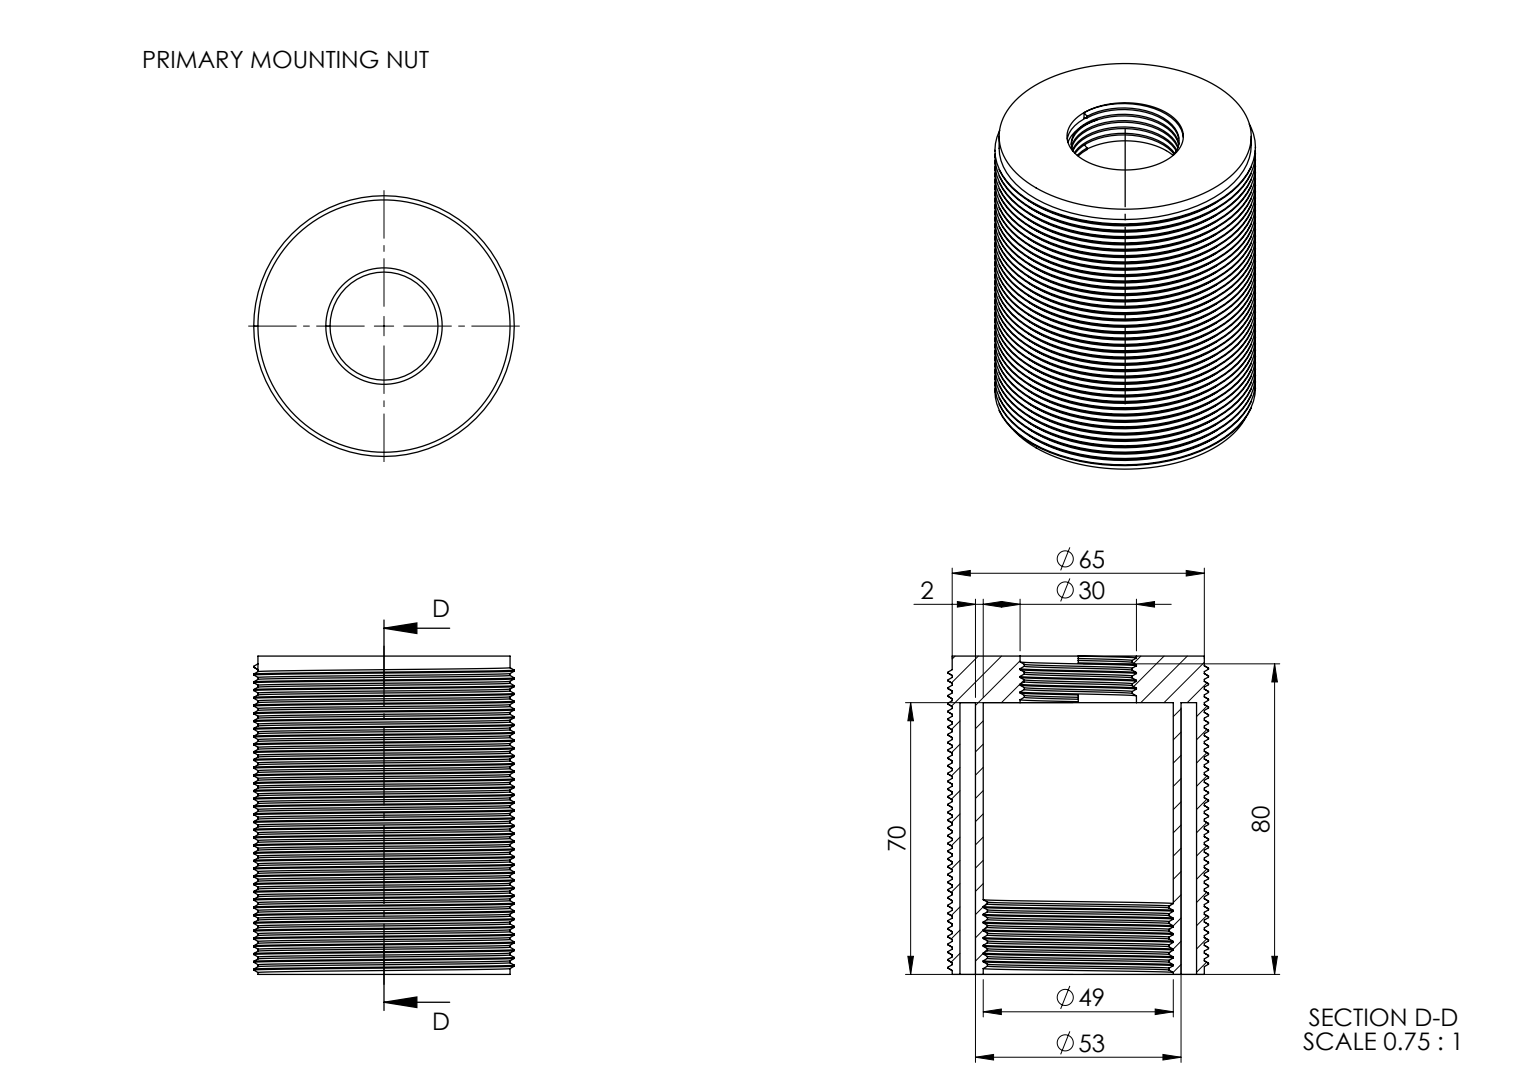
ISO-10303-21;
HEADER;
FILE_DESCRIPTION (('STEP AP214'),
    '1' );
FILE_NAME ('primary mounting nut.step',
    '2026-10-02T18:08:48',
    ( '' ),
    ( '' ),
    'SwSTEP 2.0',
    'SolidWorks 2026',
    '' );
FILE_SCHEMA (( 'AUTOMOTIVE_DESIGN' ));
ENDSEC;

DATA;
#4=ORIENTED_EDGE ( 'NONE', *, *, #32426, .T. ) ;
#10=CARTESIAN_POINT ( 'NONE',  ( -2.162160676586881955E-15, 52.87500000273119838, -35.31076352940723240 ) ) ;
#11=CARTESIAN_POINT ( 'NONE',  ( -2.092463501923844636E-15, 58.00000000546235412, -34.17252228774368916 ) ) ;
#14=CARTESIAN_POINT ( 'NONE',  ( -2.162160676586881955E-15, 42.62500000273119838, -35.31076352940723240 ) ) ;
#15=CARTESIAN_POINT ( 'NONE',  ( -4.635254915624208216, 72.40000000000001990, 14.26584774442730463 ) ) ;
#16=CARTESIAN_POINT ( 'NONE',  ( 33.58253175000000113, 68.47500000273119269, -10.91162601494193751 ) ) ;
#21=CARTESIAN_POINT ( 'NONE',  ( 6.277390505771533514E-15, 44.49999999999999289, 34.17252228774368916 ) ) ;
#23=CARTESIAN_POINT ( 'NONE',  ( -10.37757302488624411, 12.97500000273119092, -31.93888565452638417 ) ) ;
#27=CARTESIAN_POINT ( 'NONE',  ( 15.00000000000000355, 75.15000000546237402, 4.873795443493592394 ) ) ;
#28=CARTESIAN_POINT ( 'NONE',  ( 0.000000000000000000, 82.00000000000001421, 0.000000000000000000 ) ) ;
#30=EDGE_LOOP ( 'NONE', ( #10708, #16576, #32789, #18480 ) ) ;
#33=EDGE_CURVE ( 'NONE', #10375, #21334, #32773, .T. ) ;
#41=( BOUNDED_CURVE ( )  B_SPLINE_CURVE ( 2, ( #27655, #11863, #29882, #19433, #17198, #32453, #30382, #1391, #9453, #17026, #24905, #17535, #22341 ),
 .UNSPECIFIED., .F., .T. ) 
 B_SPLINE_CURVE_WITH_KNOTS ( ( 3, 2, 2, 2, 2, 2, 3 ),
 ( 0.2756410256410256610, 0.2769230769230769384, 0.2794871794871794934, 0.2820512820512820484, 0.2846153846153846034, 0.2871794871794871584, 0.2884615384615384914 ),
 .UNSPECIFIED. ) 
 CURVE ( )  GEOMETRIC_REPRESENTATION_ITEM ( )  RATIONAL_B_SPLINE_CURVE ( ( 0.9755282581475768211, 0.9755282581475768211, 1.000000000000000000, 0.9510565162951535312, 1.000000000000000000, 0.9510565162951535312, 1.000000000000000000, 0.9510565162951535312, 1.000000000000000000, 0.9510565162951535312, 1.000000000000000000, 0.9755282581475762660, 0.9755282581475768211 ) ) 
 REPRESENTATION_ITEM ( '' )  );
#43=CARTESIAN_POINT ( 'NONE',  ( 27.16883889988623935, 38.32500000273120122, -19.73931689729374384 ) ) ;
#46=CARTESIAN_POINT ( 'NONE',  ( -5.147494310547430452, 2.051254287009222299, -32.49999999999999289 ) ) ;
#49=CARTESIAN_POINT ( 'NONE',  ( -12.13525491562420910, 70.45000000546237118, 8.816778784387098611 ) ) ;
#51=CARTESIAN_POINT ( 'NONE',  ( 10.37757302488624056, 76.77500000273118985, -31.93888565452638417 ) ) ;
#57=CARTESIAN_POINT ( 'NONE',  ( -2.162160676586881955E-15, 60.62500000273117706, -35.31076352940723240 ) ) ;
#59=CARTESIAN_POINT ( 'NONE',  ( -5.147494310547423346, 66.94874572391552192, 32.50000000000000000 ) ) ;
#60=CARTESIAN_POINT ( 'NONE',  ( 14.47279130897151767, 8.824999997268804464, 19.92008829642072953 ) ) ;
#61=CARTESIAN_POINT ( 'NONE',  ( 27.16883889988624290, 1.925000002731186433, 19.73931689729373673 ) ) ;
#62=CARTESIAN_POINT ( 'NONE',  ( -1.778240108872766143E-15, 8.000000005462370112, -32.49999999999999289 ) ) ;
#65=CARTESIAN_POINT ( 'NONE',  ( -15.00000000000000000, 80.25000000546239676, 0.000000000000000000 ) ) ;
#67=CARTESIAN_POINT ( 'NONE',  ( -5.147494310547423346, 4.448745718453162468, 32.50000000000000000 ) ) ;
#71=CARTESIAN_POINT ( 'NONE',  ( 9.270509831248423538, 73.55000000546237970, -12.75976212528059861 ) ) ;
#73=CARTESIAN_POINT ( 'NONE',  ( 6.486482029760649416E-15, 29.62500000273120193, 35.31076352940723240 ) ) ;
#75=AXIS2_PLACEMENT_3D ( 'NONE', #28014, #5016, #30577 ) ;
#77=CARTESIAN_POINT ( 'NONE',  ( -2.162160676586882350E-15, 12.87500000273117884, -35.31076352940722529 ) ) ;
#78=PRODUCT_DEFINITION ( 'UNKNOWN', '', #3307, #996 ) ;
#79=CARTESIAN_POINT ( 'NONE',  ( -10.04305231718579172, 63.59999999999998721, -30.90933677959248982 ) ) ;
#81=CARTESIAN_POINT ( 'NONE',  ( -27.16883889988623935, 75.32500000273117280, 19.73931689729374739 ) ) ;
#82=CARTESIAN_POINT ( 'NONE',  ( 3.880418787951153803, 7.551254281546842861, 24.49999999999999645 ) ) ;
#84=CARTESIAN_POINT ( 'NONE',  ( 1.507698388325705758E-15, 17.12499999726880517, -24.62258325217400312 ) ) ;
#85=CARTESIAN_POINT ( 'NONE',  ( 33.58253175000000113, 58.12500000273118417, -4.112674001490185761E-15 ) ) ;
#87=ORIENTED_EDGE ( 'NONE', *, *, #10321, .T. ) ;
#89=CARTESIAN_POINT ( 'NONE',  ( 33.58253175000000113, 6.225000002731185589, -10.91162601494193574 ) ) ;
#90=CARTESIAN_POINT ( 'NONE',  ( -7.236395654485763274, 16.52499999726880731, 22.27133577429736633 ) ) ;
#92=EDGE_LOOP ( 'NONE', ( #2130, #17184, #1564 ) ) ;
#94=ORIENTED_EDGE ( 'NONE', *, *, #21026, .F. ) ;
#98=CARTESIAN_POINT ( 'NONE',  ( -20.75514604977248112, 77.42500000273119554, 28.56700777964554661 ) ) ;
#100=CARTESIAN_POINT ( 'NONE',  ( 1.577395562988744260E-15, 2.500000000000008882, -25.76082449383753925 ) ) ;
#101=CARTESIAN_POINT ( 'NONE',  ( 27.16883889988623935, 12.57500000273120655, -19.73931689729374384 ) ) ;
#102=CARTESIAN_POINT ( 'NONE',  ( 26.29305231718578995, 59.20000000000000284, -19.10302069950538240 ) ) ;
#103=CARTESIAN_POINT ( 'NONE',  ( 10.04305231718578817, 73.90000000546237402, -30.90933677959249337 ) ) ;
#105=CARTESIAN_POINT ( 'NONE',  ( -11.25946833292375793, 75.57500000273120122, 8.180482586598737171 ) ) ;
#107=CARTESIAN_POINT ( 'NONE',  ( 0.000000000000000000, 82.00000000000001421, 0.000000000000000000 ) ) ;
#108=CARTESIAN_POINT ( 'NONE',  ( -24.50000000000000000, 12.90000000000000036, -7.960532557706207157 ) ) ;
#109=CARTESIAN_POINT ( 'NONE',  ( 32.50000000000000711, 4.899999999999989697, 10.55989012756945122 ) ) ;
#112=CARTESIAN_POINT ( 'NONE',  ( 27.16883889988624290, 47.92500000273120264, 19.73931689729373673 ) ) ;
#114=CARTESIAN_POINT ( 'NONE',  ( -27.16883889988623935, 33.57500000273120122, 19.73931689729374739 ) ) ;
#117=CARTESIAN_POINT ( 'NONE',  ( 5.147494310547434893, 15.05125428700922541, 32.49999999999999289 ) ) ;
#118=CARTESIAN_POINT ( 'NONE',  ( -1.778240108872766143E-15, 22.00000000546237899, -32.49999999999999289 ) ) ;
#121=DIRECTION ( 'NONE',  ( -0.000000000000000000, 1.000000000000000000, -0.000000000000000000 ) ) ;
#124=CARTESIAN_POINT ( 'NONE',  ( -10.04305231718578462, 40.39999999999999147, 30.90933677959249337 ) ) ;
#127=CARTESIAN_POINT ( 'NONE',  ( 5.779280353836490358E-15, 12.49999999999999112, 32.49999999999999289 ) ) ;
#128=CARTESIAN_POINT ( 'NONE',  ( 10.37757302488624056, 26.52500000273119696, -31.93888565452638417 ) ) ;
#132=EDGE_CURVE ( 'NONE', #774, #12058, #32938, .T. ) ;
#138=CARTESIAN_POINT ( 'NONE',  ( -23.41746825000000243, 1.524999997268801755, -7.608796670333730638 ) ) ;
#139=CARTESIAN_POINT ( 'NONE',  ( 33.58253175000000113, 32.37500000273119127, -4.112674001490185761E-15 ) ) ;
#140=CARTESIAN_POINT ( 'NONE',  ( -32.50000000000000000, 36.40000000546236691, -10.55989012756945478 ) ) ;
#141=( BOUNDED_CURVE ( )  B_SPLINE_CURVE ( 2, ( #20409, #30859, #4610, #33262, #20067, #17493, #25204, #17837, #11988, #19888, #1681, #4780, #33084 ),
 .UNSPECIFIED., .F., .T. ) 
 B_SPLINE_CURVE_WITH_KNOTS ( ( 3, 2, 2, 2, 2, 2, 3 ),
 ( 0.2243589743589743668, 0.2256410256410256443, 0.2282051282051281993, 0.2307692307692307820, 0.2333333333333333370, 0.2358974358974358920, 0.2371794871794871973 ),
 .UNSPECIFIED. ) 
 CURVE ( )  GEOMETRIC_REPRESENTATION_ITEM ( )  RATIONAL_B_SPLINE_CURVE ( ( 0.9755282581475768211, 0.9755282581475768211, 1.000000000000000000, 0.9510565162951535312, 1.000000000000000000, 0.9510565162951535312, 1.000000000000000000, 0.9510565162951535312, 1.000000000000000000, 0.9510565162951535312, 1.000000000000000000, 0.9755282581475764880, 0.9755282581475768211 ) ) 
 REPRESENTATION_ITEM ( '' )  );
#144=CARTESIAN_POINT ( 'NONE',  ( 20.08610463437158344, 76.69999999999998863, 27.64615127144129403 ) ) ;
#145=CARTESIAN_POINT ( 'NONE',  ( 27.16883889988623935, 50.57500000273118701, -19.73931689729374384 ) ) ;
#148=CARTESIAN_POINT ( 'NONE',  ( -32.50000000000000000, 18.09999999999998010, 10.55989012756946366 ) ) ;
#150=CARTESIAN_POINT ( 'NONE',  ( 20.75514604977248467, 68.42500000273120975, -28.56700777964554305 ) ) ;
#151=CARTESIAN_POINT ( 'NONE',  ( -32.50000000000000000, 78.10000000000002274, 10.55989012756946366 ) ) ;
#153=CARTESIAN_POINT ( 'NONE',  ( 27.16883889988623935, 56.57500000273118701, -19.73931689729374384 ) ) ;
#154=CARTESIAN_POINT ( 'NONE',  ( 20.08610463437158344, 72.70000000000000284, 27.64615127144129403 ) ) ;
#155=CARTESIAN_POINT ( 'NONE',  ( -10.37757302488623701, 13.52500000273118630, 31.93888565452638417 ) ) ;
#158=AXIS2_PLACEMENT_3D ( 'NONE', #33870, #18769, #28713 ) ;
#159=CARTESIAN_POINT ( 'NONE',  ( 33.58253175000000113, 2.475000002731187809, -10.91162601494193574 ) ) ;
#167=LINE ( 'NONE', #25929, #20571 ) ;
#169=CARTESIAN_POINT ( 'NONE',  ( -23.41746825000000243, 8.024999997268801977, -7.608796670333730638 ) ) ;
#170=CARTESIAN_POINT ( 'NONE',  ( 10.04305231718578817, 69.90000000546237402, -30.90933677959249337 ) ) ;
#179=CARTESIAN_POINT ( 'NONE',  ( -33.58253175000000113, 53.37500000273118417, 0.000000000000000000 ) ) ;
#180=CARTESIAN_POINT ( 'NONE',  ( -20.08610463437156923, 54.80000000546237260, 27.64615127144130113 ) ) ;
#182=DIRECTION ( 'NONE',  ( -0.000000000000000000, -1.000000000000000000, -0.000000000000000000 ) ) ;
#183=CARTESIAN_POINT ( 'NONE',  ( 6.486482029760649416E-15, 41.62500000273116996, 35.31076352940723240 ) ) ;
#184=CARTESIAN_POINT ( 'NONE',  ( 12.13525491562420910, 73.45000000546237118, -8.816778784387098611 ) ) ;
#185=CARTESIAN_POINT ( 'NONE',  ( 10.37757302488624056, 68.77500000273117564, -31.93888565452638417 ) ) ;
#186=CARTESIAN_POINT ( 'NONE',  ( -32.50000000000000000, 0.6000000054623972900, 10.55989012756946366 ) ) ;
#190=CARTESIAN_POINT ( 'NONE',  ( 32.50000000000000000, 44.99999999999998579, -3.980102097228898626E-15 ) ) ;
#192=CARTESIAN_POINT ( 'NONE',  ( 20.75514604977249178, 14.07500000273119944, 28.56700777964553950 ) ) ;
#193=CYLINDRICAL_SURFACE ( 'NONE', #6349, 32.50000000000000000 ) ;
#195=CARTESIAN_POINT ( 'NONE',  ( -4.300734207923759378, 74.97500000273119269, -13.23629886949340495 ) ) ;
#197=CARTESIAN_POINT ( 'NONE',  ( -1.778240108872766143E-15, 21.50000000000000000, -32.49999999999999289 ) ) ;
#200=FACE_OUTER_BOUND ( 'NONE', #19419, .T. ) ;
#211=CARTESIAN_POINT ( 'NONE',  ( 33.58253175000000113, 40.12500000273119838, -4.112674001490185761E-15 ) ) ;
#216=ORIENTED_EDGE ( 'NONE', *, *, #8928, .T. ) ;
#219=CARTESIAN_POINT ( 'NONE',  ( 33.58253175000000823, 72.27500000273118985, 10.91162601494192863 ) ) ;
#223=EDGE_CURVE ( 'NONE', #23252, #23800, #3174, .T. ) ;
#224=EDGE_LOOP ( 'NONE', ( #22388, #1047, #13319, #25437 ) ) ;
#226=CARTESIAN_POINT ( 'NONE',  ( 27.16883889988624290, 61.92500000273118133, 19.73931689729373673 ) ) ;
#230=CARTESIAN_POINT ( 'NONE',  ( 23.41746824999999887, 7.224999997268826135, -7.608796670333727974 ) ) ;
#232=CARTESIAN_POINT ( 'NONE',  ( 33.58253175000000823, 4.025000002731196957, 10.91162601494192863 ) ) ;
#233=CARTESIAN_POINT ( 'NONE',  ( -27.16883889988624290, 31.17500000273118488, -19.73931689729374028 ) ) ;
#234=CARTESIAN_POINT ( 'NONE',  ( 32.50000000000000000, 5.600000005462384856, -10.55989012756945833 ) ) ;
#236=CARTESIAN_POINT ( 'NONE',  ( -33.58253175000000113, 79.37500000273118417, 0.000000000000000000 ) ) ;
#238=CARTESIAN_POINT ( 'NONE',  ( -26.29305231718579350, 31.79999999999999361, -19.10302069950537884 ) ) ;
#239=CARTESIAN_POINT ( 'NONE',  ( -1.778240108872766143E-15, 69.49999999999998579, -32.49999999999999289 ) ) ;
#243=CARTESIAN_POINT ( 'NONE',  ( -4.300734207923755825, 79.27500000273118985, 13.23629886949340673 ) ) ;
#246=CARTESIAN_POINT ( 'NONE',  ( 10.37757302488624767, 21.72500000273119980, 31.93888565452638417 ) ) ;
#249=CARTESIAN_POINT ( 'NONE',  ( -10.37757302488624411, 12.97500000273119092, -31.93888565452638417 ) ) ;
#250=CARTESIAN_POINT ( 'NONE',  ( -20.08610463437156923, 64.29999999999996874, 27.64615127144130113 ) ) ;
#252=CARTESIAN_POINT ( 'NONE',  ( 27.16883889988623935, 70.32500000273117280, -19.73931689729374384 ) ) ;
#255=CARTESIAN_POINT ( 'NONE',  ( 15.00000000000000355, 79.15000000546238823, 4.873795443493592394 ) ) ;
#256=CARTESIAN_POINT ( 'NONE',  ( 20.75514604977249178, 55.82500000273118701, 28.56700777964553950 ) ) ;
#260=CARTESIAN_POINT ( 'NONE',  ( 20.75514604977248467, 2.425000002731188875, -28.56700777964554305 ) ) ;
#261=CARTESIAN_POINT ( 'NONE',  ( 23.41746825000000243, 19.02499999726880375, 7.608796670333735079 ) ) ;
#263=ORIENTED_EDGE ( 'NONE', *, *, #29784, .F. ) ;
#268=CARTESIAN_POINT ( 'NONE',  ( 10.04305231718579705, 11.10000000546237864, 30.90933677959248982 ) ) ;
#270=CARTESIAN_POINT ( 'NONE',  ( -32.50000000000000000, 72.00000000000001421, 0.000000000000000000 ) ) ;
#272=CARTESIAN_POINT ( 'NONE',  ( 7.570916362186213000, 0.4000000000000114575, -23.30088464923126423 ) ) ;
#273=CARTESIAN_POINT ( 'NONE',  ( -20.75514604977248112, 11.67500000273118843, 28.56700777964554661 ) ) ;
#274=CARTESIAN_POINT ( 'NONE',  ( 32.50000000000000711, 60.89999999999999147, 10.55989012756945122 ) ) ;
#275=CARTESIAN_POINT ( 'NONE',  ( -11.25946833292375793, 77.07500000273121543, 8.180482586598737171 ) ) ;
#276=CARTESIAN_POINT ( 'NONE',  ( 32.50000000000000711, 73.40000000546235981, 10.55989012756945122 ) ) ;
#278=CARTESIAN_POINT ( 'NONE',  ( 13.91746825000000065, 76.27500000273118985, 4.522059556121114987 ) ) ;
#282=CARTESIAN_POINT ( 'NONE',  ( 4.445600272181915325E-13, 15.49999999999999822, -32.50000000000000000 ) ) ;
#283=CARTESIAN_POINT ( 'NONE',  ( -20.08610463437156923, 4.300000000000009592, 27.64615127144130113 ) ) ;
#286=CARTESIAN_POINT ( 'NONE',  ( -10.37757302488623701, 43.52500000273118275, 31.93888565452638417 ) ) ;
#289=CARTESIAN_POINT ( 'NONE',  ( -27.16883889988624290, 35.17500000273118843, -19.73931689729374028 ) ) ;
#290=CARTESIAN_POINT ( 'NONE',  ( 32.50000000000000000, 24.99999999999999289, -3.980102097228898626E-15 ) ) ;
#292=CARTESIAN_POINT ( 'NONE',  ( -19.82091636218621389, 9.199999999999985079, 14.40073868116558842 ) ) ;
#297=CARTESIAN_POINT ( 'NONE',  ( 14.47279130897151944, 0.9249999972688209837, -19.92008829642072598 ) ) ;
#298=CARTESIAN_POINT ( 'NONE',  ( -32.50000000000000000, 39.89999999999999147, -10.55989012756945300 ) ) ;
#301=DIRECTION ( 'NONE',  ( 0.000000000000000000, 0.000000000000000000, -1.000000000000000000 ) ) ;
#302=CARTESIAN_POINT ( 'NONE',  ( -20.75514604977248112, 21.42500000273119909, 28.56700777964554661 ) ) ;
#304=EDGE_LOOP ( 'NONE', ( #18948, #25383, #642, #30344 ) ) ;
#306=ORIENTED_EDGE ( 'NONE', *, *, #17553, .T. ) ;
#310=ORIENTED_EDGE ( 'NONE', *, *, #3089, .T. ) ;
#311=DIRECTION ( 'NONE',  ( -0.000000000000000000, -1.000000000000000000, -0.000000000000000000 ) ) ;
#312=CARTESIAN_POINT ( 'NONE',  ( 20.75514604977248467, 26.67500000273118133, -28.56700777964554305 ) ) ;
#313=CARTESIAN_POINT ( 'NONE',  ( -32.50000000000000000, 36.50000000546238255, 0.000000000000000000 ) ) ;
#315=DIRECTION ( 'NONE',  ( -0.000000000000000000, -1.000000000000000000, -0.000000000000000000 ) ) ;
#316=CARTESIAN_POINT ( 'NONE',  ( 5.779280353836490358E-15, 76.49999999999998579, 32.49999999999999289 ) ) ;
#317=CARTESIAN_POINT ( 'NONE',  ( 10.37757302488624767, 39.97500000273118559, 31.93888565452638417 ) ) ;
#319=ADVANCED_FACE ( 'NONE', ( #18042 ), #31233, .T. ) ;
#321=CARTESIAN_POINT ( 'NONE',  ( -32.50000000000000000, 23.90000000000000213, -10.55989012756945478 ) ) ;
#323=CARTESIAN_POINT ( 'NONE',  ( 27.16883889988623935, 68.32500000273117280, -19.73931689729374384 ) ) ;
#326=CARTESIAN_POINT ( 'NONE',  ( -2.162160676586882350E-15, 54.87500000273119838, -35.31076352940722529 ) ) ;
#329=CARTESIAN_POINT ( 'NONE',  ( 32.50000000000000000, 7.500000005462359454, -3.980102097228898626E-15 ) ) ;
#330=CARTESIAN_POINT ( 'NONE',  ( 20.75514604977249178, 11.82500000273118346, 28.56700777964553950 ) ) ;
#337=EDGE_CURVE ( 'NONE', #9595, #9120, #6660, .T. ) ;
#344=( BOUNDED_CURVE ( )  B_SPLINE_CURVE ( 2, ( #18329, #28774, #33583, #26207, #28942, #8342, #10762, #18832, #29443, #10593, #13679, #5610, #16585 ),
 .UNSPECIFIED., .F., .T. ) 
 B_SPLINE_CURVE_WITH_KNOTS ( ( 3, 2, 2, 2, 2, 2, 3 ),
 ( 0.2628205128205128305, 0.2641025641025641080, 0.2666666666666666630, 0.2692307692307692180, 0.2717948717948717730, 0.2743589743589743835, 0.2756410256410256610 ),
 .UNSPECIFIED. ) 
 CURVE ( )  GEOMETRIC_REPRESENTATION_ITEM ( )  RATIONAL_B_SPLINE_CURVE ( ( 0.9755282581475768211, 0.9755282581475768211, 1.000000000000000000, 0.9510565162951535312, 1.000000000000000000, 0.9510565162951535312, 1.000000000000000000, 0.9510565162951535312, 1.000000000000000000, 0.9510565162951535312, 1.000000000000000000, 0.9755282581475768211, 0.9755282581475768211 ) ) 
 REPRESENTATION_ITEM ( '' )  );
#345=CARTESIAN_POINT ( 'NONE',  ( -2.092463501923844636E-15, 68.00000000546236834, -34.17252228774368916 ) ) ;
#349=CYLINDRICAL_SURFACE ( 'NONE', #12439, 32.50000000000000000 ) ;
#354=CARTESIAN_POINT ( 'NONE',  ( -10.04305231718579172, 35.59999999999999432, -30.90933677959248982 ) ) ;
#355=CARTESIAN_POINT ( 'NONE',  ( 6.486482029760649416E-15, 51.87500000273119127, 35.31076352940723240 ) ) ;
#356=CARTESIAN_POINT ( 'NONE',  ( -20.08610463437157989, 58.20000000546238539, -27.64615127144129758 ) ) ;
#358=CARTESIAN_POINT ( 'NONE',  ( -20.75514604977248823, 32.82500000273118701, -28.56700777964554305 ) ) ;
#359=CARTESIAN_POINT ( 'NONE',  ( 5.779280353836490358E-15, 54.49999999999999289, 32.49999999999999289 ) ) ;
#360=CARTESIAN_POINT ( 'NONE',  ( 10.37757302488624056, 60.77500000273117564, -31.93888565452638417 ) ) ;
#361=( LENGTH_UNIT ( ) NAMED_UNIT ( * ) SI_UNIT ( .MILLI., .METRE. ) );
#364=CARTESIAN_POINT ( 'NONE',  ( -10.04305231718579172, 37.59999999999999432, -30.90933677959248982 ) ) ;
#366=CARTESIAN_POINT ( 'NONE',  ( 27.16883889988624290, 8.175000002731191984, 19.73931689729373673 ) ) ;
#367=CARTESIAN_POINT ( 'NONE',  ( 32.50000000000000711, 35.40000000546237402, 10.55989012756945122 ) ) ;
#369=CARTESIAN_POINT ( 'NONE',  ( -4.300734207923759378, 72.97500000273119269, -13.23629886949340495 ) ) ;
#370=CARTESIAN_POINT ( 'NONE',  ( -10.37757302488623701, 71.77500000273117564, 31.93888565452638417 ) ) ;
#382=AXIS2_PLACEMENT_3D ( 'NONE', #6259, #3850, #8998 ) ;
#385=CARTESIAN_POINT ( 'NONE',  ( -10.04305231718578462, 56.90000000546238823, 30.90933677959249337 ) ) ;
#386=CARTESIAN_POINT ( 'NONE',  ( 20.75514604977248467, 40.42500000273118133, -28.56700777964554305 ) ) ;
#390=VERTEX_POINT ( 'NONE', #7896 ) ;
#392=CARTESIAN_POINT ( 'NONE',  ( 5.147494310547426899, 51.44874571845315359, -32.50000000000000000 ) ) ;
#394=CARTESIAN_POINT ( 'NONE',  ( 33.58253175000000113, 68.37500000273119838, -4.112674001490185761E-15 ) ) ;
#398=ORIENTED_EDGE ( 'NONE', *, *, #26853, .F. ) ;
#399=CARTESIAN_POINT ( 'NONE',  ( 33.58253175000000113, 60.12500000273119127, -4.112674001490185761E-15 ) ) ;
#402=CARTESIAN_POINT ( 'NONE',  ( 26.29305231718578995, 19.70000000546237473, -19.10302069950538240 ) ) ;
#403=CARTESIAN_POINT ( 'NONE',  ( 24.50000000000000355, 16.09999999999998366, -7.960532557706203605 ) ) ;
#404=CARTESIAN_POINT ( 'NONE',  ( -18.94512977948575738, 7.924999997268811214, -13.76444248337723231 ) ) ;
#405=CARTESIAN_POINT ( 'NONE',  ( 10.37757302488624767, 29.97500000273117848, 31.93888565452638417 ) ) ;
#409=CARTESIAN_POINT ( 'NONE',  ( 11.25946833292375793, 78.07500000273121543, -8.180482586598735395 ) ) ;
#410=CARTESIAN_POINT ( 'NONE',  ( 5.779280353836490358E-15, 4.500000000000003553, 32.49999999999999289 ) ) ;
#414=CARTESIAN_POINT ( 'NONE',  ( -8.960552108402742093E-16, 78.37500000273116996, -14.63369212191046387 ) ) ;
#416=CARTESIAN_POINT ( 'NONE',  ( 20.75514604977248467, 24.42500000273119554, -28.56700777964554305 ) ) ;
#419=CARTESIAN_POINT ( 'NONE',  ( -10.37757302488623701, 17.77500000273118985, 31.93888565452638417 ) ) ;
#421=CARTESIAN_POINT ( 'NONE',  ( 10.37757302488624056, 72.52500000273120406, -31.93888565452638417 ) ) ;
#422=CARTESIAN_POINT ( 'NONE',  ( 32.50000000000000000, 3.600000005462360431, -10.55989012756945833 ) ) ;
#423=EDGE_CURVE ( 'NONE', #5175, #29096, #19145, .T. ) ;
#425=CYLINDRICAL_SURFACE ( 'NONE', #30310, 32.50000000000000000 ) ;
#426=CARTESIAN_POINT ( 'NONE',  ( 33.58253175000000823, 58.02500000273117564, 10.91162601494192685 ) ) ;
#427=EDGE_CURVE ( 'NONE', #23800, #20505, #26160, .T. ) ;
#433=CARTESIAN_POINT ( 'NONE',  ( 23.41746825000000243, 2.724999997268822138, -7.608796670333727974 ) ) ;
#435=ORIENTED_EDGE ( 'NONE', *, *, #9249, .F. ) ;
#437=CARTESIAN_POINT ( 'NONE',  ( -10.04305231718579172, 42.10000000546237686, -30.90933677959248982 ) ) ;
#438=VERTEX_POINT ( 'NONE', #27093 ) ;
#440=CARTESIAN_POINT ( 'NONE',  ( 32.50000000000000000, 11.60000000546236976, -10.55989012756945833 ) ) ;
#443=CARTESIAN_POINT ( 'NONE',  ( -15.14183272437241889, 0.7000000000000070610, -20.84094480462497856 ) ) ;
#444=CARTESIAN_POINT ( 'NONE',  ( 33.58253175000000113, 10.47500000273119802, -10.91162601494193751 ) ) ;
#445=( BOUNDED_CURVE ( )  B_SPLINE_CURVE ( 2, ( #6317, #10970, #27082, #6487, #8556, #26754, #24016, #26913, #19534, #11627, #31888, #19040, #21445 ),
 .UNSPECIFIED., .F., .T. ) 
 B_SPLINE_CURVE_WITH_KNOTS ( ( 3, 2, 2, 2, 2, 2, 3 ),
 ( 0.5192307692307692735, 0.5205128205128205510, 0.5230769230769231060, 0.5256410256410256610, 0.5282051282051282159, 0.5307692307692307709, 0.5320512820512820484 ),
 .UNSPECIFIED. ) 
 CURVE ( )  GEOMETRIC_REPRESENTATION_ITEM ( )  RATIONAL_B_SPLINE_CURVE ( ( 0.9755282581475768211, 0.9755282581475768211, 1.000000000000000000, 0.9510565162951535312, 1.000000000000000000, 0.9510565162951535312, 1.000000000000000000, 0.9510565162951535312, 1.000000000000000000, 0.9510565162951535312, 1.000000000000000000, 0.9755282581475768211, 0.9755282581475768211 ) ) 
 REPRESENTATION_ITEM ( '' )  );
#446=CARTESIAN_POINT ( 'NONE',  ( 26.29305231718579350, 60.79999999999999005, 19.10302069950537529 ) ) ;
#447=CARTESIAN_POINT ( 'NONE',  ( 11.25946833292375793, 78.07500000273121543, -8.180482586598735395 ) ) ;
#448=CARTESIAN_POINT ( 'NONE',  ( 3.000384657911015469E-15, 0.000000000000000000, -24.50000000000000000 ) ) ;
#450=CARTESIAN_POINT ( 'NONE',  ( -11.25946833292375793, 77.57500000273121543, 8.180482586598737171 ) ) ;
#453=LINE ( 'NONE', #5276, #30284 ) ;
#454=CARTESIAN_POINT ( 'NONE',  ( 32.50000000000000000, 65.10000000000000853, -10.55989012756945833 ) ) ;
#455=CARTESIAN_POINT ( 'NONE',  ( -33.58253175000000113, 79.37500000273118417, 0.000000000000000000 ) ) ;
#458=CARTESIAN_POINT ( 'NONE',  ( -10.37757302488624411, 44.72500000273119269, -31.93888565452638417 ) ) ;
#461=CARTESIAN_POINT ( 'NONE',  ( 20.75514604977249178, 36.07500000273117990, 28.56700777964553950 ) ) ;
#462=CARTESIAN_POINT ( 'NONE',  ( 20.08610463437157279, 23.80000000546236194, -27.64615127144129758 ) ) ;
#465=CARTESIAN_POINT ( 'NONE',  ( -32.50000000000000000, 44.40000000546238113, -10.55989012756945300 ) ) ;
#468=CARTESIAN_POINT ( 'NONE',  ( -14.47279130897152299, 5.924999997268808549, 19.92008829642072243 ) ) ;
#471=CARTESIAN_POINT ( 'NONE',  ( -15.00000000000000000, 76.25000000546239676, 0.000000000000000000 ) ) ;
#472=CARTESIAN_POINT ( 'NONE',  ( 20.75514604977248467, 20.42500000273120264, -28.56700777964554305 ) ) ;
#480=EDGE_CURVE ( 'NONE', #3734, #23926, #32237, .T. ) ;
#481=ORIENTED_EDGE ( 'NONE', *, *, #22056, .T. ) ;
#482=CARTESIAN_POINT ( 'NONE',  ( -18.94512977948576093, 1.824999997268816898, 13.76444248337722698 ) ) ;
#483=CARTESIAN_POINT ( 'NONE',  ( -20.75514604977248112, 25.67500000273118488, 28.56700777964554661 ) ) ;
#484=( BOUNDED_CURVE ( )  B_SPLINE_CURVE ( 2, ( #8782, #6212, #1213, #29708, #6384, #19601, #24574, #27149, #3642, #11694, #1046, #11526, #32454 ),
 .UNSPECIFIED., .F., .F. ) 
 B_SPLINE_CURVE_WITH_KNOTS ( ( 3, 2, 2, 2, 2, 2, 3 ),
 ( 0.9166666666666666297, 0.9222222222222222765, 0.9333333333333333481, 0.9444444444444444198, 0.9555555555555556024, 0.9666666666666666741, 0.9722222222222222099 ),
 .UNSPECIFIED. ) 
 CURVE ( )  GEOMETRIC_REPRESENTATION_ITEM ( )  RATIONAL_B_SPLINE_CURVE ( ( 0.9755282581475768211, 0.9755282581475765991, 1.000000000000000000, 0.9510565162951535312, 1.000000000000000000, 0.9510565162951535312, 1.000000000000000000, 0.9510565162951535312, 1.000000000000000000, 0.9510565162951535312, 1.000000000000000000, 0.9755282581475768211, 0.9755282581475768211 ) ) 
 REPRESENTATION_ITEM ( '' )  );
#485=CARTESIAN_POINT ( 'NONE',  ( -26.29305231718579350, 32.30000000546237260, -19.10302069950537884 ) ) ;
#487=CARTESIAN_POINT ( 'NONE',  ( 26.29305231718579350, 52.80000000000001137, 19.10302069950537529 ) ) ;
#488=CARTESIAN_POINT ( 'NONE',  ( -24.50000000000000711, 11.09999999999999787, 7.960532557706201828 ) ) ;
#489=CARTESIAN_POINT ( 'NONE',  ( 10.37757302488624056, 44.77500000273118275, -31.93888565452638417 ) ) ;
#491=CARTESIAN_POINT ( 'NONE',  ( -2.092463501923844636E-15, 21.49999999999998934, -34.17252228774368916 ) ) ;
#493=CARTESIAN_POINT ( 'NONE',  ( 20.75514604977248467, 64.42500000273116711, -28.56700777964554305 ) ) ;
#496=CARTESIAN_POINT ( 'NONE',  ( 10.37757302488624056, 50.77500000273118985, -31.93888565452638417 ) ) ;
#499=CARTESIAN_POINT ( 'NONE',  ( -27.16883889988623935, 5.325000002731172799, 19.73931689729374739 ) ) ;
#511=CARTESIAN_POINT ( 'NONE',  ( 1.093617666956751375E-13, 61.50000000000000000, -32.50000000000000711 ) ) ;
#513=CARTESIAN_POINT ( 'NONE',  ( -10.04305231718578462, 70.90000000546237402, 30.90933677959249337 ) ) ;
#521=CARTESIAN_POINT ( 'NONE',  ( -10.37757302488623701, 47.77500000273118985, 31.93888565452638417 ) ) ;
#522=CARTESIAN_POINT ( 'NONE',  ( -32.50000000000000000, 56.40000000546238113, -10.55989012756945478 ) ) ;
#524=CARTESIAN_POINT ( 'NONE',  ( 33.58253175000000113, 36.22500000273119980, -10.91162601494193751 ) ) ;
#525=CARTESIAN_POINT ( 'NONE',  ( 10.04305231718579705, 54.59999999999998010, 30.90933677959248982 ) ) ;
#526=CARTESIAN_POINT ( 'NONE',  ( -27.16883889988623935, 61.57500000273119412, 19.73931689729374739 ) ) ;
#530=CARTESIAN_POINT ( 'NONE',  ( -32.50000000000000000, 41.89999999999999147, -10.55989012756945478 ) ) ;
#532=CARTESIAN_POINT ( 'NONE',  ( -10.37757302488624411, 4.975000002731183812, -31.93888565452638417 ) ) ;
#533=CARTESIAN_POINT ( 'NONE',  ( 10.04305231718579705, 35.10000000546236976, 30.90933677959248982 ) ) ;
#534=LINE ( 'NONE', #11021, #18280 ) ;
#535=CARTESIAN_POINT ( 'NONE',  ( -27.16883889988624290, 71.17500000273119554, -19.73931689729374028 ) ) ;
#536=CARTESIAN_POINT ( 'NONE',  ( 0.000000000000000000, 80.00000000000001421, -32.50000000000000000 ) ) ;
#538=ORIENTED_EDGE ( 'NONE', *, *, #24194, .T. ) ;
#545=( BOUNDED_CURVE ( )  B_SPLINE_CURVE ( 2, ( #31536, #23134, #8029, #31023, #13353, #23827, #28284, #20753, #2715, #28961, #5457, #117, #10438 ),
 .UNSPECIFIED., .F., .T. ) 
 B_SPLINE_CURVE_WITH_KNOTS ( ( 3, 2, 2, 2, 2, 2, 3 ),
 ( 0.8012820512820513219, 0.8025641025641025994, 0.8051282051282051544, 0.8076923076923077094, 0.8102564102564102644, 0.8128205128205128194, 0.8141025641025640969 ),
 .UNSPECIFIED. ) 
 CURVE ( )  GEOMETRIC_REPRESENTATION_ITEM ( )  RATIONAL_B_SPLINE_CURVE ( ( 0.9755282581475768211, 0.9755282581475768211, 1.000000000000000000, 0.9510565162951535312, 1.000000000000000000, 0.9510565162951535312, 1.000000000000000000, 0.9510565162951535312, 1.000000000000000000, 0.9510565162951535312, 1.000000000000000000, 0.9755282581475768211, 0.9755282581475768211 ) ) 
 REPRESENTATION_ITEM ( '' )  );
#552=CARTESIAN_POINT ( 'NONE',  ( -2.162160676586882350E-15, 36.62500000273119127, -35.31076352940722529 ) ) ;
#558=CARTESIAN_POINT ( 'NONE',  ( -5.147494310547531704, 50.94874572391553613, 32.49999999999996447 ) ) ;
#560=CARTESIAN_POINT ( 'NONE',  ( -27.16883889988623935, 69.57500000273120122, 19.73931689729374739 ) ) ;
#561=ORIENTED_EDGE ( 'NONE', *, *, #13358, .F. ) ;
#564=VERTEX_POINT ( 'NONE', #663 ) ;
#565=DIRECTION ( 'NONE',  ( -0.000000000000000000, -1.000000000000000000, -0.000000000000000000 ) ) ;
#566=CARTESIAN_POINT ( 'NONE',  ( 33.58253175000000113, 56.22500000273117138, -10.91162601494193751 ) ) ;
#568=CARTESIAN_POINT ( 'NONE',  ( 32.50000000000000711, 17.40000000546238823, 10.55989012756945122 ) ) ;
#569=CARTESIAN_POINT ( 'NONE',  ( 0.000000000000000000, 80.00000000000001421, -32.50000000000000000 ) ) ;
#570=CARTESIAN_POINT ( 'NONE',  ( -23.41746825000000243, 6.224999997268827912, 7.608796670333725309 ) ) ;
#571=CARTESIAN_POINT ( 'NONE',  ( 20.75514604977249178, 30.07500000273118701, 28.56700777964553950 ) ) ;
#572=CARTESIAN_POINT ( 'NONE',  ( 3.980102097228898626E-15, 80.00000000000001421, 32.50000000000000000 ) ) ;
#574=CARTESIAN_POINT ( 'NONE',  ( 13.91746824999999887, 77.87500000273116996, -1.704398294459741270E-15 ) ) ;
#575=CARTESIAN_POINT ( 'NONE',  ( 5.779280353836490358E-15, 8.500000000000000000, 32.49999999999999289 ) ) ;
#579=CARTESIAN_POINT ( 'NONE',  ( -8.960552108402742093E-16, 76.37500000273116996, -14.63369212191046387 ) ) ;
#581=CARTESIAN_POINT ( 'NONE',  ( 27.16883889988624290, 23.92500000273117777, 19.73931689729373673 ) ) ;
#584=CARTESIAN_POINT ( 'NONE',  ( -27.16883889988624290, 17.17500000273119909, -19.73931689729374028 ) ) ;
#586=CARTESIAN_POINT ( 'NONE',  ( 10.37757302488624767, 67.72500000273117848, 31.93888565452638417 ) ) ;
#587=LINE ( 'NONE', #26690, #24962 ) ;
#590=CARTESIAN_POINT ( 'NONE',  ( -33.58253175000000113, 55.22500000273117848, 10.91162601494193929 ) ) ;
#592=ORIENTED_EDGE ( 'NONE', *, *, #5855, .F. ) ;
#595=CARTESIAN_POINT ( 'NONE',  ( 1.507698388325705758E-15, 9.124999997268822938, -24.62258325217400312 ) ) ;
#597=ORIENTED_EDGE ( 'NONE', *, *, #28712, .F. ) ;
#599=CARTESIAN_POINT ( 'NONE',  ( -10.04305231718578462, 68.90000000546237402, 30.90933677959249337 ) ) ;
#601=VERTEX_POINT ( 'NONE', #830 ) ;
#603=CARTESIAN_POINT ( 'NONE',  ( 20.08610463437158344, 11.20000000546238184, 27.64615127144129403 ) ) ;
#604=CARTESIAN_POINT ( 'NONE',  ( -19.82091636218621034, 2.799999999999997158, -14.40073868116559552 ) ) ;
#605=CARTESIAN_POINT ( 'NONE',  ( -10.37757302488624411, 76.72500000273119269, -31.93888565452638417 ) ) ;
#607=CARTESIAN_POINT ( 'NONE',  ( -7.570916362186215665, 7.399999999999989697, 23.30088464923126423 ) ) ;
#608=CARTESIAN_POINT ( 'NONE',  ( -20.75514604977248823, 11.07500000273117813, -28.56700777964554305 ) ) ;
#610=CARTESIAN_POINT ( 'NONE',  ( 10.37757302488624056, 24.52500000273119696, -31.93888565452638417 ) ) ;
#611=CARTESIAN_POINT ( 'NONE',  ( -8.601468415847515203, 77.17500000273120975, 11.83890561707634959 ) ) ;
#613=AXIS2_PLACEMENT_3D ( 'NONE', #20476, #12571, #28521 ) ;
#615=AXIS2_PLACEMENT_3D ( 'NONE', #16459, #8052, #21610 ) ;
#616=CARTESIAN_POINT ( 'NONE',  ( -8.601468415847518756, 77.07500000273117280, -11.83890561707634781 ) ) ;
#622=CARTESIAN_POINT ( 'NONE',  ( -2.162160676586881955E-15, 42.62500000273119838, -35.31076352940723240 ) ) ;
#625=CARTESIAN_POINT ( 'NONE',  ( 33.58253175000000823, 34.27500000273116854, 10.91162601494192685 ) ) ;
#626=CARTESIAN_POINT ( 'NONE',  ( -1.778240108872766143E-15, 16.00000000546237899, -32.49999999999999289 ) ) ;
#632=CARTESIAN_POINT ( 'NONE',  ( 23.41746824999999887, 2.624999997268812280, 0.000000000000000000 ) ) ;
#636=CARTESIAN_POINT ( 'NONE',  ( -27.16883889988623935, 21.32500000273118701, 19.73931689729374739 ) ) ;
#639=ORIENTED_EDGE ( 'NONE', *, *, #18179, .T. ) ;
#641=( BOUNDED_CURVE ( )  B_SPLINE_CURVE ( 2, ( #9073, #30506, #22800, #33255, #4263, #16979, #33077, #4432, #7006, #20237, #14568, #27436, #17488 ),
 .UNSPECIFIED., .F., .F. ) 
 B_SPLINE_CURVE_WITH_KNOTS ( ( 3, 2, 2, 2, 2, 2, 3 ),
 ( 0.1602564102564102699, 0.1615384615384615474, 0.1641025641025641024, 0.1666666666666666574, 0.1692307692307692402, 0.1717948717948717952, 0.1730769230769230727 ),
 .UNSPECIFIED. ) 
 CURVE ( )  GEOMETRIC_REPRESENTATION_ITEM ( )  RATIONAL_B_SPLINE_CURVE ( ( 0.9755282581475768211, 0.9755282581475770431, 1.000000000000000000, 0.9510565162951535312, 1.000000000000000000, 0.9510565162951535312, 1.000000000000000000, 0.9510565162951535312, 1.000000000000000000, 0.9510565162951535312, 1.000000000000000000, 0.9755282581475768211, 0.9755282581475768211 ) ) 
 REPRESENTATION_ITEM ( '' )  );
#642=ORIENTED_EDGE ( 'NONE', *, *, #21531, .T. ) ;
#645=CARTESIAN_POINT ( 'NONE',  ( 20.08610463437158344, 38.69999999999999574, 27.64615127144129403 ) ) ;
#646=ORIENTED_EDGE ( 'NONE', *, *, #15565, .T. ) ;
#648=CARTESIAN_POINT ( 'NONE',  ( -20.75514604977248823, 27.07500000273119412, -28.56700777964554305 ) ) ;
#649=CARTESIAN_POINT ( 'NONE',  ( 32.50000000000000711, 31.40000000546238823, 10.55989012756945122 ) ) ;
#652=CARTESIAN_POINT ( 'NONE',  ( -5.147494310547423346, 54.94874572391552903, 32.50000000000000000 ) ) ;
#653=CARTESIAN_POINT ( 'NONE',  ( 4.635254915624212657, 72.59999999999999432, 14.26584774442730286 ) ) ;
#654=CARTESIAN_POINT ( 'NONE',  ( 33.58253175000000823, 44.27500000273120406, 10.91162601494192863 ) ) ;
#655=EDGE_CURVE ( 'NONE', #33572, #1522, #5309, .T. ) ;
#657=CARTESIAN_POINT ( 'NONE',  ( 32.50000000000000711, 18.90000000000001634, 10.55989012756945122 ) ) ;
#659=CARTESIAN_POINT ( 'NONE',  ( 20.75514604977248467, 62.42500000273118133, -28.56700777964554305 ) ) ;
#661=CARTESIAN_POINT ( 'NONE',  ( 20.75514604977248467, 54.67500000273119554, -28.56700777964554305 ) ) ;
#663=CARTESIAN_POINT ( 'NONE',  ( -8.891200544363830713E-16, 75.75000000546236834, -15.00000000000000000 ) ) ;
#664=CARTESIAN_POINT ( 'NONE',  ( -27.16883889988624290, 6.925000002731191096, -19.73931689729374028 ) ) ;
#667=CARTESIAN_POINT ( 'NONE',  ( -32.50000000000000000, 20.10000000000000497, 10.55989012756946366 ) ) ;
#671=CARTESIAN_POINT ( 'NONE',  ( 20.08610463437157279, 1.800000005462388364, -27.64615127144129758 ) ) ;
#674=CARTESIAN_POINT ( 'NONE',  ( 5.147494310547434893, 48.55125428154685352, 32.49999999999999289 ) ) ;
#675=CARTESIAN_POINT ( 'NONE',  ( 0.000000000000000000, 80.00000000000001421, -32.50000000000000000 ) ) ;
#677=CIRCLE ( 'NONE', #3964, 30.50000000000000000 ) ;
#680=VECTOR ( 'NONE', #25652, 1000.000000000000000 ) ;
#684=VERTEX_POINT ( 'NONE', #9066 ) ;
#689=CARTESIAN_POINT ( 'NONE',  ( -10.37757302488624411, 48.97500000273119269, -31.93888565452638417 ) ) ;
#690=CARTESIAN_POINT ( 'NONE',  ( 32.50000000000000711, 53.40000000546238823, 10.55989012756945122 ) ) ;
#692=CARTESIAN_POINT ( 'NONE',  ( -10.37757302488623701, 37.52500000273117564, 31.93888565452638417 ) ) ;
#694=CARTESIAN_POINT ( 'NONE',  ( -20.75514604977248112, 63.67500000273116711, 28.56700777964554661 ) ) ;
#695=CARTESIAN_POINT ( 'NONE',  ( -1.053607264507113999E-13, 63.00000000546238255, 32.50000000000000711 ) ) ;
#696=CARTESIAN_POINT ( 'NONE',  ( -32.50000000000000000, 39.89999999999999858, -10.55989012756945478 ) ) ;
#698=CARTESIAN_POINT ( 'NONE',  ( -33.58253175000000113, 5.275000002731187188, -10.91162601494193218 ) ) ;
#699=VECTOR ( 'NONE', #19060, 1000.000000000000000 ) ;
#700=CARTESIAN_POINT ( 'NONE',  ( 26.29305231718579350, 12.79999999999997762, 19.10302069950537529 ) ) ;
#701=CARTESIAN_POINT ( 'NONE',  ( -4.300734207923755825, 73.77500000273118985, 13.23629886949340673 ) ) ;
#702=CARTESIAN_POINT ( 'NONE',  ( -2.162160676586882350E-15, 72.87500000273115575, -35.31076352940722529 ) ) ;
#703=CARTESIAN_POINT ( 'NONE',  ( 7.570916362186213000, 4.149999994537633796, -23.30088464923126423 ) ) ;
#705=EDGE_LOOP ( 'NONE', ( #26640, #8768, #26705, #27002 ) ) ;
#717=CARTESIAN_POINT ( 'NONE',  ( 27.16883889988624290, 39.92500000273119554, 19.73931689729373673 ) ) ;
#720=CARTESIAN_POINT ( 'NONE',  ( 4.445600272181915325E-13, 14.00000000546237544, -32.50000000000000000 ) ) ;
#721=ORIENTED_EDGE ( 'NONE', *, *, #5519, .F. ) ;
#723=DIRECTION ( 'NONE',  ( -0.000000000000000000, 1.000000000000000000, -0.000000000000000000 ) ) ;
#725=CARTESIAN_POINT ( 'NONE',  ( 27.16883889988624290, 68.17500000273119554, 19.73931689729373673 ) ) ;
#726=VERTEX_POINT ( 'NONE', #9227 ) ;
#730=ORIENTED_EDGE ( 'NONE', *, *, #3699, .F. ) ;
#732=CARTESIAN_POINT ( 'NONE',  ( 33.58253175000000113, 54.12500000273118417, -4.112674001490185761E-15 ) ) ;
#734=CARTESIAN_POINT ( 'NONE',  ( -32.50000000000000000, 20.50000000546237189, 0.000000000000000000 ) ) ;
#735=CYLINDRICAL_SURFACE ( 'NONE', #19090, 24.50000000000000000 ) ;
#736=CARTESIAN_POINT ( 'NONE',  ( -18.94512977948576093, 6.324999997268820451, 13.76444248337722698 ) ) ;
#737=CARTESIAN_POINT ( 'NONE',  ( 33.58253175000000823, 24.27500000273120051, 10.91162601494192863 ) ) ;
#739=CARTESIAN_POINT ( 'NONE',  ( 23.41746824999999887, 19.12499999726882649, 0.000000000000000000 ) ) ;
#740=( BOUNDED_CURVE ( )  B_SPLINE_CURVE ( 2, ( #17852, #9600, #28472, #17505, #1696, #12172, #20082, #14927, #28305, #4967, #15102, #7193, #18196 ),
 .UNSPECIFIED., .F., .T. ) 
 B_SPLINE_CURVE_WITH_KNOTS ( ( 3, 2, 2, 2, 2, 2, 3 ),
 ( 0.4294871794871795156, 0.4307692307692307931, 0.4333333333333333481, 0.4358974358974359031, 0.4384615384615384581, 0.4410256410256410131, 0.4423076923076922906 ),
 .UNSPECIFIED. ) 
 CURVE ( )  GEOMETRIC_REPRESENTATION_ITEM ( )  RATIONAL_B_SPLINE_CURVE ( ( 0.9755282581475768211, 0.9755282581475772652, 1.000000000000000000, 0.9510565162951535312, 1.000000000000000000, 0.9510565162951535312, 1.000000000000000000, 0.9510565162951535312, 1.000000000000000000, 0.9510565162951535312, 1.000000000000000000, 0.9755282581475768211, 0.9755282581475768211 ) ) 
 REPRESENTATION_ITEM ( '' )  );
#741=EDGE_CURVE ( 'NONE', #30741, #33572, #33071, .T. ) ;
#745=CARTESIAN_POINT ( 'NONE',  ( -8.601468415847515203, 77.17500000273120975, 11.83890561707634959 ) ) ;
#747=CARTESIAN_POINT ( 'NONE',  ( 20.75514604977249178, 25.82500000273117280, 28.56700777964553950 ) ) ;
#752=CARTESIAN_POINT ( 'NONE',  ( -27.16883889988624290, 11.17500000273119554, -19.73931689729374028 ) ) ;
#755=EDGE_CURVE ( 'NONE', #26901, #13370, #4599, .T. ) ;
#756=CARTESIAN_POINT ( 'NONE',  ( -33.58253175000000113, 71.22500000273117848, 10.91162601494193929 ) ) ;
#757=EDGE_CURVE ( 'NONE', #12435, #15614, #30959, .T. ) ;
#760=CARTESIAN_POINT ( 'NONE',  ( -8.960552108402744065E-16, 76.87500000273115575, -14.63369212191046209 ) ) ;
#762=CARTESIAN_POINT ( 'NONE',  ( 2.445080149700053643E-15, 72.75000000546238255, 15.00000000000000000 ) ) ;
#763=CARTESIAN_POINT ( 'NONE',  ( -27.16883889988623935, 55.32500000273118701, 19.73931689729374739 ) ) ;
#766=ORIENTED_EDGE ( 'NONE', *, *, #17973, .F. ) ;
#768=CARTESIAN_POINT ( 'NONE',  ( -33.58253175000000113, 3.225000002731193138, 10.91162601494193929 ) ) ;
#769=CARTESIAN_POINT ( 'NONE',  ( -23.41746824999999887, 7.624999997268816720, -2.867812753649727150E-15 ) ) ;
#771=VERTEX_POINT ( 'NONE', #7000 ) ;
#773=CARTESIAN_POINT ( 'NONE',  ( -5.147494310547450880, 68.94874572391553613, 32.49999999999999289 ) ) ;
#774=VERTEX_POINT ( 'NONE', #17482 ) ;
#778=CARTESIAN_POINT ( 'NONE',  ( 6.486482029760649416E-15, 71.62500000273119838, 35.31076352940723240 ) ) ;
#780=CARTESIAN_POINT ( 'NONE',  ( 15.14183272437241889, 5.699999999999993960, 20.84094480462498211 ) ) ;
#781=CARTESIAN_POINT ( 'NONE',  ( 10.37757302488624767, 7.975000002731186477, 31.93888565452638417 ) ) ;
#782=CARTESIAN_POINT ( 'NONE',  ( -2.162160676586881955E-15, 18.62500000273117351, -35.31076352940723240 ) ) ;
#783=CARTESIAN_POINT ( 'NONE',  ( -11.25946833292375793, 76.67500000273119554, -8.180482586598733619 ) ) ;
#786=CARTESIAN_POINT ( 'NONE',  ( -9.270509831248425314, 81.70000000000001705, -12.75976212528059861 ) ) ;
#791=CARTESIAN_POINT ( 'NONE',  ( -33.58253175000000113, 43.12500000273116996, 0.000000000000000000 ) ) ;
#794=CARTESIAN_POINT ( 'NONE',  ( 10.37757302488624767, 35.97500000273118559, 31.93888565452638417 ) ) ;
#799=CARTESIAN_POINT ( 'NONE',  ( 32.50000000000000000, 31.00000000000000000, -3.980102097228898626E-15 ) ) ;
#802=CARTESIAN_POINT ( 'NONE',  ( 14.47279130897151767, 2.324999997268806240, 19.92008829642072953 ) ) ;
#803=CARTESIAN_POINT ( 'NONE',  ( -26.29305231718578995, 52.70000000546237828, 19.10302069950538595 ) ) ;
#805=EDGE_CURVE ( 'NONE', #16083, #1686, #6827, .T. ) ;
#806=DIRECTION ( 'NONE',  ( 1.000000000000000000, 0.000000000000000000, 0.000000000000000000 ) ) ;
#807=CARTESIAN_POINT ( 'NONE',  ( 33.58253175000000113, 18.12500000273117706, -4.112674001490185761E-15 ) ) ;
#808=CARTESIAN_POINT ( 'NONE',  ( 14.47279130897151767, 3.424999997268800112, -19.92008829642072598 ) ) ;
#815=CARTESIAN_POINT ( 'NONE',  ( -1.778240108872766143E-15, 9.499999999999992895, -32.49999999999999289 ) ) ;
#816=CARTESIAN_POINT ( 'NONE',  ( -14.47279130897151589, 7.324999997268822227, -19.92008829642072598 ) ) ;
#817=CARTESIAN_POINT ( 'NONE',  ( -20.75514604977248823, 29.07500000273119056, -28.56700777964554305 ) ) ;
#819=CARTESIAN_POINT ( 'NONE',  ( -20.08610463437156923, 32.80000000546237260, 27.64615127144130113 ) ) ;
#820=CARTESIAN_POINT ( 'NONE',  ( -20.08610463437156923, 76.30000000000001137, 27.64615127144130113 ) ) ;
#821=CARTESIAN_POINT ( 'NONE',  ( 26.29305231718579350, 33.30000000546237970, 19.10302069950537529 ) ) ;
#822=CARTESIAN_POINT ( 'NONE',  ( 15.00000000000000355, 72.89999999999999147, 4.873795443493592394 ) ) ;
#823=CARTESIAN_POINT ( 'NONE',  ( 10.37757302488624767, 41.97500000273118559, 31.93888565452638417 ) ) ;
#825=CARTESIAN_POINT ( 'NONE',  ( 32.50000000000000000, 22.99999999999999289, -3.980102097228898626E-15 ) ) ;
#827=CARTESIAN_POINT ( 'NONE',  ( -10.37757302488624411, 62.72500000273117848, -31.93888565452638417 ) ) ;
#828=CARTESIAN_POINT ( 'NONE',  ( 6.486482029760648627E-15, 53.87500000273119127, 35.31076352940722529 ) ) ;
#830=CARTESIAN_POINT ( 'NONE',  ( 2.067204126564591252E-14, 2.500000000000004885, -24.50000000000000000 ) ) ;
#831=CARTESIAN_POINT ( 'NONE',  ( -2.162160676586881955E-15, 6.625000002731173510, -35.31076352940723240 ) ) ;
#837=CARTESIAN_POINT ( 'NONE',  ( -20.08610463437156923, 58.80000000546239391, 27.64615127144130113 ) ) ;
#838=CARTESIAN_POINT ( 'NONE',  ( 3.880418787951134707, 13.55125428154684997, 24.50000000000000000 ) ) ;
#841=EDGE_CURVE ( 'NONE', #4493, #3462, #27944, .T. ) ;
#842=CYLINDRICAL_SURFACE ( 'NONE', #18274, 32.50000000000000000 ) ;
#846=EDGE_CURVE ( 'NONE', #5395, #23148, #33249, .T. ) ;
#849=CYLINDRICAL_SURFACE ( 'NONE', #14082, 24.50000000000000000 ) ;
#850=ORIENTED_EDGE ( 'NONE', *, *, #11450, .F. ) ;
#856=CARTESIAN_POINT ( 'NONE',  ( 6.486482029760649416E-15, 45.87500000273117706, 35.31076352940723240 ) ) ;
#857=CARTESIAN_POINT ( 'NONE',  ( -20.08610463437157989, 52.20000000546236407, -27.64615127144129758 ) ) ;
#859=CARTESIAN_POINT ( 'NONE',  ( -27.16883889988624290, 36.92500000273118843, -19.73931689729374028 ) ) ;
#860=CARTESIAN_POINT ( 'NONE',  ( 5.779280353836490358E-15, 24.50000000000000711, 32.49999999999999289 ) ) ;
#861=CARTESIAN_POINT ( 'NONE',  ( 33.58253175000000823, 62.27500000273118275, 10.91162601494192863 ) ) ;
#862=CARTESIAN_POINT ( 'NONE',  ( -10.04305231718578462, 40.39999999999999147, 30.90933677959249337 ) ) ;
#864=CARTESIAN_POINT ( 'NONE',  ( 27.16883889988624290, 6.175000002731190207, 19.73931689729373673 ) ) ;
#867=CARTESIAN_POINT ( 'NONE',  ( -20.75514604977248823, 73.07500000273115859, -28.56700777964554305 ) ) ;
#872=CARTESIAN_POINT ( 'NONE',  ( 24.50000000000000355, 1.849999994537612436, -7.960532557706203605 ) ) ;
#875=AXIS2_PLACEMENT_3D ( 'NONE', #13004, #5617, #5447 ) ;
#886=ADVANCED_FACE ( 'NONE', ( #6499 ), #15076, .T. ) ;
#888=ORIENTED_EDGE ( 'NONE', *, *, #28451, .T. ) ;
#892=CARTESIAN_POINT ( 'NONE',  ( -27.16883889988623935, 67.57500000273120122, 19.73931689729374739 ) ) ;
#896=ORIENTED_EDGE ( 'NONE', *, *, #24751, .F. ) ;
#897=CARTESIAN_POINT ( 'NONE',  ( 5.147494310547481966, 65.94874572391552192, -32.49999999999998579 ) ) ;
#898=CARTESIAN_POINT ( 'NONE',  ( 10.37757302488624767, 57.72500000273117848, 31.93888565452638417 ) ) ;
#900=CARTESIAN_POINT ( 'NONE',  ( 32.50000000000000711, 13.40000000546237047, 10.55989012756945122 ) ) ;
#901=CARTESIAN_POINT ( 'NONE',  ( -20.08610463437157989, 66.20000000546238539, -27.64615127144129758 ) ) ;
#902=CARTESIAN_POINT ( 'NONE',  ( 23.41746824999999887, 17.02499999726880731, 7.608796670333735079 ) ) ;
#903=CARTESIAN_POINT ( 'NONE',  ( 33.58253175000000113, 24.37500000273118417, -4.112674001490185761E-15 ) ) ;
#904=CARTESIAN_POINT ( 'NONE',  ( -10.04305231718578462, 24.90000000546238468, 30.90933677959249337 ) ) ;
#908=VECTOR ( 'NONE', #32914, 1000.000000000000000 ) ;
#912=CARTESIAN_POINT ( 'NONE',  ( 13.91746824999999887, 75.87500000273116996, -1.704398294459741270E-15 ) ) ;
#914=CARTESIAN_POINT ( 'NONE',  ( 20.75514604977248467, 22.42500000273119909, -28.56700777964554305 ) ) ;
#918=CARTESIAN_POINT ( 'NONE',  ( 6.486482029760648627E-15, 9.875000002731187720, 35.31076352940722529 ) ) ;
#922=CARTESIAN_POINT ( 'NONE',  ( 8.601468415847520532, 78.07500000273118701, 11.83890561707634603 ) ) ;
#924=DIRECTION ( 'NONE',  ( 0.000000000000000000, 0.000000000000000000, -1.000000000000000000 ) ) ;
#925=CARTESIAN_POINT ( 'NONE',  ( -27.16883889988624290, 48.92500000273120264, -19.73931689729374028 ) ) ;
#929=CARTESIAN_POINT ( 'NONE',  ( -5.147494310547423346, 16.44874571845315359, 32.50000000000000000 ) ) ;
#930=CARTESIAN_POINT ( 'NONE',  ( -14.47279130897152122, 5.924999997268808549, 19.92008829642072243 ) ) ;
#932=ORIENTED_EDGE ( 'NONE', *, *, #13358, .T. ) ;
#933=AXIS2_PLACEMENT_3D ( 'NONE', #24052, #13238, #23712 ) ;
#936=ORIENTED_EDGE ( 'NONE', *, *, #9999, .F. ) ;
#938=CARTESIAN_POINT ( 'NONE',  ( -27.16883889988623935, 59.57500000273119412, 19.73931689729374739 ) ) ;
#939=CARTESIAN_POINT ( 'NONE',  ( 5.147494310547426899, 69.94874572391553613, -32.50000000000000000 ) ) ;
#940=CARTESIAN_POINT ( 'NONE',  ( -33.58253175000000113, 75.22500000273119269, 10.91162601494193929 ) ) ;
#942=CARTESIAN_POINT ( 'NONE',  ( -24.50000000000001066, 5.100000000000012967, 7.960532557706201828 ) ) ;
#943=CARTESIAN_POINT ( 'NONE',  ( -2.162160676586881955E-15, 10.87500000273118417, -35.31076352940723240 ) ) ;
#944=CARTESIAN_POINT ( 'NONE',  ( -33.58253175000000113, 17.12500000273120548, 0.000000000000000000 ) ) ;
#945=CARTESIAN_POINT ( 'NONE',  ( -13.91746824999999532, 72.77500000273118985, -4.522059556121115875 ) ) ;
#947=CARTESIAN_POINT ( 'NONE',  ( -8.601468415847515203, 71.67500000273116711, 11.83890561707634959 ) ) ;
#952=CARTESIAN_POINT ( 'NONE',  ( -33.58253175000000113, 45.12500000273117706, 0.000000000000000000 ) ) ;
#955=CARTESIAN_POINT ( 'NONE',  ( -20.75514604977248112, 27.67500000273117777, 28.56700777964554661 ) ) ;
#959=CARTESIAN_POINT ( 'NONE',  ( -12.13525491562421088, 75.80000000000001137, -8.816778784387096835 ) ) ;
#962=CARTESIAN_POINT ( 'NONE',  ( -7.236395654485757944, 7.224999997268804819, -22.27133577429736988 ) ) ;
#965=CARTESIAN_POINT ( 'NONE',  ( -9.270509831248419985, 76.55000000546239391, 12.75976212528060039 ) ) ;
#966=CARTESIAN_POINT ( 'NONE',  ( -27.16883889988624290, 16.92500000273117067, -19.73931689729374028 ) ) ;
#967=CARTESIAN_POINT ( 'NONE',  ( -4.523095164977116484E-15, 4.624999997268820273, 24.62258325217400312 ) ) ;
#969=VERTEX_POINT ( 'NONE', #14731 ) ;
#972=ORIENTED_EDGE ( 'NONE', *, *, #6119, .F. ) ;
#976=CARTESIAN_POINT ( 'NONE',  ( -24.50000000000000000, 16.74999999453763522, -3.000384657911015469E-15 ) ) ;
#977=CARTESIAN_POINT ( 'NONE',  ( -18.94512977948575738, 5.424999997268809437, -13.76444248337723231 ) ) ;
#978=CARTESIAN_POINT ( 'NONE',  ( -10.37757302488624411, 30.97500000273117848, -31.93888565452638417 ) ) ;
#979=CARTESIAN_POINT ( 'NONE',  ( -32.50000000000000000, 28.40000000546235981, -10.55989012756945478 ) ) ;
#980=CARTESIAN_POINT ( 'NONE',  ( -26.29305231718579350, 73.80000000000001137, -19.10302069950537884 ) ) ;
#981=CARTESIAN_POINT ( 'NONE',  ( -7.570916362186210335, 10.59999999999999787, -23.30088464923126779 ) ) ;
#983=CARTESIAN_POINT ( 'NONE',  ( -33.58253175000000113, 43.37500000273119838, 0.000000000000000000 ) ) ;
#984=CARTESIAN_POINT ( 'NONE',  ( -14.47279130897152122, 12.42499999726880766, 19.92008829642072243 ) ) ;
#985=CARTESIAN_POINT ( 'NONE',  ( 32.50000000000000000, 13.00000000000001066, -3.980102097228898626E-15 ) ) ;
#988=CARTESIAN_POINT ( 'NONE',  ( 27.16883889988624290, 63.92500000273118843, 19.73931689729373673 ) ) ;
#989=CARTESIAN_POINT ( 'NONE',  ( -10.37757302488623701, 45.77500000273118985, 31.93888565452638417 ) ) ;
#992=CARTESIAN_POINT ( 'NONE',  ( -33.58253175000000113, 3.225000002731193138, 10.91162601494193929 ) ) ;
#996=PRODUCT_DEFINITION_CONTEXT ( 'detailed design', #19086, 'design' ) ;
#1008=DIRECTION ( 'NONE',  ( 0.000000000000000000, -1.000000000000000000, 0.000000000000000000 ) ) ;
#1013=CARTESIAN_POINT ( 'NONE',  ( 20.08610463437158344, 20.69999999999998508, 27.64615127144129403 ) ) ;
#1014=CARTESIAN_POINT ( 'NONE',  ( -33.58253175000000113, 49.27500000273118985, -10.91162601494193218 ) ) ;
#1015=CARTESIAN_POINT ( 'NONE',  ( 10.04305231718579705, 47.10000000546238397, 30.90933677959248982 ) ) ;
#1017=CARTESIAN_POINT ( 'NONE',  ( -20.75514604977248823, 36.82500000273117990, -28.56700777964554305 ) ) ;
#1019=CARTESIAN_POINT ( 'NONE',  ( 27.16883889988624290, 60.17500000273118133, 19.73931689729373673 ) ) ;
#1022=CARTESIAN_POINT ( 'NONE',  ( 10.04305231718579705, 40.59999999999999432, 30.90933677959248982 ) ) ;
#1025=CARTESIAN_POINT ( 'NONE',  ( -33.58253175000000113, 1.375000002731191495, 0.000000000000000000 ) ) ;
#1028=CARTESIAN_POINT ( 'NONE',  ( -27.16883889988623935, 71.57500000273120122, 19.73931689729374739 ) ) ;
#1029=FACE_OUTER_BOUND ( 'NONE', #7707, .T. ) ;
#1033=CARTESIAN_POINT ( 'NONE',  ( 24.50000000000000000, 5.749999994537624559, 0.000000000000000000 ) ) ;
#1035=CARTESIAN_POINT ( 'NONE',  ( 2.445080149700053643E-15, 74.50000000000001421, 15.00000000000000000 ) ) ;
#1045=FACE_OUTER_BOUND ( 'NONE', #30735, .T. ) ;
#1046=CARTESIAN_POINT ( 'NONE',  ( -7.570916362186215665, 17.39999999999999858, 23.30088464923126423 ) ) ;
#1047=ORIENTED_EDGE ( 'NONE', *, *, #18602, .T. ) ;
#1056=CARTESIAN_POINT ( 'NONE',  ( -20.08610463437156923, 48.80000000546236549, 27.64615127144130113 ) ) ;
#1057=CARTESIAN_POINT ( 'NONE',  ( 27.16883889988624290, 53.92500000273120264, 19.73931689729373673 ) ) ;
#1059=CARTESIAN_POINT ( 'NONE',  ( 32.50000000000000000, 13.50000000546236478, -3.980102097228898626E-15 ) ) ;
#1060=CARTESIAN_POINT ( 'NONE',  ( 15.14183272437242067, 15.44999999453762207, 20.84094480462498211 ) ) ;
#1061=CARTESIAN_POINT ( 'NONE',  ( -18.94512977948576093, 16.32499999726880091, 13.76444248337722698 ) ) ;
#1062=CARTESIAN_POINT ( 'NONE',  ( 32.50000000000000000, 57.09999999999999432, -10.55989012756945833 ) ) ;
#1064=CARTESIAN_POINT ( 'NONE',  ( -2.162160676586881955E-15, 24.87500000273117351, -35.31076352940723240 ) ) ;
#1065=CARTESIAN_POINT ( 'NONE',  ( 2.375766604868043252, 77.44874571845313938, -14.99999999999999822 ) ) ;
#1067=CARTESIAN_POINT ( 'NONE',  ( 13.91746825000000065, 75.77500000273120406, 4.522059556121114987 ) ) ;
#1068=CARTESIAN_POINT ( 'NONE',  ( -7.570916362186215665, 1.400000000000012346, 23.30088464923126423 ) ) ;
#1071=ORIENTED_EDGE ( 'NONE', *, *, #11450, .T. ) ;
#1073=CARTESIAN_POINT ( 'NONE',  ( 8.601468415847520532, 75.57500000273120122, 11.83890561707634781 ) ) ;
#1075=CARTESIAN_POINT ( 'NONE',  ( 33.58253175000000823, 18.02500000273118630, 10.91162601494192863 ) ) ;
#1079=CARTESIAN_POINT ( 'NONE',  ( -33.58253175000000113, 9.275000002731177418, -10.91162601494193041 ) ) ;
#1083=CARTESIAN_POINT ( 'NONE',  ( -8.601468415847518756, 77.07500000273118701, -11.83890561707634603 ) ) ;
#1085=CARTESIAN_POINT ( 'NONE',  ( -7.570916362186210335, 2.349999994537638415, -23.30088464923126779 ) ) ;
#1086=CARTESIAN_POINT ( 'NONE',  ( 20.75514604977249178, 51.82500000273120122, 28.56700777964553950 ) ) ;
#1090=CYLINDRICAL_SURFACE ( 'NONE', #17945, 32.50000000000000000 ) ;
#1091=CARTESIAN_POINT ( 'NONE',  ( -23.41746825000000243, 7.524999997268816188, -7.608796670333730638 ) ) ;
#1093=EDGE_LOOP ( 'NONE', ( #6927, #11913, #5390 ) ) ;
#1098=CARTESIAN_POINT ( 'NONE',  ( 33.58253175000000113, 58.37500000273118417, -4.112674001490185761E-15 ) ) ;
#1100=CARTESIAN_POINT ( 'NONE',  ( -10.37757302488624411, 72.72500000273119269, -31.93888565452638417 ) ) ;
#1102=CARTESIAN_POINT ( 'NONE',  ( -24.50000000000001066, 3.099999999999989875, 7.960532557706201828 ) ) ;
#1103=CARTESIAN_POINT ( 'NONE',  ( -33.58253175000000113, 5.275000002731187188, -10.91162601494193218 ) ) ;
#1104=CARTESIAN_POINT ( 'NONE',  ( 10.37757302488624767, 19.72500000273119625, 31.93888565452638417 ) ) ;
#1107=CARTESIAN_POINT ( 'NONE',  ( 13.91746824999999532, 72.47500000273119269, -4.522059556121118540 ) ) ;
#1112=CARTESIAN_POINT ( 'NONE',  ( -2.162160676586881955E-15, 34.62500000273119127, -35.31076352940723240 ) ) ;
#1115=CARTESIAN_POINT ( 'NONE',  ( -33.58253175000000113, 31.47500000273117138, 10.91162601494193929 ) ) ;
#1119=CARTESIAN_POINT ( 'NONE',  ( -5.147494310547430452, 44.05125428700922896, -32.49999999999999289 ) ) ;
#1122=CARTESIAN_POINT ( 'NONE',  ( 18.94512977948576093, 2.824999997268817786, -13.76444248337722875 ) ) ;
#1124=CARTESIAN_POINT ( 'NONE',  ( 3.000384657911015469E-15, 0.000000000000000000, -24.50000000000000000 ) ) ;
#1126=CARTESIAN_POINT ( 'NONE',  ( -9.270509831248423538, 75.95000000546238539, -12.75976212528059861 ) ) ;
#1127=CARTESIAN_POINT ( 'NONE',  ( -10.37757302488624411, 12.72500000273119092, -31.93888565452638417 ) ) ;
#1128=CARTESIAN_POINT ( 'NONE',  ( 18.94512977948575738, 6.924999997268810326, 13.76444248337723408 ) ) ;
#1130=ORIENTED_EDGE ( 'NONE', *, *, #31881, .F. ) ;
#1133=VERTEX_POINT ( 'NONE', #31022 ) ;
#1138=CARTESIAN_POINT ( 'NONE',  ( 10.04305231718579705, 38.59999999999999432, 30.90933677959248982 ) ) ;
#1139=CARTESIAN_POINT ( 'NONE',  ( -24.50000000000000355, 18.64999999453763380, -7.960532557706207157 ) ) ;
#1140=CARTESIAN_POINT ( 'NONE',  ( -23.41746825000000598, 5.724999997268815477, 7.608796670333726198 ) ) ;
#1141=CARTESIAN_POINT ( 'NONE',  ( -10.37757302488624411, 20.97500000273119625, -31.93888565452638417 ) ) ;
#1142=CARTESIAN_POINT ( 'NONE',  ( -26.29305231718579350, 30.30000000546237260, -19.10302069950537884 ) ) ;
#1143=CARTESIAN_POINT ( 'NONE',  ( 26.29305231718578995, 71.19999999999998863, -19.10302069950538240 ) ) ;
#1144=LINE ( 'NONE', #19370, #25835 ) ;
#1145=CARTESIAN_POINT ( 'NONE',  ( -15.14183272437242778, 11.29999999999999361, 20.84094480462497856 ) ) ;
#1147=CARTESIAN_POINT ( 'NONE',  ( 33.58253175000000113, 38.37500000273119838, -4.112674001490185761E-15 ) ) ;
#1151=CARTESIAN_POINT ( 'NONE',  ( 18.94512977948576093, 7.324999997268822227, -13.76444248337722875 ) ) ;
#1152=CARTESIAN_POINT ( 'NONE',  ( 26.29305231718578995, 13.19999999999998863, -19.10302069950538240 ) ) ;
#1155=CARTESIAN_POINT ( 'NONE',  ( 27.16883889988623935, 60.32500000273119412, -19.73931689729374384 ) ) ;
#1156=CARTESIAN_POINT ( 'NONE',  ( -20.75514604977248823, 45.07500000273117990, -28.56700777964554305 ) ) ;
#1158=ADVANCED_FACE ( 'NONE', ( #10099 ), #7341, .F. ) ;
#1160=CARTESIAN_POINT ( 'NONE',  ( 27.16883889988623935, 4.325000002731171911, -19.73931689729374384 ) ) ;
#1167=CARTESIAN_POINT ( 'NONE',  ( -14.45873412499999944, 71.68750000136559208, 0.000000000000000000 ) ) ;
#1168=EDGE_CURVE ( 'NONE', #33174, #33755, #10608, .T. ) ;
#1169=CYLINDRICAL_SURFACE ( 'NONE', #10005, 15.00000000000000000 ) ;
#1170=EDGE_CURVE ( 'NONE', #17032, #21850, #8028, .T. ) ;
#1178=CARTESIAN_POINT ( 'NONE',  ( 3.000384657911015469E-15, 0.000000000000000000, -24.50000000000000000 ) ) ;
#1179=VERTEX_POINT ( 'NONE', #5114 ) ;
#1183=CARTESIAN_POINT ( 'NONE',  ( -5.147494310547423346, 64.94874572391549350, 32.50000000000000000 ) ) ;
#1184=CARTESIAN_POINT ( 'NONE',  ( 27.16883889988623935, 44.57500000273117990, -19.73931689729374384 ) ) ;
#1185=CARTESIAN_POINT ( 'NONE',  ( 6.277390505771533514E-15, 51.00000000546238255, 34.17252228774368916 ) ) ;
#1187=CARTESIAN_POINT ( 'NONE',  ( 10.37757302488624056, 30.52500000273117209, -31.93888565452638417 ) ) ;
#1188=CARTESIAN_POINT ( 'NONE',  ( 32.50000000000000711, 77.40000000546238823, 10.55989012756945122 ) ) ;
#1189=CARTESIAN_POINT ( 'NONE',  ( -10.37757302488623701, 57.77500000273119696, 31.93888565452638417 ) ) ;
#1190=( NAMED_UNIT ( * ) PLANE_ANGLE_UNIT ( ) SI_UNIT ( $, .RADIAN. ) );
#1192=CARTESIAN_POINT ( 'NONE',  ( 20.08610463437158344, 32.69999999999998863, 27.64615127144129403 ) ) ;
#1194=CARTESIAN_POINT ( 'NONE',  ( 20.75514604977248467, 4.675000002731176885, -28.56700777964554305 ) ) ;
#1197=CARTESIAN_POINT ( 'NONE',  ( 33.58253175000000113, 64.47500000273120691, -10.91162601494193574 ) ) ;
#1198=CARTESIAN_POINT ( 'NONE',  ( -3.880418787951099180, 18.30125427608446387, -24.50000000000001421 ) ) ;
#1200=CARTESIAN_POINT ( 'NONE',  ( 24.50000000000000355, 7.649999994537632908, 7.960532557706212486 ) ) ;
#1202=CARTESIAN_POINT ( 'NONE',  ( 5.779280353836490358E-15, 5.000000005462372776, 32.49999999999999289 ) ) ;
#1212=CYLINDRICAL_SURFACE ( 'NONE', #29644, 24.50000000000000000 ) ;
#1213=CARTESIAN_POINT ( 'NONE',  ( -7.570916362186210335, 16.60000000000000497, -23.30088464923126779 ) ) ;
#1217=CARTESIAN_POINT ( 'NONE',  ( -32.50000000000000000, 75.89999999999996305, -10.55989012756945300 ) ) ;
#1219=VERTEX_POINT ( 'NONE', #31123 ) ;
#1223=VECTOR ( 'NONE', #14066, 1000.000000000000000 ) ;
#1224=CARTESIAN_POINT ( 'NONE',  ( 5.147494310547434893, 26.55125428154685352, 32.49999999999999289 ) ) ;
#1225=CARTESIAN_POINT ( 'NONE',  ( 10.37757302488624767, 49.72500000273119269, 31.93888565452638417 ) ) ;
#1227=CARTESIAN_POINT ( 'NONE',  ( -26.29305231718578995, 8.700000005462394270, 19.10302069950538595 ) ) ;
#1230=CARTESIAN_POINT ( 'NONE',  ( -18.94512977948576093, 18.32499999726880446, 13.76444248337722698 ) ) ;
#1231=CARTESIAN_POINT ( 'NONE',  ( 32.50000000000000000, 51.09999999999998721, -10.55989012756945833 ) ) ;
#1233=CARTESIAN_POINT ( 'NONE',  ( 33.58253175000000113, 24.47500000273118914, -10.91162601494193751 ) ) ;
#1236=CARTESIAN_POINT ( 'NONE',  ( 13.91746824999999532, 75.97500000273119269, -4.522059556121118540 ) ) ;
#1238=CARTESIAN_POINT ( 'NONE',  ( -32.50000000000000000, 34.00000000000000000, 0.000000000000000000 ) ) ;
#1240=ORIENTED_EDGE ( 'NONE', *, *, #655, .T. ) ;
#1242=CARTESIAN_POINT ( 'NONE',  ( 10.04305231718578817, 71.90000000546237402, -30.90933677959249337 ) ) ;
#1247=CARTESIAN_POINT ( 'NONE',  ( -10.37757302488624411, 8.975000002731187365, -31.93888565452638417 ) ) ;
#1251=CARTESIAN_POINT ( 'NONE',  ( -11.25946833292375793, 79.57500000273121543, 8.180482586598737171 ) ) ;
#1254=CARTESIAN_POINT ( 'NONE',  ( 33.58253175000000823, 52.02500000273118985, 10.91162601494192685 ) ) ;
#1259=DIRECTION ( 'NONE',  ( -0.000000000000000000, -1.000000000000000000, -0.000000000000000000 ) ) ;
#1260=CARTESIAN_POINT ( 'NONE',  ( 18.94512977948575738, 8.424999997268811214, 13.76444248337723408 ) ) ;
#1265=CARTESIAN_POINT ( 'NONE',  ( -32.50000000000000000, 34.60000000546236976, 10.55989012756946366 ) ) ;
#1266=EDGE_LOOP ( 'NONE', ( #10520, #19154, #1302, #23049 ) ) ;
#1268=CARTESIAN_POINT ( 'NONE',  ( -10.37757302488623701, 61.77500000273117564, 31.93888565452638417 ) ) ;
#1270=CARTESIAN_POINT ( 'NONE',  ( -10.37757302488623701, 73.52500000273121827, 31.93888565452638417 ) ) ;
#1272=CARTESIAN_POINT ( 'NONE',  ( 24.50000000000000355, 6.100000000000010303, -7.960532557706203605 ) ) ;
#1273=CARTESIAN_POINT ( 'NONE',  ( 27.16883889988624290, 2.175000002731186655, 19.73931689729373673 ) ) ;
#1274=CARTESIAN_POINT ( 'NONE',  ( 20.75514604977248467, 14.42500000273119021, -28.56700777964554305 ) ) ;
#1275=CARTESIAN_POINT ( 'NONE',  ( -13.91746824999999887, 70.87500000273119838, 0.000000000000000000 ) ) ;
#1277=CARTESIAN_POINT ( 'NONE',  ( -13.91746824999999532, 71.47500000273119269, 4.522059556121122093 ) ) ;
#1279=CIRCLE ( 'NONE', #33640, 32.50000000000000000 ) ;
#1280=CARTESIAN_POINT ( 'NONE',  ( -19.82091636218621034, 8.549999994537621717, -14.40073868116559552 ) ) ;
#1282=CARTESIAN_POINT ( 'NONE',  ( 9.270509831248423538, 79.55000000546237970, -12.75976212528059861 ) ) ;
#1284=CARTESIAN_POINT ( 'NONE',  ( 10.37757302488624767, 37.72500000273118559, 31.93888565452638417 ) ) ;
#1287=CARTESIAN_POINT ( 'NONE',  ( -27.16883889988623935, 27.57500000273119412, 19.73931689729374739 ) ) ;
#1288=DIRECTION ( 'NONE',  ( -0.000000000000000000, -1.000000000000000000, -0.000000000000000000 ) ) ;
#1290=CARTESIAN_POINT ( 'NONE',  ( -24.50000000000000000, 14.64999999453761603, -7.960532557706207157 ) ) ;
#1293=CARTESIAN_POINT ( 'NONE',  ( -18.94512977948576093, 13.82499999726882756, 13.76444248337722698 ) ) ;
#1298=CARTESIAN_POINT ( 'NONE',  ( 27.16883889988623935, 10.32500000273117635, -19.73931689729374384 ) ) ;
#1299=CARTESIAN_POINT ( 'NONE',  ( -23.41746825000000598, 4.224999997268803931, 7.608796670333726198 ) ) ;
#1302=ORIENTED_EDGE ( 'NONE', *, *, #9021, .T. ) ;
#1305=ORIENTED_EDGE ( 'NONE', *, *, #10511, .F. ) ;
#1308=CARTESIAN_POINT ( 'NONE',  ( 20.08610463437157279, 39.30000000000001137, -27.64615127144129758 ) ) ;
#1309=CARTESIAN_POINT ( 'NONE',  ( 15.14183272437241889, 19.44999999453763806, 20.84094480462498211 ) ) ;
#1310=CARTESIAN_POINT ( 'NONE',  ( 7.236395654485755280, 4.224999997268802154, 22.27133577429736988 ) ) ;
#1311=CARTESIAN_POINT ( 'NONE',  ( 27.16883889988624290, 22.17500000273120264, 19.73931689729373673 ) ) ;
#1312=CARTESIAN_POINT ( 'NONE',  ( 10.04305231718578817, 25.90000000546238823, -30.90933677959249337 ) ) ;
#1313=CARTESIAN_POINT ( 'NONE',  ( 6.277390505771533514E-15, 72.50000000000001421, 34.17252228774368916 ) ) ;
#1314=DIRECTION ( 'NONE',  ( 0.000000000000000000, 0.000000000000000000, -1.000000000000000000 ) ) ;
#1317=CARTESIAN_POINT ( 'NONE',  ( -33.58253175000000113, 33.47500000273119269, 10.91162601494193929 ) ) ;
#1321=CARTESIAN_POINT ( 'NONE',  ( 7.236395654485760609, 9.524999997268801977, -22.27133577429736633 ) ) ;
#1322=CARTESIAN_POINT ( 'NONE',  ( -10.04305231718579172, 15.60000000000000320, -30.90933677959248982 ) ) ;
#1325=EDGE_CURVE ( 'NONE', #33879, #30610, #2908, .T. ) ;
#1327=CARTESIAN_POINT ( 'NONE',  ( 6.486482029760649416E-15, 59.62500000273118417, 35.31076352940723240 ) ) ;
#1328=CARTESIAN_POINT ( 'NONE',  ( 33.58253175000000113, 44.47500000273119980, -10.91162601494193574 ) ) ;
#1330=CARTESIAN_POINT ( 'NONE',  ( 7.570916362186213000, 10.39999999999999325, -23.30088464923126423 ) ) ;
#1333=( BOUNDED_CURVE ( )  B_SPLINE_CURVE ( 2, ( #15070, #17820, #9916, #23127, #1664, #17476, #22612, #9222, #28276, #28106, #9570, #4763, #19706 ),
 .UNSPECIFIED., .F., .T. ) 
 B_SPLINE_CURVE_WITH_KNOTS ( ( 3, 2, 2, 2, 2, 2, 3 ),
 ( 0.3525641025641025883, 0.3538461538461538658, 0.3564102564102564208, 0.3589743589743589758, 0.3615384615384615308, 0.3641025641025640858, 0.3653846153846153633 ),
 .UNSPECIFIED. ) 
 CURVE ( )  GEOMETRIC_REPRESENTATION_ITEM ( )  RATIONAL_B_SPLINE_CURVE ( ( 0.9755282581475768211, 0.9755282581475772652, 1.000000000000000000, 0.9510565162951535312, 1.000000000000000000, 0.9510565162951535312, 1.000000000000000000, 0.9510565162951535312, 1.000000000000000000, 0.9510565162951535312, 1.000000000000000000, 0.9755282581475768211, 0.9755282581475768211 ) ) 
 REPRESENTATION_ITEM ( '' )  );
#1337=CYLINDRICAL_SURFACE ( 'NONE', #3434, 32.50000000000000000 ) ;
#1339=CARTESIAN_POINT ( 'NONE',  ( 24.50000000000000000, 13.89999999999999680, 7.960532557706212486 ) ) ;
#1342=CYLINDRICAL_SURFACE ( 'NONE', #21108, 15.00000000000000000 ) ;
#1343=CARTESIAN_POINT ( 'NONE',  ( 33.58253175000000113, 34.22500000273117138, -10.91162601494193574 ) ) ;
#1350=ORIENTED_EDGE ( 'NONE', *, *, #9950, .T. ) ;
#1356=CARTESIAN_POINT ( 'NONE',  ( 20.75514604977249178, 44.07500000273117990, 28.56700777964553950 ) ) ;
#1357=CARTESIAN_POINT ( 'NONE',  ( 26.29305231718579350, 53.30000000546236549, 19.10302069950537529 ) ) ;
#1359=CARTESIAN_POINT ( 'NONE',  ( 6.486482029760649416E-15, 29.62500000273120193, 35.31076352940723240 ) ) ;
#1360=CARTESIAN_POINT ( 'NONE',  ( 10.04305231718579705, 77.10000000546237686, 30.90933677959248982 ) ) ;
#1361=CARTESIAN_POINT ( 'NONE',  ( -2.162160676586881955E-15, 58.87500000273117706, -35.31076352940723240 ) ) ;
#1362=( NAMED_UNIT ( * ) SI_UNIT ( $, .STERADIAN. ) SOLID_ANGLE_UNIT ( ) );
#1363=EDGE_CURVE ( 'NONE', #32007, #6723, #33631, .T. ) ;
#1365=CARTESIAN_POINT ( 'NONE',  ( 20.08610463437157279, 31.30000000000000071, -27.64615127144129758 ) ) ;
#1367=CARTESIAN_POINT ( 'NONE',  ( -27.16883889988623935, 73.32500000273117280, 19.73931689729374739 ) ) ;
#1369=FACE_OUTER_BOUND ( 'NONE', #17714, .T. ) ;
#1371=CARTESIAN_POINT ( 'NONE',  ( 10.37757302488624767, 63.97500000273120691, 31.93888565452638417 ) ) ;
#1375=CARTESIAN_POINT ( 'NONE',  ( -19.82091636218621389, 2.949999994537627401, 14.40073868116558842 ) ) ;
#1376=AXIS2_PLACEMENT_3D ( 'NONE', #6186, #27460, #21818 ) ;
#1390=AXIS2_PLACEMENT_3D ( 'NONE', #28452, #10100, #31024 ) ;
#1391=CARTESIAN_POINT ( 'NONE',  ( -32.50000000000000000, 57.89999999999999858, -10.55989012756945300 ) ) ;
#1392=CARTESIAN_POINT ( 'NONE',  ( -3.880418787951127602, 4.301254276084477191, -24.50000000000000000 ) ) ;
#1395=CARTESIAN_POINT ( 'NONE',  ( -5.147494310547423346, 76.44874571845313938, 32.50000000000000000 ) ) ;
#1397=EDGE_LOOP ( 'NONE', ( #10454, #24913, #25682, #18863, #18814, #27071, #26820, #24496 ) ) ;
#1400=CARTESIAN_POINT ( 'NONE',  ( -24.50000000000000711, 12.84999999453761532, 7.960532557706201828 ) ) ;
#1401=CARTESIAN_POINT ( 'NONE',  ( 33.58253175000000113, 46.12500000273117706, -4.112674001490185761E-15 ) ) ;
#1403=CARTESIAN_POINT ( 'NONE',  ( 20.08610463437157279, 13.80000000546235839, -27.64615127144129758 ) ) ;
#1405=CARTESIAN_POINT ( 'NONE',  ( -18.94512977948575738, 15.92499999726881832, -13.76444248337723231 ) ) ;
#1406=CARTESIAN_POINT ( 'NONE',  ( 10.04305231718579705, 54.59999999999998010, 30.90933677959248982 ) ) ;
#1407=CARTESIAN_POINT ( 'NONE',  ( -8.891200544363830713E-16, 71.75000000546238255, -15.00000000000000000 ) ) ;
#1408=CARTESIAN_POINT ( 'NONE',  ( 6.486482029760649416E-15, 15.87500000273120015, 35.31076352940723240 ) ) ;
#1411=CARTESIAN_POINT ( 'NONE',  ( 8.601468415847520532, 77.57500000273118701, 11.83890561707634781 ) ) ;
#1413=CARTESIAN_POINT ( 'NONE',  ( 5.779280353836490358E-15, 34.49999999999998579, 32.49999999999999289 ) ) ;
#1417=CARTESIAN_POINT ( 'NONE',  ( 32.50000000000000711, 71.40000000546240244, 10.55989012756945122 ) ) ;
#1422=CARTESIAN_POINT ( 'NONE',  ( -10.37757302488624411, 10.97500000273118914, -31.93888565452638417 ) ) ;
#1425=CARTESIAN_POINT ( 'NONE',  ( 8.601468415847520532, 80.07500000273118701, 11.83890561707634603 ) ) ;
#1428=CARTESIAN_POINT ( 'NONE',  ( -27.16883889988624290, 50.92500000273120264, -19.73931689729374028 ) ) ;
#1430=ORIENTED_EDGE ( 'NONE', *, *, #8739, .T. ) ;
#1432=CARTESIAN_POINT ( 'NONE',  ( 23.41746824999999887, 14.62499999726882294, 0.000000000000000000 ) ) ;
#1434=( BOUNDED_CURVE ( )  B_SPLINE_CURVE ( 2, ( #18708, #3410, #13883, #11465, #16132, #13552, #24015, #31887, #821, #22110, #30143, #14548, #25007 ),
 .UNSPECIFIED., .F., .T. ) 
 B_SPLINE_CURVE_WITH_KNOTS ( ( 3, 2, 2, 2, 2, 2, 3 ),
 ( 0.5705128205128204844, 0.5717948717948717618, 0.5743589743589743168, 0.5769230769230768718, 0.5794871794871795379, 0.5820512820512820928, 0.5833333333333333703 ),
 .UNSPECIFIED. ) 
 CURVE ( )  GEOMETRIC_REPRESENTATION_ITEM ( )  RATIONAL_B_SPLINE_CURVE ( ( 0.9755282581475768211, 0.9755282581475768211, 1.000000000000000000, 0.9510565162951535312, 1.000000000000000000, 0.9510565162951535312, 1.000000000000000000, 0.9510565162951535312, 1.000000000000000000, 0.9510565162951535312, 1.000000000000000000, 0.9755282581475768211, 0.9755282581475768211 ) ) 
 REPRESENTATION_ITEM ( '' )  );
#1435=ORIENTED_EDGE ( 'NONE', *, *, #13848, .T. ) ;
#1438=CARTESIAN_POINT ( 'NONE',  ( 7.570916362186207671, 5.599999999999994316, 23.30088464923126779 ) ) ;
#1439=ORIENTED_EDGE ( 'NONE', *, *, #19442, .T. ) ;
#1440=( BOUNDED_SURFACE ( )  B_SPLINE_SURFACE ( 1, 2, ( 
 ( #26586, #29145, #13713, #31724, #10968, #2737, #24179, #10632, #31886, #18707, #18867, #16458, #29315, #29477, #26416, #26249, #21443, #21110, #8215, #5818, #31554, #3082, #3409, #5481, #26911, #13200, #16294, #21609, #23677, #5981, #32054, #2910, #8554, #19038, #13882, #24348, #13378, #820, #21282, #11301, #5649, #21779, #16131, #7879, #18369, #21938, #9213, #32717, #11796, #17127, #22274, #3907, #29812, #14213, #19198, #16791, #19532, #19697, #27249, #11625, #6315, #16958, #980, #22433, #27080, #32388, #6486, #6812, #27583, #27417, #24669, #16625, #3574, #11464, #30315, #1313, #30142, #14716, #6646, #14547, #8883, #4072, #6140, #3742, #14376, #1488, #25006, #19369, #1143, #29637, #24835, #22109, #32553, #11962, #32880, #24507, #9379, #25176, #19861, #17293, #8715, #14046, #27754, #9052, #29981, #4242, #1654, #12129, #32226, #17467, #33582, #18156, #4584, #7325, #27927, #7670, #33408, #23297, #17635, #20215, #25861, #20382, #30483, #25528, #2528, #22601, #28267, #28096, #22950, #4411, #33055, #10256, #20038, #7503, #2351, #9905, #14888, #9560, #20737, #6984, #17987, #12825, #25349, #12647, #30833, #23118, #31179, #10082, #28598, #7152, #1828, #15230, #12306, #12481, #20561, #22778, #17809, #5098, #33230, #15583, #9729, #4753, #28435, #30655, #26034, #4925, #15061, #15405, #2174, #25693, #33764, #2005, #31006, #15920, #6401, #7839, #16875, #13160, #5439, #26206, #2700, #23975, #13512, #26544, #31848, #3040, #18666, #10592, #28941, #33929, #31518, #274, #446, #8012, #26376, #21069, #31682, #15752, #3658, #18328, #23636, #21239, #22025, #8341, #8176, #2867, #31346, #28773, #102, #11543, #16093, #10928, #29898, #21403, #29276, #18497, #18831, #20897, #13336, #29104, #16711, #6231, #23809, #10761, #10420, #5609, #27165, #14134, #24590, #1062, #5270, #32469, #27338, #8970, #19453, #23467, #12996, #1742, #11884, #14297, #14804, #30062, #24755, #22519, #32640, #25269, #33326, #19780, #32970, #9135, #22868, #14635, #4500, #32802, #1406, #7072, #1572, #11710, #6731, #17728, #3824, #9474, #9295, #28013, #19617, #3993, #12049, #12397, #33146, #19955, #30229, #22194, #6568, #17042, #1921, #6902, #17383, #20300, #27848, #20131, #14465, #22695, #27502, #22355, #30403, #17556, #4331, #24921, #17214, #1231, #12222, #27673, #4162, #9651, #30576, #25095, #14976, #30750, #25445, #9823, #7239, #33499, #26123, #2270, #4673, #5191, #20475, #15152, #12912, #23041, #15675, #23723, #10175, #23388, #10002, #13250, #5015, #28861, #23216, #25782, #31437, #25953, #2097, #31097, #8098, #28185, #33850, #33676, #28520, #30926, #25616, #15838, #12570, #13083, #7929, #7419, #18246, #15497, #28693, #2784, #2620, #26295, #12743, #17905, #20821, #28358, #18071, #23557, #4844, #10345, #190, #15326, #10677, #20657, #31265, #21, #7594, #21158, #10509, #2446, #20987, #7760, #18416, #5358, #31600, #11182, #21487, #11504, #13425, #21984, #18751, #11017, #31766, #8259, #29519, #19079, #32098, #3452, #8595, #24226, #16176, #530, #5528, #3126, #5862, #6022, #13598, #31934, #26632, #3290, #21325, #16669, #21653, #16500, #1022, #26953, #862, #29193, #13924, #26463, #24064, #696, #21819, #24388, #5699, #8427, #16008, #11343, #18916, #29361, #32267, #8760, #10850, #19243, #32432, #26796, #29682, #29025, #23893, #6187, #16340, #2955, #27126, #13755, #364, #3620, #14094, #24550, #18585, #24882, #27634, #14257, #27975, #19744, #9609, #3952, #6532, #12182, #6692, #16839, #11842, #22825, #8930, #14597, #14427, #9260, #3787, #19411, #30535, #6360, #27805, #22652, #11673, #32929, #30190, #9428, #17514, #30362, #7031, #27462, #27295, #1535, #22156, #32766, #6863, #32598, #4122, #4460, #9098, #14936, #24715, #25054, #14764, #1192, #25401, #25229, #19579, #4289, #22480, #12011, #33104, #30027, #19913, #22321, #1879, #17005, #12356, #1365, #17176, #17342, #1703, #20090, #29860, #12872, #18206, #23349, #4977, #30882, #15281, #20262, #17862, #20614, #20782, #28313, #12700, #7378, #18035, #2055, #23515, #28146, #33457, #7551, #7886, #28649, #28481, #25741, #17686, #4632, #12531, #15455, #15111, #5145, #2223, #15632, #25575, #9956, #4801, #25910, #2404, #30707, #7202, #33285, #18375, #33811, #20947, #10468, #31396, #2580, #7719, #28820, #20432, #13044, #33975, #23000, #5318, #10304, #23171, #26084, #31226, #15798, #33633, #26254, #2742, #13206, #10132, #9782, #31058, #21116, #26917, #10637, #24021, #321, #3414, #29149, #28988, #5487, #18713, #2916, #16301, #26758, #825, #13888, #13383, #32060, #5655, #31728, #29643, #3250, #8560, #13720, #21448, #31891, #16137, #24354, #8057, #491, #3581, #31559, #10808, #21288, #18872, #27087, #8387, #26591, #21615, #10974, #23682, #8219, #18542, #3087, #15966, #19044, #13559, #26422, #23855, #11306, #29321, #5823, #21784, #29482, #24184, #657, #11145, #5986, #16463, #32232, #8722, #19206, #6146, #148, #16631, #19705, #30151, #12138, #24844, #4081, #17302, #6655, #16800, #20047, #16966, #22611, #14222, #27764, #11972, #29819, #33064, #14725, #9569, #30492, #29989, #17138, #17475, #32728, #1322, #32888, #3915, #22283, #6993, #9387, #9221, #6493, #32394, #8889, #27257, #27936, #27591, #14555, #14053, #25016, #30324, #24678, #19871, #21944, #22117, #1496, #4250, #22442, #1152, #27424, #985, #6820, #11634, #14387, #25186, #1663, #6324, #24515, #11470, #19374, #3748, #32561, #9060, #19541, #11805, #14895, #15415, #30664, #25359, #23126, #33240, #25870, #33938, #20391, #33591, #9738, #23476, #15239, #5107, #33417, #2015, #7679, #2183, #12316, #7334, #18336, #4420, #10092, #9915, #4762, #20224, #1837, #26043, #22787, #23307, #18165, #7161, #28442, #25702, #4933, #13005, #2360, #2538, #22959, #17644, #31014, #28105, #28275, #12833, #4592, #20570, #10430, #15068, #20905, #25536, #7512, #10264, #12490, #31356, #20746, #30843, #33773, #17996, #31189, #28607, #17818, #15591, #12657, #7848, #26215, #21412, #109, #18505, #23647, #10600, #21248, #31691, #283, #18675, #10771, #13345, #21078, #8020, #5278, #31526, #26385, #8185, #28951, #5448, #15929, #2877, #13169, #16102, #2708, #23817, #29114, #5618, #13520, #26553, #3048, #23984 ),
 ( #455, #28781, #10936, #15762, #10371, #15357, #7621, #20331, #20849, #7452, #31295, #30781, #25647, #23070, #31129, #18101, #12430, #22899, #25477, #10539, #28549, #13112, #2649, #23586, #28723, #33878, #51, #2125, #5218, #15701, #7274, #21016, #5046, #4876, #7787, #20688, #33709, #12600, #18276, #26155, #31467, #25811, #7959, #18446, #33357, #28889, #9854, #2302, #33531, #5389, #30955, #17757, #28215, #20509, #4702, #15530, #25983, #1956, #15183, #10034, #17937, #28387, #12774, #23248, #2476, #10207, #12943, #23416, #13628, #8288, #16531, #219, #26660, #29713, #13279, #2987, #26492, #11050, #19272, #24092, #18778, #13787, #3156, #15867, #13456, #10706, #29222, #21187, #11211, #5728, #31629, #2812, #26982, #16206, #8127, #13952, #24255, #18615, #560, #31964, #23924, #29053, #21515, #5558, #21684, #8458, #16037, #23754, #3481, #18947, #394, #24415, #725, #10879, #29392, #5892, #16370, #26824, #892, #3320, #32131, #8626, #26324, #21849, #19109, #29547, #11373, #6048, #32294, #8788, #21354, #31796, #23146, #20069, #10111, #6842, #33437, #2036, #11990, #17157, #4101, #1515, #9408, #12159, #1860, #19891, #33264, #9758, #22978, #30513, #20243, #17321, #27784, #22633, #4270, #14744, #30684, #7182, #4199, #27204, #32506, #1442, #9330, #8837, #32673, #9511, #24789, #19816, #27033, #21893, #14501, #24625, #3528, #27539, #19320, #14000, #1268, #11418, #4026, #12085, #9007, #11748, #32343, #1607, #27373, #17249, #11581, #14168, #30268, #14333, #24462, #19487, #30915, #16578, #22227, #22062, #16911, #29762, #938, #14670, #6269, #11919, #6768, #16746, #6602, #3861, #17079, #25130, #24958, #22553, #1098, #3695, #9169, #29936, #6440, #22390, #19653, #30095, #33006, #32839, #20464, #27709, #13073, #13239, #23204, #5518, #23713, #18405, #7920, #20977, #26285, #31427, #23548, #5005, #23378, #28348, #25942, #28683, #28850, #2436, #20812, #15488, #26113, #10163, #31590, #2259, #7585, #15664, #15998, #2775, #2611, #33840, #25773, #12733, #20646, #26454, #10499, #5349, #23884, #15830, #179, #18063, #10669, #15314, #12903, #10, #21148, #8089, #4834, #18576, #29017, #2945, #28508, #10336, #13416, #355, #33666, #10839, #21316, #7409, #17895, #31088, #31256, #7748, #18237, #5181, #8753, #24053, #8249, #16491, #26622, #19237, #27287, #13747, #26946, #3118, #16832, #8588, #32424, #26788, #29353, #1014, #29512, #5689, #689, #11665, #31758, #3446, #3280, #32092, #13589, #18741, #19404, #29184, #16662, #11497, #521, #21812, #19072, #32260, #6353, #29675, #29852, #16332, #16167, #24383, #11008, #21646, #6180, #21478, #13916, #3779, #31925, #14250, #8417, #856, #3612, #18906, #24707, #14085, #5853, #27119, #11336, #24543, #21976, #24218, #8921, #11175, #1184, #6016, #25568, #22313, #14587, #1356, #11835, #14928, #14420, #4282, #15103, #30354, #25394, #32591, #27454, #20083, #30181, #9090, #33098, #24873, #19572, #6856, #16996, #9601, #17676, #4113, #17334, #3945, #7194, #32921, #22818, #17169, #19737, #1871, #19905, #30020, #25047, #2048, #22147, #27798, #27626, #22473, #32758, #6524, #9772, #9252, #7024, #12349, #6685, #12173, #9420, #22645, #30698, #30526, #20255, #1528, #12002, #14756, #25219, #1697, #17506, #27968, #4450, #28138, #33277, #4624, #20424, #18197, #18366, #28306, #10630, #28811, #4794, #7877, #26074, #31217, #26247, #23161, #5136, #15446, #5479, #7368, #15958, #12692, #4968, #25734, #2213, #23508, #13037, #2569, #31387, #33966, #28640, #10123, #28473, #33450, #31050, #33803, #10460, #7542, #25901, #20604, #7710, #15273, #2735, #17853, #33624, #20773, #21107, #5308, #15622, #2394, #30873, #18027, #12863, #31551, #20938, #15790, #28980, #13198, #23675, #23340, #139, #10296, #8049, #18534, #26414, #12523, #9948, #22991, #16456, #24504, #13549, #18865, #21777, #11138, #978, #29474, #11298, #5815, #16789, #8881, #8551, #19036, #11462, #13711, #26908, #6138, #5979, #5647, #19367, #16292, #21936, #3079, #16623, #817, #18705, #32386, #3572, #29810, #6311, #29312, #3407, #2907, #21607, #24177, #32224, #26749, #13879, #31721, #8713, #3243, #19196, #8212, #24011, #648, #29143, #32050, #23847, #312, #13376, #10800, #24346, #21279, #14043, #16129, #27077, #29635, #26583, #483, #10966, #21440, #31884, #8380, #19858, #6644, #22599, #22431, #1486, #3905, #12127, #30481, #33053, #17124, #6982, #9558, #24667, #17465, #14211, #27581, #14374, #27925, #32714, #32551, #9050, #22272, #6484, #30313, #6810, #4408, #14885, #16956, #1652, #9211, #1311, #33228, #17289, #20035, #27752, #25004, #11960, #19694, #25346, #11623, #4070, #7150, #1141, #24833, #11793, #32878, #30653, #9377, #30140, #25173, #14545, #27247, #4240, #22106, #14714, #19529, #1826, #12304, #29979, #27415, #22776, #9727, #20213, #3740, #15582, #22948, #17985, #33762, #31177, #2526, #10419, #9903, #10254, #10590, #25859, #20896, #28093, #33406, #26033, #25691, #4582, #28596, #20380, #15059, #2348, #12478, #5095, #13159, #33579, #12823, #30829, #2699, #28433, #18327, #12645, #15228, #31345, #15403, #25526, #20559, #31517, #17632, #23294, #23116, #4923, #7323, #2003, #5268, #17807, #12995, #7837, #28265, #7667, #20735, #18154, #26205, #23466, #15750, #2172, #4751, #33928, #10078, #7501, #28772, #31004, #23635, #101, #21068, #16583, #15919, #13677, #13840, #23808, #6102, #24307, #273, #3370, #21569, #26713, #21739, #18665, #608, #10927, #943, #2865, #11423, #8174, #444, #21238, #31681, #18997, #8510, #32014, #26875, #29441, #24141, #5608, #23974, #28939, #26543, #29275, #5943, #3038, #21401, #16092, #3209, #10760, #32184, #13334, #29103, #16256, #27038, #781, #11100, #31847, #26375, #13511, #8340, #3533, #16423, #11263, #24468, #8679, #19162, #18830, #29600, #5776, #14005, #21898, #8011, #18496, #5438, #4203, #11925, #19997, #9012, #14338, #17254, #12090, #1103, #22395, #9174, #32844, #6943, #19821, #30445, #16917, #16751, #24965, #11587, #22234, #30273, #22067, #27544, #27887, #32511, #17426, #6274, #4031, #14675, #14173, #4370, #25135, #24630, #27715, #9336, #17084, #22559, #19492, #1447, #1273, #25311, #27209, #1784, #29941, #24794, #6445, #27377, #6773 ) ),
 .UNSPECIFIED., .F., .F., .T. ) 
 B_SPLINE_SURFACE_WITH_KNOTS ( ( 2, 2 ),
 ( 3, 2, 2, 2, 2, 2, 2, 2, 2, 2, 2, 2, 2, 2, 2, 2, 2, 2, 2, 2, 2, 2, 2, 2, 2, 2, 2, 2, 2, 2, 2, 2, 2, 2, 2, 2, 2, 2, 2, 2, 2, 2, 2, 2, 2, 2, 2, 2, 2, 2, 2, 2, 2, 2, 2, 2, 2, 2, 2, 2, 2, 2, 2, 2, 2, 2, 2, 2, 2, 2, 2, 2, 2, 2, 2, 2, 2, 2, 2, 2, 2, 2, 2, 2, 2, 2, 2, 2, 2, 2, 2, 2, 2, 2, 2, 2, 2, 2, 2, 2, 2, 2, 2, 2, 2, 2, 2, 2, 2, 2, 2, 2, 2, 2, 2, 2, 2, 2, 2, 2, 2, 2, 2, 2, 2, 2, 2, 2, 2, 2, 2, 2, 2, 2, 2, 2, 2, 2, 2, 2, 2, 2, 2, 2, 2, 2, 2, 2, 2, 2, 2, 2, 2, 2, 2, 2, 2, 2, 2, 2, 2, 2, 2, 2, 2, 2, 2, 2, 2, 2, 2, 2, 2, 2, 2, 2, 2, 2, 2, 2, 2, 2, 2, 2, 2, 2, 2, 2, 2, 2, 2, 2, 2, 2, 2, 2, 2, 2, 2, 2, 2, 2, 2, 2, 2, 2, 2, 2, 2, 2, 2, 2, 2, 2, 2, 2, 2, 2, 2, 2, 2, 2, 2, 2, 2, 2, 2, 2, 2, 2, 2, 2, 2, 2, 2, 2, 2, 2, 2, 2, 2, 2, 2, 2, 2, 2, 2, 2, 2, 2, 2, 2, 2, 2, 2, 2, 2, 2, 2, 2, 2, 2, 2, 2, 2, 2, 2, 2, 2, 2, 2, 2, 2, 2, 2, 2, 2, 2, 2, 2, 2, 2, 2, 2, 2, 2, 2, 2, 2, 2, 2, 2, 2, 2, 2, 2, 2, 2, 2, 2, 2, 2, 2, 2, 2, 2, 2, 2, 2, 2, 2, 2, 2, 2, 2, 2, 2, 2, 2, 2, 2, 2, 2, 2, 2, 2, 2, 2, 2, 2, 2, 2, 2, 2, 2, 2, 2, 2, 2, 2, 2, 2, 2, 2, 2, 2, 2, 2, 2, 2, 2, 2, 2, 2, 2, 2, 2, 2, 2, 2, 2, 2, 2, 2, 2, 2, 2, 2, 2, 2, 2, 2, 2, 2, 2, 2, 2, 2, 2, 2, 2, 2, 2, 2, 2, 2, 2, 2, 2, 2, 3 ),
 ( 0.000000000000000000, 1.000000000000000000 ),
 ( 0.000000000000000000, 0.002564102564102564100, 0.005128205128205128201, 0.007692307692307692735, 0.01025641025641025640, 0.01282051282051282007, 0.01538461538461538547, 0.01794871794871794740, 0.02051282051282051280, 0.02307692307692307820, 0.02564102564102564014, 0.02820512820512820554, 0.03076923076923077094, 0.03333333333333333287, 0.03589743589743589480, 0.03846153846153846367, 0.04102564102564102561, 0.04358974358974358754, 0.04615384615384615641, 0.04871794871794871834, 0.05128205128205128027, 0.05384615384615384914, 0.05641025641025641107, 0.05897435897435897301, 0.06153846153846154188, 0.06410256410256409687, 0.06666666666666666574, 0.06923076923076923461, 0.07179487179487178961, 0.07435897435897435848, 0.07692307692307692735, 0.07948717948717948234, 0.08205128205128205121, 0.08461538461538462008, 0.08717948717948717507, 0.08974358974358974395, 0.09230769230769231282, 0.09487179487179486781, 0.09743589743589743668, 0.1000000000000000056, 0.1025641025641025605, 0.1051282051282051294, 0.1076923076923076983, 0.1102564102564102533, 0.1128205128205128221, 0.1153846153846153910, 0.1179487179487179460, 0.1205128205128205149, 0.1230769230769230838, 0.1256410256410256387, 0.1282051282051281937, 0.1307692307692307765, 0.1333333333333333315, 0.1358974358974358865, 0.1384615384615384692, 0.1410256410256410242, 0.1435897435897435792, 0.1461538461538461620, 0.1487179487179487170, 0.1512820512820512719, 0.1538461538461538547, 0.1564102564102564097, 0.1589743589743589647, 0.1615384615384615474, 0.1641025641025641024, 0.1666666666666666574, 0.1692307692307692402, 0.1717948717948717952, 0.1743589743589743501, 0.1769230769230769329, 0.1794871794871794879, 0.1820512820512820429, 0.1846153846153846256, 0.1871794871794871806, 0.1897435897435897356, 0.1923076923076923184, 0.1948717948717948734, 0.1974358974358974284, 0.2000000000000000111, 0.2025641025641025661, 0.2051282051282051211, 0.2076923076923077038, 0.2102564102564102588, 0.2128205128205128138, 0.2153846153846153966, 0.2179487179487179516, 0.2205128205128205066, 0.2230769230769230893, 0.2256410256410256443, 0.2282051282051281993, 0.2307692307692307820, 0.2333333333333333370, 0.2358974358974358920, 0.2384615384615384748, 0.2410256410256410298, 0.2435897435897435848, 0.2461538461538461675, 0.2487179487179487225, 0.2512820512820512775, 0.2538461538461538325, 0.2564102564102563875, 0.2589743589743589980, 0.2615384615384615530, 0.2641025641025641080, 0.2666666666666666630, 0.2692307692307692180, 0.2717948717948717730, 0.2743589743589743835, 0.2769230769230769384, 0.2794871794871794934, 0.2820512820512820484, 0.2846153846153846034, 0.2871794871794871584, 0.2897435897435897689, 0.2923076923076923239, 0.2948717948717948789, 0.2974358974358974339, 0.2999999999999999889, 0.3025641025641025439, 0.3051282051282051544, 0.3076923076923077094, 0.3102564102564102644, 0.3128205128205128194, 0.3153846153846153744, 0.3179487179487179294, 0.3205128205128205399, 0.3230769230769230949, 0.3256410256410256499, 0.3282051282051282048, 0.3307692307692307598, 0.3333333333333333148, 0.3358974358974358698, 0.3384615384615384803, 0.3410256410256410353, 0.3435897435897435903, 0.3461538461538461453, 0.3487179487179487003, 0.3512820512820512553, 0.3538461538461538658, 0.3564102564102564208, 0.3589743589743589758, 0.3615384615384615308, 0.3641025641025640858, 0.3666666666666666408, 0.3692307692307692513, 0.3717948717948718063, 0.3743589743589743613, 0.3769230769230769162, 0.3794871794871794712, 0.3820512820512820262, 0.3846153846153846367, 0.3871794871794871917, 0.3897435897435897467, 0.3923076923076923017, 0.3948717948717948567, 0.3974358974358974117, 0.4000000000000000222, 0.4025641025641025772, 0.4051282051282051322, 0.4076923076923076872, 0.4102564102564102422, 0.4128205128205127972, 0.4153846153846154077, 0.4179487179487179627, 0.4205128205128205177, 0.4230769230769230727, 0.4256410256410256276, 0.4282051282051281826, 0.4307692307692307931, 0.4333333333333333481, 0.4358974358974359031, 0.4384615384615384581, 0.4410256410256410131, 0.4435897435897435681, 0.4461538461538461786, 0.4487179487179487336, 0.4512820512820512886, 0.4538461538461538436, 0.4564102564102563986, 0.4589743589743589536, 0.4615384615384615641, 0.4641025641025641191, 0.4666666666666666741, 0.4692307692307692291, 0.4717948717948717841, 0.4743589743589743390, 0.4769230769230769496, 0.4794871794871795045, 0.4820512820512820595, 0.4846153846153846145, 0.4871794871794871695, 0.4897435897435897245, 0.4923076923076923350, 0.4948717948717948900, 0.4974358974358974450, 0.5000000000000000000, 0.5025641025641025550, 0.5051282051282051100, 0.5076923076923076650, 0.5102564102564102200, 0.5128205128205127750, 0.5153846153846153300, 0.5179487179487179960, 0.5205128205128205510, 0.5230769230769231060, 0.5256410256410256610, 0.5282051282051282159, 0.5307692307692307709, 0.5333333333333333259, 0.5358974358974358809, 0.5384615384615384359, 0.5410256410256409909, 0.5435897435897435459, 0.5461538461538461009, 0.5487179487179487669, 0.5512820512820513219, 0.5538461538461538769, 0.5564102564102564319, 0.5589743589743589869, 0.5615384615384615419, 0.5641025641025640969, 0.5666666666666666519, 0.5692307692307692069, 0.5717948717948717618, 0.5743589743589743168, 0.5769230769230768718, 0.5794871794871795379, 0.5820512820512820928, 0.5846153846153846478, 0.5871794871794872028, 0.5897435897435897578, 0.5923076923076923128, 0.5948717948717948678, 0.5974358974358974228, 0.5999999999999999778, 0.6025641025641025328, 0.6051282051282050878, 0.6076923076923076428, 0.6102564102564103088, 0.6128205128205128638, 0.6153846153846154188, 0.6179487179487179738, 0.6205128205128205288, 0.6230769230769230838, 0.6256410256410256387, 0.6282051282051281937, 0.6307692307692307487, 0.6333333333333333037, 0.6358974358974358587, 0.6384615384615384137, 0.6410256410256410797, 0.6435897435897436347, 0.6461538461538461897, 0.6487179487179487447, 0.6512820512820512997, 0.6538461538461538547, 0.6564102564102564097, 0.6589743589743589647, 0.6615384615384615197, 0.6641025641025640747, 0.6666666666666666297, 0.6692307692307691847, 0.6717948717948717396, 0.6743589743589744057, 0.6769230769230769607, 0.6794871794871795156, 0.6820512820512820706, 0.6846153846153846256, 0.6871794871794871806, 0.6897435897435897356, 0.6923076923076922906, 0.6948717948717948456, 0.6974358974358974006, 0.6999999999999999556, 0.7025641025641025106, 0.7051282051282051766, 0.7076923076923077316, 0.7102564102564102866, 0.7128205128205128416, 0.7153846153846153966, 0.7179487179487179516, 0.7205128205128205066, 0.7230769230769230616, 0.7256410256410256165, 0.7282051282051281715, 0.7307692307692307265, 0.7333333333333332815, 0.7358974358974359475, 0.7384615384615385025, 0.7410256410256410575, 0.7435897435897436125, 0.7461538461538461675, 0.7487179487179487225, 0.7512820512820512775, 0.7538461538461538325, 0.7564102564102563875, 0.7589743589743589425, 0.7615384615384614975, 0.7641025641025640525, 0.7666666666666667185, 0.7692307692307692735, 0.7717948717948718285, 0.7743589743589743835, 0.7769230769230769384, 0.7794871794871794934, 0.7820512820512820484, 0.7846153846153846034, 0.7871794871794871584, 0.7897435897435897134, 0.7923076923076922684, 0.7948717948717948234, 0.7974358974358974894, 0.8000000000000000444, 0.8025641025641025994, 0.8051282051282051544, 0.8076923076923077094, 0.8102564102564102644, 0.8128205128205128194, 0.8153846153846153744, 0.8179487179487179294, 0.8205128205128204844, 0.8230769230769230393, 0.8256410256410255943, 0.8282051282051282604, 0.8307692307692308153, 0.8333333333333333703, 0.8358974358974359253, 0.8384615384615384803, 0.8410256410256410353, 0.8435897435897435903, 0.8461538461538461453, 0.8487179487179487003, 0.8512820512820512553, 0.8538461538461538103, 0.8564102564102563653, 0.8589743589743589203, 0.8615384615384615863, 0.8641025641025641413, 0.8666666666666666963, 0.8692307692307692513, 0.8717948717948718063, 0.8743589743589743613, 0.8769230769230769162, 0.8794871794871794712, 0.8820512820512820262, 0.8846153846153845812, 0.8871794871794871362, 0.8897435897435896912, 0.8923076923076923572, 0.8948717948717949122, 0.8974358974358974672, 0.9000000000000000222, 0.9025641025641025772, 0.9051282051282051322, 0.9076923076923076872, 0.9102564102564102422, 0.9128205128205127972, 0.9153846153846153522, 0.9179487179487179072, 0.9205128205128204621, 0.9230769230769231282, 0.9256410256410256832, 0.9282051282051282382, 0.9307692307692307931, 0.9333333333333333481, 0.9358974358974359031, 0.9384615384615384581, 0.9410256410256410131, 0.9435897435897435681, 0.9461538461538461231, 0.9487179487179486781, 0.9512820512820512331, 0.9538461538461538991, 0.9564102564102564541, 0.9589743589743590091, 0.9615384615384615641, 0.9641025641025641191, 0.9666666666666666741, 0.9692307692307692291, 0.9717948717948717841, 0.9743589743589743390, 0.9769230769230768940, 0.9794871794871794490, 0.9820512820512820040, 0.9846153846153846700, 0.9871794871794872250, 0.9897435897435897800, 0.9923076923076923350, 0.9948717948717948900, 0.9974358974358974450, 1.000000000000000000 ),
 .UNSPECIFIED. ) 
 GEOMETRIC_REPRESENTATION_ITEM ( )  RATIONAL_B_SPLINE_SURFACE ( (
 ( 1.000000000000000000, 0.9510565162951535312, 1.000000000000000000, 0.9510565162951535312, 1.000000000000000000, 0.9510565162951535312, 1.000000000000000000, 0.9510565162951535312, 1.000000000000000000, 0.9510565162951535312, 1.000000000000000000, 0.9510565162951535312, 1.000000000000000000, 0.9510565162951535312, 1.000000000000000000, 0.9510565162951535312, 1.000000000000000000, 0.9510565162951535312, 1.000000000000000000, 0.9510565162951535312, 1.000000000000000000, 0.9510565162951535312, 1.000000000000000000, 0.9510565162951535312, 1.000000000000000000, 0.9510565162951535312, 1.000000000000000000, 0.9510565162951535312, 1.000000000000000000, 0.9510565162951535312, 1.000000000000000000, 0.9510565162951535312, 1.000000000000000000, 0.9510565162951535312, 1.000000000000000000, 0.9510565162951535312, 1.000000000000000000, 0.9510565162951535312, 1.000000000000000000, 0.9510565162951535312, 1.000000000000000000, 0.9510565162951535312, 1.000000000000000000, 0.9510565162951535312, 1.000000000000000000, 0.9510565162951535312, 1.000000000000000000, 0.9510565162951535312, 1.000000000000000000, 0.9510565162951535312, 1.000000000000000000, 0.9510565162951535312, 1.000000000000000000, 0.9510565162951535312, 1.000000000000000000, 0.9510565162951535312, 1.000000000000000000, 0.9510565162951535312, 1.000000000000000000, 0.9510565162951535312, 1.000000000000000000, 0.9510565162951535312, 1.000000000000000000, 0.9510565162951535312, 1.000000000000000000, 0.9510565162951535312, 1.000000000000000000, 0.9510565162951535312, 1.000000000000000000, 0.9510565162951535312, 1.000000000000000000, 0.9510565162951535312, 1.000000000000000000, 0.9510565162951535312, 1.000000000000000000, 0.9510565162951535312, 1.000000000000000000, 0.9510565162951535312, 1.000000000000000000, 0.9510565162951535312, 1.000000000000000000, 0.9510565162951535312, 1.000000000000000000, 0.9510565162951535312, 1.000000000000000000, 0.9510565162951535312, 1.000000000000000000, 0.9510565162951535312, 1.000000000000000000, 0.9510565162951535312, 1.000000000000000000, 0.9510565162951535312, 1.000000000000000000, 0.9510565162951535312, 1.000000000000000000, 0.9510565162951535312, 1.000000000000000000, 0.9510565162951535312, 1.000000000000000000, 0.9510565162951535312, 1.000000000000000000, 0.9510565162951535312, 1.000000000000000000, 0.9510565162951535312, 1.000000000000000000, 0.9510565162951535312, 1.000000000000000000, 0.9510565162951535312, 1.000000000000000000, 0.9510565162951535312, 1.000000000000000000, 0.9510565162951535312, 1.000000000000000000, 0.9510565162951535312, 1.000000000000000000, 0.9510565162951535312, 1.000000000000000000, 0.9510565162951535312, 1.000000000000000000, 0.9510565162951535312, 1.000000000000000000, 0.9510565162951535312, 1.000000000000000000, 0.9510565162951535312, 1.000000000000000000, 0.9510565162951535312, 1.000000000000000000, 0.9510565162951535312, 1.000000000000000000, 0.9510565162951535312, 1.000000000000000000, 0.9510565162951535312, 1.000000000000000000, 0.9510565162951535312, 1.000000000000000000, 0.9510565162951535312, 1.000000000000000000, 0.9510565162951535312, 1.000000000000000000, 0.9510565162951535312, 1.000000000000000000, 0.9510565162951535312, 1.000000000000000000, 0.9510565162951535312, 1.000000000000000000, 0.9510565162951535312, 1.000000000000000000, 0.9510565162951535312, 1.000000000000000000, 0.9510565162951535312, 1.000000000000000000, 0.9510565162951535312, 1.000000000000000000, 0.9510565162951535312, 1.000000000000000000, 0.9510565162951535312, 1.000000000000000000, 0.9510565162951535312, 1.000000000000000000, 0.9510565162951535312, 1.000000000000000000, 0.9510565162951535312, 1.000000000000000000, 0.9510565162951535312, 1.000000000000000000, 0.9510565162951535312, 1.000000000000000000, 0.9510565162951535312, 1.000000000000000000, 0.9510565162951535312, 1.000000000000000000, 0.9510565162951535312, 1.000000000000000000, 0.9510565162951535312, 1.000000000000000000, 0.9510565162951535312, 1.000000000000000000, 0.9510565162951535312, 1.000000000000000000, 0.9510565162951535312, 1.000000000000000000, 0.9510565162951535312, 1.000000000000000000, 0.9510565162951535312, 1.000000000000000000, 0.9510565162951535312, 1.000000000000000000, 0.9510565162951535312, 1.000000000000000000, 0.9510565162951535312, 1.000000000000000000, 0.9510565162951535312, 1.000000000000000000, 0.9510565162951535312, 1.000000000000000000, 0.9510565162951535312, 1.000000000000000000, 0.9510565162951535312, 1.000000000000000000, 0.9510565162951535312, 1.000000000000000000, 0.9510565162951535312, 1.000000000000000000, 0.9510565162951535312, 1.000000000000000000, 0.9510565162951535312, 1.000000000000000000, 0.9510565162951535312, 1.000000000000000000, 0.9510565162951535312, 1.000000000000000000, 0.9510565162951535312, 1.000000000000000000, 0.9510565162951535312, 1.000000000000000000, 0.9510565162951535312, 1.000000000000000000, 0.9510565162951535312, 1.000000000000000000, 0.9510565162951535312, 1.000000000000000000, 0.9510565162951535312, 1.000000000000000000, 0.9510565162951535312, 1.000000000000000000, 0.9510565162951535312, 1.000000000000000000, 0.9510565162951535312, 1.000000000000000000, 0.9510565162951535312, 1.000000000000000000, 0.9510565162951535312, 1.000000000000000000, 0.9510565162951535312, 1.000000000000000000, 0.9510565162951535312, 1.000000000000000000, 0.9510565162951535312, 1.000000000000000000, 0.9510565162951535312, 1.000000000000000000, 0.9510565162951535312, 1.000000000000000000, 0.9510565162951535312, 1.000000000000000000, 0.9510565162951535312, 1.000000000000000000, 0.9510565162951535312, 1.000000000000000000, 0.9510565162951535312, 1.000000000000000000, 0.9510565162951535312, 1.000000000000000000, 0.9510565162951535312, 1.000000000000000000, 0.9510565162951535312, 1.000000000000000000, 0.9510565162951535312, 1.000000000000000000, 0.9510565162951535312, 1.000000000000000000, 0.9510565162951535312, 1.000000000000000000, 0.9510565162951535312, 1.000000000000000000, 0.9510565162951535312, 1.000000000000000000, 0.9510565162951535312, 1.000000000000000000, 0.9510565162951535312, 1.000000000000000000, 0.9510565162951535312, 1.000000000000000000, 0.9510565162951535312, 1.000000000000000000, 0.9510565162951535312, 1.000000000000000000, 0.9510565162951535312, 1.000000000000000000, 0.9510565162951535312, 1.000000000000000000, 0.9510565162951535312, 1.000000000000000000, 0.9510565162951535312, 1.000000000000000000, 0.9510565162951535312, 1.000000000000000000, 0.9510565162951535312, 1.000000000000000000, 0.9510565162951535312, 1.000000000000000000, 0.9510565162951535312, 1.000000000000000000, 0.9510565162951535312, 1.000000000000000000, 0.9510565162951535312, 1.000000000000000000, 0.9510565162951535312, 1.000000000000000000, 0.9510565162951535312, 1.000000000000000000, 0.9510565162951535312, 1.000000000000000000, 0.9510565162951535312, 1.000000000000000000, 0.9510565162951535312, 1.000000000000000000, 0.9510565162951535312, 1.000000000000000000, 0.9510565162951535312, 1.000000000000000000, 0.9510565162951535312, 1.000000000000000000, 0.9510565162951535312, 1.000000000000000000, 0.9510565162951535312, 1.000000000000000000, 0.9510565162951535312, 1.000000000000000000, 0.9510565162951535312, 1.000000000000000000, 0.9510565162951535312, 1.000000000000000000, 0.9510565162951535312, 1.000000000000000000, 0.9510565162951535312, 1.000000000000000000, 0.9510565162951535312, 1.000000000000000000, 0.9510565162951535312, 1.000000000000000000, 0.9510565162951535312, 1.000000000000000000, 0.9510565162951535312, 1.000000000000000000, 0.9510565162951535312, 1.000000000000000000, 0.9510565162951535312, 1.000000000000000000, 0.9510565162951535312, 1.000000000000000000, 0.9510565162951535312, 1.000000000000000000, 0.9510565162951535312, 1.000000000000000000, 0.9510565162951535312, 1.000000000000000000, 0.9510565162951535312, 1.000000000000000000, 0.9510565162951535312, 1.000000000000000000, 0.9510565162951535312, 1.000000000000000000, 0.9510565162951535312, 1.000000000000000000, 0.9510565162951535312, 1.000000000000000000, 0.9510565162951535312, 1.000000000000000000, 0.9510565162951535312, 1.000000000000000000, 0.9510565162951535312, 1.000000000000000000, 0.9510565162951535312, 1.000000000000000000, 0.9510565162951535312, 1.000000000000000000, 0.9510565162951535312, 1.000000000000000000, 0.9510565162951535312, 1.000000000000000000, 0.9510565162951535312, 1.000000000000000000, 0.9510565162951535312, 1.000000000000000000, 0.9510565162951535312, 1.000000000000000000, 0.9510565162951535312, 1.000000000000000000, 0.9510565162951535312, 1.000000000000000000, 0.9510565162951535312, 1.000000000000000000, 0.9510565162951535312, 1.000000000000000000, 0.9510565162951535312, 1.000000000000000000, 0.9510565162951535312, 1.000000000000000000, 0.9510565162951535312, 1.000000000000000000, 0.9510565162951535312, 1.000000000000000000, 0.9510565162951535312, 1.000000000000000000, 0.9510565162951535312, 1.000000000000000000, 0.9510565162951535312, 1.000000000000000000, 0.9510565162951535312, 1.000000000000000000, 0.9510565162951535312, 1.000000000000000000, 0.9510565162951535312, 1.000000000000000000, 0.9510565162951535312, 1.000000000000000000, 0.9510565162951535312, 1.000000000000000000, 0.9510565162951535312, 1.000000000000000000, 0.9510565162951535312, 1.000000000000000000, 0.9510565162951535312, 1.000000000000000000, 0.9510565162951535312, 1.000000000000000000, 0.9510565162951535312, 1.000000000000000000, 0.9510565162951535312, 1.000000000000000000, 0.9510565162951535312, 1.000000000000000000, 0.9510565162951535312, 1.000000000000000000, 0.9510565162951535312, 1.000000000000000000, 0.9510565162951535312, 1.000000000000000000, 0.9510565162951535312, 1.000000000000000000, 0.9510565162951535312, 1.000000000000000000, 0.9510565162951535312, 1.000000000000000000, 0.9510565162951535312, 1.000000000000000000, 0.9510565162951535312, 1.000000000000000000, 0.9510565162951535312, 1.000000000000000000, 0.9510565162951535312, 1.000000000000000000, 0.9510565162951535312, 1.000000000000000000, 0.9510565162951535312, 1.000000000000000000, 0.9510565162951535312, 1.000000000000000000, 0.9510565162951535312, 1.000000000000000000, 0.9510565162951535312, 1.000000000000000000, 0.9510565162951535312, 1.000000000000000000, 0.9510565162951535312, 1.000000000000000000, 0.9510565162951535312, 1.000000000000000000, 0.9510565162951535312, 1.000000000000000000, 0.9510565162951535312, 1.000000000000000000, 0.9510565162951535312, 1.000000000000000000, 0.9510565162951535312, 1.000000000000000000, 0.9510565162951535312, 1.000000000000000000, 0.9510565162951535312, 1.000000000000000000, 0.9510565162951535312, 1.000000000000000000, 0.9510565162951535312, 1.000000000000000000, 0.9510565162951535312, 1.000000000000000000, 0.9510565162951535312, 1.000000000000000000, 0.9510565162951535312, 1.000000000000000000, 0.9510565162951535312, 1.000000000000000000, 0.9510565162951535312, 1.000000000000000000, 0.9510565162951535312, 1.000000000000000000, 0.9510565162951535312, 1.000000000000000000, 0.9510565162951535312, 1.000000000000000000, 0.9510565162951535312, 1.000000000000000000, 0.9510565162951535312, 1.000000000000000000, 0.9510565162951535312, 1.000000000000000000, 0.9510565162951535312, 1.000000000000000000, 0.9510565162951535312, 1.000000000000000000, 0.9510565162951535312, 1.000000000000000000, 0.9510565162951535312, 1.000000000000000000, 0.9510565162951535312, 1.000000000000000000, 0.9510565162951535312, 1.000000000000000000, 0.9510565162951535312, 1.000000000000000000, 0.9510565162951535312, 1.000000000000000000, 0.9510565162951535312, 1.000000000000000000, 0.9510565162951535312, 1.000000000000000000, 0.9510565162951535312, 1.000000000000000000, 0.9510565162951535312, 1.000000000000000000, 0.9510565162951535312, 1.000000000000000000, 0.9510565162951535312, 1.000000000000000000, 0.9510565162951535312, 1.000000000000000000, 0.9510565162951535312, 1.000000000000000000, 0.9510565162951535312, 1.000000000000000000, 0.9510565162951535312, 1.000000000000000000, 0.9510565162951535312, 1.000000000000000000, 0.9510565162951535312, 1.000000000000000000, 0.9510565162951535312, 1.000000000000000000, 0.9510565162951535312, 1.000000000000000000, 0.9510565162951535312, 1.000000000000000000, 0.9510565162951535312, 1.000000000000000000, 0.9510565162951535312, 1.000000000000000000, 0.9510565162951535312, 1.000000000000000000, 0.9510565162951535312, 1.000000000000000000, 0.9510565162951535312, 1.000000000000000000, 0.9510565162951535312, 1.000000000000000000, 0.9510565162951535312, 1.000000000000000000, 0.9510565162951535312, 1.000000000000000000, 0.9510565162951535312, 1.000000000000000000, 0.9510565162951535312, 1.000000000000000000, 0.9510565162951535312, 1.000000000000000000, 0.9510565162951535312, 1.000000000000000000, 0.9510565162951535312, 1.000000000000000000, 0.9510565162951535312, 1.000000000000000000, 0.9510565162951535312, 1.000000000000000000, 0.9510565162951535312, 1.000000000000000000, 0.9510565162951535312, 1.000000000000000000, 0.9510565162951535312, 1.000000000000000000, 0.9510565162951535312, 1.000000000000000000, 0.9510565162951535312, 1.000000000000000000, 0.9510565162951535312, 1.000000000000000000, 0.9510565162951535312, 1.000000000000000000, 0.9510565162951535312, 1.000000000000000000, 0.9510565162951535312, 1.000000000000000000, 0.9510565162951535312, 1.000000000000000000, 0.9510565162951535312, 1.000000000000000000, 0.9510565162951535312, 1.000000000000000000, 0.9510565162951535312, 1.000000000000000000, 0.9510565162951535312, 1.000000000000000000, 0.9510565162951535312, 1.000000000000000000, 0.9510565162951535312, 1.000000000000000000, 0.9510565162951535312, 1.000000000000000000, 0.9510565162951535312, 1.000000000000000000, 0.9510565162951535312, 1.000000000000000000, 0.9510565162951535312, 1.000000000000000000, 0.9510565162951535312, 1.000000000000000000, 0.9510565162951535312, 1.000000000000000000, 0.9510565162951535312, 1.000000000000000000, 0.9510565162951535312, 1.000000000000000000, 0.9510565162951535312, 1.000000000000000000, 0.9510565162951535312, 1.000000000000000000, 0.9510565162951535312, 1.000000000000000000, 0.9510565162951535312, 1.000000000000000000, 0.9510565162951535312, 1.000000000000000000, 0.9510565162951535312, 1.000000000000000000, 0.9510565162951535312, 1.000000000000000000, 0.9510565162951535312, 1.000000000000000000, 0.9510565162951535312, 1.000000000000000000, 0.9510565162951535312, 1.000000000000000000, 0.9510565162951535312, 1.000000000000000000, 0.9510565162951535312, 1.000000000000000000, 0.9510565162951535312, 1.000000000000000000, 0.9510565162951535312, 1.000000000000000000, 0.9510565162951535312, 1.000000000000000000, 0.9510565162951535312, 1.000000000000000000, 0.9510565162951535312, 1.000000000000000000, 0.9510565162951535312, 1.000000000000000000, 0.9510565162951535312, 1.000000000000000000, 0.9510565162951535312, 1.000000000000000000, 0.9510565162951535312, 1.000000000000000000, 0.9510565162951535312, 1.000000000000000000, 0.9510565162951535312, 1.000000000000000000, 0.9510565162951535312, 1.000000000000000000, 0.9510565162951535312, 1.000000000000000000, 0.9510565162951535312, 1.000000000000000000, 0.9510565162951535312, 1.000000000000000000, 0.9510565162951535312, 1.000000000000000000, 0.9510565162951535312, 1.000000000000000000, 0.9510565162951535312, 1.000000000000000000, 0.9510565162951535312, 1.000000000000000000, 0.9510565162951535312, 1.000000000000000000, 0.9510565162951535312, 1.000000000000000000, 0.9510565162951535312, 1.000000000000000000, 0.9510565162951535312, 1.000000000000000000, 0.9510565162951535312, 1.000000000000000000, 0.9510565162951535312, 1.000000000000000000, 0.9510565162951535312, 1.000000000000000000, 0.9510565162951535312, 1.000000000000000000, 0.9510565162951535312, 1.000000000000000000, 0.9510565162951535312, 1.000000000000000000, 0.9510565162951535312, 1.000000000000000000, 0.9510565162951535312, 1.000000000000000000, 0.9510565162951535312, 1.000000000000000000, 0.9510565162951535312, 1.000000000000000000, 0.9510565162951535312, 1.000000000000000000, 0.9510565162951535312, 1.000000000000000000, 0.9510565162951535312, 1.000000000000000000, 0.9510565162951535312, 1.000000000000000000, 0.9510565162951535312, 1.000000000000000000, 0.9510565162951535312, 1.000000000000000000, 0.9510565162951535312, 1.000000000000000000, 0.9510565162951535312, 1.000000000000000000, 0.9510565162951535312, 1.000000000000000000, 0.9510565162951535312, 1.000000000000000000, 0.9510565162951535312, 1.000000000000000000, 0.9510565162951535312, 1.000000000000000000, 0.9510565162951535312, 1.000000000000000000, 0.9510565162951535312, 1.000000000000000000, 0.9510565162951535312, 1.000000000000000000, 0.9510565162951535312, 1.000000000000000000, 0.9510565162951535312, 1.000000000000000000, 0.9510565162951535312, 1.000000000000000000, 0.9510565162951535312, 1.000000000000000000, 0.9510565162951535312, 1.000000000000000000, 0.9510565162951535312, 1.000000000000000000, 0.9510565162951535312, 1.000000000000000000, 0.9510565162951535312, 1.000000000000000000, 0.9510565162951535312, 1.000000000000000000, 0.9510565162951535312, 1.000000000000000000, 0.9510565162951535312, 1.000000000000000000, 0.9510565162951535312, 1.000000000000000000, 0.9510565162951535312, 1.000000000000000000, 0.9510565162951535312, 1.000000000000000000, 0.9510565162951535312, 1.000000000000000000, 0.9510565162951535312, 1.000000000000000000, 0.9510565162951535312, 1.000000000000000000, 0.9510565162951535312, 1.000000000000000000, 0.9510565162951535312, 1.000000000000000000, 0.9510565162951535312, 1.000000000000000000),
 ( 1.000000000000000000, 0.9510565162951535312, 1.000000000000000000, 0.9510565162951535312, 1.000000000000000000, 0.9510565162951535312, 1.000000000000000000, 0.9510565162951535312, 1.000000000000000000, 0.9510565162951535312, 1.000000000000000000, 0.9510565162951535312, 1.000000000000000000, 0.9510565162951535312, 1.000000000000000000, 0.9510565162951535312, 1.000000000000000000, 0.9510565162951535312, 1.000000000000000000, 0.9510565162951535312, 1.000000000000000000, 0.9510565162951535312, 1.000000000000000000, 0.9510565162951535312, 1.000000000000000000, 0.9510565162951535312, 1.000000000000000000, 0.9510565162951535312, 1.000000000000000000, 0.9510565162951535312, 1.000000000000000000, 0.9510565162951535312, 1.000000000000000000, 0.9510565162951535312, 1.000000000000000000, 0.9510565162951535312, 1.000000000000000000, 0.9510565162951535312, 1.000000000000000000, 0.9510565162951535312, 1.000000000000000000, 0.9510565162951535312, 1.000000000000000000, 0.9510565162951535312, 1.000000000000000000, 0.9510565162951535312, 1.000000000000000000, 0.9510565162951535312, 1.000000000000000000, 0.9510565162951535312, 1.000000000000000000, 0.9510565162951535312, 1.000000000000000000, 0.9510565162951535312, 1.000000000000000000, 0.9510565162951535312, 1.000000000000000000, 0.9510565162951535312, 1.000000000000000000, 0.9510565162951535312, 1.000000000000000000, 0.9510565162951535312, 1.000000000000000000, 0.9510565162951535312, 1.000000000000000000, 0.9510565162951535312, 1.000000000000000000, 0.9510565162951535312, 1.000000000000000000, 0.9510565162951535312, 1.000000000000000000, 0.9510565162951535312, 1.000000000000000000, 0.9510565162951535312, 1.000000000000000000, 0.9510565162951535312, 1.000000000000000000, 0.9510565162951535312, 1.000000000000000000, 0.9510565162951535312, 1.000000000000000000, 0.9510565162951535312, 1.000000000000000000, 0.9510565162951535312, 1.000000000000000000, 0.9510565162951535312, 1.000000000000000000, 0.9510565162951535312, 1.000000000000000000, 0.9510565162951535312, 1.000000000000000000, 0.9510565162951535312, 1.000000000000000000, 0.9510565162951535312, 1.000000000000000000, 0.9510565162951535312, 1.000000000000000000, 0.9510565162951535312, 1.000000000000000000, 0.9510565162951535312, 1.000000000000000000, 0.9510565162951535312, 1.000000000000000000, 0.9510565162951535312, 1.000000000000000000, 0.9510565162951535312, 1.000000000000000000, 0.9510565162951535312, 1.000000000000000000, 0.9510565162951535312, 1.000000000000000000, 0.9510565162951535312, 1.000000000000000000, 0.9510565162951535312, 1.000000000000000000, 0.9510565162951535312, 1.000000000000000000, 0.9510565162951535312, 1.000000000000000000, 0.9510565162951535312, 1.000000000000000000, 0.9510565162951535312, 1.000000000000000000, 0.9510565162951535312, 1.000000000000000000, 0.9510565162951535312, 1.000000000000000000, 0.9510565162951535312, 1.000000000000000000, 0.9510565162951535312, 1.000000000000000000, 0.9510565162951535312, 1.000000000000000000, 0.9510565162951535312, 1.000000000000000000, 0.9510565162951535312, 1.000000000000000000, 0.9510565162951535312, 1.000000000000000000, 0.9510565162951535312, 1.000000000000000000, 0.9510565162951535312, 1.000000000000000000, 0.9510565162951535312, 1.000000000000000000, 0.9510565162951535312, 1.000000000000000000, 0.9510565162951535312, 1.000000000000000000, 0.9510565162951535312, 1.000000000000000000, 0.9510565162951535312, 1.000000000000000000, 0.9510565162951535312, 1.000000000000000000, 0.9510565162951535312, 1.000000000000000000, 0.9510565162951535312, 1.000000000000000000, 0.9510565162951535312, 1.000000000000000000, 0.9510565162951535312, 1.000000000000000000, 0.9510565162951535312, 1.000000000000000000, 0.9510565162951535312, 1.000000000000000000, 0.9510565162951535312, 1.000000000000000000, 0.9510565162951535312, 1.000000000000000000, 0.9510565162951535312, 1.000000000000000000, 0.9510565162951535312, 1.000000000000000000, 0.9510565162951535312, 1.000000000000000000, 0.9510565162951535312, 1.000000000000000000, 0.9510565162951535312, 1.000000000000000000, 0.9510565162951535312, 1.000000000000000000, 0.9510565162951535312, 1.000000000000000000, 0.9510565162951535312, 1.000000000000000000, 0.9510565162951535312, 1.000000000000000000, 0.9510565162951535312, 1.000000000000000000, 0.9510565162951535312, 1.000000000000000000, 0.9510565162951535312, 1.000000000000000000, 0.9510565162951535312, 1.000000000000000000, 0.9510565162951535312, 1.000000000000000000, 0.9510565162951535312, 1.000000000000000000, 0.9510565162951535312, 1.000000000000000000, 0.9510565162951535312, 1.000000000000000000, 0.9510565162951535312, 1.000000000000000000, 0.9510565162951535312, 1.000000000000000000, 0.9510565162951535312, 1.000000000000000000, 0.9510565162951535312, 1.000000000000000000, 0.9510565162951535312, 1.000000000000000000, 0.9510565162951535312, 1.000000000000000000, 0.9510565162951535312, 1.000000000000000000, 0.9510565162951535312, 1.000000000000000000, 0.9510565162951535312, 1.000000000000000000, 0.9510565162951535312, 1.000000000000000000, 0.9510565162951535312, 1.000000000000000000, 0.9510565162951535312, 1.000000000000000000, 0.9510565162951535312, 1.000000000000000000, 0.9510565162951535312, 1.000000000000000000, 0.9510565162951535312, 1.000000000000000000, 0.9510565162951535312, 1.000000000000000000, 0.9510565162951535312, 1.000000000000000000, 0.9510565162951535312, 1.000000000000000000, 0.9510565162951535312, 1.000000000000000000, 0.9510565162951535312, 1.000000000000000000, 0.9510565162951535312, 1.000000000000000000, 0.9510565162951535312, 1.000000000000000000, 0.9510565162951535312, 1.000000000000000000, 0.9510565162951535312, 1.000000000000000000, 0.9510565162951535312, 1.000000000000000000, 0.9510565162951535312, 1.000000000000000000, 0.9510565162951535312, 1.000000000000000000, 0.9510565162951535312, 1.000000000000000000, 0.9510565162951535312, 1.000000000000000000, 0.9510565162951535312, 1.000000000000000000, 0.9510565162951535312, 1.000000000000000000, 0.9510565162951535312, 1.000000000000000000, 0.9510565162951535312, 1.000000000000000000, 0.9510565162951535312, 1.000000000000000000, 0.9510565162951535312, 1.000000000000000000, 0.9510565162951535312, 1.000000000000000000, 0.9510565162951535312, 1.000000000000000000, 0.9510565162951535312, 1.000000000000000000, 0.9510565162951535312, 1.000000000000000000, 0.9510565162951535312, 1.000000000000000000, 0.9510565162951535312, 1.000000000000000000, 0.9510565162951535312, 1.000000000000000000, 0.9510565162951535312, 1.000000000000000000, 0.9510565162951535312, 1.000000000000000000, 0.9510565162951535312, 1.000000000000000000, 0.9510565162951535312, 1.000000000000000000, 0.9510565162951535312, 1.000000000000000000, 0.9510565162951535312, 1.000000000000000000, 0.9510565162951535312, 1.000000000000000000, 0.9510565162951535312, 1.000000000000000000, 0.9510565162951535312, 1.000000000000000000, 0.9510565162951535312, 1.000000000000000000, 0.9510565162951535312, 1.000000000000000000, 0.9510565162951535312, 1.000000000000000000, 0.9510565162951535312, 1.000000000000000000, 0.9510565162951535312, 1.000000000000000000, 0.9510565162951535312, 1.000000000000000000, 0.9510565162951535312, 1.000000000000000000, 0.9510565162951535312, 1.000000000000000000, 0.9510565162951535312, 1.000000000000000000, 0.9510565162951535312, 1.000000000000000000, 0.9510565162951535312, 1.000000000000000000, 0.9510565162951535312, 1.000000000000000000, 0.9510565162951535312, 1.000000000000000000, 0.9510565162951535312, 1.000000000000000000, 0.9510565162951535312, 1.000000000000000000, 0.9510565162951535312, 1.000000000000000000, 0.9510565162951535312, 1.000000000000000000, 0.9510565162951535312, 1.000000000000000000, 0.9510565162951535312, 1.000000000000000000, 0.9510565162951535312, 1.000000000000000000, 0.9510565162951535312, 1.000000000000000000, 0.9510565162951535312, 1.000000000000000000, 0.9510565162951535312, 1.000000000000000000, 0.9510565162951535312, 1.000000000000000000, 0.9510565162951535312, 1.000000000000000000, 0.9510565162951535312, 1.000000000000000000, 0.9510565162951535312, 1.000000000000000000, 0.9510565162951535312, 1.000000000000000000, 0.9510565162951535312, 1.000000000000000000, 0.9510565162951535312, 1.000000000000000000, 0.9510565162951535312, 1.000000000000000000, 0.9510565162951535312, 1.000000000000000000, 0.9510565162951535312, 1.000000000000000000, 0.9510565162951535312, 1.000000000000000000, 0.9510565162951535312, 1.000000000000000000, 0.9510565162951535312, 1.000000000000000000, 0.9510565162951535312, 1.000000000000000000, 0.9510565162951535312, 1.000000000000000000, 0.9510565162951535312, 1.000000000000000000, 0.9510565162951535312, 1.000000000000000000, 0.9510565162951535312, 1.000000000000000000, 0.9510565162951535312, 1.000000000000000000, 0.9510565162951535312, 1.000000000000000000, 0.9510565162951535312, 1.000000000000000000, 0.9510565162951535312, 1.000000000000000000, 0.9510565162951535312, 1.000000000000000000, 0.9510565162951535312, 1.000000000000000000, 0.9510565162951535312, 1.000000000000000000, 0.9510565162951535312, 1.000000000000000000, 0.9510565162951535312, 1.000000000000000000, 0.9510565162951535312, 1.000000000000000000, 0.9510565162951535312, 1.000000000000000000, 0.9510565162951535312, 1.000000000000000000, 0.9510565162951535312, 1.000000000000000000, 0.9510565162951535312, 1.000000000000000000, 0.9510565162951535312, 1.000000000000000000, 0.9510565162951535312, 1.000000000000000000, 0.9510565162951535312, 1.000000000000000000, 0.9510565162951535312, 1.000000000000000000, 0.9510565162951535312, 1.000000000000000000, 0.9510565162951535312, 1.000000000000000000, 0.9510565162951535312, 1.000000000000000000, 0.9510565162951535312, 1.000000000000000000, 0.9510565162951535312, 1.000000000000000000, 0.9510565162951535312, 1.000000000000000000, 0.9510565162951535312, 1.000000000000000000, 0.9510565162951535312, 1.000000000000000000, 0.9510565162951535312, 1.000000000000000000, 0.9510565162951535312, 1.000000000000000000, 0.9510565162951535312, 1.000000000000000000, 0.9510565162951535312, 1.000000000000000000, 0.9510565162951535312, 1.000000000000000000, 0.9510565162951535312, 1.000000000000000000, 0.9510565162951535312, 1.000000000000000000, 0.9510565162951535312, 1.000000000000000000, 0.9510565162951535312, 1.000000000000000000, 0.9510565162951535312, 1.000000000000000000, 0.9510565162951535312, 1.000000000000000000, 0.9510565162951535312, 1.000000000000000000, 0.9510565162951535312, 1.000000000000000000, 0.9510565162951535312, 1.000000000000000000, 0.9510565162951535312, 1.000000000000000000, 0.9510565162951535312, 1.000000000000000000, 0.9510565162951535312, 1.000000000000000000, 0.9510565162951535312, 1.000000000000000000, 0.9510565162951535312, 1.000000000000000000, 0.9510565162951535312, 1.000000000000000000, 0.9510565162951535312, 1.000000000000000000, 0.9510565162951535312, 1.000000000000000000, 0.9510565162951535312, 1.000000000000000000, 0.9510565162951535312, 1.000000000000000000, 0.9510565162951535312, 1.000000000000000000, 0.9510565162951535312, 1.000000000000000000, 0.9510565162951535312, 1.000000000000000000, 0.9510565162951535312, 1.000000000000000000, 0.9510565162951535312, 1.000000000000000000, 0.9510565162951535312, 1.000000000000000000, 0.9510565162951535312, 1.000000000000000000, 0.9510565162951535312, 1.000000000000000000, 0.9510565162951535312, 1.000000000000000000, 0.9510565162951535312, 1.000000000000000000, 0.9510565162951535312, 1.000000000000000000, 0.9510565162951535312, 1.000000000000000000, 0.9510565162951535312, 1.000000000000000000, 0.9510565162951535312, 1.000000000000000000, 0.9510565162951535312, 1.000000000000000000, 0.9510565162951535312, 1.000000000000000000, 0.9510565162951535312, 1.000000000000000000, 0.9510565162951535312, 1.000000000000000000, 0.9510565162951535312, 1.000000000000000000, 0.9510565162951535312, 1.000000000000000000, 0.9510565162951535312, 1.000000000000000000, 0.9510565162951535312, 1.000000000000000000, 0.9510565162951535312, 1.000000000000000000, 0.9510565162951535312, 1.000000000000000000, 0.9510565162951535312, 1.000000000000000000, 0.9510565162951535312, 1.000000000000000000, 0.9510565162951535312, 1.000000000000000000, 0.9510565162951535312, 1.000000000000000000, 0.9510565162951535312, 1.000000000000000000, 0.9510565162951535312, 1.000000000000000000, 0.9510565162951535312, 1.000000000000000000, 0.9510565162951535312, 1.000000000000000000, 0.9510565162951535312, 1.000000000000000000, 0.9510565162951535312, 1.000000000000000000, 0.9510565162951535312, 1.000000000000000000, 0.9510565162951535312, 1.000000000000000000, 0.9510565162951535312, 1.000000000000000000, 0.9510565162951535312, 1.000000000000000000, 0.9510565162951535312, 1.000000000000000000, 0.9510565162951535312, 1.000000000000000000, 0.9510565162951535312, 1.000000000000000000, 0.9510565162951535312, 1.000000000000000000, 0.9510565162951535312, 1.000000000000000000, 0.9510565162951535312, 1.000000000000000000, 0.9510565162951535312, 1.000000000000000000, 0.9510565162951535312, 1.000000000000000000, 0.9510565162951535312, 1.000000000000000000, 0.9510565162951535312, 1.000000000000000000, 0.9510565162951535312, 1.000000000000000000, 0.9510565162951535312, 1.000000000000000000, 0.9510565162951535312, 1.000000000000000000, 0.9510565162951535312, 1.000000000000000000, 0.9510565162951535312, 1.000000000000000000, 0.9510565162951535312, 1.000000000000000000, 0.9510565162951535312, 1.000000000000000000, 0.9510565162951535312, 1.000000000000000000, 0.9510565162951535312, 1.000000000000000000, 0.9510565162951535312, 1.000000000000000000, 0.9510565162951535312, 1.000000000000000000, 0.9510565162951535312, 1.000000000000000000, 0.9510565162951535312, 1.000000000000000000, 0.9510565162951535312, 1.000000000000000000, 0.9510565162951535312, 1.000000000000000000, 0.9510565162951535312, 1.000000000000000000, 0.9510565162951535312, 1.000000000000000000, 0.9510565162951535312, 1.000000000000000000, 0.9510565162951535312, 1.000000000000000000, 0.9510565162951535312, 1.000000000000000000, 0.9510565162951535312, 1.000000000000000000, 0.9510565162951535312, 1.000000000000000000, 0.9510565162951535312, 1.000000000000000000, 0.9510565162951535312, 1.000000000000000000, 0.9510565162951535312, 1.000000000000000000, 0.9510565162951535312, 1.000000000000000000, 0.9510565162951535312, 1.000000000000000000, 0.9510565162951535312, 1.000000000000000000, 0.9510565162951535312, 1.000000000000000000, 0.9510565162951535312, 1.000000000000000000, 0.9510565162951535312, 1.000000000000000000, 0.9510565162951535312, 1.000000000000000000, 0.9510565162951535312, 1.000000000000000000, 0.9510565162951535312, 1.000000000000000000, 0.9510565162951535312, 1.000000000000000000, 0.9510565162951535312, 1.000000000000000000, 0.9510565162951535312, 1.000000000000000000, 0.9510565162951535312, 1.000000000000000000, 0.9510565162951535312, 1.000000000000000000, 0.9510565162951535312, 1.000000000000000000, 0.9510565162951535312, 1.000000000000000000, 0.9510565162951535312, 1.000000000000000000, 0.9510565162951535312, 1.000000000000000000, 0.9510565162951535312, 1.000000000000000000, 0.9510565162951535312, 1.000000000000000000, 0.9510565162951535312, 1.000000000000000000, 0.9510565162951535312, 1.000000000000000000, 0.9510565162951535312, 1.000000000000000000, 0.9510565162951535312, 1.000000000000000000, 0.9510565162951535312, 1.000000000000000000, 0.9510565162951535312, 1.000000000000000000, 0.9510565162951535312, 1.000000000000000000, 0.9510565162951535312, 1.000000000000000000, 0.9510565162951535312, 1.000000000000000000, 0.9510565162951535312, 1.000000000000000000, 0.9510565162951535312, 1.000000000000000000, 0.9510565162951535312, 1.000000000000000000, 0.9510565162951535312, 1.000000000000000000, 0.9510565162951535312, 1.000000000000000000, 0.9510565162951535312, 1.000000000000000000, 0.9510565162951535312, 1.000000000000000000, 0.9510565162951535312, 1.000000000000000000, 0.9510565162951535312, 1.000000000000000000, 0.9510565162951535312, 1.000000000000000000, 0.9510565162951535312, 1.000000000000000000, 0.9510565162951535312, 1.000000000000000000, 0.9510565162951535312, 1.000000000000000000, 0.9510565162951535312, 1.000000000000000000, 0.9510565162951535312, 1.000000000000000000, 0.9510565162951535312, 1.000000000000000000, 0.9510565162951535312, 1.000000000000000000, 0.9510565162951535312, 1.000000000000000000, 0.9510565162951535312, 1.000000000000000000, 0.9510565162951535312, 1.000000000000000000, 0.9510565162951535312, 1.000000000000000000, 0.9510565162951535312, 1.000000000000000000, 0.9510565162951535312, 1.000000000000000000, 0.9510565162951535312, 1.000000000000000000, 0.9510565162951535312, 1.000000000000000000, 0.9510565162951535312, 1.000000000000000000, 0.9510565162951535312, 1.000000000000000000, 0.9510565162951535312, 1.000000000000000000, 0.9510565162951535312, 1.000000000000000000, 0.9510565162951535312, 1.000000000000000000, 0.9510565162951535312, 1.000000000000000000, 0.9510565162951535312, 1.000000000000000000, 0.9510565162951535312, 1.000000000000000000, 0.9510565162951535312, 1.000000000000000000, 0.9510565162951535312, 1.000000000000000000, 0.9510565162951535312, 1.000000000000000000, 0.9510565162951535312, 1.000000000000000000, 0.9510565162951535312, 1.000000000000000000, 0.9510565162951535312, 1.000000000000000000, 0.9510565162951535312, 1.000000000000000000, 0.9510565162951535312, 1.000000000000000000, 0.9510565162951535312, 1.000000000000000000, 0.9510565162951535312, 1.000000000000000000, 0.9510565162951535312, 1.000000000000000000) ) ) 
 REPRESENTATION_ITEM ( '' )  SURFACE ( )  );
#1442=CARTESIAN_POINT ( 'NONE',  ( -33.58253175000000113, 63.27500000273118985, -10.91162601494193218 ) ) ;
#1444=CARTESIAN_POINT ( 'NONE',  ( -27.16883889988624290, 70.92500000273119554, -19.73931689729374028 ) ) ;
#1446=CARTESIAN_POINT ( 'NONE',  ( -15.14183272437241889, 12.70000000000000639, -20.84094480462497856 ) ) ;
#1447=CARTESIAN_POINT ( 'NONE',  ( 33.58253175000000823, 2.275000002731194293, 10.91162601494192863 ) ) ;
#1448=CARTESIAN_POINT ( 'NONE',  ( -33.58253175000000113, 19.22500000273118204, 10.91162601494193929 ) ) ;
#1449=CARTESIAN_POINT ( 'NONE',  ( -5.147494310547423346, 0.9487457239155284716, 32.50000000000000000 ) ) ;
#1451=CARTESIAN_POINT ( 'NONE',  ( 2.688165632520823219E-15, 71.87500000273121259, 14.63369212191046387 ) ) ;
#1453=CARTESIAN_POINT ( 'NONE',  ( 32.50000000000000711, 22.90000000000000213, 10.55989012756945122 ) ) ;
#1455=CARTESIAN_POINT ( 'NONE',  ( -15.00000000000000000, 78.15000000546235981, -4.873795443493594171 ) ) ;
#1457=EDGE_CURVE ( 'NONE', #7536, #10957, #5384, .T. ) ;
#1458=CARTESIAN_POINT ( 'NONE',  ( 33.58253175000000823, 38.02500000273117564, 10.91162601494192863 ) ) ;
#1461=CARTESIAN_POINT ( 'NONE',  ( -2.162160676586882350E-15, 26.87500000273117706, -35.31076352940722529 ) ) ;
#1462=CARTESIAN_POINT ( 'NONE',  ( 26.29305231718579350, 40.80000000000000426, 19.10302069950537529 ) ) ;
#1464=CARTESIAN_POINT ( 'NONE',  ( -20.08610463437157989, 8.200000005462390718, -27.64615127144129758 ) ) ;
#1466=CARTESIAN_POINT ( 'NONE',  ( -13.91746824999999887, 71.37500000273119838, 0.000000000000000000 ) ) ;
#1468=CARTESIAN_POINT ( 'NONE',  ( 23.41746824999999887, 8.524999997268812635, 7.608796670333735079 ) ) ;
#1474=CARTESIAN_POINT ( 'NONE',  ( -33.58253175000000113, 11.22500000273120335, 10.91162601494193929 ) ) ;
#1475=CARTESIAN_POINT ( 'NONE',  ( 18.94512977948576093, 9.324999997268824004, -13.76444248337722875 ) ) ;
#1477=ORIENTED_EDGE ( 'NONE', *, *, #11880, .F. ) ;
#1484=CARTESIAN_POINT ( 'NONE',  ( -24.50000000000000000, 14.74999999453763166, -3.000384657911015469E-15 ) ) ;
#1485=CARTESIAN_POINT ( 'NONE',  ( 23.41746824999999887, 6.624999997268815832, 0.000000000000000000 ) ) ;
#1486=CARTESIAN_POINT ( 'NONE',  ( 10.37757302488624056, 24.77500000273119696, -31.93888565452638417 ) ) ;
#1487=CARTESIAN_POINT ( 'NONE',  ( 32.50000000000000000, 23.60000000546236976, -10.55989012756945833 ) ) ;
#1488=CARTESIAN_POINT ( 'NONE',  ( -2.092463501923844636E-15, 71.50000000000001421, -34.17252228774368916 ) ) ;
#1490=CARTESIAN_POINT ( 'NONE',  ( -1.778240108872766143E-15, 44.00000000546238255, -32.49999999999999289 ) ) ;
#1492=CARTESIAN_POINT ( 'NONE',  ( 27.16883889988624290, 36.17500000273118843, 19.73931689729373673 ) ) ;
#1495=CARTESIAN_POINT ( 'NONE',  ( -18.94512977948575738, 7.924999997268811214, -13.76444248337723231 ) ) ;
#1496=CARTESIAN_POINT ( 'NONE',  ( -2.092463501923844636E-15, 13.50000000000001066, -34.17252228774368916 ) ) ;
#1499=CARTESIAN_POINT ( 'NONE',  ( -33.58253175000000113, 57.22500000273117848, 10.91162601494193929 ) ) ;
#1500=CARTESIAN_POINT ( 'NONE',  ( 33.58253175000000113, 48.47500000273118559, -10.91162601494193574 ) ) ;
#1502=CARTESIAN_POINT ( 'NONE',  ( 5.147494310547426899, 67.94874572391553613, -32.50000000000000000 ) ) ;
#1505=CARTESIAN_POINT ( 'NONE',  ( -1.778240108872766143E-15, 38.00000000546237544, -32.49999999999999289 ) ) ;
#1506=CARTESIAN_POINT ( 'NONE',  ( -10.04305231718579172, 41.60000000000000142, -30.90933677959248982 ) ) ;
#1510=DIRECTION ( 'NONE',  ( -0.000000000000000000, -1.000000000000000000, -0.000000000000000000 ) ) ;
#1513=CARTESIAN_POINT ( 'NONE',  ( 9.270509831248425314, 70.95000000546235697, 12.75976212528059683 ) ) ;
#1514=CARTESIAN_POINT ( 'NONE',  ( -20.75514604977248112, 29.42500000273118133, 28.56700777964554661 ) ) ;
#1515=CARTESIAN_POINT ( 'NONE',  ( -33.58253175000000113, 65.27500000273117564, -10.91162601494193218 ) ) ;
#1520=VECTOR ( 'NONE', #23993, 1000.000000000000000 ) ;
#1521=FACE_BOUND ( 'NONE', #23198, .T. ) ;
#1522=VERTEX_POINT ( 'NONE', #29217 ) ;
#1527=CARTESIAN_POINT ( 'NONE',  ( 20.08610463437158344, 56.69999999999998153, 27.64615127144129403 ) ) ;
#1528=CARTESIAN_POINT ( 'NONE',  ( -20.75514604977248823, 39.07500000273119412, -28.56700777964554305 ) ) ;
#1529=CARTESIAN_POINT ( 'NONE',  ( -26.29305231718578995, 40.70000000546236407, 19.10302069950538595 ) ) ;
#1531=CARTESIAN_POINT ( 'NONE',  ( -20.75514604977248823, 26.82500000273117280, -28.56700777964554305 ) ) ;
#1532=CARTESIAN_POINT ( 'NONE',  ( 7.313012447739250820E-14, 13.24999999453762456, 24.50000000000000000 ) ) ;
#1533=CARTESIAN_POINT ( 'NONE',  ( -27.16883889988624290, 55.17500000273118133, -19.73931689729374028 ) ) ;
#1535=CARTESIAN_POINT ( 'NONE',  ( -32.50000000000000000, 33.90000000000001279, -10.55989012756945478 ) ) ;
#1537=( BOUNDED_CURVE ( )  B_SPLINE_CURVE ( 2, ( #4163, #14636, #25096, #1573, #8178, #7420, #7240, #1922, #4332, #30927, #25270, #1743, #4674 ),
 .UNSPECIFIED., .F., .T. ) 
 B_SPLINE_CURVE_WITH_KNOTS ( ( 3, 2, 2, 2, 2, 2, 3 ),
 ( 0.08333333333333334259, 0.08888888888888889228, 0.1000000000000000056, 0.1111111111111111049, 0.1222222222222222182, 0.1333333333333333315, 0.1388888888888888673 ),
 .UNSPECIFIED. ) 
 CURVE ( )  GEOMETRIC_REPRESENTATION_ITEM ( )  RATIONAL_B_SPLINE_CURVE ( ( 0.9755282581475768211, 0.9755282581475768211, 1.000000000000000000, 0.9510565162951535312, 1.000000000000000000, 0.9510565162951535312, 1.000000000000000000, 0.9510565162951535312, 1.000000000000000000, 0.9510565162951535312, 1.000000000000000000, 0.9755282581475768211, 0.9755282581475768211 ) ) 
 REPRESENTATION_ITEM ( '' )  );
#1538=CARTESIAN_POINT ( 'NONE',  ( -33.58253175000000113, 79.02500000273118985, -10.91162601494193218 ) ) ;
#1540=CARTESIAN_POINT ( 'NONE',  ( 6.486482029760648627E-15, 67.87500000273118417, 35.31076352940722529 ) ) ;
#1542=ORIENTED_EDGE ( 'NONE', *, *, #10080, .F. ) ;
#1543=CARTESIAN_POINT ( 'NONE',  ( -24.50000000000000355, 2.649999994537616477, -7.960532557706207157 ) ) ;
#1545=CARTESIAN_POINT ( 'NONE',  ( 10.04305231718578817, 47.39999999999999858, -30.90933677959249337 ) ) ;
#1555=CARTESIAN_POINT ( 'NONE',  ( 0.000000000000000000, 80.00000000000001421, -32.50000000000000000 ) ) ;
#1559=VERTEX_POINT ( 'NONE', #5551 ) ;
#1563=CARTESIAN_POINT ( 'NONE',  ( -26.29305231718579350, 60.30000000546237260, -19.10302069950537884 ) ) ;
#1564=ORIENTED_EDGE ( 'NONE', *, *, #32911, .F. ) ;
#1565=CARTESIAN_POINT ( 'NONE',  ( -10.04305231718579172, 74.10000000546237686, -30.90933677959248982 ) ) ;
#1566=CARTESIAN_POINT ( 'NONE',  ( 33.58253175000000113, 50.22500000273118559, -10.91162601494193751 ) ) ;
#1567=CARTESIAN_POINT ( 'NONE',  ( -14.47279130897151589, 15.32499999726880269, -19.92008829642072598 ) ) ;
#1569=CARTESIAN_POINT ( 'NONE',  ( -32.50000000000000000, 10.40000000546237935, -10.55989012756945478 ) ) ;
#1571=CARTESIAN_POINT ( 'NONE',  ( 18.94512977948576093, 13.32499999726882756, -13.76444248337722875 ) ) ;
#1572=CARTESIAN_POINT ( 'NONE',  ( -10.04305231718578462, 54.40000000000000568, 30.90933677959249337 ) ) ;
#1573=CARTESIAN_POINT ( 'NONE',  ( 15.14183272437242067, 1.700000000000004396, 20.84094480462498211 ) ) ;
#1574=CARTESIAN_POINT ( 'NONE',  ( -20.75514604977248112, 19.67500000273119909, 28.56700777964554661 ) ) ;
#1577=CARTESIAN_POINT ( 'NONE',  ( 11.25946833292375793, 71.67500000273119554, 8.180482586598731842 ) ) ;
#1578=CARTESIAN_POINT ( 'NONE',  ( -7.570916362186215665, 13.39999999999999503, 23.30088464923126423 ) ) ;
#1579=CARTESIAN_POINT ( 'NONE',  ( -20.08610463437156923, 22.29999999999999361, 27.64615127144130113 ) ) ;
#1581=VERTEX_POINT ( 'NONE', #10534 ) ;
#1583=CARTESIAN_POINT ( 'NONE',  ( -13.91746824999999532, 70.97500000273116427, 4.522059556121122093 ) ) ;
#1585=ADVANCED_FACE ( 'NONE', ( #13622 ), #23917, .F. ) ;
#1591=CARTESIAN_POINT ( 'NONE',  ( 8.601468415847520532, 74.07500000273120122, 11.83890561707634603 ) ) ;
#1593=CARTESIAN_POINT ( 'NONE',  ( -2.162160676586882350E-15, 52.62500000273117706, -35.31076352940722529 ) ) ;
#1597=CARTESIAN_POINT ( 'NONE',  ( 4.635254915624212657, 78.60000000000000853, 14.26584774442730286 ) ) ;
#1600=DIRECTION ( 'NONE',  ( 1.000000000000000000, 0.000000000000000000, -0.000000000000000000 ) ) ;
#1601=CARTESIAN_POINT ( 'NONE',  ( 18.94512977948576093, 10.82499999726882578, -13.76444248337722875 ) ) ;
#1603=VERTEX_POINT ( 'NONE', #10701 ) ;
#1605=VERTEX_POINT ( 'NONE', #13450 ) ;
#1607=CARTESIAN_POINT ( 'NONE',  ( -20.75514604977248823, 61.07500000273119412, -28.56700777964554305 ) ) ;
#1609=CARTESIAN_POINT ( 'NONE',  ( 33.58253175000000823, 70.02500000273121827, 10.91162601494192863 ) ) ;
#1611=CARTESIAN_POINT ( 'NONE',  ( 24.50000000000000355, 14.09999999999999254, -7.960532557706203605 ) ) ;
#1613=CARTESIAN_POINT ( 'NONE',  ( -33.58253175000000113, 9.225000002731178483, 10.91162601494193929 ) ) ;
#1614=CARTESIAN_POINT ( 'NONE',  ( -4.300734207923755825, 71.27500000273117564, 13.23629886949340673 ) ) ;
#1616=CARTESIAN_POINT ( 'NONE',  ( 26.29305231718578995, 37.20000000000000995, -19.10302069950538240 ) ) ;
#1619=CARTESIAN_POINT ( 'NONE',  ( 32.50000000000000000, 61.50000000546238255, -3.980102097228898626E-15 ) ) ;
#1621=CARTESIAN_POINT ( 'NONE',  ( 4.635254915624212657, 76.85000000546237686, 14.26584774442730286 ) ) ;
#1623=CARTESIAN_POINT ( 'NONE',  ( -27.16883889988624290, 38.92500000273118843, -19.73931689729374028 ) ) ;
#1626=CARTESIAN_POINT ( 'NONE',  ( 27.16883889988623935, 30.57500000273119412, -19.73931689729374384 ) ) ;
#1627=CARTESIAN_POINT ( 'NONE',  ( 7.313012447739250820E-14, 17.24999999453762456, 24.50000000000000000 ) ) ;
#1628=CARTESIAN_POINT ( 'NONE',  ( -10.04305231718578462, 8.900000005462372243, 30.90933677959249337 ) ) ;
#1629=CARTESIAN_POINT ( 'NONE',  ( 20.08610463437157279, 33.29999999999999716, -27.64615127144129758 ) ) ;
#1631=CARTESIAN_POINT ( 'NONE',  ( -18.94512977948576093, 9.824999997268824004, 13.76444248337722698 ) ) ;
#1633=( BOUNDED_CURVE ( )  B_SPLINE_CURVE ( 2, ( #18273, #5216, #2647, #23584, #49, #18945, #24413 ),
 .UNSPECIFIED., .F., .T. ) 
 B_SPLINE_CURVE_WITH_KNOTS ( ( 3, 2, 2, 3 ),
 ( 0.9499999999999999556, 0.9599999999999999645, 0.9799999999999999822, 1.000000000000000000 ),
 .UNSPECIFIED. ) 
 CURVE ( )  GEOMETRIC_REPRESENTATION_ITEM ( )  RATIONAL_B_SPLINE_CURVE ( ( 0.9755282581475768211, 0.9755282581475768211, 1.000000000000000000, 0.9510565162951535312, 1.000000000000000000, 0.9510565162951535312, 1.000000000000000000 ) ) 
 REPRESENTATION_ITEM ( '' )  );
#1637=( BOUNDED_CURVE ( )  B_SPLINE_CURVE ( 2, ( #30999, #31340, #15055, #10413, #9723, #7497, #7662 ),
 .UNSPECIFIED., .F., .T. ) 
 B_SPLINE_CURVE_WITH_KNOTS ( ( 3, 2, 2, 3 ),
 ( 0.000000000000000000, 0.002564102564102564100, 0.005128205128205128201, 0.006410256410256410901 ),
 .UNSPECIFIED. ) 
 CURVE ( )  GEOMETRIC_REPRESENTATION_ITEM ( )  RATIONAL_B_SPLINE_CURVE ( ( 1.000000000000000000, 0.9510565162951535312, 1.000000000000000000, 0.9510565162951535312, 1.000000000000000000, 0.9755282581475768211, 0.9755282581475768211 ) ) 
 REPRESENTATION_ITEM ( '' )  );
#1638=CARTESIAN_POINT ( 'NONE',  ( -20.75514604977248112, 13.42500000273119198, 28.56700777964554661 ) ) ;
#1639=CARTESIAN_POINT ( 'NONE',  ( 14.47279130897151589, 12.82499999726882400, 19.92008829642072953 ) ) ;
#1641=EDGE_LOOP ( 'NONE', ( #19114, #3299, #32177, #24096 ) ) ;
#1645=ORIENTED_EDGE ( 'NONE', *, *, #18742, .F. ) ;
#1649=CARTESIAN_POINT ( 'NONE',  ( 24.50000000000000355, 13.84999999453764197, -7.960532557706203605 ) ) ;
#1650=ADVANCED_FACE ( 'NONE', ( #31958 ), #29048, .T. ) ;
#1651=CARTESIAN_POINT ( 'NONE',  ( -7.236395654485763274, 10.02499999726880198, 22.27133577429736633 ) ) ;
#1652=CARTESIAN_POINT ( 'NONE',  ( 33.58253175000000113, 22.37500000273118417, -4.112674001490185761E-15 ) ) ;
#1653=CARTESIAN_POINT ( 'NONE',  ( -32.50000000000000000, 26.60000000546239107, 10.55989012756946366 ) ) ;
#1654=CARTESIAN_POINT ( 'NONE',  ( 10.04305231718578817, 69.40000000000001990, -30.90933677959249337 ) ) ;
#1655=CARTESIAN_POINT ( 'NONE',  ( 26.29305231718579350, 47.30000000546235839, 19.10302069950537529 ) ) ;
#1658=CARTESIAN_POINT ( 'NONE',  ( 20.75514604977248467, 34.67500000273118843, -28.56700777964554305 ) ) ;
#1659=CARTESIAN_POINT ( 'NONE',  ( 26.29305231718579350, 43.30000000546238681, 19.10302069950537529 ) ) ;
#1662=CARTESIAN_POINT ( 'NONE',  ( 18.94512977948575738, 12.92499999726881654, 13.76444248337723408 ) ) ;
#1663=CARTESIAN_POINT ( 'NONE',  ( 6.277390505771533514E-15, 12.49999999999998401, 34.17252228774368916 ) ) ;
#1664=CARTESIAN_POINT ( 'NONE',  ( -26.29305231718578995, 52.19999999999999574, 19.10302069950538595 ) ) ;
#1666=CARTESIAN_POINT ( 'NONE',  ( -10.37757302488623701, 55.52500000273119696, 31.93888565452638417 ) ) ;
#1668=CARTESIAN_POINT ( 'NONE',  ( 20.75514604977249178, 48.07500000273120122, 28.56700777964553950 ) ) ;
#1670=CARTESIAN_POINT ( 'NONE',  ( 32.50000000000000711, 67.40000000546240244, 10.55989012756945122 ) ) ;
#1671=CARTESIAN_POINT ( 'NONE',  ( 5.779280353836490358E-15, 50.50000000000000000, 32.49999999999999289 ) ) ;
#1676=CARTESIAN_POINT ( 'NONE',  ( -1.053607264507113999E-13, 63.00000000546238255, 32.50000000000000711 ) ) ;
#1678=CARTESIAN_POINT ( 'NONE',  ( 10.04305231718579705, 41.10000000546237686, 30.90933677959248982 ) ) ;
#1681=CARTESIAN_POINT ( 'NONE',  ( -10.04305231718579172, 60.10000000546239818, -30.90933677959248982 ) ) ;
#1682=CARTESIAN_POINT ( 'NONE',  ( 27.16883889988624290, 29.92500000273118488, 19.73931689729373673 ) ) ;
#1684=AXIS2_PLACEMENT_3D ( 'NONE', #15585, #25863, #20563 ) ;
#1686=VERTEX_POINT ( 'NONE', #26487 ) ;
#1694=EDGE_CURVE ( 'NONE', #7536, #19359, #32051, .T. ) ;
#1696=CARTESIAN_POINT ( 'NONE',  ( -26.29305231718578995, 46.19999999999998863, 19.10302069950538595 ) ) ;
#1697=CARTESIAN_POINT ( 'NONE',  ( 20.75514604977248467, 38.67500000273117422, -28.56700777964554305 ) ) ;
#1698=CARTESIAN_POINT ( 'NONE',  ( -20.08610463437157989, 42.20000000546239249, -27.64615127144129758 ) ) ;
#1700=CARTESIAN_POINT ( 'NONE',  ( 33.58253175000000823, 30.02500000273118985, 10.91162601494192863 ) ) ;
#1701=CARTESIAN_POINT ( 'NONE',  ( -33.58253175000000113, 53.37500000273118417, 0.000000000000000000 ) ) ;
#1703=CARTESIAN_POINT ( 'NONE',  ( 32.50000000000000000, 31.00000000000000000, -3.980102097228898626E-15 ) ) ;
#1705=CARTESIAN_POINT ( 'NONE',  ( -10.37757302488623701, 77.52500000273118985, 31.93888565452638417 ) ) ;
#1708=CARTESIAN_POINT ( 'NONE',  ( -32.50000000000000000, 37.89999999999999858, -10.55989012756945300 ) ) ;
#1709=CARTESIAN_POINT ( 'NONE',  ( -20.75514604977248823, 67.07500000273118701, -28.56700777964554305 ) ) ;
#1711=ORIENTED_EDGE ( 'NONE', *, *, #805, .F. ) ;
#1712=CARTESIAN_POINT ( 'NONE',  ( -33.58253175000000113, 19.12500000273118062, 0.000000000000000000 ) ) ;
#1713=CARTESIAN_POINT ( 'NONE',  ( 19.82091636218621034, 11.54999999453762349, 14.40073868116559730 ) ) ;
#1715=CARTESIAN_POINT ( 'NONE',  ( 0.000000000000000000, 80.00000000000001421, -32.50000000000000000 ) ) ;
#1725=CARTESIAN_POINT ( 'NONE',  ( 6.277390505771533514E-15, 77.00000000546235412, 34.17252228774368916 ) ) ;
#1730=CARTESIAN_POINT ( 'NONE',  ( 20.75514604977249178, 72.07500000273120122, 28.56700777964553950 ) ) ;
#1732=VERTEX_POINT ( 'NONE', #14281 ) ;
#1734=CARTESIAN_POINT ( 'NONE',  ( 20.08610463437157279, 65.80000000546237970, -27.64615127144129758 ) ) ;
#1735=ORIENTED_EDGE ( 'NONE', *, *, #7267, .T. ) ;
#1737=CARTESIAN_POINT ( 'NONE',  ( -27.16883889988623935, 47.32500000273117990, 19.73931689729374739 ) ) ;
#1738=CARTESIAN_POINT ( 'NONE',  ( 5.779280353836490358E-15, 55.00000000546238965, 32.49999999999999289 ) ) ;
#1739=CARTESIAN_POINT ( 'NONE',  ( -10.04305231718579172, 6.100000005462375086, -30.90933677959248982 ) ) ;
#1742=CARTESIAN_POINT ( 'NONE',  ( -20.08610463437156923, 56.29999999999999716, 27.64615127144130113 ) ) ;
#1743=CARTESIAN_POINT ( 'NONE',  ( 3.880418787951150694, 2.448745718453165132, -24.49999999999999645 ) ) ;
#1744=CARTESIAN_POINT ( 'NONE',  ( -27.16883889988624290, 19.17500000273120264, -19.73931689729374028 ) ) ;
#1745=CARTESIAN_POINT ( 'NONE',  ( 3.880418787951141812, 0.4487457184531665200, -24.50000000000000000 ) ) ;
#1747=CARTESIAN_POINT ( 'NONE',  ( 13.91746824999999887, 71.87500000273119838, -1.704398294459741270E-15 ) ) ;
#1758=CARTESIAN_POINT ( 'NONE',  ( 33.58253175000000113, 4.375000002731193938, -4.112674001490185761E-15 ) ) ;
#1762=CARTESIAN_POINT ( 'NONE',  ( 10.04305231718579705, 68.59999999999999432, 30.90933677959248982 ) ) ;
#1764=CARTESIAN_POINT ( 'NONE',  ( 20.75514604977249178, 45.82500000273118701, 28.56700777964553950 ) ) ;
#1769=PLANE ( 'NONE',  #26702 ) ;
#1771=CARTESIAN_POINT ( 'NONE',  ( -4.523095164977116484E-15, 10.12499999726881938, 24.62258325217400312 ) ) ;
#1773=ORIENTED_EDGE ( 'NONE', *, *, #8175, .T. ) ;
#1775=CIRCLE ( 'NONE', #13857, 26.50000000000000355 ) ;
#1777=( BOUNDED_CURVE ( )  B_SPLINE_CURVE ( 2, ( #17992, #22606, #25698, #33235, #17472, #20741, #4929, #9734, #12829, #31011, #15410, #23301, #7157 ),
 .UNSPECIFIED., .F., .T. ) 
 B_SPLINE_CURVE_WITH_KNOTS ( ( 3, 2, 2, 2, 2, 2, 3 ),
 ( 0.5833333333333333703, 0.5846153846153846478, 0.5871794871794872028, 0.5897435897435897578, 0.5923076923076923128, 0.5948717948717948678, 0.5961538461538461453 ),
 .UNSPECIFIED. ) 
 CURVE ( )  GEOMETRIC_REPRESENTATION_ITEM ( )  RATIONAL_B_SPLINE_CURVE ( ( 0.9755282581475768211, 0.9755282581475768211, 1.000000000000000000, 0.9510565162951535312, 1.000000000000000000, 0.9510565162951535312, 1.000000000000000000, 0.9510565162951535312, 1.000000000000000000, 0.9510565162951535312, 1.000000000000000000, 0.9755282581475768211, 0.9755282581475768211 ) ) 
 REPRESENTATION_ITEM ( '' )  );
#1778=ORIENTED_EDGE ( 'NONE', *, *, #3857, .T. ) ;
#1779=CARTESIAN_POINT ( 'NONE',  ( 5.147494310547408247, 69.05125428700922896, 32.50000000000000711 ) ) ;
#1780=CARTESIAN_POINT ( 'NONE',  ( 33.58253175000000823, 66.02500000273118985, 10.91162601494192863 ) ) ;
#1783=CARTESIAN_POINT ( 'NONE',  ( 19.82091636218621389, 10.19999999999998685, -14.40073868116559197 ) ) ;
#1784=CARTESIAN_POINT ( 'NONE',  ( 6.486482029760649416E-15, 1.875000002731177728, 35.31076352940723240 ) ) ;
#1785=CARTESIAN_POINT ( 'NONE',  ( 6.486482029760649416E-15, 7.625000002731170845, 35.31076352940723240 ) ) ;
#1788=CARTESIAN_POINT ( 'NONE',  ( 32.50000000000000000, 37.09999999999999432, -10.55989012756945833 ) ) ;
#1790=CARTESIAN_POINT ( 'NONE',  ( 5.779280353836490358E-15, 19.00000000546237544, 32.49999999999999289 ) ) ;
#1791=EDGE_CURVE ( 'NONE', #438, #17032, #10195, .T. ) ;
#1794=CARTESIAN_POINT ( 'NONE',  ( -9.270509831248425314, 75.95000000546237118, -12.75976212528059861 ) ) ;
#1796=CARTESIAN_POINT ( 'NONE',  ( -20.75514604977248112, 37.42500000273118843, 28.56700777964554661 ) ) ;
#1800=CARTESIAN_POINT ( 'NONE',  ( 33.58253175000000113, 22.37500000273118417, -4.112674001490185761E-15 ) ) ;
#1801=CARTESIAN_POINT ( 'NONE',  ( -5.147494310547430452, 12.05125428700922718, -32.49999999999999289 ) ) ;
#1802=AXIS2_PLACEMENT_3D ( 'NONE', #18407, #5351, #3448 ) ;
#1803=EDGE_CURVE ( 'NONE', #29733, #5805, #14784, .T. ) ;
#1804=CARTESIAN_POINT ( 'NONE',  ( -26.29305231718579350, 17.79999999999998295, -19.10302069950537884 ) ) ;
#1805=CARTESIAN_POINT ( 'NONE',  ( 20.08610463437157279, 79.29999999999999716, -27.64615127144129758 ) ) ;
#1807=CARTESIAN_POINT ( 'NONE',  ( -7.236395654485763274, 12.02499999726880375, 22.27133577429736633 ) ) ;
#1812=CARTESIAN_POINT ( 'NONE',  ( 6.486482029760648627E-15, 13.62500000273118417, 35.31076352940722529 ) ) ;
#1813=CARTESIAN_POINT ( 'NONE',  ( -14.47279130897151589, 11.82499999726882578, -19.92008829642072598 ) ) ;
#1818=ORIENTED_EDGE ( 'NONE', *, *, #11970, .T. ) ;
#1821=CARTESIAN_POINT ( 'NONE',  ( -1.778240108872766143E-15, 7.500000000000001776, -32.49999999999999289 ) ) ;
#1823=CARTESIAN_POINT ( 'NONE',  ( 18.94512977948576093, 1.324999997268816454, -13.76444248337722875 ) ) ;
#1825=CARTESIAN_POINT ( 'NONE',  ( 14.47279130897151589, 12.32499999726880802, 19.92008829642072953 ) ) ;
#1826=CARTESIAN_POINT ( 'NONE',  ( -27.16883889988623935, 19.57500000273118701, 19.73931689729374739 ) ) ;
#1827=CARTESIAN_POINT ( 'NONE',  ( 32.50000000000000711, 25.40000000546236691, 10.55989012756945122 ) ) ;
#1828=CARTESIAN_POINT ( 'NONE',  ( 32.50000000000000000, 65.00000000000000000, -3.980102097228898626E-15 ) ) ;
#1829=DIRECTION ( 'NONE',  ( -0.000000000000000000, -1.000000000000000000, -0.000000000000000000 ) ) ;
#1832=CARTESIAN_POINT ( 'NONE',  ( -33.58253175000000113, 37.47500000273118559, 10.91162601494193929 ) ) ;
#1833=CARTESIAN_POINT ( 'NONE',  ( 10.04305231718579705, 43.10000000546237686, 30.90933677959248982 ) ) ;
#1836=CARTESIAN_POINT ( 'NONE',  ( 23.41746825000000243, 15.22499999726880482, -7.608796670333727974 ) ) ;
#1837=CARTESIAN_POINT ( 'NONE',  ( 32.50000000000000711, 8.900000000000011013, 10.55989012756945122 ) ) ;
#1838=CARTESIAN_POINT ( 'NONE',  ( 26.29305231718579350, 9.300000005462383257, 19.10302069950537529 ) ) ;
#1840=CARTESIAN_POINT ( 'NONE',  ( 10.37757302488624056, 54.52500000273119696, -31.93888565452638417 ) ) ;
#1842=CARTESIAN_POINT ( 'NONE',  ( -2.162160676586882350E-15, 40.87500000273119838, -35.31076352940722529 ) ) ;
#1843=( BOUNDED_CURVE ( )  B_SPLINE_CURVE ( 2, ( #32968, #22353, #6566, #30573, #9293, #22693, #7070, #2095, #17554, #19778, #25443, #1918, #12395 ),
 .UNSPECIFIED., .F., .F. ) 
 B_SPLINE_CURVE_WITH_KNOTS ( ( 3, 2, 2, 2, 2, 2, 3 ),
 ( 0.3500000000000000333, 0.3599999999999999867, 0.3800000000000000044, 0.4000000000000000222, 0.4199999999999999845, 0.4400000000000000022, 0.4500000000000000111 ),
 .UNSPECIFIED. ) 
 CURVE ( )  GEOMETRIC_REPRESENTATION_ITEM ( )  RATIONAL_B_SPLINE_CURVE ( ( 0.9755282581475768211, 0.9755282581475768211, 1.000000000000000000, 0.9510565162951535312, 1.000000000000000000, 0.9510565162951535312, 1.000000000000000000, 0.9510565162951535312, 1.000000000000000000, 0.9510565162951535312, 1.000000000000000000, 0.9755282581475768211, 0.9755282581475768211 ) ) 
 REPRESENTATION_ITEM ( '' )  );
#1845=CARTESIAN_POINT ( 'NONE',  ( -5.147494310547430452, 49.55125428154685352, -32.49999999999999289 ) ) ;
#1847=EDGE_CURVE ( 'NONE', #3734, #17459, #13698, .T. ) ;
#1849=CARTESIAN_POINT ( 'NONE',  ( -5.147494310547430452, 41.55125428154684641, -32.49999999999999289 ) ) ;
#1851=FACE_OUTER_BOUND ( 'NONE', #29137, .T. ) ;
#1855=CARTESIAN_POINT ( 'NONE',  ( -5.147494310547427787, 78.05125428700921475, -32.49999999999999289 ) ) ;
#1858=CARTESIAN_POINT ( 'NONE',  ( 5.779280353836490358E-15, 34.49999999999998579, 32.49999999999999289 ) ) ;
#1859=CARTESIAN_POINT ( 'NONE',  ( -33.58253175000000113, 31.22500000273118204, 10.91162601494193929 ) ) ;
#1860=CARTESIAN_POINT ( 'NONE',  ( -10.37757302488624411, 64.97500000273120691, -31.93888565452638417 ) ) ;
#1865=VERTEX_POINT ( 'NONE', #24906 ) ;
#1871=CARTESIAN_POINT ( 'NONE',  ( -33.58253175000000113, 41.27500000273117564, -10.91162601494193218 ) ) ;
#1872=CARTESIAN_POINT ( 'NONE',  ( 26.29305231718579350, 43.30000000546238681, 19.10302069950537529 ) ) ;
#1874=CARTESIAN_POINT ( 'NONE',  ( -20.75514604977248112, 29.42500000273118133, 28.56700777964554661 ) ) ;
#1876=CARTESIAN_POINT ( 'NONE',  ( -20.75514604977248112, 55.67500000273118843, 28.56700777964554661 ) ) ;
#1879=CARTESIAN_POINT ( 'NONE',  ( -10.04305231718579172, 31.59999999999999076, -30.90933677959248982 ) ) ;
#1881=CARTESIAN_POINT ( 'NONE',  ( 10.37757302488624056, 76.52500000273118985, -31.93888565452638417 ) ) ;
#1883=CARTESIAN_POINT ( 'NONE',  ( 5.779280353836490358E-15, 38.50000000000000000, 32.49999999999999289 ) ) ;
#1884=CARTESIAN_POINT ( 'NONE',  ( 33.58253175000000113, 68.37500000273119838, -4.112674001490185761E-15 ) ) ;
#1887=CARTESIAN_POINT ( 'NONE',  ( 27.16883889988624290, 19.92500000273117422, 19.73931689729373673 ) ) ;
#1889=CARTESIAN_POINT ( 'NONE',  ( 15.14183272437241889, 11.44999999453763095, 20.84094480462498211 ) ) ;
#1891=EDGE_CURVE ( 'NONE', #6637, #30070, #484, .T. ) ;
#1903=CARTESIAN_POINT ( 'NONE',  ( 7.236395654485760609, 1.524999997268822183, -22.27133577429736633 ) ) ;
#1904=CARTESIAN_POINT ( 'NONE',  ( -20.08610463437156923, 76.80000000546239391, 27.64615127144130113 ) ) ;
#1905=CARTESIAN_POINT ( 'NONE',  ( 0.000000000000000000, 70.00000000000000000, 0.000000000000000000 ) ) ;
#1909=CARTESIAN_POINT ( 'NONE',  ( -33.58253175000000113, 75.37500000273116996, 0.000000000000000000 ) ) ;
#1912=CARTESIAN_POINT ( 'NONE',  ( -20.08610463437157989, 66.20000000546238539, -27.64615127144129758 ) ) ;
#1913=EDGE_LOOP ( 'NONE', ( #4571, #8333, #33317, #766, #26937, #32376, #8454, #22179 ) ) ;
#1915=CARTESIAN_POINT ( 'NONE',  ( -10.37757302488624411, 48.72500000273119269, -31.93888565452638417 ) ) ;
#1916=CARTESIAN_POINT ( 'NONE',  ( -23.41746825000000598, 17.72499999726881725, 7.608796670333726198 ) ) ;
#1917=CARTESIAN_POINT ( 'NONE',  ( -10.04305231718578462, 6.900000005462370467, 30.90933677959249337 ) ) ;
#1918=CARTESIAN_POINT ( 'NONE',  ( -2.375766604868045029, 77.55125428154684641, -14.99999999999999822 ) ) ;
#1921=CARTESIAN_POINT ( 'NONE',  ( 10.04305231718579705, 52.60000000000000853, 30.90933677959248982 ) ) ;
#1922=CARTESIAN_POINT ( 'NONE',  ( 24.50000000000000000, 2.099999999999991651, -7.960532557706203605 ) ) ;
#1923=CARTESIAN_POINT ( 'NONE',  ( -2.162160676586881955E-15, 16.87500000273120193, -35.31076352940723240 ) ) ;
#1924=DIRECTION ( 'NONE',  ( -0.000000000000000000, -1.000000000000000000, -0.000000000000000000 ) ) ;
#1926=CARTESIAN_POINT ( 'NONE',  ( -8.601468415847515203, 71.17500000273115290, 11.83890561707634959 ) ) ;
#1938=CARTESIAN_POINT ( 'NONE',  ( 27.16883889988623935, 4.575000002731199444, -19.73931689729374384 ) ) ;
#1940=EDGE_CURVE ( 'NONE', #28718, #20887, #4791, .T. ) ;
#1944=CARTESIAN_POINT ( 'NONE',  ( 32.50000000000000000, 69.00000000000000000, -3.980102097228898626E-15 ) ) ;
#1946=CARTESIAN_POINT ( 'NONE',  ( -2.162160676586882350E-15, 44.62500000273119838, -35.31076352940722529 ) ) ;
#1948=CARTESIAN_POINT ( 'NONE',  ( 10.04305231718579705, 21.10000000546238752, 30.90933677959248982 ) ) ;
#1953=CARTESIAN_POINT ( 'NONE',  ( 5.147494310547434893, 42.55125428154684641, 32.49999999999999289 ) ) ;
#1954=CARTESIAN_POINT ( 'NONE',  ( 1.507698388325705758E-15, 13.12499999726881228, -24.62258325217400312 ) ) ;
#1956=CARTESIAN_POINT ( 'NONE',  ( -20.75514604977248112, 73.67500000273120975, 28.56700777964554661 ) ) ;
#1960=EDGE_LOOP ( 'NONE', ( #18655, #11215, #15221, #19732 ) ) ;
#1963=CARTESIAN_POINT ( 'NONE',  ( 20.75514604977249178, 65.82500000273115859, 28.56700777964553950 ) ) ;
#1965=CARTESIAN_POINT ( 'NONE',  ( -7.570916362186215665, 9.399999999999991473, 23.30088464923126423 ) ) ;
#1966=CARTESIAN_POINT ( 'NONE',  ( 14.47279130897151767, 4.824999997268814234, 19.92008829642072953 ) ) ;
#1967=CARTESIAN_POINT ( 'NONE',  ( 33.58253175000000113, 10.22500000273117671, -10.91162601494193751 ) ) ;
#1968=CARTESIAN_POINT ( 'NONE',  ( -7.570916362186215665, 7.149999994537637349, 23.30088464923126423 ) ) ;
#1970=CARTESIAN_POINT ( 'NONE',  ( -9.270509831248425314, 75.69999999999998863, -12.75976212528059861 ) ) ;
#1972=CARTESIAN_POINT ( 'NONE',  ( -10.04305231718578462, 70.40000000000001990, 30.90933677959249337 ) ) ;
#1975=CARTESIAN_POINT ( 'NONE',  ( 9.270509831248425314, 74.95000000546237118, 12.75976212528059683 ) ) ;
#1977=CARTESIAN_POINT ( 'NONE',  ( -27.16883889988623935, 29.32500000273119412, 19.73931689729374739 ) ) ;
#1980=CARTESIAN_POINT ( 'NONE',  ( -10.37757302488624411, 18.97500000273119625, -31.93888565452638417 ) ) ;
#1982=CARTESIAN_POINT ( 'NONE',  ( -24.50000000000000000, 14.74999999453763166, -3.000384657911015469E-15 ) ) ;
#1983=CARTESIAN_POINT ( 'NONE',  ( 32.50000000000000000, 33.00000000000000000, -3.980102097228898626E-15 ) ) ;
#1985=CARTESIAN_POINT ( 'NONE',  ( 23.41746824999999887, 16.62499999726882294, 0.000000000000000000 ) ) ;
#1986=CARTESIAN_POINT ( 'NONE',  ( 27.16883889988624290, 63.92500000273118843, 19.73931689729373673 ) ) ;
#1990=CARTESIAN_POINT ( 'NONE',  ( -2.162160676586882350E-15, 8.625000002731168181, -35.31076352940722529 ) ) ;
#1991=CARTESIAN_POINT ( 'NONE',  ( -4.523095164977116484E-15, 12.62499999726879985, 24.62258325217400312 ) ) ;
#1999=DIRECTION ( 'NONE',  ( -0.000000000000000000, -1.000000000000000000, -0.000000000000000000 ) ) ;
#2001=CARTESIAN_POINT ( 'NONE',  ( 23.41746825000000243, 7.024999997268802865, 7.608796670333735079 ) ) ;
#2002=CARTESIAN_POINT ( 'NONE',  ( 7.236395654485755280, 14.22499999726881192, 22.27133577429736988 ) ) ;
#2003=CARTESIAN_POINT ( 'NONE',  ( 27.16883889988623935, 14.57500000273120833, -19.73931689729374384 ) ) ;
#2004=CARTESIAN_POINT ( 'NONE',  ( -32.50000000000000000, 24.60000000546236620, 10.55989012756946366 ) ) ;
#2005=CARTESIAN_POINT ( 'NONE',  ( 32.50000000000000711, 62.89999999999999147, 10.55989012756945122 ) ) ;
#2006=CARTESIAN_POINT ( 'NONE',  ( -8.891200544363830713E-16, 77.75000000546236834, -15.00000000000000000 ) ) ;
#2009=CARTESIAN_POINT ( 'NONE',  ( 33.58253175000000823, 32.27500000273117564, 10.91162601494192863 ) ) ;
#2010=CARTESIAN_POINT ( 'NONE',  ( -4.300734207923759378, 80.97500000273119269, -13.23629886949340495 ) ) ;
#2014=CARTESIAN_POINT ( 'NONE',  ( -14.47279130897152122, 18.42499999726882365, 19.92008829642072243 ) ) ;
#2015=CARTESIAN_POINT ( 'NONE',  ( -32.50000000000000000, 10.00000000000000888, 0.000000000000000000 ) ) ;
#2016=CYLINDRICAL_SURFACE ( 'NONE', #30194, 32.50000000000000000 ) ;
#2018=CARTESIAN_POINT ( 'NONE',  ( -33.58253175000000113, 51.22500000273119269, 10.91162601494193929 ) ) ;
#2020=CARTESIAN_POINT ( 'NONE',  ( 27.16883889988624290, 40.17500000273119554, 19.73931689729373673 ) ) ;
#2023=CARTESIAN_POINT ( 'NONE',  ( 19.82091636218621389, 10.19999999999998685, -14.40073868116559197 ) ) ;
#2024=CARTESIAN_POINT ( 'NONE',  ( -32.50000000000000000, 49.99999999999998579, 0.000000000000000000 ) ) ;
#2029=CARTESIAN_POINT ( 'NONE',  ( -32.50000000000000000, 62.50000000546238255, 0.000000000000000000 ) ) ;
#2035=CARTESIAN_POINT ( 'NONE',  ( 10.37757302488624056, 32.52500000273117564, -31.93888565452638417 ) ) ;
#2036=CARTESIAN_POINT ( 'NONE',  ( -20.75514604977248112, 65.67500000273118133, 28.56700777964554661 ) ) ;
#2042=ORIENTED_EDGE ( 'NONE', *, *, #20115, .T. ) ;
#2048=CARTESIAN_POINT ( 'NONE',  ( -2.162160676586881955E-15, 40.87500000273119838, -35.31076352940723240 ) ) ;
#2049=CARTESIAN_POINT ( 'NONE',  ( 10.04305231718579705, 41.10000000546237686, 30.90933677959248982 ) ) ;
#2051=CARTESIAN_POINT ( 'NONE',  ( -27.16883889988624290, 22.92500000273117777, -19.73931689729374028 ) ) ;
#2053=CARTESIAN_POINT ( 'NONE',  ( 33.58253175000000113, 52.47500000273117138, -10.91162601494193751 ) ) ;
#2055=CARTESIAN_POINT ( 'NONE',  ( 20.08610463437157279, 29.30000000000000782, -27.64615127144129758 ) ) ;
#2057=CARTESIAN_POINT ( 'NONE',  ( -27.16883889988624290, 76.92500000273119554, -19.73931689729374028 ) ) ;
#2058=CARTESIAN_POINT ( 'NONE',  ( -10.04305231718579172, 70.10000000546237686, -30.90933677959248982 ) ) ;
#2059=CARTESIAN_POINT ( 'NONE',  ( -10.04305231718578462, 20.90000000546238113, 30.90933677959249337 ) ) ;
#2060=CARTESIAN_POINT ( 'NONE',  ( -33.58253175000000113, 59.47500000273119269, 10.91162601494193929 ) ) ;
#2063=CARTESIAN_POINT ( 'NONE',  ( -10.37757302488624411, 18.72500000273119625, -31.93888565452638417 ) ) ;
#2064=CARTESIAN_POINT ( 'NONE',  ( 7.570916362186213000, 10.14999999453763913, -23.30088464923126423 ) ) ;
#2066=CARTESIAN_POINT ( 'NONE',  ( 32.50000000000000000, 46.99999999999998579, -3.980102097228898626E-15 ) ) ;
#2078=CARTESIAN_POINT ( 'NONE',  ( -26.29305231718578995, 54.19999999999999574, 19.10302069950538595 ) ) ;
#2079=CARTESIAN_POINT ( 'NONE',  ( 20.08610463437157279, 75.80000000546237970, -27.64615127144129758 ) ) ;
#2084=CARTESIAN_POINT ( 'NONE',  ( -20.75514604977248112, 75.67500000273118133, 28.56700777964554661 ) ) ;
#2087=CARTESIAN_POINT ( 'NONE',  ( 32.50000000000000711, 61.40000000546237402, 10.55989012756945122 ) ) ;
#2089=ORIENTED_EDGE ( 'NONE', *, *, #29548, .T. ) ;
#2091=CARTESIAN_POINT ( 'NONE',  ( -27.16883889988624290, 42.92500000273119554, -19.73931689729374028 ) ) ;
#2092=CARTESIAN_POINT ( 'NONE',  ( 3.980102097228898626E-15, 80.00000000000001421, 32.50000000000000000 ) ) ;
#2094=CARTESIAN_POINT ( 'NONE',  ( 32.50000000000000000, 7.600000005462379526, -10.55989012756945833 ) ) ;
#2095=CARTESIAN_POINT ( 'NONE',  ( -15.00000000000000000, 77.90000000000000568, -4.873795443493594171 ) ) ;
#2097=CARTESIAN_POINT ( 'NONE',  ( -26.29305231718579350, 47.80000000000001137, -19.10302069950537884 ) ) ;
#2099=CARTESIAN_POINT ( 'NONE',  ( -33.58253175000000113, 15.27500000273118985, -10.91162601494193218 ) ) ;
#2100=CARTESIAN_POINT ( 'NONE',  ( -20.08610463437157989, 24.20000000546238184, -27.64615127144129758 ) ) ;
#2102=CARTESIAN_POINT ( 'NONE',  ( 11.25946833292375793, 76.17500000273119554, 8.180482586598731842 ) ) ;
#2103=CARTESIAN_POINT ( 'NONE',  ( -20.75514604977248823, 79.07500000273121543, -28.56700777964554305 ) ) ;
#2117=CARTESIAN_POINT ( 'NONE',  ( 11.25946833292375793, 72.17500000273119554, 8.180482586598731842 ) ) ;
#2119=CARTESIAN_POINT ( 'NONE',  ( 10.37757302488624056, 46.52500000273118985, -31.93888565452638417 ) ) ;
#2121=VERTEX_POINT ( 'NONE', #13415 ) ;
#2123=CARTESIAN_POINT ( 'NONE',  ( -26.29305231718579350, 4.300000005462378816, -19.10302069950537884 ) ) ;
#2125=CARTESIAN_POINT ( 'NONE',  ( 20.75514604977248467, 76.67500000273116711, -28.56700777964554305 ) ) ;
#2126=VERTEX_POINT ( 'NONE', #21645 ) ;
#2129=EDGE_CURVE ( 'NONE', #12058, #1865, #8800, .T. ) ;
#2130=ORIENTED_EDGE ( 'NONE', *, *, #28233, .F. ) ;
#2131=CARTESIAN_POINT ( 'NONE',  ( -10.04305231718579172, 14.10000000546238219, -30.90933677959248982 ) ) ;
#2132=CARTESIAN_POINT ( 'NONE',  ( 20.75514604977249178, 69.82500000273118701, 28.56700777964553950 ) ) ;
#2134=CARTESIAN_POINT ( 'NONE',  ( -19.82091636218621034, 14.80000000000000782, -14.40073868116559552 ) ) ;
#2136=CARTESIAN_POINT ( 'NONE',  ( 27.16883889988623935, 10.32500000273117635, -19.73931689729374384 ) ) ;
#2137=CARTESIAN_POINT ( 'NONE',  ( 20.08610463437158344, 28.69999999999999574, 27.64615127144129403 ) ) ;
#2139=CARTESIAN_POINT ( 'NONE',  ( 15.00000000000000000, 73.00000000000001421, -1.836970198721029589E-15 ) ) ;
#2144=CARTESIAN_POINT ( 'NONE',  ( 12.13525491562420910, 73.45000000546237118, -8.816778784387098611 ) ) ;
#2146=CARTESIAN_POINT ( 'NONE',  ( 27.16883889988623935, 28.32500000273119412, -19.73931689729374384 ) ) ;
#2149=CARTESIAN_POINT ( 'NONE',  ( -2.162160676586882350E-15, 20.87500000273119127, -35.31076352940722529 ) ) ;
#2150=CARTESIAN_POINT ( 'NONE',  ( -10.04305231718578462, 12.90000000546237580, 30.90933677959249337 ) ) ;
#2151=CARTESIAN_POINT ( 'NONE',  ( -20.75514604977248823, 74.82500000273115859, -28.56700777964554305 ) ) ;
#2152=CARTESIAN_POINT ( 'NONE',  ( 19.82091636218621389, 8.200000000000013500, -14.40073868116559197 ) ) ;
#2155=CARTESIAN_POINT ( 'NONE',  ( 14.47279130897151767, 14.32499999726880624, 19.92008829642072953 ) ) ;
#2156=CARTESIAN_POINT ( 'NONE',  ( 27.16883889988623935, 66.32500000273117280, -19.73931689729374384 ) ) ;
#2159=CARTESIAN_POINT ( 'NONE',  ( -33.58253175000000113, 9.125000002731198379, 0.000000000000000000 ) ) ;
#2160=CARTESIAN_POINT ( 'NONE',  ( -23.41746825000000243, 14.02499999726881263, -7.608796670333730638 ) ) ;
#2162=ORIENTED_EDGE ( 'NONE', *, *, #22859, .F. ) ;
#2164=ORIENTED_EDGE ( 'NONE', *, *, #33212, .F. ) ;
#2170=CARTESIAN_POINT ( 'NONE',  ( -23.41746825000000243, 6.024999997268805529, -7.608796670333730638 ) ) ;
#2171=CARTESIAN_POINT ( 'NONE',  ( -18.94512977948575738, 9.424999997268812990, -13.76444248337723231 ) ) ;
#2172=CARTESIAN_POINT ( 'NONE',  ( -33.58253175000000113, 13.37500000273117351, 0.000000000000000000 ) ) ;
#2173=CARTESIAN_POINT ( 'NONE',  ( 26.29305231718578995, 15.70000000546237295, -19.10302069950538240 ) ) ;
#2174=CARTESIAN_POINT ( 'NONE',  ( 26.29305231718578995, 63.20000000000000284, -19.10302069950538240 ) ) ;
#2175=CARTESIAN_POINT ( 'NONE',  ( 5.779280353836490358E-15, 6.500000000000002665, 32.49999999999999289 ) ) ;
#2176=CARTESIAN_POINT ( 'NONE',  ( 32.50000000000000000, 73.50000000546236834, -3.980102097228898626E-15 ) ) ;
#2178=CARTESIAN_POINT ( 'NONE',  ( 10.37757302488624056, 30.77500000273120051, -31.93888565452638417 ) ) ;
#2179=CARTESIAN_POINT ( 'NONE',  ( -11.25946833292375793, 79.57500000273121543, 8.180482586598737171 ) ) ;
#2182=CARTESIAN_POINT ( 'NONE',  ( -7.236395654485757944, 13.72499999726881015, -22.27133577429736988 ) ) ;
#2183=CARTESIAN_POINT ( 'NONE',  ( -26.29305231718579350, 9.800000000000002487, -19.10302069950537884 ) ) ;
#2186=CARTESIAN_POINT ( 'NONE',  ( -27.16883889988624290, 52.92500000273120264, -19.73931689729374028 ) ) ;
#2188=CARTESIAN_POINT ( 'NONE',  ( -20.75514604977248112, 41.67500000273117422, 28.56700777964554661 ) ) ;
#2191=CARTESIAN_POINT ( 'NONE',  ( -19.82091636218621034, 8.800000000000002487, -14.40073868116559552 ) ) ;
#2192=FACE_OUTER_BOUND ( 'NONE', #4061, .T. ) ;
#2195=CARTESIAN_POINT ( 'NONE',  ( 8.601468415847516980, 80.67500000273115290, -11.83890561707634603 ) ) ;
#2196=LINE ( 'NONE', #10278, #24858 ) ;
#2197=CARTESIAN_POINT ( 'NONE',  ( -4.934616302121927505E-14, 70.50000000000000000, 32.50000000000000000 ) ) ;
#2200=CARTESIAN_POINT ( 'NONE',  ( 26.29305231718578995, 11.19999999999998863, -19.10302069950538240 ) ) ;
#2201=CARTESIAN_POINT ( 'NONE',  ( 10.37757302488624056, 24.52500000273119696, -31.93888565452638417 ) ) ;
#2207=ORIENTED_EDGE ( 'NONE', *, *, #12302, .F. ) ;
#2212=CARTESIAN_POINT ( 'NONE',  ( 3.980102097228898626E-15, 80.00000000000001421, 32.50000000000000000 ) ) ;
#2213=CARTESIAN_POINT ( 'NONE',  ( 10.37757302488624767, 35.97500000273118559, 31.93888565452638417 ) ) ;
#2214=CARTESIAN_POINT ( 'NONE',  ( 10.04305231718578817, 41.90000000546237402, -30.90933677959249337 ) ) ;
#2217=CARTESIAN_POINT ( 'NONE',  ( -33.58253175000000113, 23.12500000273118417, 0.000000000000000000 ) ) ;
#2219=CARTESIAN_POINT ( 'NONE',  ( -20.75514604977248112, 49.67500000273118133, 28.56700777964554661 ) ) ;
#2223=CARTESIAN_POINT ( 'NONE',  ( -26.29305231718579350, 27.79999999999999005, -19.10302069950537884 ) ) ;
#2225=CARTESIAN_POINT ( 'NONE',  ( -2.162160676586881955E-15, 66.62500000273118417, -35.31076352940723240 ) ) ;
#2228=CARTESIAN_POINT ( 'NONE',  ( 6.486482029760648627E-15, 61.87500000273117706, 35.31076352940722529 ) ) ;
#2231=EDGE_CURVE ( 'NONE', #21272, #32007, #8416, .T. ) ;
#2233=CARTESIAN_POINT ( 'NONE',  ( -20.75514604977248823, 16.82500000273120122, -28.56700777964554305 ) ) ;
#2234=CARTESIAN_POINT ( 'NONE',  ( -19.82091636218621034, 10.54999999453762349, -14.40073868116559552 ) ) ;
#2238=LINE ( 'NONE', #20959, #2903 ) ;
#2239=DIRECTION ( 'NONE',  ( 0.000000000000000000, 1.000000000000000000, 0.000000000000000000 ) ) ;
#2241=ADVANCED_FACE ( 'NONE', ( #11007 ), #7919, .T. ) ;
#2246=CARTESIAN_POINT ( 'NONE',  ( 32.50000000000000000, 63.00000000000000000, -3.980102097228898626E-15 ) ) ;
#2249=CARTESIAN_POINT ( 'NONE',  ( 20.08610463437158344, 77.20000000546238539, 27.64615127144129403 ) ) ;
#2251=VECTOR ( 'NONE', #32207, 1000.000000000000000 ) ;
#2255=CARTESIAN_POINT ( 'NONE',  ( -27.16883889988623935, 73.57500000273120122, 19.73931689729374739 ) ) ;
#2259=CARTESIAN_POINT ( 'NONE',  ( -2.162160676586881955E-15, 54.87500000273119127, -35.31076352940723240 ) ) ;
#2260=CARTESIAN_POINT ( 'NONE',  ( 32.50000000000000711, 65.40000000546237402, 10.55989012756945122 ) ) ;
#2263=CARTESIAN_POINT ( 'NONE',  ( -10.37757302488623701, 43.52500000273118275, 31.93888565452638417 ) ) ;
#2264=CARTESIAN_POINT ( 'NONE',  ( -14.47279130897152122, 15.92499999726881121, 19.92008829642072243 ) ) ;
#2266=CARTESIAN_POINT ( 'NONE',  ( -33.58253175000000113, 69.37500000273119838, 0.000000000000000000 ) ) ;
#2267=CARTESIAN_POINT ( 'NONE',  ( -26.29305231718578995, 6.700000005462392494, 19.10302069950538595 ) ) ;
#2269=CARTESIAN_POINT ( 'NONE',  ( -1.778240108872766143E-15, 50.00000000546237544, -32.49999999999999289 ) ) ;
#2270=CARTESIAN_POINT ( 'NONE',  ( -20.08610463437157989, 49.70000000000000284, -27.64615127144129758 ) ) ;
#2272=CARTESIAN_POINT ( 'NONE',  ( -2.162160676586881955E-15, 12.87500000273117884, -35.31076352940723240 ) ) ;
#2273=CARTESIAN_POINT ( 'NONE',  ( -3.880418787951136483, 6.551254281546842861, -24.50000000000000000 ) ) ;
#2275=CARTESIAN_POINT ( 'NONE',  ( 11.25946833292375793, 80.17500000273119554, 8.180482586598731842 ) ) ;
#2276=CARTESIAN_POINT ( 'NONE',  ( -20.75514604977248112, 77.67500000273119554, 28.56700777964554661 ) ) ;
#2277=CARTESIAN_POINT ( 'NONE',  ( 5.779280353836490358E-15, 44.49999999999999289, 32.49999999999999289 ) ) ;
#2279=EDGE_LOOP ( 'NONE', ( #16616, #14323, #15089, #592 ) ) ;
#2292=CARTESIAN_POINT ( 'NONE',  ( -8.601468415847518756, 73.07500000273115859, -11.83890561707634603 ) ) ;
#2294=AXIS2_PLACEMENT_3D ( 'NONE', #9518, #16753, #24632 ) ;
#2295=CARTESIAN_POINT ( 'NONE',  ( 6.486482029760648627E-15, 47.62500000273118417, 35.31076352940722529 ) ) ;
#2302=CARTESIAN_POINT ( 'NONE',  ( 20.75514604977248467, 74.67500000273118133, -28.56700777964554305 ) ) ;
#2303=ORIENTED_EDGE ( 'NONE', *, *, #8928, .F. ) ;
#2306=ORIENTED_EDGE ( 'NONE', *, *, #4748, .F. ) ;
#2307=CARTESIAN_POINT ( 'NONE',  ( 32.50000000000000000, 29.60000000546238041, -10.55989012756945833 ) ) ;
#2308=CARTESIAN_POINT ( 'NONE',  ( 27.16883889988624290, 63.92500000273118843, 19.73931689729373673 ) ) ;
#2310=CARTESIAN_POINT ( 'NONE',  ( -15.14183272437242600, 17.30000000000000782, 20.84094480462497856 ) ) ;
#2311=CARTESIAN_POINT ( 'NONE',  ( 3.980102097228898626E-15, 80.00000000000001421, 32.50000000000000000 ) ) ;
#2312=CARTESIAN_POINT ( 'NONE',  ( 33.58253175000000113, 6.125000002731195714, -4.112674001490185761E-15 ) ) ;
#2315=CARTESIAN_POINT ( 'NONE',  ( -4.635254915624211769, 75.59999999999999432, -14.26584774442730286 ) ) ;
#2320=CARTESIAN_POINT ( 'NONE',  ( 12.13525491562420910, 71.45000000546237118, -8.816778784387098611 ) ) ;
#2322=CARTESIAN_POINT ( 'NONE',  ( 10.37757302488624767, 31.72500000273117848, 31.93888565452638417 ) ) ;
#2325=CARTESIAN_POINT ( 'NONE',  ( 33.58253175000000113, 24.37500000273118417, -4.112674001490185761E-15 ) ) ;
#2326=CARTESIAN_POINT ( 'NONE',  ( -32.50000000000000000, 64.00000000000000000, 0.000000000000000000 ) ) ;
#2327=CARTESIAN_POINT ( 'NONE',  ( -10.04305231718579172, 26.10000000546236620, -30.90933677959248982 ) ) ;
#2329=AXIS2_PLACEMENT_3D ( 'NONE', #5294, #29129, #33951 ) ;
#2330=CARTESIAN_POINT ( 'NONE',  ( 18.94512977948575738, 18.42499999726882010, 13.76444248337723408 ) ) ;
#2331=CARTESIAN_POINT ( 'NONE',  ( 10.37757302488624056, 66.52500000273120406, -31.93888565452638417 ) ) ;
#2332=EDGE_CURVE ( 'NONE', #6218, #23029, #17197, .T. ) ;
#2336=CARTESIAN_POINT ( 'NONE',  ( -10.37757302488623701, 5.525000002731205839, 31.93888565452638417 ) ) ;
#2337=CARTESIAN_POINT ( 'NONE',  ( 18.94512977948576093, 2.824999997268817786, -13.76444248337722875 ) ) ;
#2344=CARTESIAN_POINT ( 'NONE',  ( 24.50000000000000000, 19.74999999453763877, 0.000000000000000000 ) ) ;
#2346=CARTESIAN_POINT ( 'NONE',  ( -18.94512977948576093, 4.324999997268818674, 13.76444248337722698 ) ) ;
#2347=CARTESIAN_POINT ( 'NONE',  ( 7.236395654485760609, 15.02499999726880731, -22.27133577429736633 ) ) ;
#2348=CARTESIAN_POINT ( 'NONE',  ( 10.37757302488624056, 16.77500000273118985, -31.93888565452638417 ) ) ;
#2349=CARTESIAN_POINT ( 'NONE',  ( -10.04305231718579172, 20.10000000546238752, -30.90933677959248982 ) ) ;
#2350=AXIS2_PLACEMENT_3D ( 'NONE', #3763, #24691, #6833 ) ;
#2351=CARTESIAN_POINT ( 'NONE',  ( 10.04305231718579705, 66.59999999999999432, 30.90933677959248982 ) ) ;
#2353=CYLINDRICAL_SURFACE ( 'NONE', #25262, 32.50000000000000000 ) ;
#2359=CARTESIAN_POINT ( 'NONE',  ( 1.507698388325705758E-15, 17.62499999726881938, -24.62258325217400312 ) ) ;
#2360=CARTESIAN_POINT ( 'NONE',  ( -32.50000000000000000, 7.900000000000012790, -10.55989012756945478 ) ) ;
#2361=CARTESIAN_POINT ( 'NONE',  ( -2.375766604868045029, 73.55125428154683220, -14.99999999999999822 ) ) ;
#2363=( BOUNDED_CURVE ( )  B_SPLINE_CURVE ( 2, ( #13188, #18355, #10283, #28626, #33609, #31373, #18183, #21097, #18523, #26063, #20762, #7864, #15432 ),
 .UNSPECIFIED., .F., .T. ) 
 B_SPLINE_CURVE_WITH_KNOTS ( ( 3, 2, 2, 2, 2, 2, 3 ),
 ( 0.8611111111111111605, 0.8666666666666666963, 0.8777777777777777679, 0.8888888888888888395, 0.9000000000000000222, 0.9111111111111110938, 0.9166666666666666297 ),
 .UNSPECIFIED. ) 
 CURVE ( )  GEOMETRIC_REPRESENTATION_ITEM ( )  RATIONAL_B_SPLINE_CURVE ( ( 0.9755282581475768211, 0.9755282581475770431, 1.000000000000000000, 0.9510565162951535312, 1.000000000000000000, 0.9510565162951535312, 1.000000000000000000, 0.9510565162951535312, 1.000000000000000000, 0.9510565162951535312, 1.000000000000000000, 0.9755282581475770431, 0.9755282581475768211 ) ) 
 REPRESENTATION_ITEM ( '' )  );
#2364=CARTESIAN_POINT ( 'NONE',  ( -33.58253175000000113, 51.12500000273117706, 0.000000000000000000 ) ) ;
#2366=CARTESIAN_POINT ( 'NONE',  ( 33.58253175000000823, 38.27500000273119696, 10.91162601494192685 ) ) ;
#2370=CARTESIAN_POINT ( 'NONE',  ( 23.95873412499999944, 1.437499995903229744, 0.000000000000000000 ) ) ;
#2373=CARTESIAN_POINT ( 'NONE',  ( -32.50000000000000000, 78.50000000546236834, 0.000000000000000000 ) ) ;
#2374=DIRECTION ( 'NONE',  ( -0.000000000000000000, 1.000000000000000000, -0.000000000000000000 ) ) ;
#2375=CARTESIAN_POINT ( 'NONE',  ( 3.880418787951172011, 11.55125428154683576, 24.49999999999998579 ) ) ;
#2377=EDGE_CURVE ( 'NONE', #17974, #13948, #20725, .T. ) ;
#2381=CARTESIAN_POINT ( 'NONE',  ( 6.486482029760648627E-15, 27.62500000273118062, 35.31076352940722529 ) ) ;
#2384=VERTEX_POINT ( 'NONE', #3778 ) ;
#2393=DIRECTION ( 'NONE',  ( -0.000000000000000000, 1.000000000000000000, -0.000000000000000000 ) ) ;
#2394=CARTESIAN_POINT ( 'NONE',  ( -33.58253175000000113, 33.47500000273119269, 10.91162601494193929 ) ) ;
#2395=CARTESIAN_POINT ( 'NONE',  ( 32.50000000000000000, 37.50000000546238255, -3.980102097228898626E-15 ) ) ;
#2399=CARTESIAN_POINT ( 'NONE',  ( 10.37757302488624767, 23.72500000273119980, 31.93888565452638417 ) ) ;
#2400=CARTESIAN_POINT ( 'NONE',  ( 32.50000000000000000, 77.09999999999998010, -10.55989012756945833 ) ) ;
#2401=CARTESIAN_POINT ( 'NONE',  ( -2.162160676586881955E-15, 48.87500000273117706, -35.31076352940723240 ) ) ;
#2404=CARTESIAN_POINT ( 'NONE',  ( 26.29305231718578995, 27.20000000000000284, -19.10302069950538240 ) ) ;
#2406=CARTESIAN_POINT ( 'NONE',  ( -27.16883889988623935, 67.32500000273117280, 19.73931689729374739 ) ) ;
#2410=CARTESIAN_POINT ( 'NONE',  ( -10.37757302488623701, 61.77500000273117564, 31.93888565452638417 ) ) ;
#2412=CARTESIAN_POINT ( 'NONE',  ( 32.50000000000000711, 7.400000005462386454, 10.55989012756945122 ) ) ;
#2413=CARTESIAN_POINT ( 'NONE',  ( 10.37757302488624767, 13.72500000273119092, 31.93888565452638417 ) ) ;
#2415=CARTESIAN_POINT ( 'NONE',  ( 19.82091636218621389, 1.949999994537626735, -14.40073868116559197 ) ) ;
#2423=CARTESIAN_POINT ( 'NONE',  ( 5.147494310547481966, 61.44874571845315359, -32.49999999999998579 ) ) ;
#2425=CARTESIAN_POINT ( 'NONE',  ( 26.29305231718579350, 63.30000000546237260, 19.10302069950537529 ) ) ;
#2426=CARTESIAN_POINT ( 'NONE',  ( -20.08610463437157989, 78.20000000546235697, -27.64615127144129758 ) ) ;
#2431=CARTESIAN_POINT ( 'NONE',  ( 20.75514604977249178, 78.07500000273117280, 28.56700777964553950 ) ) ;
#2433=EDGE_CURVE ( 'NONE', #28550, #7938, #3992, .T. ) ;
#2436=CARTESIAN_POINT ( 'NONE',  ( -33.58253175000000113, 55.47500000273119980, 10.91162601494193929 ) ) ;
#2437=CARTESIAN_POINT ( 'NONE',  ( -32.50000000000000000, 56.60000000546236976, 10.55989012756946366 ) ) ;
#2439=CARTESIAN_POINT ( 'NONE',  ( 27.16883889988623935, 40.32500000273120122, -19.73931689729374384 ) ) ;
#2441=CARTESIAN_POINT ( 'NONE',  ( -33.58253175000000113, 67.27500000273117564, -10.91162601494193218 ) ) ;
#2442=CARTESIAN_POINT ( 'NONE',  ( 10.04305231718579705, 3.100000005462372421, 30.90933677959248982 ) ) ;
#2443=ADVANCED_FACE ( 'NONE', ( #22312 ), #9419, .T. ) ;
#2445=CARTESIAN_POINT ( 'NONE',  ( 0.000000000000000000, 80.00000000000001421, 0.000000000000000000 ) ) ;
#2446=CARTESIAN_POINT ( 'NONE',  ( -32.50000000000000000, 44.10000000000000142, 10.55989012756946366 ) ) ;
#2447=LINE ( 'NONE', #10176, #26928 ) ;
#2448=CARTESIAN_POINT ( 'NONE',  ( 10.37757302488624767, 13.97500000273119092, 31.93888565452638417 ) ) ;
#2449=CARTESIAN_POINT ( 'NONE',  ( -26.29305231718578995, 74.19999999999998863, 19.10302069950538595 ) ) ;
#2451=CARTESIAN_POINT ( 'NONE',  ( -13.91746824999999532, 77.27500000273117564, -4.522059556121115875 ) ) ;
#2452=CARTESIAN_POINT ( 'NONE',  ( 20.75514604977249178, 78.07500000273118701, 28.56700777964553950 ) ) ;
#2467=CYLINDRICAL_SURFACE ( 'NONE', #158, 32.50000000000000000 ) ;
#2468=CARTESIAN_POINT ( 'NONE',  ( 20.75514604977249178, 43.82500000273119412, 28.56700777964553950 ) ) ;
#2472=ORIENTED_EDGE ( 'NONE', *, *, #1363, .F. ) ;
#2476=CARTESIAN_POINT ( 'NONE',  ( -10.37757302488624411, 72.97500000273119269, -31.93888565452638417 ) ) ;
#2477=ORIENTED_EDGE ( 'NONE', *, *, #6511, .T. ) ;
#2483=CARTESIAN_POINT ( 'NONE',  ( 20.75514604977248467, 62.42500000273118133, -28.56700777964554305 ) ) ;
#2486=CARTESIAN_POINT ( 'NONE',  ( 7.236395654485755280, 2.724999997268801266, 22.27133577429736988 ) ) ;
#2487=CARTESIAN_POINT ( 'NONE',  ( -10.37757302488623701, 3.525000002731204507, 31.93888565452638417 ) ) ;
#2489=CARTESIAN_POINT ( 'NONE',  ( 33.58253175000000113, 78.37500000273116996, -4.112674001490185761E-15 ) ) ;
#2491=CARTESIAN_POINT ( 'NONE',  ( -10.04305231718579172, 69.59999999999999432, -30.90933677959248982 ) ) ;
#2495=CARTESIAN_POINT ( 'NONE',  ( -12.13525491562420910, 72.45000000546237118, 8.816778784387098611 ) ) ;
#2497=CARTESIAN_POINT ( 'NONE',  ( -2.162160676586881955E-15, 32.62500000273119838, -35.31076352940723240 ) ) ;
#2501=CARTESIAN_POINT ( 'NONE',  ( 20.75514604977248467, 22.67500000273119198, -28.56700777964554305 ) ) ;
#2502=CARTESIAN_POINT ( 'NONE',  ( -9.270509831248423538, 79.70000000000000284, -12.75976212528059861 ) ) ;
#2504=CARTESIAN_POINT ( 'NONE',  ( 27.16883889988624290, 75.92500000273119554, 19.73931689729373673 ) ) ;
#2506=CARTESIAN_POINT ( 'NONE',  ( -5.147494310547213736, 26.05125428700921475, -32.50000000000007105 ) ) ;
#2508=DIRECTION ( 'NONE',  ( 0.000000000000000000, 0.000000000000000000, -1.000000000000000000 ) ) ;
#2509=CARTESIAN_POINT ( 'NONE',  ( 20.75514604977248467, 62.42500000273118133, -28.56700777964554305 ) ) ;
#2512=CARTESIAN_POINT ( 'NONE',  ( 33.58253175000000113, 8.225000002731182036, -10.91162601494193574 ) ) ;
#2513=VECTOR ( 'NONE', #32270, 1000.000000000000000 ) ;
#2514=CARTESIAN_POINT ( 'NONE',  ( 1.507698388325705758E-15, 3.124999997268809615, -24.62258325217400312 ) ) ;
#2523=CARTESIAN_POINT ( 'NONE',  ( -1.778240108872766143E-15, 71.50000000000001421, -32.49999999999999289 ) ) ;
#2524=CARTESIAN_POINT ( 'NONE',  ( -23.41746824999999887, 2.124999997268811391, -2.867812753649727150E-15 ) ) ;
#2525=CARTESIAN_POINT ( 'NONE',  ( -7.570916362186210335, 0.5999999999999894307, -23.30088464923126779 ) ) ;
#2526=CARTESIAN_POINT ( 'NONE',  ( 33.58253175000000823, 18.27500000273118275, 10.91162601494192863 ) ) ;
#2527=EDGE_CURVE ( 'NONE', #22201, #20335, #24215, .T. ) ;
#2528=CARTESIAN_POINT ( 'NONE',  ( -10.04305231718579172, 67.59999999999999432, -30.90933677959248982 ) ) ;
#2530=CARTESIAN_POINT ( 'NONE',  ( -32.50000000000000000, 30.00000000000000000, 0.000000000000000000 ) ) ;
#2532=CARTESIAN_POINT ( 'NONE',  ( -8.601468415847515203, 73.67500000273120975, 11.83890561707634959 ) ) ;
#2535=EDGE_CURVE ( 'NONE', #2384, #4493, #31224, .T. ) ;
#2537=CARTESIAN_POINT ( 'NONE',  ( -14.47279130897151589, 17.82499999726881157, -19.92008829642072598 ) ) ;
#2538=CARTESIAN_POINT ( 'NONE',  ( -26.29305231718579350, 7.800000000000001599, -19.10302069950537884 ) ) ;
#2539=CARTESIAN_POINT ( 'NONE',  ( -1.778240108872766143E-15, 18.00000000546237544, -32.49999999999999289 ) ) ;
#2541=CARTESIAN_POINT ( 'NONE',  ( -27.16883889988624290, 48.92500000273120264, -19.73931689729374028 ) ) ;
#2544=CARTESIAN_POINT ( 'NONE',  ( -10.37757302488623701, 41.77500000273118275, 31.93888565452638417 ) ) ;
#2545=DIRECTION ( 'NONE',  ( -0.000000000000000000, -1.000000000000000000, -0.000000000000000000 ) ) ;
#2547=CARTESIAN_POINT ( 'NONE',  ( -20.08610463437157989, 61.69999999999999574, -27.64615127144129758 ) ) ;
#2548=DIRECTION ( 'NONE',  ( 1.000000000000000000, 0.000000000000000000, 0.000000000000000000 ) ) ;
#2553=CARTESIAN_POINT ( 'NONE',  ( 24.50000000000000000, 12.09999999999999609, -7.960532557706203605 ) ) ;
#2556=CARTESIAN_POINT ( 'NONE',  ( -24.50000000000000000, 10.74999999453762811, -3.000384657911015469E-15 ) ) ;
#2557=CARTESIAN_POINT ( 'NONE',  ( -10.37757302488623701, 25.52500000273119696, 31.93888565452638417 ) ) ;
#2559=ORIENTED_EDGE ( 'NONE', *, *, #9203, .F. ) ;
#2565=VERTEX_POINT ( 'NONE', #33097 ) ;
#2568=CIRCLE ( 'NONE', #27225, 30.50000000000000000 ) ;
#2569=CARTESIAN_POINT ( 'NONE',  ( -20.75514604977248112, 35.67500000273118843, 28.56700777964554661 ) ) ;
#2570=CARTESIAN_POINT ( 'NONE',  ( -2.092463501923844636E-15, 40.00000000546237544, -34.17252228774368916 ) ) ;
#2571=EDGE_CURVE ( 'NONE', #18361, #11875, #25218, .T. ) ;
#2572=( BOUNDED_CURVE ( )  B_SPLINE_CURVE ( 2, ( #31231, #4981, #15460, #7723, #18211, #14768, #25233, #1708, #12186, #15970, #28992, #28824, #18717 ),
 .UNSPECIFIED., .F., .T. ) 
 B_SPLINE_CURVE_WITH_KNOTS ( ( 3, 2, 2, 2, 2, 2, 3 ),
 ( 0.5320512820512820484, 0.5333333333333333259, 0.5358974358974358809, 0.5384615384615384359, 0.5410256410256409909, 0.5435897435897435459, 0.5448717948717948234 ),
 .UNSPECIFIED. ) 
 CURVE ( )  GEOMETRIC_REPRESENTATION_ITEM ( )  RATIONAL_B_SPLINE_CURVE ( ( 0.9755282581475768211, 0.9755282581475768211, 1.000000000000000000, 0.9510565162951535312, 1.000000000000000000, 0.9510565162951535312, 1.000000000000000000, 0.9510565162951535312, 1.000000000000000000, 0.9510565162951535312, 1.000000000000000000, 0.9755282581475768211, 0.9755282581475768211 ) ) 
 REPRESENTATION_ITEM ( '' )  );
#2575=CARTESIAN_POINT ( 'NONE',  ( 33.58253175000000113, 20.12500000273118062, -4.112674001490185761E-15 ) ) ;
#2576=CARTESIAN_POINT ( 'NONE',  ( 26.29305231718579350, 76.80000000000001137, 19.10302069950537529 ) ) ;
#2577=CARTESIAN_POINT ( 'NONE',  ( 20.75514604977249178, 52.07500000273119412, 28.56700777964553950 ) ) ;
#2580=CARTESIAN_POINT ( 'NONE',  ( -20.08610463437156923, 26.29999999999998295, 27.64615127144130113 ) ) ;
#2582=CARTESIAN_POINT ( 'NONE',  ( 10.37757302488624056, 68.52500000273120406, -31.93888565452638417 ) ) ;
#2583=CARTESIAN_POINT ( 'NONE',  ( -32.50000000000000000, 77.90000000000000568, -10.55989012756945300 ) ) ;
#2585=CARTESIAN_POINT ( 'NONE',  ( -20.75514604977248823, 61.07500000273119412, -28.56700777964554305 ) ) ;
#2587=CARTESIAN_POINT ( 'NONE',  ( 10.37757302488624767, 11.72500000273118914, 31.93888565452638417 ) ) ;
#2589=DIRECTION ( 'NONE',  ( -0.000000000000000000, 1.000000000000000000, -0.000000000000000000 ) ) ;
#2592=DIRECTION ( 'NONE',  ( -0.000000000000000000, -1.000000000000000000, -0.000000000000000000 ) ) ;
#2600=CARTESIAN_POINT ( 'NONE',  ( -5.147494310547423346, 54.44874571845315359, 32.50000000000000000 ) ) ;
#2602=CARTESIAN_POINT ( 'NONE',  ( -26.29305231718579350, 70.30000000546237970, -19.10302069950537884 ) ) ;
#2606=ORIENTED_EDGE ( 'NONE', *, *, #25136, .F. ) ;
#2611=CARTESIAN_POINT ( 'NONE',  ( 33.58253175000000113, 54.37500000273118417, -4.112674001490185761E-15 ) ) ;
#2612=CARTESIAN_POINT ( 'NONE',  ( -26.29305231718578995, 54.70000000546237828, 19.10302069950538595 ) ) ;
#2614=CARTESIAN_POINT ( 'NONE',  ( 10.37757302488624767, 43.72500000273119269, 31.93888565452638417 ) ) ;
#2615=CARTESIAN_POINT ( 'NONE',  ( -12.13525491562420910, 72.19999999999998863, 8.816778784387098611 ) ) ;
#2616=CARTESIAN_POINT ( 'NONE',  ( -33.58253175000000113, 71.37500000273119838, 0.000000000000000000 ) ) ;
#2617=CARTESIAN_POINT ( 'NONE',  ( 32.50000000000000711, 1.400000005462371799, 10.55989012756945122 ) ) ;
#2620=CARTESIAN_POINT ( 'NONE',  ( -32.50000000000000000, 45.99999999999998579, 0.000000000000000000 ) ) ;
#2622=CARTESIAN_POINT ( 'NONE',  ( -2.162160676586881955E-15, 8.875000002731189497, -35.31076352940723240 ) ) ;
#2625=CARTESIAN_POINT ( 'NONE',  ( 8.601468415847516980, 78.67500000273119554, -11.83890561707634781 ) ) ;
#2627=DIRECTION ( 'NONE',  ( 0.000000000000000000, 1.000000000000000000, 0.000000000000000000 ) ) ;
#2630=ORIENTED_EDGE ( 'NONE', *, *, #12936, .T. ) ;
#2631=DIRECTION ( 'NONE',  ( 0.000000000000000000, -1.000000000000000000, 0.000000000000000000 ) ) ;
#2641=CARTESIAN_POINT ( 'NONE',  ( 33.58253175000000113, 38.12500000273119838, -4.112674001490185761E-15 ) ) ;
#2644=CARTESIAN_POINT ( 'NONE',  ( -26.29305231718578995, 2.700000005462388497, 19.10302069950538595 ) ) ;
#2647=CARTESIAN_POINT ( 'NONE',  ( -4.635254915624208216, 70.65000000546240244, 14.26584774442730463 ) ) ;
#2649=CARTESIAN_POINT ( 'NONE',  ( -27.16883889988624290, 77.17500000273119554, -19.73931689729374028 ) ) ;
#2654=VECTOR ( 'NONE', #16217, 1000.000000000000000 ) ;
#2656=CARTESIAN_POINT ( 'NONE',  ( -10.37757302488624411, 62.72500000273117848, -31.93888565452638417 ) ) ;
#2659=CARTESIAN_POINT ( 'NONE',  ( -18.94512977948576093, 4.324999997268818674, 13.76444248337722698 ) ) ;
#2661=CARTESIAN_POINT ( 'NONE',  ( -10.37757302488624411, 2.725000002731181592, -31.93888565452638417 ) ) ;
#2662=CARTESIAN_POINT ( 'NONE',  ( -15.00000000000000000, 78.25000000546239676, 0.000000000000000000 ) ) ;
#2664=CARTESIAN_POINT ( 'NONE',  ( 5.779280353836490358E-15, 57.00000000546238965, 32.49999999999999289 ) ) ;
#2666=CARTESIAN_POINT ( 'NONE',  ( -1.778240108872766143E-15, 9.499999999999992895, -32.49999999999999289 ) ) ;
#2671=CARTESIAN_POINT ( 'NONE',  ( -9.270509831248425314, 71.95000000546238539, -12.75976212528059861 ) ) ;
#2674=CARTESIAN_POINT ( 'NONE',  ( 33.58253175000000113, 30.12500000273118772, -4.112674001490185761E-15 ) ) ;
#2677=CARTESIAN_POINT ( 'NONE',  ( 33.58253175000000113, 18.37500000273117706, -4.112674001490185761E-15 ) ) ;
#2678=CARTESIAN_POINT ( 'NONE',  ( -32.50000000000000000, 63.89999999999998437, -10.55989012756945300 ) ) ;
#2680=CARTESIAN_POINT ( 'NONE',  ( -20.75514604977248112, 77.42500000273119554, 28.56700777964554661 ) ) ;
#2683=CARTESIAN_POINT ( 'NONE',  ( -23.41746825000000243, 15.72499999726882081, 7.608796670333725309 ) ) ;
#2684=CARTESIAN_POINT ( 'NONE',  ( 27.16883889988624290, 65.92500000273118133, 19.73931689729373673 ) ) ;
#2687=CARTESIAN_POINT ( 'NONE',  ( -27.16883889988624290, 4.925000002731189319, -19.73931689729374028 ) ) ;
#2688=CARTESIAN_POINT ( 'NONE',  ( -14.47279130897152122, 18.42499999726882365, 19.92008829642072243 ) ) ;
#2694=CARTESIAN_POINT ( 'NONE',  ( 32.50000000000000711, 11.40000000546237757, 10.55989012756945122 ) ) ;
#2696=CARTESIAN_POINT ( 'NONE',  ( -27.16883889988624290, 78.92500000273116711, -19.73931689729374028 ) ) ;
#2698=CARTESIAN_POINT ( 'NONE',  ( 18.94512977948575738, 18.42499999726882010, 13.76444248337723408 ) ) ;
#2699=CARTESIAN_POINT ( 'NONE',  ( 20.75514604977249178, 16.07500000273119412, 28.56700777964553950 ) ) ;
#2700=CARTESIAN_POINT ( 'NONE',  ( -32.50000000000000000, 62.00000000000000000, 0.000000000000000000 ) ) ;
#2704=CARTESIAN_POINT ( 'NONE',  ( 4.300734207923757602, 78.77500000273118985, -13.23629886949340673 ) ) ;
#2707=CARTESIAN_POINT ( 'NONE',  ( 19.82091636218621034, 15.80000000000000782, 14.40073868116559730 ) ) ;
#2708=CARTESIAN_POINT ( 'NONE',  ( 20.08610463437158344, 2.700000000000001954, 27.64615127144129403 ) ) ;
#2709=CARTESIAN_POINT ( 'NONE',  ( -2.375766604868041476, 74.44874571845315359, 14.99999999999999822 ) ) ;
#2711=CARTESIAN_POINT ( 'NONE',  ( 33.58253175000000113, 48.22500000273119269, -10.91162601494193751 ) ) ;
#2713=CARTESIAN_POINT ( 'NONE',  ( 27.16883889988624290, 34.17500000273118843, 19.73931689729373673 ) ) ;
#2715=CARTESIAN_POINT ( 'NONE',  ( 26.29305231718579350, 15.30000000546238859, 19.10302069950537529 ) ) ;
#2719=CARTESIAN_POINT ( 'NONE',  ( 5.147494310547434893, 6.551254281546842861, 32.49999999999999289 ) ) ;
#2721=CARTESIAN_POINT ( 'NONE',  ( 15.14183272437242067, 9.449999994537636283, 20.84094480462498211 ) ) ;
#2724=EDGE_CURVE ( 'NONE', #32915, #3462, #740, .T. ) ;
#2725=CARTESIAN_POINT ( 'NONE',  ( -10.37757302488623701, 23.52500000273119340, 31.93888565452638417 ) ) ;
#2734=DIRECTION ( 'NONE',  ( -0.000000000000000000, 1.000000000000000000, -0.000000000000000000 ) ) ;
#2735=CARTESIAN_POINT ( 'NONE',  ( 27.16883889988624290, 34.17500000273118843, 19.73931689729373673 ) ) ;
#2736=CARTESIAN_POINT ( 'NONE',  ( 26.29305231718578995, 39.70000000546236407, -19.10302069950538240 ) ) ;
#2737=CARTESIAN_POINT ( 'NONE',  ( -2.092463501923844636E-15, 79.49999999999998579, -34.17252228774368916 ) ) ;
#2739=CARTESIAN_POINT ( 'NONE',  ( 19.82091636218621389, 5.949999994537630066, -14.40073868116559197 ) ) ;
#2740=CARTESIAN_POINT ( 'NONE',  ( 33.58253175000000113, 50.37500000273120548, -4.112674001490185761E-15 ) ) ;
#2742=CARTESIAN_POINT ( 'NONE',  ( 26.29305231718579350, 24.79999999999999005, 19.10302069950537529 ) ) ;
#2744=CARTESIAN_POINT ( 'NONE',  ( 20.75514604977249178, 69.82500000273118701, 28.56700777964553950 ) ) ;
#2747=CARTESIAN_POINT ( 'NONE',  ( 27.16883889988623935, 60.57500000273119412, -19.73931689729374384 ) ) ;
#2748=CARTESIAN_POINT ( 'NONE',  ( -4.934616302121927505E-14, 72.50000000000001421, 32.50000000000000000 ) ) ;
#2749=CARTESIAN_POINT ( 'NONE',  ( -20.75514604977248823, 14.82500000273117635, -28.56700777964554305 ) ) ;
#2752=CARTESIAN_POINT ( 'NONE',  ( 10.37757302488624056, 4.775000002731177418, -31.93888565452638417 ) ) ;
#2754=CARTESIAN_POINT ( 'NONE',  ( 0.000000000000000000, 80.00000000000001421, 0.000000000000000000 ) ) ;
#2755=CARTESIAN_POINT ( 'NONE',  ( 10.04305231718578817, 19.40000000000000213, -30.90933677959249337 ) ) ;
#2759=EDGE_CURVE ( 'NONE', #8583, #21853, #17675, .T. ) ;
#2762=( BOUNDED_CURVE ( )  B_SPLINE_CURVE ( 2, ( #15329, #30407, #33502, #25448, #2449, #12915, #19959, #17559, #10178, #28361, #23220, #4848, #20478 ),
 .UNSPECIFIED., .F., .T. ) 
 B_SPLINE_CURVE_WITH_KNOTS ( ( 3, 2, 2, 2, 2, 2, 3 ),
 ( 0.07051282051282051211, 0.07179487179487178961, 0.07435897435897435848, 0.07692307692307692735, 0.07948717948717948234, 0.08205128205128205121, 0.08333333333333334259 ),
 .UNSPECIFIED. ) 
 CURVE ( )  GEOMETRIC_REPRESENTATION_ITEM ( )  RATIONAL_B_SPLINE_CURVE ( ( 0.9755282581475768211, 0.9755282581475768211, 1.000000000000000000, 0.9510565162951535312, 1.000000000000000000, 0.9510565162951535312, 1.000000000000000000, 0.9510565162951535312, 1.000000000000000000, 0.9510565162951535312, 1.000000000000000000, 0.9755282581475765991, 0.9755282581475767101 ) ) 
 REPRESENTATION_ITEM ( '' )  );
#2763=CARTESIAN_POINT ( 'NONE',  ( -18.94512977948576093, 4.324999997268818674, 13.76444248337722698 ) ) ;
#2764=EDGE_CURVE ( 'NONE', #21391, #5051, #15272, .T. ) ;
#2765=CARTESIAN_POINT ( 'NONE',  ( -32.50000000000000000, 72.40000000546235981, -10.55989012756945478 ) ) ;
#2768=( BOUNDED_CURVE ( )  B_SPLINE_CURVE ( 2, ( #26802, #21990, #3296, #19585, #6367, #19085, #11023, #32438, #9104, #27301, #703, #30033, #17011 ),
 .UNSPECIFIED., .F., .T. ) 
 B_SPLINE_CURVE_WITH_KNOTS ( ( 3, 2, 2, 2, 2, 2, 3 ),
 ( 0.08333333333333334259, 0.08888888888888889228, 0.1000000000000000056, 0.1111111111111111049, 0.1222222222222222182, 0.1333333333333333315, 0.1388888888888888673 ),
 .UNSPECIFIED. ) 
 CURVE ( )  GEOMETRIC_REPRESENTATION_ITEM ( )  RATIONAL_B_SPLINE_CURVE ( ( 0.9755282581475768211, 0.9755282581475768211, 1.000000000000000000, 0.9510565162951535312, 1.000000000000000000, 0.9510565162951535312, 1.000000000000000000, 0.9510565162951535312, 1.000000000000000000, 0.9510565162951535312, 1.000000000000000000, 0.9755282581475768211, 0.9755282581475768211 ) ) 
 REPRESENTATION_ITEM ( '' )  );
#2775=CARTESIAN_POINT ( 'NONE',  ( 33.58253175000000113, 54.47500000273117138, -10.91162601494193751 ) ) ;
#2776=CARTESIAN_POINT ( 'NONE',  ( -20.08610463437157989, 54.20000000546237118, -27.64615127144129758 ) ) ;
#2778=CARTESIAN_POINT ( 'NONE',  ( -10.37757302488623701, 39.52500000273118275, 31.93888565452638417 ) ) ;
#2779=CARTESIAN_POINT ( 'NONE',  ( 20.08610463437158344, 54.69999999999998153, 27.64615127144129403 ) ) ;
#2780=CARTESIAN_POINT ( 'NONE',  ( 10.37757302488624767, 67.97500000273117848, 31.93888565452638417 ) ) ;
#2781=LINE ( 'NONE', #21154, #30983 ) ;
#2784=CARTESIAN_POINT ( 'NONE',  ( -32.50000000000000000, 46.09999999999999432, 10.55989012756946366 ) ) ;
#2786=CARTESIAN_POINT ( 'NONE',  ( 33.58253175000000113, 8.475000002731173154, -10.91162601494193751 ) ) ;
#2787=CARTESIAN_POINT ( 'NONE',  ( 2.445080149700053643E-15, 72.75000000546238255, 15.00000000000000000 ) ) ;
#2790=CYLINDRICAL_SURFACE ( 'NONE', #29718, 32.50000000000000000 ) ;
#2791=DIRECTION ( 'NONE',  ( -0.000000000000000000, 1.000000000000000000, -0.000000000000000000 ) ) ;
#2793=ORIENTED_EDGE ( 'NONE', *, *, #24665, .F. ) ;
#2804=CARTESIAN_POINT ( 'NONE',  ( -33.58253175000000113, 39.22500000273119269, 10.91162601494193929 ) ) ;
#2807=CARTESIAN_POINT ( 'NONE',  ( -1.778240108872766143E-15, 2.000000005462374997, -32.49999999999999289 ) ) ;
#2812=CARTESIAN_POINT ( 'NONE',  ( 33.58253175000000823, 70.27500000273118985, 10.91162601494192863 ) ) ;
#2813=EDGE_LOOP ( 'NONE', ( #32705, #11051, #23902, #10204 ) ) ;
#2817=CARTESIAN_POINT ( 'NONE',  ( -26.29305231718579350, 14.30000000546238681, -19.10302069950537884 ) ) ;
#2818=CARTESIAN_POINT ( 'NONE',  ( 27.16883889988623935, 62.32500000273119412, -19.73931689729374384 ) ) ;
#2821=CARTESIAN_POINT ( 'NONE',  ( 23.41746824999999887, 7.024999997268802865, 7.608796670333735079 ) ) ;
#2823=CARTESIAN_POINT ( 'NONE',  ( -20.75514604977248112, 5.425000002731182214, 28.56700777964554661 ) ) ;
#2824=CARTESIAN_POINT ( 'NONE',  ( -27.16883889988623935, 29.57500000273119412, 19.73931689729374739 ) ) ;
#2825=CARTESIAN_POINT ( 'NONE',  ( 10.04305231718578817, 5.900000005462368691, -30.90933677959249337 ) ) ;
#2828=CARTESIAN_POINT ( 'NONE',  ( -13.91746824999999532, 78.97500000273117848, 4.522059556121122093 ) ) ;
#2829=CARTESIAN_POINT ( 'NONE',  ( 10.04305231718579705, 8.599999999999996092, 30.90933677959248982 ) ) ;
#2833=CARTESIAN_POINT ( 'NONE',  ( 13.91746824999999532, 79.97500000273117848, -4.522059556121118540 ) ) ;
#2835=CARTESIAN_POINT ( 'NONE',  ( 33.58253175000000113, 22.12500000273118062, -4.112674001490185761E-15 ) ) ;
#2837=AXIS2_PLACEMENT_3D ( 'NONE', #5449, #28608, #23309 ) ;
#2839=CARTESIAN_POINT ( 'NONE',  ( 10.37757302488624056, 12.77500000273118452, -31.93888565452638417 ) ) ;
#2842=CARTESIAN_POINT ( 'NONE',  ( -10.37757302488623701, 77.52500000273118985, 31.93888565452638417 ) ) ;
#2843=CYLINDRICAL_SURFACE ( 'NONE', #14633, 32.50000000000000000 ) ;
#2845=CARTESIAN_POINT ( 'NONE',  ( 15.00000000000000000, 79.35000000546239107, -4.873795443493596835 ) ) ;
#2846=CARTESIAN_POINT ( 'NONE',  ( 27.16883889988623935, 60.32500000273119412, -19.73931689729374384 ) ) ;
#2848=ORIENTED_EDGE ( 'NONE', *, *, #15661, .T. ) ;
#2851=CARTESIAN_POINT ( 'NONE',  ( -7.236395654485757944, 15.72499999726881192, -22.27133577429736988 ) ) ;
#2853=EDGE_CURVE ( 'NONE', #27023, #19766, #20254, .T. ) ;
#2854=ORIENTED_EDGE ( 'NONE', *, *, #32725, .T. ) ;
#2857=ORIENTED_EDGE ( 'NONE', *, *, #17508, .T. ) ;
#2861=CARTESIAN_POINT ( 'NONE',  ( -20.75514604977248823, 78.82500000273120122, -28.56700777964554305 ) ) ;
#2864=CARTESIAN_POINT ( 'NONE',  ( -23.41746825000000243, 15.52499999726882507, -7.608796670333730638 ) ) ;
#2865=CARTESIAN_POINT ( 'NONE',  ( 10.37757302488624056, 10.77500000273118275, -31.93888565452638417 ) ) ;
#2867=CARTESIAN_POINT ( 'NONE',  ( -2.092463501923844636E-15, 59.50000000000001421, -34.17252228774368916 ) ) ;
#2868=CARTESIAN_POINT ( 'NONE',  ( 4.300734207923757602, 80.27500000273118985, -13.23629886949340673 ) ) ;
#2869=CYLINDRICAL_SURFACE ( 'NONE', #23639, 24.50000000000000000 ) ;
#2871=CARTESIAN_POINT ( 'NONE',  ( 13.91746824999999532, 78.47500000273116427, -4.522059556121118540 ) ) ;
#2875=CARTESIAN_POINT ( 'NONE',  ( 0.000000000000000000, 82.00000000000001421, 0.000000000000000000 ) ) ;
#2877=CARTESIAN_POINT ( 'NONE',  ( 32.50000000000000000, 3.000000000000002665, -3.980102097228898626E-15 ) ) ;
#2878=CARTESIAN_POINT ( 'NONE',  ( 0.000000000000000000, 80.00000000000001421, 0.000000000000000000 ) ) ;
#2880=CARTESIAN_POINT ( 'NONE',  ( 10.37757302488624056, 42.52500000273118275, -31.93888565452638417 ) ) ;
#2884=CARTESIAN_POINT ( 'NONE',  ( -20.75514604977248823, 37.07500000273120122, -28.56700777964554305 ) ) ;
#2885=CARTESIAN_POINT ( 'NONE',  ( 26.29305231718578995, 23.70000000546237828, -19.10302069950538240 ) ) ;
#2887=CARTESIAN_POINT ( 'NONE',  ( -4.223320258572819786E-15, 9.499999999999992895, 24.50000000000000000 ) ) ;
#2888=CARTESIAN_POINT ( 'NONE',  ( 32.50000000000000711, 51.40000000546238823, 10.55989012756945122 ) ) ;
#2892=CARTESIAN_POINT ( 'NONE',  ( 7.570916362186213000, 10.14999999453763913, -23.30088464923126423 ) ) ;
#2895=CARTESIAN_POINT ( 'NONE',  ( -20.08610463437157989, 11.70000000000000817, -27.64615127144129758 ) ) ;
#2896=CARTESIAN_POINT ( 'NONE',  ( 6.486482029760648627E-15, 25.62500000273118417, 35.31076352940722529 ) ) ;
#2903=VECTOR ( 'NONE', #2592, 1000.000000000000000 ) ;
#2906=CARTESIAN_POINT ( 'NONE',  ( 0.000000000000000000, 80.00000000000001421, 0.000000000000000000 ) ) ;
#2907=CARTESIAN_POINT ( 'NONE',  ( 33.58253175000000823, 28.27500000273118985, 10.91162601494192863 ) ) ;
#2908=( BOUNDED_CURVE ( )  B_SPLINE_CURVE ( 2, ( #17410, #22724, #12074, #28382, #30427, #4527, #20156, #27872, #33172, #7616, #1948, #33525, #12769 ),
 .UNSPECIFIED., .F., .F. ) 
 B_SPLINE_CURVE_WITH_KNOTS ( ( 3, 2, 2, 2, 2, 2, 3 ),
 ( 0.7243589743589743390, 0.7256410256410256165, 0.7282051282051281715, 0.7307692307692307265, 0.7333333333333332815, 0.7358974358974359475, 0.7371794871794872250 ),
 .UNSPECIFIED. ) 
 CURVE ( )  GEOMETRIC_REPRESENTATION_ITEM ( )  RATIONAL_B_SPLINE_CURVE ( ( 0.9755282581475768211, 0.9755282581475768211, 1.000000000000000000, 0.9510565162951535312, 1.000000000000000000, 0.9510565162951535312, 1.000000000000000000, 0.9510565162951535312, 1.000000000000000000, 0.9510565162951535312, 1.000000000000000000, 0.9755282581475768211, 0.9755282581475768211 ) ) 
 REPRESENTATION_ITEM ( '' )  );
#2909=CARTESIAN_POINT ( 'NONE',  ( 6.277390505771533514E-15, 35.00000000546237544, 34.17252228774368916 ) ) ;
#2910=CARTESIAN_POINT ( 'NONE',  ( 32.50000000000000711, 76.89999999999999147, 10.55989012756945122 ) ) ;
#2911=DIRECTION ( 'NONE',  ( -0.000000000000000000, -1.000000000000000000, -0.000000000000000000 ) ) ;
#2912=CARTESIAN_POINT ( 'NONE',  ( 2.489536152421872915E-14, 77.50000000000001421, -32.49999999999999289 ) ) ;
#2913=CARTESIAN_POINT ( 'NONE',  ( 27.16883889988623935, 42.57500000273117990, -19.73931689729374384 ) ) ;
#2916=CARTESIAN_POINT ( 'NONE',  ( 20.08610463437157279, 23.29999999999999361, -27.64615127144129758 ) ) ;
#2918=CARTESIAN_POINT ( 'NONE',  ( -20.75514604977248112, 69.42500000273116711, 28.56700777964554661 ) ) ;
#2919=CARTESIAN_POINT ( 'NONE',  ( 2.489536152421872915E-14, 76.00000000546238255, -32.49999999999999289 ) ) ;
#2920=CARTESIAN_POINT ( 'NONE',  ( -10.37757302488624411, 56.97500000273119980, -31.93888565452638417 ) ) ;
#2921=CARTESIAN_POINT ( 'NONE',  ( 10.04305231718578817, 7.900000005462370467, -30.90933677959249337 ) ) ;
#2922=CARTESIAN_POINT ( 'NONE',  ( -27.16883889988623935, 9.325000002731176352, 19.73931689729374739 ) ) ;
#2927=CARTESIAN_POINT ( 'NONE',  ( -20.08610463437156923, 18.80000000546237260, 27.64615127144130113 ) ) ;
#2936=CARTESIAN_POINT ( 'NONE',  ( -20.08610463437157989, 70.20000000546237118, -27.64615127144129758 ) ) ;
#2945=CARTESIAN_POINT ( 'NONE',  ( 33.58253175000000823, 52.27500000273118985, 10.91162601494192863 ) ) ;
#2946=CARTESIAN_POINT ( 'NONE',  ( 6.277390505771533514E-15, 59.00000000546238255, 34.17252228774368916 ) ) ;
#2948=CARTESIAN_POINT ( 'NONE',  ( 27.16883889988624290, 37.92500000273118843, 19.73931689729373673 ) ) ;
#2950=CARTESIAN_POINT ( 'NONE',  ( -2.162160676586881955E-15, 66.87500000273119838, -35.31076352940723240 ) ) ;
#2951=CARTESIAN_POINT ( 'NONE',  ( -26.29305231718578995, 0.7000000054623867207, 19.10302069950538595 ) ) ;
#2952=VECTOR ( 'NONE', #28754, 1000.000000000000114 ) ;
#2955=CARTESIAN_POINT ( 'NONE',  ( -32.50000000000000000, 37.89999999999999858, -10.55989012756945478 ) ) ;
#2957=ADVANCED_FACE ( 'NONE', ( #15621 ), #18365, .T. ) ;
#2958=CARTESIAN_POINT ( 'NONE',  ( 33.58253175000000823, 8.275000002731179194, 10.91162601494192863 ) ) ;
#2959=CARTESIAN_POINT ( 'NONE',  ( 3.880418787951134707, 19.30125427608447808, 24.50000000000000000 ) ) ;
#2962=CARTESIAN_POINT ( 'NONE',  ( 20.75514604977249178, 70.07500000273120122, 28.56700777964553950 ) ) ;
#2963=DIRECTION ( 'NONE',  ( -0.000000000000000000, -1.000000000000000000, -0.000000000000000000 ) ) ;
#2964=ADVANCED_FACE ( 'NONE', ( #28810 ), #8047, .T. ) ;
#2966=VERTEX_POINT ( 'NONE', #10799 ) ;
#2973=( BOUNDED_CURVE ( )  B_SPLINE_CURVE ( 2, ( #18754, #2959, #5361, #18588, #8430, #16012, #26466 ),
 .UNSPECIFIED., .F., .T. ) 
 B_SPLINE_CURVE_WITH_KNOTS ( ( 3, 2, 2, 3 ),
 ( 0.9722222222222222099, 0.9777777777777777457, 0.9888888888888889284, 1.000000000000000000 ),
 .UNSPECIFIED. ) 
 CURVE ( )  GEOMETRIC_REPRESENTATION_ITEM ( )  RATIONAL_B_SPLINE_CURVE ( ( 0.9755282581475768211, 0.9755282581475768211, 1.000000000000000000, 0.9510565162951535312, 1.000000000000000000, 0.9510565162951535312, 1.000000000000000000 ) ) 
 REPRESENTATION_ITEM ( '' )  );
#2978=VECTOR ( 'NONE', #33292, 1000.000000000000000 ) ;
#2979=CARTESIAN_POINT ( 'NONE',  ( 6.486482029760648627E-15, 37.62500000273118417, 35.31076352940722529 ) ) ;
#2987=CARTESIAN_POINT ( 'NONE',  ( 6.486482029760649416E-15, 71.87500000273116996, 35.31076352940723240 ) ) ;
#2988=ORIENTED_EDGE ( 'NONE', *, *, #22050, .F. ) ;
#2991=EDGE_LOOP ( 'NONE', ( #1711, #23249, #6389, #2164 ) ) ;
#2992=CARTESIAN_POINT ( 'NONE',  ( 20.75514604977248467, 60.42500000273118133, -28.56700777964554305 ) ) ;
#2994=CARTESIAN_POINT ( 'NONE',  ( -20.08610463437156923, 18.80000000546237615, 27.64615127144130113 ) ) ;
#2995=CARTESIAN_POINT ( 'NONE',  ( -7.570916362186210335, 16.60000000000000497, -23.30088464923126779 ) ) ;
#2996=CARTESIAN_POINT ( 'NONE',  ( 14.47279130897151767, 6.824999997268808904, 19.92008829642072953 ) ) ;
#2997=CARTESIAN_POINT ( 'NONE',  ( -27.16883889988623935, 5.325000002731172799, 19.73931689729374739 ) ) ;
#2998=CARTESIAN_POINT ( 'NONE',  ( -27.16883889988624290, 29.17500000273118133, -19.73931689729374028 ) ) ;
#3001=CYLINDRICAL_SURFACE ( 'NONE', #24012, 32.50000000000000000 ) ;
#3002=CARTESIAN_POINT ( 'NONE',  ( 13.91746824999999532, 79.97500000273117848, -4.522059556121118540 ) ) ;
#3008=CARTESIAN_POINT ( 'NONE',  ( 8.601468415847520532, 77.57500000273118701, 11.83890561707634781 ) ) ;
#3010=CARTESIAN_POINT ( 'NONE',  ( 20.75514604977249178, 27.82500000273116925, 28.56700777964553950 ) ) ;
#3013=CARTESIAN_POINT ( 'NONE',  ( 20.75514604977248467, 16.67500000273117422, -28.56700777964554305 ) ) ;
#3015=CARTESIAN_POINT ( 'NONE',  ( -27.16883889988623935, 71.32500000273117280, 19.73931689729374739 ) ) ;
#3016=CARTESIAN_POINT ( 'NONE',  ( 10.04305231718578817, 3.900000005462367358, -30.90933677959249337 ) ) ;
#3018=CARTESIAN_POINT ( 'NONE',  ( -8.891200544363830713E-16, 71.75000000546238255, -15.00000000000000000 ) ) ;
#3019=CARTESIAN_POINT ( 'NONE',  ( -33.58253175000000113, 59.02500000273120406, -10.91162601494193041 ) ) ;
#3023=ORIENTED_EDGE ( 'NONE', *, *, #32629, .T. ) ;
#3026=CARTESIAN_POINT ( 'NONE',  ( -23.41746825000000598, 1.724999997268824581, 7.608796670333726198 ) ) ;
#3028=ORIENTED_EDGE ( 'NONE', *, *, #2332, .F. ) ;
#3030=CARTESIAN_POINT ( 'NONE',  ( -26.29305231718579350, 68.30000000546237970, -19.10302069950537884 ) ) ;
#3033=CARTESIAN_POINT ( 'NONE',  ( 32.50000000000000711, 4.899999999999990585, 10.55989012756945122 ) ) ;
#3035=CARTESIAN_POINT ( 'NONE',  ( 20.08610463437158344, 27.20000000546237118, 27.64615127144129403 ) ) ;
#3037=CARTESIAN_POINT ( 'NONE',  ( -14.47279130897151589, 17.32499999726882933, -19.92008829642072598 ) ) ;
#3038=CARTESIAN_POINT ( 'NONE',  ( -10.37757302488624411, 8.975000002731187365, -31.93888565452638417 ) ) ;
#3040=CARTESIAN_POINT ( 'NONE',  ( -2.092463501923844636E-15, 61.50000000000000000, -34.17252228774368916 ) ) ;
#3041=CARTESIAN_POINT ( 'NONE',  ( -13.91746824999999887, 78.87500000273118417, 0.000000000000000000 ) ) ;
#3044=CARTESIAN_POINT ( 'NONE',  ( 8.601468415847516980, 78.67500000273119554, -11.83890561707634781 ) ) ;
#3046=FACE_OUTER_BOUND ( 'NONE', #9410, .T. ) ;
#3048=CARTESIAN_POINT ( 'NONE',  ( -32.50000000000000000, 2.099999999999991651, 10.55989012756946366 ) ) ;
#3049=VECTOR ( 'NONE', #18827, 1000.000000000000000 ) ;
#3050=CARTESIAN_POINT ( 'NONE',  ( 32.50000000000000000, 17.60000000546238397, -10.55989012756945833 ) ) ;
#3052=CARTESIAN_POINT ( 'NONE',  ( -27.16883889988623935, 45.32500000273117990, 19.73931689729374739 ) ) ;
#3055=CARTESIAN_POINT ( 'NONE',  ( 33.58253175000000113, 34.47500000273119269, -10.91162601494193574 ) ) ;
#3056=CARTESIAN_POINT ( 'NONE',  ( 10.04305231718579705, 23.10000000546236265, 30.90933677959248982 ) ) ;
#3059=CARTESIAN_POINT ( 'NONE',  ( 26.29305231718578995, 31.20000000000000639, -19.10302069950538240 ) ) ;
#3061=VECTOR ( 'NONE', #7554, 1000.000000000000000 ) ;
#3063=CARTESIAN_POINT ( 'NONE',  ( -23.41746824999999887, 3.524999997268825958, -7.608796670333730638 ) ) ;
#3065=FACE_OUTER_BOUND ( 'NONE', #27303, .T. ) ;
#3068=CARTESIAN_POINT ( 'NONE',  ( -10.37757302488623701, 17.52500000273118985, 31.93888565452638417 ) ) ;
#3070=ORIENTED_EDGE ( 'NONE', *, *, #20795, .T. ) ;
#3073=ORIENTED_EDGE ( 'NONE', *, *, #13138, .T. ) ;
#3077=VERTEX_POINT ( 'NONE', #26246 ) ;
#3079=CARTESIAN_POINT ( 'NONE',  ( -33.58253175000000113, 29.27500000273118630, -10.91162601494193218 ) ) ;
#3080=CARTESIAN_POINT ( 'NONE',  ( 32.50000000000000711, 39.40000000546236691, 10.55989012756945122 ) ) ;
#3081=AXIS2_PLACEMENT_3D ( 'NONE', #13260, #2631, #31944 ) ;
#3082=CARTESIAN_POINT ( 'NONE',  ( -32.50000000000000000, 77.90000000000001990, -10.55989012756945478 ) ) ;
#3084=LINE ( 'NONE', #22111, #29632 ) ;
#3085=CARTESIAN_POINT ( 'NONE',  ( -20.75514604977248823, 43.07500000273118701, -28.56700777964554305 ) ) ;
#3087=CARTESIAN_POINT ( 'NONE',  ( -32.50000000000000000, 20.10000000000000497, 10.55989012756946366 ) ) ;
#3089=EDGE_CURVE ( 'NONE', #5024, #24073, #13710, .T. ) ;
#3090=CARTESIAN_POINT ( 'NONE',  ( -2.162160676586881955E-15, 62.62500000273116996, -35.31076352940723240 ) ) ;
#3091=CARTESIAN_POINT ( 'NONE',  ( -20.08610463437157989, 77.70000000000001705, -27.64615127144129758 ) ) ;
#3093=CARTESIAN_POINT ( 'NONE',  ( -27.16883889988624290, 51.17500000273117422, -19.73931689729374028 ) ) ;
#3095=CARTESIAN_POINT ( 'NONE',  ( 10.04305231718579705, 39.10000000546237686, 30.90933677959248982 ) ) ;
#3096=CARTESIAN_POINT ( 'NONE',  ( 33.58253175000000113, 6.225000002731185589, -10.91162601494193751 ) ) ;
#3099=CARTESIAN_POINT ( 'NONE',  ( 1.093617666956751375E-13, 66.00000000546238255, -32.50000000000000711 ) ) ;
#3100=UNCERTAINTY_MEASURE_WITH_UNIT (LENGTH_MEASURE( 1.000000000000000082E-05 ), #27441, 'distance_accuracy_value', 'NONE');
#3102=CARTESIAN_POINT ( 'NONE',  ( -32.50000000000000000, 18.50000000546236834, 0.000000000000000000 ) ) ;
#3110=CARTESIAN_POINT ( 'NONE',  ( 32.50000000000000000, 71.50000000546235412, -3.980102097228898626E-15 ) ) ;
#3113=ORIENTED_EDGE ( 'NONE', *, *, #27812, .T. ) ;
#3117=CARTESIAN_POINT ( 'NONE',  ( 5.147494310547434893, 74.55125428154683220, 32.49999999999999289 ) ) ;
#3118=CARTESIAN_POINT ( 'NONE',  ( 6.486482029760649416E-15, 49.87500000273119838, 35.31076352940723240 ) ) ;
#3119=CARTESIAN_POINT ( 'NONE',  ( -20.08610463437157989, 56.20000000546239249, -27.64615127144129758 ) ) ;
#3121=CARTESIAN_POINT ( 'NONE',  ( -27.16883889988624290, 34.92500000273118843, -19.73931689729374028 ) ) ;
#3122=CARTESIAN_POINT ( 'NONE',  ( 20.75514604977248467, 62.67500000273117422, -28.56700777964554305 ) ) ;
#3124=CARTESIAN_POINT ( 'NONE',  ( -1.778240108872766143E-15, 23.49999999999999645, -32.49999999999999289 ) ) ;
#3126=CARTESIAN_POINT ( 'NONE',  ( -20.08610463437157989, 41.69999999999999574, -27.64615127144129758 ) ) ;
#3128=CARTESIAN_POINT ( 'NONE',  ( 6.486482029760649416E-15, 5.875000002731167292, 35.31076352940723240 ) ) ;
#3129=CARTESIAN_POINT ( 'NONE',  ( 32.50000000000000000, 35.60000000546237686, -10.55989012756945833 ) ) ;
#3130=CARTESIAN_POINT ( 'NONE',  ( 11.25946833292375793, 72.17500000273119554, 8.180482586598731842 ) ) ;
#3131=CARTESIAN_POINT ( 'NONE',  ( -10.37757302488624411, 72.97500000273119269, -31.93888565452638417 ) ) ;
#3132=DIRECTION ( 'NONE',  ( 0.000000000000000000, -0.000000000000000000, 1.000000000000000000 ) ) ;
#3136=DIRECTION ( 'NONE',  ( -0.000000000000000000, -1.000000000000000000, -0.000000000000000000 ) ) ;
#3146=CARTESIAN_POINT ( 'NONE',  ( -20.08610463437157989, 56.20000000546238539, -27.64615127144129758 ) ) ;
#3147=CARTESIAN_POINT ( 'NONE',  ( 6.486482029760648627E-15, 41.62500000273116285, 35.31076352940722529 ) ) ;
#3151=ORIENTED_EDGE ( 'NONE', *, *, #9021, .F. ) ;
#3152=ADVANCED_FACE ( 'NONE', ( #24010 ), #5814, .F. ) ;
#3154=LINE ( 'NONE', #13784, #21763 ) ;
#3156=CARTESIAN_POINT ( 'NONE',  ( -27.16883889988624290, 71.17500000273119554, -19.73931689729374028 ) ) ;
#3161=ORIENTED_EDGE ( 'NONE', *, *, #22557, .F. ) ;
#3162=CARTESIAN_POINT ( 'NONE',  ( 32.50000000000000711, 65.40000000546237402, 10.55989012756945122 ) ) ;
#3163=CARTESIAN_POINT ( 'NONE',  ( -27.16883889988624290, 54.92500000273120264, -19.73931689729374028 ) ) ;
#3166=CARTESIAN_POINT ( 'NONE',  ( 26.29305231718579350, 15.30000000546238859, 19.10302069950537529 ) ) ;
#3168=CARTESIAN_POINT ( 'NONE',  ( -14.47279130897151767, 5.824999997268811569, -19.92008829642072598 ) ) ;
#3169=CARTESIAN_POINT ( 'NONE',  ( -10.37757302488624411, 28.97500000273117848, -31.93888565452638417 ) ) ;
#3173=CARTESIAN_POINT ( 'NONE',  ( -26.29305231718578995, 4.199999999999981526, 19.10302069950538595 ) ) ;
#3174=( BOUNDED_CURVE ( )  B_SPLINE_CURVE ( 2, ( #22328, #20439, #30890, #9436, #3960, #31565, #5153, #25748, #7557, #28486, #10475, #28657, #10310 ),
 .UNSPECIFIED., .F., .F. ) 
 B_SPLINE_CURVE_WITH_KNOTS ( ( 3, 2, 2, 2, 2, 2, 3 ),
 ( 0.4807692307692307820, 0.4820512820512820595, 0.4846153846153846145, 0.4871794871794871695, 0.4897435897435897245, 0.4923076923076923350, 0.4935897435897436125 ),
 .UNSPECIFIED. ) 
 CURVE ( )  GEOMETRIC_REPRESENTATION_ITEM ( )  RATIONAL_B_SPLINE_CURVE ( ( 0.9755282581475768211, 0.9755282581475768211, 1.000000000000000000, 0.9510565162951535312, 1.000000000000000000, 0.9510565162951535312, 1.000000000000000000, 0.9510565162951535312, 1.000000000000000000, 0.9510565162951535312, 1.000000000000000000, 0.9755282581475768211, 0.9755282581475768211 ) ) 
 REPRESENTATION_ITEM ( '' )  );
#3178=CARTESIAN_POINT ( 'NONE',  ( -13.91746824999999887, 76.87500000273116996, 0.000000000000000000 ) ) ;
#3180=CARTESIAN_POINT ( 'NONE',  ( -33.58253175000000113, 23.02500000273117919, -10.91162601494193218 ) ) ;
#3183=CARTESIAN_POINT ( 'NONE',  ( 10.37757302488624767, 17.97500000273119625, 31.93888565452638417 ) ) ;
#3185=CARTESIAN_POINT ( 'NONE',  ( 10.37757302488624056, 68.52500000273120406, -31.93888565452638417 ) ) ;
#3186=CARTESIAN_POINT ( 'NONE',  ( 20.08610463437158344, 59.20000000546237828, 27.64615127144129403 ) ) ;
#3189=CARTESIAN_POINT ( 'NONE',  ( 20.75514604977248467, 58.42500000273119554, -28.56700777964554305 ) ) ;
#3192=EDGE_CURVE ( 'NONE', #24073, #25557, #13036, .T. ) ;
#3193=VERTEX_POINT ( 'NONE', #10459 ) ;
#3195=CARTESIAN_POINT ( 'NONE',  ( -5.147494310547213736, 15.55125428154684641, -32.50000000000007105 ) ) ;
#3196=CARTESIAN_POINT ( 'NONE',  ( 14.47279130897151767, 8.924999997268800556, -19.92008829642072598 ) ) ;
#3198=ADVANCED_FACE ( 'NONE', ( #31720 ), #15848, .F. ) ;
#3199=ORIENTED_EDGE ( 'NONE', *, *, #2527, .T. ) ;
#3204=CARTESIAN_POINT ( 'NONE',  ( 5.779280353836490358E-15, 11.00000000546238077, 32.49999999999999289 ) ) ;
#3206=CARTESIAN_POINT ( 'NONE',  ( 20.75514604977248467, 74.42500000273119554, -28.56700777964554305 ) ) ;
#3208=CARTESIAN_POINT ( 'NONE',  ( -4.732186688966233175E-15, 1.500000000000010880, 25.76082449383753925 ) ) ;
#3209=CARTESIAN_POINT ( 'NONE',  ( 20.75514604977248467, 8.675000002731195536, -28.56700777964554305 ) ) ;
#3210=CARTESIAN_POINT ( 'NONE',  ( -33.58253175000000113, 21.02500000273117919, -10.91162601494193218 ) ) ;
#3211=CARTESIAN_POINT ( 'NONE',  ( 2.688165632520823219E-15, 79.37500000273119838, 14.63369212191046209 ) ) ;
#3212=DIRECTION ( 'NONE',  ( -0.000000000000000000, 1.000000000000000000, -0.000000000000000000 ) ) ;
#3214=CARTESIAN_POINT ( 'NONE',  ( 2.688165632520823219E-15, 73.87500000273119838, 14.63369212191046387 ) ) ;
#3216=CYLINDRICAL_SURFACE ( 'NONE', #32141, 15.00000000000000000 ) ;
#3219=CARTESIAN_POINT ( 'NONE',  ( -10.37757302488623701, 41.52500000273118275, 31.93888565452638417 ) ) ;
#3222=CARTESIAN_POINT ( 'NONE',  ( -10.37757302488623701, 35.77500000273120406, 31.93888565452638417 ) ) ;
#3226=CARTESIAN_POINT ( 'NONE',  ( -1.778240108872766143E-15, 47.49999999999999289, -32.49999999999999289 ) ) ;
#3229=CARTESIAN_POINT ( 'NONE',  ( 7.236395654485760609, 5.024999997268825069, -22.27133577429736633 ) ) ;
#3230=CYLINDRICAL_SURFACE ( 'NONE', #6705, 32.50000000000000000 ) ;
#3233=CARTESIAN_POINT ( 'NONE',  ( -10.37757302488624411, 16.72500000273119269, -31.93888565452638417 ) ) ;
#3241=ORIENTED_EDGE ( 'NONE', *, *, #32764, .T. ) ;
#3243=CARTESIAN_POINT ( 'NONE',  ( -33.58253175000000113, 27.47500000273118204, 10.91162601494193929 ) ) ;
#3244=CARTESIAN_POINT ( 'NONE',  ( -10.04305231718579172, 34.10000000546236976, -30.90933677959248982 ) ) ;
#3246=CARTESIAN_POINT ( 'NONE',  ( -32.50000000000000000, 54.60000000546237686, 10.55989012756946366 ) ) ;
#3247=CARTESIAN_POINT ( 'NONE',  ( 0.000000000000000000, 80.00000000000001421, -32.50000000000000000 ) ) ;
#3248=CARTESIAN_POINT ( 'NONE',  ( -33.58253175000000113, 45.27500000273116854, -10.91162601494193218 ) ) ;
#3250=CARTESIAN_POINT ( 'NONE',  ( -20.08610463437156923, 22.29999999999999716, 27.64615127144130113 ) ) ;
#3252=CARTESIAN_POINT ( 'NONE',  ( 20.75514604977248467, 60.42500000273118133, -28.56700777964554305 ) ) ;
#3254=CARTESIAN_POINT ( 'NONE',  ( 6.486482029760648627E-15, 55.87500000273118417, 35.31076352940722529 ) ) ;
#3256=CARTESIAN_POINT ( 'NONE',  ( -4.223320258572819786E-15, 9.499999999999992895, 24.50000000000000000 ) ) ;
#3257=CARTESIAN_POINT ( 'NONE',  ( -33.58253175000000113, 7.025000002731188964, -10.91162601494193218 ) ) ;
#3264=CARTESIAN_POINT ( 'NONE',  ( 3.880418787951140036, 14.44874571845315536, -24.49999999999999645 ) ) ;
#3267=CARTESIAN_POINT ( 'NONE',  ( 10.04305231718579705, 48.60000000000000142, 30.90933677959248982 ) ) ;
#3271=CARTESIAN_POINT ( 'NONE',  ( 20.08610463437157279, 67.80000000546236549, -27.64615127144129758 ) ) ;
#3274=ORIENTED_EDGE ( 'NONE', *, *, #19531, .T. ) ;
#3280=CARTESIAN_POINT ( 'NONE',  ( 27.16883889988623935, 48.57500000273118701, -19.73931689729374384 ) ) ;
#3281=CARTESIAN_POINT ( 'NONE',  ( 32.50000000000000000, 51.60000000546239107, -10.55989012756945833 ) ) ;
#3283=CARTESIAN_POINT ( 'NONE',  ( -10.37757302488624411, 32.72500000273117848, -31.93888565452638417 ) ) ;
#3284=CARTESIAN_POINT ( 'NONE',  ( 20.08610463437157279, 77.80000000546237970, -27.64615127144129758 ) ) ;
#3285=CARTESIAN_POINT ( 'NONE',  ( 20.75514604977249178, 62.07500000273118701, 28.56700777964553950 ) ) ;
#3290=CARTESIAN_POINT ( 'NONE',  ( 32.50000000000000000, 41.10000000000001563, -10.55989012756945833 ) ) ;
#3292=CARTESIAN_POINT ( 'NONE',  ( -10.37757302488624411, 6.975000002731185589, -31.93888565452638417 ) ) ;
#3293=CARTESIAN_POINT ( 'NONE',  ( 26.29305231718578995, 35.70000000546236407, -19.10302069950538240 ) ) ;
#3294=CARTESIAN_POINT ( 'NONE',  ( -13.91746824999999532, 75.27500000273121827, -4.522059556121115875 ) ) ;
#3295=CARTESIAN_POINT ( 'NONE',  ( 10.37757302488624767, 71.97500000273119269, 31.93888565452638417 ) ) ;
#3296=CARTESIAN_POINT ( 'NONE',  ( 7.570916362186207671, 3.349999994537639303, 23.30088464923126779 ) ) ;
#3299=ORIENTED_EDGE ( 'NONE', *, *, #21276, .F. ) ;
#3307=PRODUCT_DEFINITION_FORMATION_WITH_SPECIFIED_SOURCE ( 'ANY', '', #9557, .NOT_KNOWN. ) ;
#3312=CARTESIAN_POINT ( 'NONE',  ( -20.75514604977248823, 36.82500000273117990, -28.56700777964554305 ) ) ;
#3315=CARTESIAN_POINT ( 'NONE',  ( -1.778240108872766143E-15, 59.50000000000000711, -32.49999999999999289 ) ) ;
#3320=CARTESIAN_POINT ( 'NONE',  ( -33.58253175000000113, 67.47500000273117848, 10.91162601494193929 ) ) ;
#3321=ORIENTED_EDGE ( 'NONE', *, *, #2853, .F. ) ;
#3324=ORIENTED_EDGE ( 'NONE', *, *, #2535, .F. ) ;
#3325=CARTESIAN_POINT ( 'NONE',  ( -5.147494310547423346, 48.94874572391553613, 32.50000000000000000 ) ) ;
#3326=CARTESIAN_POINT ( 'NONE',  ( -20.75514604977248112, 57.42500000273118843, 28.56700777964554661 ) ) ;
#3328=CARTESIAN_POINT ( 'NONE',  ( -2.092463501923844636E-15, 18.00000000546237189, -34.17252228774368916 ) ) ;
#3329=CARTESIAN_POINT ( 'NONE',  ( 4.445600272181915325E-13, 14.00000000546237544, -32.50000000000000000 ) ) ;
#3330=CARTESIAN_POINT ( 'NONE',  ( 23.41746824999999887, 11.02499999726882152, 7.608796670333735079 ) ) ;
#3331=CARTESIAN_POINT ( 'NONE',  ( -27.16883889988624290, 23.17500000273120619, -19.73931689729374028 ) ) ;
#3334=CARTESIAN_POINT ( 'NONE',  ( -5.147494310547430452, 28.05125428700921475, -32.49999999999999289 ) ) ;
#3338=CARTESIAN_POINT ( 'NONE',  ( -11.25946833292375793, 77.07500000273121543, 8.180482586598737171 ) ) ;
#3341=CARTESIAN_POINT ( 'NONE',  ( -33.58253175000000113, 23.22500000273117138, 10.91162601494193929 ) ) ;
#3346=CARTESIAN_POINT ( 'NONE',  ( 10.37757302488624767, 13.97500000273119092, 31.93888565452638417 ) ) ;
#3348=CARTESIAN_POINT ( 'NONE',  ( 27.16883889988623935, 72.32500000273117280, -19.73931689729374384 ) ) ;
#3350=CARTESIAN_POINT ( 'NONE',  ( -13.91746824999999532, 77.27500000273118985, -4.522059556121115875 ) ) ;
#3353=CARTESIAN_POINT ( 'NONE',  ( 10.37757302488624767, 55.72500000273117138, 31.93888565452638417 ) ) ;
#3357=CARTESIAN_POINT ( 'NONE',  ( 5.779280353836490358E-15, 16.50000000000000000, 32.49999999999999289 ) ) ;
#3358=CARTESIAN_POINT ( 'NONE',  ( -14.47279130897151589, 9.324999997268816898, -19.92008829642072598 ) ) ;
#3360=ORIENTED_EDGE ( 'NONE', *, *, #16600, .F. ) ;
#3362=DIRECTION ( 'NONE',  ( -0.000000000000000000, -1.000000000000000000, -0.000000000000000000 ) ) ;
#3363=ORIENTED_EDGE ( 'NONE', *, *, #7756, .F. ) ;
#3365=CARTESIAN_POINT ( 'NONE',  ( 5.147494310547426899, 5.448745718453162468, -32.50000000000000000 ) ) ;
#3366=CARTESIAN_POINT ( 'NONE',  ( 0.000000000000000000, 82.00000000000001421, 0.000000000000000000 ) ) ;
#3367=CARTESIAN_POINT ( 'NONE',  ( 10.37757302488624767, 75.72500000273119269, 31.93888565452638417 ) ) ;
#3369=CARTESIAN_POINT ( 'NONE',  ( 24.50000000000000355, 8.100000000000006750, -7.960532557706203605 ) ) ;
#3370=CARTESIAN_POINT ( 'NONE',  ( -27.16883889988623935, 11.57500000273120655, 19.73931689729374739 ) ) ;
#3371=CARTESIAN_POINT ( 'NONE',  ( -20.75514604977248112, 13.42500000273119198, 28.56700777964554661 ) ) ;
#3372=CARTESIAN_POINT ( 'NONE',  ( -13.91746824999999532, 80.77500000273118985, -4.522059556121115875 ) ) ;
#3376=CARTESIAN_POINT ( 'NONE',  ( 13.91746825000000065, 72.27500000273118985, 4.522059556121114987 ) ) ;
#3379=CARTESIAN_POINT ( 'NONE',  ( 32.50000000000000000, 71.09999999999999432, -10.55989012756945833 ) ) ;
#3382=CARTESIAN_POINT ( 'NONE',  ( 10.37757302488624056, 44.52500000273118275, -31.93888565452638417 ) ) ;
#3385=CARTESIAN_POINT ( 'NONE',  ( 33.58253175000000113, 32.37500000273119127, -4.112674001490185761E-15 ) ) ;
#3387=EDGE_CURVE ( 'NONE', #15614, #12770, #32314, .T. ) ;
#3389=CARTESIAN_POINT ( 'NONE',  ( 5.779280353836490358E-15, 18.50000000000000000, 32.49999999999999289 ) ) ;
#3390=CARTESIAN_POINT ( 'NONE',  ( 0.000000000000000000, 70.00000000000000000, -15.00000000000000000 ) ) ;
#3393=CARTESIAN_POINT ( 'NONE',  ( 18.94512977948575738, 4.424999997268807661, 13.76444248337723408 ) ) ;
#3396=CARTESIAN_POINT ( 'NONE',  ( -2.375766604868045029, 75.80125428700921475, -14.99999999999999822 ) ) ;
#3397=CARTESIAN_POINT ( 'NONE',  ( 33.58253175000000113, 20.22500000273117848, -10.91162601494193574 ) ) ;
#3398=CARTESIAN_POINT ( 'NONE',  ( 7.236395654485755280, 8.724999997268806595, 22.27133577429736988 ) ) ;
#3400=ORIENTED_EDGE ( 'NONE', *, *, #24650, .F. ) ;
#3402=ORIENTED_EDGE ( 'NONE', *, *, #17508, .F. ) ;
#3406=CARTESIAN_POINT ( 'NONE',  ( 14.47279130897151589, 6.324999997268824892, 19.92008829642072953 ) ) ;
#3407=CARTESIAN_POINT ( 'NONE',  ( 33.58253175000000113, 28.37500000273118772, -4.112674001490185761E-15 ) ) ;
#3408=CARTESIAN_POINT ( 'NONE',  ( -32.50000000000000000, 28.50000000546237899, 0.000000000000000000 ) ) ;
#3409=CARTESIAN_POINT ( 'NONE',  ( -26.29305231718579350, 77.80000000000001137, -19.10302069950537884 ) ) ;
#3410=CARTESIAN_POINT ( 'NONE',  ( 5.147494310547426899, 33.94874572391552192, -32.50000000000000000 ) ) ;
#3411=CYLINDRICAL_SURFACE ( 'NONE', #33493, 32.50000000000000000 ) ;
#3412=CARTESIAN_POINT ( 'NONE',  ( -10.37757302488624411, 40.97500000273118559, -31.93888565452638417 ) ) ;
#3414=CARTESIAN_POINT ( 'NONE',  ( -26.29305231718579350, 23.79999999999998650, -19.10302069950537884 ) ) ;
#3416=CARTESIAN_POINT ( 'NONE',  ( 33.58253175000000113, 62.22500000273119269, -10.91162601494193751 ) ) ;
#3417=CARTESIAN_POINT ( 'NONE',  ( -20.75514604977248823, 57.07500000273117990, -28.56700777964554305 ) ) ;
#3420=CARTESIAN_POINT ( 'NONE',  ( -10.37757302488624411, 8.725000002731187365, -31.93888565452638417 ) ) ;
#3425=CARTESIAN_POINT ( 'NONE',  ( -1.778240108872766143E-15, 19.50000000000000000, -32.49999999999999289 ) ) ;
#3429=CARTESIAN_POINT ( 'NONE',  ( -5.147494310547430452, 30.05125428700921475, -32.49999999999999289 ) ) ;
#3432=FACE_OUTER_BOUND ( 'NONE', #27371, .T. ) ;
#3434=AXIS2_PLACEMENT_3D ( 'NONE', #11819, #22295, #32740 ) ;
#3436=ORIENTED_EDGE ( 'NONE', *, *, #13366, .T. ) ;
#3441=ORIENTED_EDGE ( 'NONE', *, *, #3192, .T. ) ;
#3445=CARTESIAN_POINT ( 'NONE',  ( -20.08610463437156923, 36.29999999999998295, 27.64615127144130113 ) ) ;
#3446=CARTESIAN_POINT ( 'NONE',  ( 20.75514604977248467, 48.67500000273117422, -28.56700777964554305 ) ) ;
#3447=CARTESIAN_POINT ( 'NONE',  ( -10.04305231718579172, 52.10000000546239107, -30.90933677959248982 ) ) ;
#3448=DIRECTION ( 'NONE',  ( 1.000000000000000000, 0.000000000000000000, 0.000000000000000000 ) ) ;
#3449=CARTESIAN_POINT ( 'NONE',  ( -27.16883889988623935, 37.32500000273120122, 19.73931689729374739 ) ) ;
#3451=CARTESIAN_POINT ( 'NONE',  ( -2.162160676586881955E-15, 62.87500000273120548, -35.31076352940723240 ) ) ;
#3452=CARTESIAN_POINT ( 'NONE',  ( -20.08610463437156923, 42.30000000000000426, 27.64615127144130113 ) ) ;
#3454=CARTESIAN_POINT ( 'NONE',  ( 27.16883889988623935, 6.575000002731201221, -19.73931689729374384 ) ) ;
#3456=CYLINDRICAL_SURFACE ( 'NONE', #17855, 32.50000000000000000 ) ;
#3457=CARTESIAN_POINT ( 'NONE',  ( 2.688165632520823219E-15, 71.87500000273121259, 14.63369212191046387 ) ) ;
#3458=CARTESIAN_POINT ( 'NONE',  ( -20.75514604977248112, 75.67500000273119554, 28.56700777964554661 ) ) ;
#3459=DIRECTION ( 'NONE',  ( 0.000000000000000000, 0.000000000000000000, -1.000000000000000000 ) ) ;
#3460=AXIS2_PLACEMENT_3D ( 'NONE', #4843, #28357, #7418 ) ;
#3462=VERTEX_POINT ( 'NONE', #16708 ) ;
#3463=CARTESIAN_POINT ( 'NONE',  ( -24.50000000000000355, 4.649999994537640902, -7.960532557706207157 ) ) ;
#3477=ORIENTED_EDGE ( 'NONE', *, *, #17444, .F. ) ;
#3481=CARTESIAN_POINT ( 'NONE',  ( 27.16883889988623935, 68.57500000273120122, -19.73931689729374384 ) ) ;
#3489=CARTESIAN_POINT ( 'NONE',  ( 6.486482029760649416E-15, 53.62500000273119838, 35.31076352940723240 ) ) ;
#3491=CARTESIAN_POINT ( 'NONE',  ( -32.50000000000000000, 14.40000000546236691, -10.55989012756945478 ) ) ;
#3493=CARTESIAN_POINT ( 'NONE',  ( -23.41746824999999887, 16.02499999726881086, -7.608796670333730638 ) ) ;
#3494=CARTESIAN_POINT ( 'NONE',  ( -10.37757302488624411, 20.97500000273119625, -31.93888565452638417 ) ) ;
#3498=CARTESIAN_POINT ( 'NONE',  ( -20.08610463437157989, 33.70000000000001705, -27.64615127144129758 ) ) ;
#3500=ORIENTED_EDGE ( 'NONE', *, *, #3387, .F. ) ;
#3502=CARTESIAN_POINT ( 'NONE',  ( -4.300734207923759378, 76.47500000273119269, -13.23629886949340495 ) ) ;
#3504=CARTESIAN_POINT ( 'NONE',  ( -33.58253175000000113, 27.02500000273119696, -10.91162601494193218 ) ) ;
#3508=CARTESIAN_POINT ( 'NONE',  ( -2.162160676586882350E-15, 6.875000002731194826, -35.31076352940722529 ) ) ;
#3510=CARTESIAN_POINT ( 'NONE',  ( 20.75514604977249178, 69.82500000273118701, 28.56700777964553950 ) ) ;
#3512=DIRECTION ( 'NONE',  ( -0.000000000000000000, -1.000000000000000000, -0.000000000000000000 ) ) ;
#3513=CARTESIAN_POINT ( 'NONE',  ( 13.91746824999999887, 78.37500000273116996, -1.704398294459741270E-15 ) ) ;
#3515=CARTESIAN_POINT ( 'NONE',  ( -12.13525491562420910, 72.45000000546237118, 8.816778784387098611 ) ) ;
#3516=CARTESIAN_POINT ( 'NONE',  ( 10.37757302488624056, 58.52500000273119696, -31.93888565452638417 ) ) ;
#3520=CARTESIAN_POINT ( 'NONE',  ( -32.50000000000000000, 16.00000000000001421, 0.000000000000000000 ) ) ;
#3521=CARTESIAN_POINT ( 'NONE',  ( 18.94512977948576093, 4.824999997268819563, -13.76444248337722875 ) ) ;
#3523=ORIENTED_EDGE ( 'NONE', *, *, #21121, .F. ) ;
#3526=ORIENTED_EDGE ( 'NONE', *, *, #33800, .F. ) ;
#3528=CARTESIAN_POINT ( 'NONE',  ( 27.16883889988624290, 62.17500000273118133, 19.73931689729373673 ) ) ;
#3530=CARTESIAN_POINT ( 'NONE',  ( -33.58253175000000113, 77.12500000273119838, 0.000000000000000000 ) ) ;
#3532=CARTESIAN_POINT ( 'NONE',  ( -15.14183272437241889, 4.699999999999995737, -20.84094480462497856 ) ) ;
#3533=CARTESIAN_POINT ( 'NONE',  ( -33.58253175000000113, 7.375000002731169069, 0.000000000000000000 ) ) ;
#3534=CARTESIAN_POINT ( 'NONE',  ( 20.75514604977249178, 15.82500000273117102, 28.56700777964553950 ) ) ;
#3535=CARTESIAN_POINT ( 'NONE',  ( 13.91746824999999887, 73.87500000273116996, -1.704398294459741270E-15 ) ) ;
#3536=CARTESIAN_POINT ( 'NONE',  ( 0.000000000000000000, 0.000000000000000000, 24.50000000000000000 ) ) ;
#3538=CARTESIAN_POINT ( 'NONE',  ( 15.00000000000000000, 79.10000000000000853, -4.873795443493596835 ) ) ;
#3541=CARTESIAN_POINT ( 'NONE',  ( -1.778240108872766143E-15, 38.00000000546237544, -32.49999999999999289 ) ) ;
#3543=CARTESIAN_POINT ( 'NONE',  ( 20.75514604977248467, 46.42500000273119554, -28.56700777964554305 ) ) ;
#3546=CARTESIAN_POINT ( 'NONE',  ( -33.58253175000000113, 29.37500000273118772, 0.000000000000000000 ) ) ;
#3553=CARTESIAN_POINT ( 'NONE',  ( 23.41746824999999887, 6.624999997268815832, 0.000000000000000000 ) ) ;
#3556=( BOUNDED_CURVE ( )  B_SPLINE_CURVE ( 2, ( #18342, #31195, #7685, #462, #2885, #5455, #10944, #29122, #5625, #28614, #3056, #28787, #5113 ),
 .UNSPECIFIED., .F., .F. ) 
 B_SPLINE_CURVE_WITH_KNOTS ( ( 3, 2, 2, 2, 2, 2, 3 ),
 ( 0.6987179487179486781, 0.6999999999999999556, 0.7025641025641025106, 0.7051282051282051766, 0.7076923076923077316, 0.7102564102564102866, 0.7115384615384615641 ),
 .UNSPECIFIED. ) 
 CURVE ( )  GEOMETRIC_REPRESENTATION_ITEM ( )  RATIONAL_B_SPLINE_CURVE ( ( 0.9755282581475768211, 0.9755282581475768211, 1.000000000000000000, 0.9510565162951535312, 1.000000000000000000, 0.9510565162951535312, 1.000000000000000000, 0.9510565162951535312, 1.000000000000000000, 0.9510565162951535312, 1.000000000000000000, 0.9755282581475768211, 0.9755282581475768211 ) ) 
 REPRESENTATION_ITEM ( '' )  );
#3558=CARTESIAN_POINT ( 'NONE',  ( 6.486482029760648627E-15, 17.62500000273117351, 35.31076352940722529 ) ) ;
#3559=CARTESIAN_POINT ( 'NONE',  ( 23.41746824999999887, 5.124999997268814056, 0.000000000000000000 ) ) ;
#3561=ORIENTED_EDGE ( 'NONE', *, *, #25807, .F. ) ;
#3568=CARTESIAN_POINT ( 'NONE',  ( 5.147494310547434893, 38.55125428154683220, 32.49999999999999289 ) ) ;
#3569=CARTESIAN_POINT ( 'NONE',  ( 1.577395562988744260E-15, 16.24999999453762456, -25.76082449383753925 ) ) ;
#3570=EDGE_CURVE ( 'NONE', #30585, #14202, #13435, .T. ) ;
#3571=CARTESIAN_POINT ( 'NONE',  ( -23.41746825000000598, 3.724999997268819918, 7.608796670333726198 ) ) ;
#3572=CARTESIAN_POINT ( 'NONE',  ( 10.37757302488624056, 28.77500000273120051, -31.93888565452638417 ) ) ;
#3573=CARTESIAN_POINT ( 'NONE',  ( -20.08610463437157989, 34.20000000546238539, -27.64615127144129758 ) ) ;
#3574=CARTESIAN_POINT ( 'NONE',  ( 26.29305231718579350, 72.79999999999999716, 19.10302069950537529 ) ) ;
#3576=CARTESIAN_POINT ( 'NONE',  ( 15.00000000000000000, 73.09999999999996589, -4.873795443493596835 ) ) ;
#3578=CARTESIAN_POINT ( 'NONE',  ( -10.37757302488624411, 42.97500000273119269, -31.93888565452638417 ) ) ;
#3580=CARTESIAN_POINT ( 'NONE',  ( -23.41746825000000243, 12.02499999726881974, -7.608796670333730638 ) ) ;
#3581=CARTESIAN_POINT ( 'NONE',  ( 10.04305231718578817, 21.40000000000000213, -30.90933677959249337 ) ) ;
#3584=CARTESIAN_POINT ( 'NONE',  ( -20.75514604977248823, 62.82500000273119412, -28.56700777964554305 ) ) ;
#3585=CARTESIAN_POINT ( 'NONE',  ( -20.75514604977248823, 51.07500000273116569, -28.56700777964554305 ) ) ;
#3587=CARTESIAN_POINT ( 'NONE',  ( -20.75514604977248112, 3.425000002731186655, 28.56700777964554661 ) ) ;
#3589=CARTESIAN_POINT ( 'NONE',  ( 20.08610463437158344, 25.20000000546237473, 27.64615127144129403 ) ) ;
#3592=CARTESIAN_POINT ( 'NONE',  ( 0.000000000000000000, 80.00000000000001421, -32.50000000000000000 ) ) ;
#3606=ORIENTED_EDGE ( 'NONE', *, *, #14450, .F. ) ;
#3612=CARTESIAN_POINT ( 'NONE',  ( -10.37757302488623701, 45.77500000273118985, 31.93888565452638417 ) ) ;
#3613=CARTESIAN_POINT ( 'NONE',  ( -2.092463501923844636E-15, 50.00000000546237544, -34.17252228774368916 ) ) ;
#3615=CARTESIAN_POINT ( 'NONE',  ( 27.16883889988623935, 36.32500000273120122, -19.73931689729374384 ) ) ;
#3617=CARTESIAN_POINT ( 'NONE',  ( 20.75514604977249178, 60.07500000273119412, 28.56700777964553950 ) ) ;
#3620=CARTESIAN_POINT ( 'NONE',  ( -2.092463501923844636E-15, 37.50000000000000711, -34.17252228774368916 ) ) ;
#3622=CARTESIAN_POINT ( 'NONE',  ( 33.58253175000000823, 4.275000002731189852, 10.91162601494192863 ) ) ;
#3623=CARTESIAN_POINT ( 'NONE',  ( -5.147494310547450880, 70.94874572391553613, 32.49999999999999289 ) ) ;
#3625=CARTESIAN_POINT ( 'NONE',  ( 6.486482029760648627E-15, 71.87500000273116996, 35.31076352940722529 ) ) ;
#3626=CARTESIAN_POINT ( 'NONE',  ( -7.570916362186210335, 4.599999999999992539, -23.30088464923126779 ) ) ;
#3628=ORIENTED_EDGE ( 'NONE', *, *, #1325, .T. ) ;
#3629=CARTESIAN_POINT ( 'NONE',  ( 24.50000000000000355, 5.849999994537631309, -7.960532557706203605 ) ) ;
#3639=DIRECTION ( 'NONE',  ( -0.000000000000000000, -1.000000000000000000, -0.000000000000000000 ) ) ;
#3642=CARTESIAN_POINT ( 'NONE',  ( -19.82091636218621389, 17.19999999999999218, 14.40073868116558842 ) ) ;
#3643=ORIENTED_EDGE ( 'NONE', *, *, #13848, .F. ) ;
#3647=VERTEX_POINT ( 'NONE', #32467 ) ;
#3650=ORIENTED_EDGE ( 'NONE', *, *, #20550, .F. ) ;
#3651=FACE_OUTER_BOUND ( 'NONE', #29908, .T. ) ;
#3652=CARTESIAN_POINT ( 'NONE',  ( -27.16883889988624290, 52.92500000273120264, -19.73931689729374028 ) ) ;
#3654=CARTESIAN_POINT ( 'NONE',  ( -20.08610463437156923, 12.80000000546236016, 27.64615127144130113 ) ) ;
#3655=CARTESIAN_POINT ( 'NONE',  ( 1.555960095263670572E-15, 16.24999999453762101, -24.50000000000000000 ) ) ;
#3657=CARTESIAN_POINT ( 'NONE',  ( -4.523095164977117273E-15, 12.62499999726879807, 24.62258325217400312 ) ) ;
#3658=CARTESIAN_POINT ( 'NONE',  ( -26.29305231718578995, 60.20000000000000284, 19.10302069950538595 ) ) ;
#3659=CARTESIAN_POINT ( 'NONE',  ( 20.75514604977248467, 22.67500000273119198, -28.56700777964554305 ) ) ;
#3660=CARTESIAN_POINT ( 'NONE',  ( 9.270509831248425314, 76.69999999999998863, 12.75976212528059683 ) ) ;
#3662=CARTESIAN_POINT ( 'NONE',  ( 8.601468415847516980, 74.17500000273119554, -11.83890561707634781 ) ) ;
#3663=CARTESIAN_POINT ( 'NONE',  ( 24.50000000000000000, 15.89999999999998970, 7.960532557706212486 ) ) ;
#3667=ORIENTED_EDGE ( 'NONE', *, *, #14686, .T. ) ;
#3669=CARTESIAN_POINT ( 'NONE',  ( -13.91746824999999532, 76.77500000273117564, -4.522059556121115875 ) ) ;
#3671=CARTESIAN_POINT ( 'NONE',  ( -33.58253175000000113, 19.22500000273118204, 10.91162601494193929 ) ) ;
#3675=CARTESIAN_POINT ( 'NONE',  ( 27.16883889988624290, 6.175000002731190207, 19.73931689729373673 ) ) ;
#3678=DIRECTION ( 'NONE',  ( -0.000000000000000000, -1.000000000000000000, -0.000000000000000000 ) ) ;
#3679=CARTESIAN_POINT ( 'NONE',  ( 13.91746824999999887, 80.37500000273118417, -1.704398294459741270E-15 ) ) ;
#3682=CARTESIAN_POINT ( 'NONE',  ( 10.37757302488624767, 49.72500000273119269, 31.93888565452638417 ) ) ;
#3684=ORIENTED_EDGE ( 'NONE', *, *, #5519, .T. ) ;
#3686=CARTESIAN_POINT ( 'NONE',  ( 5.779280353836490358E-15, 59.00000000546238255, 32.49999999999999289 ) ) ;
#3687=CARTESIAN_POINT ( 'NONE',  ( 14.47279130897151767, 4.924999997268811214, -19.92008829642072598 ) ) ;
#3689=VERTEX_POINT ( 'NONE', #26833 ) ;
#3693=EDGE_LOOP ( 'NONE', ( #11136, #25558, #33859, #1240 ) ) ;
#3695=CARTESIAN_POINT ( 'NONE',  ( 33.58253175000000823, 58.27500000273116854, 10.91162601494192863 ) ) ;
#3697=CARTESIAN_POINT ( 'NONE',  ( -33.58253175000000113, 77.22500000273117848, 10.91162601494193929 ) ) ;
#3699=EDGE_CURVE ( 'NONE', #12256, #17243, #8968, .T. ) ;
#3700=CARTESIAN_POINT ( 'NONE',  ( 7.570916362186207671, 3.599999999999992095, 23.30088464923126779 ) ) ;
#3701=CARTESIAN_POINT ( 'NONE',  ( 2.205017735002230837E-13, 57.49999999999999289, -32.50000000000000000 ) ) ;
#3702=CARTESIAN_POINT ( 'NONE',  ( -27.16883889988623935, 19.32500000273118701, 19.73931689729374739 ) ) ;
#3703=CARTESIAN_POINT ( 'NONE',  ( -8.601468415847518756, 72.57500000273117280, -11.83890561707634603 ) ) ;
#3705=CARTESIAN_POINT ( 'NONE',  ( 12.13525491562420910, 81.19999999999998863, -8.816778784387098611 ) ) ;
#3708=EDGE_CURVE ( 'NONE', #13932, #6218, #14295, .T. ) ;
#3710=CARTESIAN_POINT ( 'NONE',  ( 5.779280353836490358E-15, 49.00000000546238255, 32.49999999999999289 ) ) ;
#3712=CARTESIAN_POINT ( 'NONE',  ( -27.16883889988623935, 39.32500000273120122, 19.73931689729374739 ) ) ;
#3715=CARTESIAN_POINT ( 'NONE',  ( 10.37757302488624056, 26.77500000273119696, -31.93888565452638417 ) ) ;
#3716=CARTESIAN_POINT ( 'NONE',  ( 24.50000000000000000, 17.89999999999998437, 7.960532557706212486 ) ) ;
#3719=VECTOR ( 'NONE', #3822, 1000.000000000000000 ) ;
#3720=CARTESIAN_POINT ( 'NONE',  ( 5.147494310547434893, 30.55125428154684997, 32.49999999999999289 ) ) ;
#3723=CARTESIAN_POINT ( 'NONE',  ( -7.236395654485763274, 2.024999997268822405, 22.27133577429736633 ) ) ;
#3727=DIRECTION ( 'NONE',  ( 0.000000000000000000, -1.000000000000000000, 0.000000000000000000 ) ) ;
#3728=CARTESIAN_POINT ( 'NONE',  ( -10.37757302488624411, 22.72500000273119980, -31.93888565452638417 ) ) ;
#3729=CARTESIAN_POINT ( 'NONE',  ( -18.94512977948575738, 5.924999997268809437, -13.76444248337723231 ) ) ;
#3734=VERTEX_POINT ( 'NONE', #3329 ) ;
#3737=CARTESIAN_POINT ( 'NONE',  ( 26.29305231718579350, 38.80000000000000426, 19.10302069950537529 ) ) ;
#3738=CARTESIAN_POINT ( 'NONE',  ( -24.50000000000001066, 16.84999999453763309, 7.960532557706201828 ) ) ;
#3739=CARTESIAN_POINT ( 'NONE',  ( 18.94512977948576093, 2.824999997268817786, -13.76444248337722875 ) ) ;
#3740=CARTESIAN_POINT ( 'NONE',  ( -2.162160676586881955E-15, 18.87500000273119483, -35.31076352940723240 ) ) ;
#3741=CARTESIAN_POINT ( 'NONE',  ( 26.29305231718578995, 31.70000000546238539, -19.10302069950538240 ) ) ;
#3742=CARTESIAN_POINT ( 'NONE',  ( -20.08610463437157989, 71.69999999999997442, -27.64615127144129758 ) ) ;
#3745=CARTESIAN_POINT ( 'NONE',  ( -10.37757302488623701, 37.77500000273118275, 31.93888565452638417 ) ) ;
#3747=CARTESIAN_POINT ( 'NONE',  ( 23.41746825000000243, 11.22499999726881548, -7.608796670333727974 ) ) ;
#3748=CARTESIAN_POINT ( 'NONE',  ( -32.50000000000000000, 12.00000000000001066, 0.000000000000000000 ) ) ;
#3751=CARTESIAN_POINT ( 'NONE',  ( -27.16883889988623935, 61.32500000273119412, 19.73931689729374739 ) ) ;
#3752=CARTESIAN_POINT ( 'NONE',  ( 20.75514604977249178, 46.07500000273117280, 28.56700777964553950 ) ) ;
#3755=CARTESIAN_POINT ( 'NONE',  ( 10.37757302488624767, 7.725000002731185589, 31.93888565452638417 ) ) ;
#3758=( BOUNDED_CURVE ( )  B_SPLINE_CURVE ( 2, ( #13535, #15776, #26232, #2721, #23998, #10106, #20585, #26399, #10615, #28457, #2892, #13020, #18180 ),
 .UNSPECIFIED., .F., .T. ) 
 B_SPLINE_CURVE_WITH_KNOTS ( ( 3, 2, 2, 2, 2, 2, 3 ),
 ( 0.4166666666666666852, 0.4222222222222222210, 0.4333333333333333481, 0.4444444444444444198, 0.4555555555555555469, 0.4666666666666666741, 0.4722222222222222099 ),
 .UNSPECIFIED. ) 
 CURVE ( )  GEOMETRIC_REPRESENTATION_ITEM ( )  RATIONAL_B_SPLINE_CURVE ( ( 0.9755282581475767101, 0.9755282581475768211, 1.000000000000000000, 0.9510565162951535312, 1.000000000000000000, 0.9510565162951535312, 1.000000000000000000, 0.9510565162951535312, 1.000000000000000000, 0.9510565162951535312, 1.000000000000000000, 0.9755282581475768211, 0.9755282581475765991 ) ) 
 REPRESENTATION_ITEM ( '' )  );
#3760=CARTESIAN_POINT ( 'NONE',  ( -20.08610463437157989, 41.69999999999999574, -27.64615127144129758 ) ) ;
#3763=CARTESIAN_POINT ( 'NONE',  ( 0.000000000000000000, 0.000000000000000000, 0.000000000000000000 ) ) ;
#3764=DIRECTION ( 'NONE',  ( 0.000000000000000000, 0.000000000000000000, -1.000000000000000000 ) ) ;
#3765=CARTESIAN_POINT ( 'NONE',  ( -1.778240108872766143E-15, 30.00000000546237189, -32.49999999999999289 ) ) ;
#3770=ORIENTED_EDGE ( 'NONE', *, *, #15128, .F. ) ;
#3778=CARTESIAN_POINT ( 'NONE',  ( 5.779280353836490358E-15, 47.00000000546238255, 32.49999999999999289 ) ) ;
#3779=CARTESIAN_POINT ( 'NONE',  ( 33.58253175000000823, 46.27500000273120406, 10.91162601494192863 ) ) ;
#3780=CARTESIAN_POINT ( 'NONE',  ( -26.29305231718579350, 52.30000000546236549, -19.10302069950537884 ) ) ;
#3782=CARTESIAN_POINT ( 'NONE',  ( -10.37757302488624411, 30.72500000273117848, -31.93888565452638417 ) ) ;
#3784=CARTESIAN_POINT ( 'NONE',  ( -27.16883889988623935, 59.57500000273119412, 19.73931689729374739 ) ) ;
#3787=CARTESIAN_POINT ( 'NONE',  ( 10.04305231718578817, 35.39999999999998437, -30.90933677959249337 ) ) ;
#3789=CARTESIAN_POINT ( 'NONE',  ( 20.75514604977249178, 4.075000002731195892, 28.56700777964553950 ) ) ;
#3790=CARTESIAN_POINT ( 'NONE',  ( 10.04305231718579705, 12.59999999999999964, 30.90933677959248982 ) ) ;
#3792=CARTESIAN_POINT ( 'NONE',  ( 10.37757302488624056, 64.77500000273117564, -31.93888565452638417 ) ) ;
#3795=CARTESIAN_POINT ( 'NONE',  ( 7.570916362186207671, 7.349999994537615322, 23.30088464923126779 ) ) ;
#3797=ADVANCED_FACE ( 'NONE', ( #8468 ), #735, .F. ) ;
#3809=DIRECTION ( 'NONE',  ( -0.000000000000000000, -1.000000000000000000, -0.000000000000000000 ) ) ;
#3811=VERTEX_POINT ( 'NONE', #20298 ) ;
#3815=VERTEX_POINT ( 'NONE', #30748 ) ;
#3818=CARTESIAN_POINT ( 'NONE',  ( -32.50000000000000000, 74.40000000546234560, -10.55989012756945300 ) ) ;
#3819=CARTESIAN_POINT ( 'NONE',  ( -10.37757302488624411, 56.72500000273117138, -31.93888565452638417 ) ) ;
#3821=CARTESIAN_POINT ( 'NONE',  ( -10.04305231718579172, 12.10000000546238041, -30.90933677959248982 ) ) ;
#3822=DIRECTION ( 'NONE',  ( -0.000000000000000000, -1.000000000000000000, -0.000000000000000000 ) ) ;
#3823=CARTESIAN_POINT ( 'NONE',  ( 18.94512977948576093, 15.32499999726882933, -13.76444248337722875 ) ) ;
#3824=CARTESIAN_POINT ( 'NONE',  ( -32.50000000000000000, 53.99999999999999289, 0.000000000000000000 ) ) ;
#3825=CARTESIAN_POINT ( 'NONE',  ( 10.37757302488624056, 26.77500000273119696, -31.93888565452638417 ) ) ;
#3828=CARTESIAN_POINT ( 'NONE',  ( -13.91746824999999532, 72.97500000273117848, 4.522059556121122093 ) ) ;
#3829=CARTESIAN_POINT ( 'NONE',  ( -8.891200544363830713E-16, 75.75000000546236834, -15.00000000000000000 ) ) ;
#3830=CARTESIAN_POINT ( 'NONE',  ( -5.147494310547423346, 34.44874571845313938, 32.50000000000000000 ) ) ;
#3834=CARTESIAN_POINT ( 'NONE',  ( 32.50000000000000000, 71.60000000546240528, -10.55989012756945833 ) ) ;
#3839=CARTESIAN_POINT ( 'NONE',  ( -20.75514604977248112, 11.67500000273118843, 28.56700777964554661 ) ) ;
#3843=CARTESIAN_POINT ( 'NONE',  ( 13.91746825000000065, 74.27500000273118985, 4.522059556121115875 ) ) ;
#3846=CARTESIAN_POINT ( 'NONE',  ( 20.75514604977248467, 52.42500000273118133, -28.56700777964554305 ) ) ;
#3848=ORIENTED_EDGE ( 'NONE', *, *, #23533, .F. ) ;
#3850=DIRECTION ( 'NONE',  ( 0.000000000000000000, -1.000000000000000000, 0.000000000000000000 ) ) ;
#3851=CARTESIAN_POINT ( 'NONE',  ( -14.47279130897151589, 7.324999997268822227, -19.92008829642072598 ) ) ;
#3856=CYLINDRICAL_SURFACE ( 'NONE', #19802, 32.50000000000000000 ) ;
#3857=EDGE_CURVE ( 'NONE', #6723, #33526, #1843, .T. ) ;
#3859=( BOUNDED_CURVE ( )  B_SPLINE_CURVE ( 2, ( #1413, #3830, #8805, #9140, #5909, #32313, #1238, #3998, #14471, #3498, #8641, #8976, #24760 ),
 .UNSPECIFIED., .F., .T. ) 
 B_SPLINE_CURVE_WITH_KNOTS ( ( 3, 2, 2, 2, 2, 2, 3 ),
 ( 0.5833333333333333703, 0.5846153846153846478, 0.5871794871794872028, 0.5897435897435897578, 0.5923076923076923128, 0.5948717948717948678, 0.5961538461538461453 ),
 .UNSPECIFIED. ) 
 CURVE ( )  GEOMETRIC_REPRESENTATION_ITEM ( )  RATIONAL_B_SPLINE_CURVE ( ( 0.9755282581475768211, 0.9755282581475768211, 1.000000000000000000, 0.9510565162951535312, 1.000000000000000000, 0.9510565162951535312, 1.000000000000000000, 0.9510565162951535312, 1.000000000000000000, 0.9510565162951535312, 1.000000000000000000, 0.9755282581475768211, 0.9755282581475768211 ) ) 
 REPRESENTATION_ITEM ( '' )  );
#3861=CARTESIAN_POINT ( 'NONE',  ( -2.162160676586881955E-15, 58.87500000273117706, -35.31076352940723240 ) ) ;
#3862=CARTESIAN_POINT ( 'NONE',  ( -20.08610463437157989, 36.20000000546237828, -27.64615127144129758 ) ) ;
#3863=CARTESIAN_POINT ( 'NONE',  ( 33.58253175000000823, 74.02500000273120406, 10.91162601494192863 ) ) ;
#3865=CARTESIAN_POINT ( 'NONE',  ( -7.570916362186215665, 5.399999999999987921, 23.30088464923126423 ) ) ;
#3866=CARTESIAN_POINT ( 'NONE',  ( 0.000000000000000000, 0.000000000000000000, 24.50000000000000000 ) ) ;
#3867=CARTESIAN_POINT ( 'NONE',  ( -27.16883889988623935, 15.32500000273118168, 19.73931689729374739 ) ) ;
#3868=CARTESIAN_POINT ( 'NONE',  ( -4.300734207923755825, 73.27500000273118985, 13.23629886949340673 ) ) ;
#3870=CARTESIAN_POINT ( 'NONE',  ( -4.635254915624208216, 80.40000000000000568, 14.26584774442730463 ) ) ;
#3876=CARTESIAN_POINT ( 'NONE',  ( 10.37757302488624056, 36.52500000273117564, -31.93888565452638417 ) ) ;
#3879=CARTESIAN_POINT ( 'NONE',  ( -27.16883889988624290, 31.17500000273118488, -19.73931689729374028 ) ) ;
#3882=CARTESIAN_POINT ( 'NONE',  ( -20.08610463437157989, 17.69999999999999218, -27.64615127144129758 ) ) ;
#3885=CARTESIAN_POINT ( 'NONE',  ( 23.41746824999999887, 12.72499999726882791, -7.608796670333727974 ) ) ;
#3887=EDGE_CURVE ( 'NONE', #438, #26701, #7237, .T. ) ;
#3891=CARTESIAN_POINT ( 'NONE',  ( 10.37757302488624056, 10.52500000273118275, -31.93888565452638417 ) ) ;
#3892=CARTESIAN_POINT ( 'NONE',  ( -14.47279130897151589, 7.824999997268807128, -19.92008829642072598 ) ) ;
#3894=EDGE_CURVE ( 'NONE', #24457, #29888, #5374, .T. ) ;
#3895=ORIENTED_EDGE ( 'NONE', *, *, #24650, .T. ) ;
#3902=CARTESIAN_POINT ( 'NONE',  ( 7.570916362186207671, 17.34999999453762243, 23.30088464923126779 ) ) ;
#3904=CARTESIAN_POINT ( 'NONE',  ( -18.94512977948575738, 3.424999997268807217, -13.76444248337723231 ) ) ;
#3905=CARTESIAN_POINT ( 'NONE',  ( 20.75514604977248467, 24.67500000273118843, -28.56700777964554305 ) ) ;
#3906=CARTESIAN_POINT ( 'NONE',  ( 20.08610463437157279, 29.80000000546237970, -27.64615127144129758 ) ) ;
#3907=CARTESIAN_POINT ( 'NONE',  ( 32.50000000000000711, 74.90000000000000568, 10.55989012756945122 ) ) ;
#3911=CARTESIAN_POINT ( 'NONE',  ( 10.37757302488624056, 38.77500000273118275, -31.93888565452638417 ) ) ;
#3914=CARTESIAN_POINT ( 'NONE',  ( 23.41746825000000243, 11.02499999726882152, 7.608796670333735079 ) ) ;
#3915=CARTESIAN_POINT ( 'NONE',  ( 10.04305231718578817, 15.39999999999999680, -30.90933677959249337 ) ) ;
#3918=CARTESIAN_POINT ( 'NONE',  ( 6.486482029760649416E-15, 53.62500000273119838, 35.31076352940723240 ) ) ;
#3919=CARTESIAN_POINT ( 'NONE',  ( 20.75514604977248467, 46.67500000273118133, -28.56700777964554305 ) ) ;
#3921=CARTESIAN_POINT ( 'NONE',  ( 24.50000000000000000, 10.00000000000000888, 0.000000000000000000 ) ) ;
#3925=CARTESIAN_POINT ( 'NONE',  ( -5.147494310547423346, 42.44874571845314648, 32.50000000000000000 ) ) ;
#3927=CARTESIAN_POINT ( 'NONE',  ( 0.000000000000000000, 80.00000000000001421, -32.50000000000000000 ) ) ;
#3930=CARTESIAN_POINT ( 'NONE',  ( 5.147494310547426899, 1.948745723915527472, -32.50000000000000000 ) ) ;
#3934=CARTESIAN_POINT ( 'NONE',  ( -33.58253175000000113, 31.12500000273119127, 0.000000000000000000 ) ) ;
#3936=VERTEX_POINT ( 'NONE', #3124 ) ;
#3940=ORIENTED_EDGE ( 'NONE', *, *, #25677, .T. ) ;
#3944=CARTESIAN_POINT ( 'NONE',  ( 26.29305231718578995, 57.20000000000000284, -19.10302069950538240 ) ) ;
#3945=CARTESIAN_POINT ( 'NONE',  ( 6.486482029760649416E-15, 41.87500000273119127, 35.31076352940723240 ) ) ;
#3946=CARTESIAN_POINT ( 'NONE',  ( -32.50000000000000000, 52.40000000546239534, -10.55989012756945478 ) ) ;
#3948=CARTESIAN_POINT ( 'NONE',  ( -27.16883889988624290, 28.92500000273118133, -19.73931689729374028 ) ) ;
#3950=CARTESIAN_POINT ( 'NONE',  ( -20.75514604977248823, 57.07500000273117280, -28.56700777964554305 ) ) ;
#3952=CARTESIAN_POINT ( 'NONE',  ( 6.277390505771533514E-15, 36.49999999999997868, 34.17252228774368916 ) ) ;
#3954=( BOUNDED_CURVE ( )  B_SPLINE_CURVE ( 2, ( #31520, #20899, #103, #31348, #25695, #10594, #2176, #276, #23811, #13338, #8014, #18499, #21241 ),
 .UNSPECIFIED., .F., .T. ) 
 B_SPLINE_CURVE_WITH_KNOTS ( ( 3, 2, 2, 2, 2, 2, 3 ),
 ( 0.05769230769230769551, 0.05897435897435897301, 0.06153846153846154188, 0.06410256410256409687, 0.06666666666666666574, 0.06923076923076923461, 0.07051282051282051211 ),
 .UNSPECIFIED. ) 
 CURVE ( )  GEOMETRIC_REPRESENTATION_ITEM ( )  RATIONAL_B_SPLINE_CURVE ( ( 0.9755282581475768211, 0.9755282581475768211, 1.000000000000000000, 0.9510565162951535312, 1.000000000000000000, 0.9510565162951535312, 1.000000000000000000, 0.9510565162951535312, 1.000000000000000000, 0.9510565162951535312, 1.000000000000000000, 0.9755282581475768211, 0.9755282581475768211 ) ) 
 REPRESENTATION_ITEM ( '' )  );
#3955=CARTESIAN_POINT ( 'NONE',  ( -27.16883889988623935, 77.32500000273118701, 19.73931689729374739 ) ) ;
#3956=CARTESIAN_POINT ( 'NONE',  ( 5.147494310547426899, 13.44874571845315536, -32.50000000000000000 ) ) ;
#3958=CARTESIAN_POINT ( 'NONE',  ( -33.58253175000000113, 65.37500000273119838, 0.000000000000000000 ) ) ;
#3960=CARTESIAN_POINT ( 'NONE',  ( -26.29305231718578995, 40.70000000546236407, 19.10302069950538595 ) ) ;
#3961=CARTESIAN_POINT ( 'NONE',  ( 19.82091636218621389, 3.949999994537628289, -14.40073868116559197 ) ) ;
#3964=AXIS2_PLACEMENT_3D ( 'NONE', #20628, #30900, #15297 ) ;
#3976=CARTESIAN_POINT ( 'NONE',  ( 10.04305231718579705, 58.59999999999998721, 30.90933677959248982 ) ) ;
#3981=ORIENTED_EDGE ( 'NONE', *, *, #24113, .F. ) ;
#3983=EDGE_CURVE ( 'NONE', #21770, #2565, #11026, .T. ) ;
#3985=CARTESIAN_POINT ( 'NONE',  ( -3.880418787951099180, 12.30125427608447097, -24.50000000000001421 ) ) ;
#3986=CARTESIAN_POINT ( 'NONE',  ( -10.37757302488623701, 51.52500000273118985, 31.93888565452638417 ) ) ;
#3988=EDGE_CURVE ( 'NONE', #1219, #27572, #1777, .T. ) ;
#3989=CARTESIAN_POINT ( 'NONE',  ( 20.08610463437157279, 9.800000005462369046, -27.64615127144129758 ) ) ;
#3991=CARTESIAN_POINT ( 'NONE',  ( 23.41746824999999887, 13.12499999726882116, 0.000000000000000000 ) ) ;
#3992=( BOUNDED_CURVE ( )  B_SPLINE_CURVE ( 2, ( #9251, #9089, #25046, #30019, #3944, #14586, #24872, #32259, #19571, #1527, #4112, #14249, #17333 ),
 .UNSPECIFIED., .F., .F. ) 
 B_SPLINE_CURVE_WITH_KNOTS ( ( 3, 2, 2, 2, 2, 2, 3 ),
 ( 0.2884615384615384914, 0.2897435897435897689, 0.2923076923076923239, 0.2948717948717948789, 0.2974358974358974339, 0.2999999999999999889, 0.3012820512820512664 ),
 .UNSPECIFIED. ) 
 CURVE ( )  GEOMETRIC_REPRESENTATION_ITEM ( )  RATIONAL_B_SPLINE_CURVE ( ( 0.9755282581475768211, 0.9755282581475772652, 1.000000000000000000, 0.9510565162951535312, 1.000000000000000000, 0.9510565162951535312, 1.000000000000000000, 0.9510565162951535312, 1.000000000000000000, 0.9510565162951535312, 1.000000000000000000, 0.9755282581475768211, 0.9755282581475768211 ) ) 
 REPRESENTATION_ITEM ( '' )  );
#3993=CARTESIAN_POINT ( 'NONE',  ( -2.092463501923844636E-15, 53.50000000000000000, -34.17252228774368916 ) ) ;
#3994=CARTESIAN_POINT ( 'NONE',  ( -10.37757302488623701, 23.77500000273119340, 31.93888565452638417 ) ) ;
#3996=CARTESIAN_POINT ( 'NONE',  ( -8.960552108402742093E-16, 76.37500000273116996, -14.63369212191046387 ) ) ;
#3998=CARTESIAN_POINT ( 'NONE',  ( -32.50000000000000000, 33.90000000000000568, -10.55989012756945300 ) ) ;
#4007=CARTESIAN_POINT ( 'NONE',  ( 6.486482029760648627E-15, 11.87500000273118062, 35.31076352940722529 ) ) ;
#4010=CARTESIAN_POINT ( 'NONE',  ( 11.25946833292375793, 76.57500000273120122, -8.180482586598735395 ) ) ;
#4013=CARTESIAN_POINT ( 'NONE',  ( 27.16883889988624290, 51.92500000273120264, 19.73931689729373673 ) ) ;
#4016=VERTEX_POINT ( 'NONE', #20387 ) ;
#4019=CARTESIAN_POINT ( 'NONE',  ( -7.236395654485763274, 10.02499999726880198, 22.27133577429736633 ) ) ;
#4021=ORIENTED_EDGE ( 'NONE', *, *, #28655, .T. ) ;
#4024=ORIENTED_EDGE ( 'NONE', *, *, #25175, .F. ) ;
#4026=CARTESIAN_POINT ( 'NONE',  ( -27.16883889988623935, 61.57500000273119412, 19.73931689729374739 ) ) ;
#4027=CARTESIAN_POINT ( 'NONE',  ( -10.04305231718579172, 36.10000000546237686, -30.90933677959248982 ) ) ;
#4028=CARTESIAN_POINT ( 'NONE',  ( -2.162160676586881955E-15, 64.62500000273121259, -35.31076352940723240 ) ) ;
#4030=CARTESIAN_POINT ( 'NONE',  ( -15.14183272437242600, 5.300000000000006928, 20.84094480462497856 ) ) ;
#4031=CARTESIAN_POINT ( 'NONE',  ( -33.58253175000000113, 3.375000002731193049, 0.000000000000000000 ) ) ;
#4032=CARTESIAN_POINT ( 'NONE',  ( 10.37757302488624767, 13.72500000273119092, 31.93888565452638417 ) ) ;
#4033=CARTESIAN_POINT ( 'NONE',  ( -13.91746824999999887, 72.87500000273119838, 0.000000000000000000 ) ) ;
#4035=CARTESIAN_POINT ( 'NONE',  ( 4.635254915624212657, 78.60000000000000853, 14.26584774442730286 ) ) ;
#4038=CARTESIAN_POINT ( 'NONE',  ( -8.891200544363830713E-16, 73.75000000546239676, -15.00000000000000000 ) ) ;
#4040=CARTESIAN_POINT ( 'NONE',  ( -12.13525491562421088, 76.05000000546239391, -8.816778784387096835 ) ) ;
#4042=CARTESIAN_POINT ( 'NONE',  ( 33.58253175000000113, 38.12500000273119838, -4.112674001490185761E-15 ) ) ;
#4045=CARTESIAN_POINT ( 'NONE',  ( -20.75514604977248823, 27.07500000273119412, -28.56700777964554305 ) ) ;
#4046=CARTESIAN_POINT ( 'NONE',  ( 5.779280353836490358E-15, 13.00000000546238077, 32.49999999999999289 ) ) ;
#4047=CARTESIAN_POINT ( 'NONE',  ( -20.08610463437156923, 8.800000005462370822, 27.64615127144130113 ) ) ;
#4048=CARTESIAN_POINT ( 'NONE',  ( 4.635254915624209993, 81.40000000000000568, -14.26584774442730463 ) ) ;
#4050=CARTESIAN_POINT ( 'NONE',  ( 1.507698388325705758E-15, 11.12499999726881761, -24.62258325217400312 ) ) ;
#4057=CARTESIAN_POINT ( 'NONE',  ( -27.16883889988623935, 13.32500000273117990, 19.73931689729374739 ) ) ;
#4058=CARTESIAN_POINT ( 'NONE',  ( -7.236395654485763274, 14.52499999726880553, 22.27133577429736633 ) ) ;
#4059=AXIS2_PLACEMENT_3D ( 'NONE', #26318, #5213, #24087 ) ;
#4061=EDGE_LOOP ( 'NONE', ( #30369, #639, #13546, #15509 ) ) ;
#4067=CARTESIAN_POINT ( 'NONE',  ( -5.147494310547430452, 9.551254281546839309, -32.49999999999999289 ) ) ;
#4068=CARTESIAN_POINT ( 'NONE',  ( -7.570916362186215665, 19.14999999453761959, 23.30088464923126423 ) ) ;
#4069=CARTESIAN_POINT ( 'NONE',  ( 18.94512977948575738, 6.424999997268809437, 13.76444248337723408 ) ) ;
#4070=CARTESIAN_POINT ( 'NONE',  ( -27.16883889988624290, 21.17500000273120264, -19.73931689729374028 ) ) ;
#4071=CARTESIAN_POINT ( 'NONE',  ( -26.29305231718578995, 24.70000000546238184, 19.10302069950538595 ) ) ;
#4072=CARTESIAN_POINT ( 'NONE',  ( -32.50000000000000000, 71.89999999999999147, -10.55989012756945478 ) ) ;
#4073=CARTESIAN_POINT ( 'NONE',  ( 0.000000000000000000, 80.00000000000001421, -32.50000000000000000 ) ) ;
#4076=CARTESIAN_POINT ( 'NONE',  ( -33.58253175000000113, 39.37500000273119838, 0.000000000000000000 ) ) ;
#4080=CARTESIAN_POINT ( 'NONE',  ( -23.41746824999999887, 10.12499999726881938, -2.867812753649727150E-15 ) ) ;
#4081=CARTESIAN_POINT ( 'NONE',  ( -2.092463501923844636E-15, 17.50000000000000000, -34.17252228774368916 ) ) ;
#4085=CARTESIAN_POINT ( 'NONE',  ( 10.37757302488624056, 56.52500000273119696, -31.93888565452638417 ) ) ;
#4086=CARTESIAN_POINT ( 'NONE',  ( 33.58253175000000113, 50.47500000273118559, -10.91162601494193574 ) ) ;
#4089=CARTESIAN_POINT ( 'NONE',  ( -33.58253175000000113, 1.125000002731191273, 0.000000000000000000 ) ) ;
#4094=FACE_BOUND ( 'NONE', #92, .T. ) ;
#4096=CARTESIAN_POINT ( 'NONE',  ( -10.04305231718579172, 78.10000000546237686, -30.90933677959248982 ) ) ;
#4099=CARTESIAN_POINT ( 'NONE',  ( 12.13525491562420910, 71.45000000546237118, -8.816778784387098611 ) ) ;
#4100=CARTESIAN_POINT ( 'NONE',  ( 27.16883889988623935, 30.32500000273119412, -19.73931689729374384 ) ) ;
#4101=CARTESIAN_POINT ( 'NONE',  ( -33.58253175000000113, 65.37500000273119838, 0.000000000000000000 ) ) ;
#4107=CARTESIAN_POINT ( 'NONE',  ( 0.000000000000000000, 80.00000000000001421, -30.50000000000000000 ) ) ;
#4108=ORIENTED_EDGE ( 'NONE', *, *, #9396, .T. ) ;
#4112=CARTESIAN_POINT ( 'NONE',  ( 10.04305231718579705, 56.59999999999998010, 30.90933677959248982 ) ) ;
#4113=CARTESIAN_POINT ( 'NONE',  ( 20.75514604977249178, 42.07500000273117990, 28.56700777964553950 ) ) ;
#4114=CARTESIAN_POINT ( 'NONE',  ( 32.50000000000000000, 45.50000000546239676, -3.980102097228898626E-15 ) ) ;
#4115=ADVANCED_FACE ( 'NONE', ( #25533 ), #20043, .T. ) ;
#4117=CARTESIAN_POINT ( 'NONE',  ( 33.58253175000000113, 28.22500000273119269, -10.91162601494193751 ) ) ;
#4118=CARTESIAN_POINT ( 'NONE',  ( 32.50000000000000000, 31.50000000546238255, -3.980102097228898626E-15 ) ) ;
#4119=CARTESIAN_POINT ( 'NONE',  ( -20.75514604977248823, 55.07500000273117990, -28.56700777964554305 ) ) ;
#4122=CARTESIAN_POINT ( 'NONE',  ( 10.04305231718578817, 33.39999999999998437, -30.90933677959249337 ) ) ;
#4124=CARTESIAN_POINT ( 'NONE',  ( -33.58253175000000113, 77.12500000273119838, 0.000000000000000000 ) ) ;
#4126=DIRECTION ( 'NONE',  ( -0.000000000000000000, 1.000000000000000000, -0.000000000000000000 ) ) ;
#4127=CARTESIAN_POINT ( 'NONE',  ( 20.75514604977248467, 68.67500000273119554, -28.56700777964554305 ) ) ;
#4129=ADVANCED_FACE ( 'NONE', ( #33586 ), #12134, .T. ) ;
#4131=CARTESIAN_POINT ( 'NONE',  ( 24.50000000000000000, 3.749999994537622783, 0.000000000000000000 ) ) ;
#4142=AXIS2_PLACEMENT_3D ( 'NONE', #5531, #31269, #10853 ) ;
#4145=DIRECTION ( 'NONE',  ( -0.000000000000000000, 1.000000000000000000, -0.000000000000000000 ) ) ;
#4146=DIRECTION ( 'NONE',  ( 0.000000000000000000, 0.000000000000000000, -1.000000000000000000 ) ) ;
#4149=ORIENTED_EDGE ( 'NONE', *, *, #20550, .T. ) ;
#4153=ORIENTED_EDGE ( 'NONE', *, *, #30398, .F. ) ;
#4154=( BOUNDED_CURVE ( )  B_SPLINE_CURVE ( 2, ( #30771, #32823, #17576, #20322, #17927, #4522, #28035, #14997, #9314, #17232, #4183, #15173, #33347 ),
 .UNSPECIFIED., .F., .T. ) 
 B_SPLINE_CURVE_WITH_KNOTS ( ( 3, 2, 2, 2, 2, 2, 3 ),
 ( 0.9807692307692307265, 0.9820512820512820040, 0.9846153846153846700, 0.9871794871794872250, 0.9897435897435897800, 0.9923076923076923350, 0.9935897435897436125 ),
 .UNSPECIFIED. ) 
 CURVE ( )  GEOMETRIC_REPRESENTATION_ITEM ( )  RATIONAL_B_SPLINE_CURVE ( ( 0.9755282581475768211, 0.9755282581475768211, 1.000000000000000000, 0.9510565162951535312, 1.000000000000000000, 0.9510565162951535312, 1.000000000000000000, 0.9510565162951535312, 1.000000000000000000, 0.9510565162951535312, 1.000000000000000000, 0.9755282581475768211, 0.9755282581475768211 ) ) 
 REPRESENTATION_ITEM ( '' )  );
#4155=CARTESIAN_POINT ( 'NONE',  ( -20.08610463437157989, 74.20000000546238539, -27.64615127144129758 ) ) ;
#4156=CARTESIAN_POINT ( 'NONE',  ( -27.16883889988624290, 46.92500000273119554, -19.73931689729374028 ) ) ;
#4157=FACE_OUTER_BOUND ( 'NONE', #5601, .T. ) ;
#4158=CARTESIAN_POINT ( 'NONE',  ( -10.04305231718578462, 48.39999999999999858, 30.90933677959249337 ) ) ;
#4159=CARTESIAN_POINT ( 'NONE',  ( 20.08610463437158344, 11.20000000546238184, 27.64615127144129403 ) ) ;
#4160=CARTESIAN_POINT ( 'NONE',  ( -26.29305231718579350, 7.800000000000001599, -19.10302069950537884 ) ) ;
#4161=CARTESIAN_POINT ( 'NONE',  ( 23.41746824999999887, 17.12499999726882649, 0.000000000000000000 ) ) ;
#4162=CARTESIAN_POINT ( 'NONE',  ( 26.29305231718579350, 50.80000000000001137, 19.10302069950537529 ) ) ;
#4163=CARTESIAN_POINT ( 'NONE',  ( 6.001560367445586717E-15, 1.500000000000005995, 24.50000000000000000 ) ) ;
#4164=CARTESIAN_POINT ( 'NONE',  ( 33.58253175000000113, 20.47500000273120335, -10.91162601494193751 ) ) ;
#4165=CIRCLE ( 'NONE', #8553, 26.50000000000000355 ) ;
#4166=CARTESIAN_POINT ( 'NONE',  ( 12.13525491562420910, 77.19999999999998863, -8.816778784387098611 ) ) ;
#4168=CARTESIAN_POINT ( 'NONE',  ( 13.91746824999999887, 73.87500000273116996, -1.704398294459741270E-15 ) ) ;
#4179=CARTESIAN_POINT ( 'NONE',  ( -10.37757302488623701, 7.775000002731180970, 31.93888565452638417 ) ) ;
#4182=ADVANCED_FACE ( 'NONE', ( #10087 ), #21553, .F. ) ;
#4183=CARTESIAN_POINT ( 'NONE',  ( 10.04305231718579705, 2.599999999999991207, 30.90933677959248982 ) ) ;
#4185=CARTESIAN_POINT ( 'NONE',  ( -33.58253175000000113, 53.22500000273118559, 10.91162601494193929 ) ) ;
#4186=EDGE_CURVE ( 'NONE', #726, #12058, #12315, .T. ) ;
#4188=VERTEX_POINT ( 'NONE', #2664 ) ;
#4190=CARTESIAN_POINT ( 'NONE',  ( 0.000000000000000000, 80.00000000000001421, -32.50000000000000000 ) ) ;
#4191=CARTESIAN_POINT ( 'NONE',  ( 23.41746825000000243, 12.52499999726880375, 7.608796670333735079 ) ) ;
#4193=ORIENTED_EDGE ( 'NONE', *, *, #24339, .T. ) ;
#4195=VECTOR ( 'NONE', #28780, 1000.000000000000000 ) ;
#4197=VERTEX_POINT ( 'NONE', #13474 ) ;
#4199=CARTESIAN_POINT ( 'NONE',  ( -27.16883889988623935, 63.57500000273119412, 19.73931689729374739 ) ) ;
#4200=CARTESIAN_POINT ( 'NONE',  ( 27.16883889988624290, 69.92500000273119554, 19.73931689729373673 ) ) ;
#4202=CARTESIAN_POINT ( 'NONE',  ( -24.50000000000001066, 11.09999999999999964, 7.960532557706201828 ) ) ;
#4203=CARTESIAN_POINT ( 'NONE',  ( 10.37757302488624767, 5.975000002731184701, 31.93888565452638417 ) ) ;
#4204=CARTESIAN_POINT ( 'NONE',  ( 20.75514604977248467, 12.42500000273119554, -28.56700777964554305 ) ) ;
#4205=CARTESIAN_POINT ( 'NONE',  ( -8.960552108402744065E-16, 72.37500000273118417, -14.63369212191046209 ) ) ;
#4207=CARTESIAN_POINT ( 'NONE',  ( 12.13525491562420910, 73.19999999999998863, -8.816778784387098611 ) ) ;
#4209=CARTESIAN_POINT ( 'NONE',  ( 20.08610463437158344, 19.20000000546235697, 27.64615127144129403 ) ) ;
#4210=CARTESIAN_POINT ( 'NONE',  ( 10.04305231718579705, 22.60000000000000853, 30.90933677959248982 ) ) ;
#4212=CARTESIAN_POINT ( 'NONE',  ( 4.635254915624212657, 78.85000000546239107, 14.26584774442730286 ) ) ;
#4214=CARTESIAN_POINT ( 'NONE',  ( -10.37757302488624411, 40.72500000273118559, -31.93888565452638417 ) ) ;
#4217=CARTESIAN_POINT ( 'NONE',  ( 10.37757302488624767, 27.97500000273117493, 31.93888565452638417 ) ) ;
#4218=CARTESIAN_POINT ( 'NONE',  ( -19.82091636218621034, 16.54999999453762882, -14.40073868116559552 ) ) ;
#4219=CARTESIAN_POINT ( 'NONE',  ( -7.570916362186210335, 14.34999999453762065, -23.30088464923126779 ) ) ;
#4220=ADVANCED_FACE ( 'NONE', ( #16054 ), #3001, .T. ) ;
#4223=CARTESIAN_POINT ( 'NONE',  ( 18.94512977948576093, 8.824999997268822227, -13.76444248337722875 ) ) ;
#4225=EDGE_CURVE ( 'NONE', #31336, #21272, #22844, .T. ) ;
#4228=CARTESIAN_POINT ( 'NONE',  ( 33.58253175000000823, 12.02500000273117742, 10.91162601494192685 ) ) ;
#4229=CARTESIAN_POINT ( 'NONE',  ( -18.94512977948575738, 11.92499999726881477, -13.76444248337723231 ) ) ;
#4234=VERTEX_POINT ( 'NONE', #13124 ) ;
#4238=CARTESIAN_POINT ( 'NONE',  ( 24.50000000000000355, 15.64999999453761426, 7.960532557706212486 ) ) ;
#4239=CARTESIAN_POINT ( 'NONE',  ( -23.41746824999999887, 13.62499999726882116, -2.867812753649727150E-15 ) ) ;
#4240=CARTESIAN_POINT ( 'NONE',  ( 10.37757302488624767, 19.97500000273119625, 31.93888565452638417 ) ) ;
#4241=CARTESIAN_POINT ( 'NONE',  ( -32.50000000000000000, 22.40000000546237402, -10.55989012756945478 ) ) ;
#4242=CARTESIAN_POINT ( 'NONE',  ( -2.092463501923844636E-15, 69.49999999999997158, -34.17252228774368916 ) ) ;
#4243=DIRECTION ( 'NONE',  ( 0.000000000000000000, 0.000000000000000000, -1.000000000000000000 ) ) ;
#4246=CARTESIAN_POINT ( 'NONE',  ( -20.75514604977248823, 35.07500000273120833, -28.56700777964554305 ) ) ;
#4249=CARTESIAN_POINT ( 'NONE',  ( -7.236395654485763274, 12.52499999726880375, 22.27133577429736633 ) ) ;
#4250=CARTESIAN_POINT ( 'NONE',  ( 10.04305231718578817, 13.39999999999999503, -30.90933677959249337 ) ) ;
#4253=CARTESIAN_POINT ( 'NONE',  ( -27.16883889988624290, 54.92500000273120264, -19.73931689729374028 ) ) ;
#4254=CARTESIAN_POINT ( 'NONE',  ( 20.75514604977248467, 48.67500000273118133, -28.56700777964554305 ) ) ;
#4257=CARTESIAN_POINT ( 'NONE',  ( 3.980102097228898626E-15, 80.00000000000001421, 32.50000000000000000 ) ) ;
#4258=CARTESIAN_POINT ( 'NONE',  ( -33.58253175000000113, 1.225000002731198467, 10.91162601494193929 ) ) ;
#4263=CARTESIAN_POINT ( 'NONE',  ( 26.29305231718578995, 67.19999999999998863, -19.10302069950538240 ) ) ;
#4265=DIRECTION ( 'NONE',  ( -0.000000000000000000, -1.000000000000000000, -0.000000000000000000 ) ) ;
#4268=CARTESIAN_POINT ( 'NONE',  ( 32.50000000000000000, 35.10000000000000142, -10.55989012756945833 ) ) ;
#4269=CARTESIAN_POINT ( 'NONE',  ( 6.486482029760648627E-15, 31.62500000273119838, 35.31076352940722529 ) ) ;
#4270=CARTESIAN_POINT ( 'NONE',  ( 10.37757302488624767, 63.97500000273120691, 31.93888565452638417 ) ) ;
#4272=ORIENTED_EDGE ( 'NONE', *, *, #423, .T. ) ;
#4275=CARTESIAN_POINT ( 'NONE',  ( -2.165007332552593587E-13, 52.50000000000000711, 32.50000000000000000 ) ) ;
#4282=CARTESIAN_POINT ( 'NONE',  ( -20.75514604977248112, 43.67500000273119554, 28.56700777964554661 ) ) ;
#4283=CARTESIAN_POINT ( 'NONE',  ( 32.50000000000000000, 45.60000000546236265, -10.55989012756945833 ) ) ;
#4285=CARTESIAN_POINT ( 'NONE',  ( -33.58253175000000113, 31.22500000273118559, 10.91162601494193929 ) ) ;
#4286=CARTESIAN_POINT ( 'NONE',  ( 24.50000000000000000, 0.8749999972688105032, 0.000000000000000000 ) ) ;
#4287=CARTESIAN_POINT ( 'NONE',  ( -33.58253175000000113, 55.37500000273118417, 0.000000000000000000 ) ) ;
#4289=CARTESIAN_POINT ( 'NONE',  ( -20.08610463437156923, 32.29999999999999716, 27.64615127144130113 ) ) ;
#4291=CARTESIAN_POINT ( 'NONE',  ( -20.75514604977248112, 73.42500000273118133, 28.56700777964554661 ) ) ;
#4294=CARTESIAN_POINT ( 'NONE',  ( -27.16883889988623935, 69.57500000273120122, 19.73931689729374739 ) ) ;
#4296=VERTEX_POINT ( 'NONE', #18291 ) ;
#4297=CARTESIAN_POINT ( 'NONE',  ( -33.58253175000000113, 21.12500000273118062, 0.000000000000000000 ) ) ;
#4298=CARTESIAN_POINT ( 'NONE',  ( -24.50000000000000355, 12.64999999453762136, -7.960532557706207157 ) ) ;
#4300=CARTESIAN_POINT ( 'NONE',  ( 3.980102097228898626E-15, 80.00000000000001421, 32.50000000000000000 ) ) ;
#4311=CARTESIAN_POINT ( 'NONE',  ( 6.277390505771533514E-15, 75.00000000546238255, 34.17252228774368916 ) ) ;
#4314=CARTESIAN_POINT ( 'NONE',  ( -1.089172066684569321E-14, 78.50000000000000000, 15.00000000000000000 ) ) ;
#4316=CARTESIAN_POINT ( 'NONE',  ( -10.37757302488624411, 76.97500000273119269, -31.93888565452638417 ) ) ;
#4321=CARTESIAN_POINT ( 'NONE',  ( 6.277390505771533514E-15, 63.00000000546238255, 34.17252228774368916 ) ) ;
#4323=CARTESIAN_POINT ( 'NONE',  ( -5.147494310547430452, 55.55125428154683220, -32.49999999999999289 ) ) ;
#4324=CARTESIAN_POINT ( 'NONE',  ( 6.486482029760649416E-15, 51.62500000273120548, 35.31076352940723240 ) ) ;
#4325=CARTESIAN_POINT ( 'NONE',  ( 14.47279130897151589, 16.32499999726879736, 19.92008829642072953 ) ) ;
#4327=CARTESIAN_POINT ( 'NONE',  ( -26.29305231718579350, 4.300000005462378816, -19.10302069950537884 ) ) ;
#4328=ADVANCED_FACE ( 'NONE', ( #5232 ), #9914, .F. ) ;
#4331=CARTESIAN_POINT ( 'NONE',  ( 10.04305231718578817, 51.39999999999999858, -30.90933677959249337 ) ) ;
#4332=CARTESIAN_POINT ( 'NONE',  ( 19.82091636218621389, 2.200000000000007283, -14.40073868116559197 ) ) ;
#4333=CARTESIAN_POINT ( 'NONE',  ( -20.75514604977248112, 15.67500000273117600, 28.56700777964554661 ) ) ;
#4334=DIRECTION ( 'NONE',  ( -0.000000000000000000, 1.000000000000000000, -0.000000000000000000 ) ) ;
#4336=CARTESIAN_POINT ( 'NONE',  ( 11.25946833292375793, 75.67500000273119554, 8.180482586598731842 ) ) ;
#4337=CARTESIAN_POINT ( 'NONE',  ( 7.313012447739250820E-14, 13.24999999453762456, 24.50000000000000000 ) ) ;
#4341=CARTESIAN_POINT ( 'NONE',  ( -8.601468415847515203, 71.17500000273115290, 11.83890561707634959 ) ) ;
#4346=CARTESIAN_POINT ( 'NONE',  ( -33.58253175000000113, 5.375000002731167292, 0.000000000000000000 ) ) ;
#4350=CARTESIAN_POINT ( 'NONE',  ( -4.300734207923759378, 72.97500000273119269, -13.23629886949340495 ) ) ;
#4352=CARTESIAN_POINT ( 'NONE',  ( -33.58253175000000113, 43.22500000273118559, 10.91162601494193929 ) ) ;
#4358=( BOUNDED_CURVE ( )  B_SPLINE_CURVE ( 2, ( #8438, #27307, #8609, #14105, #9108, #8771, #19254, #24562, #24727, #16850, #27137, #6372, #1035 ),
 .UNSPECIFIED., .F., .T. ) 
 B_SPLINE_CURVE_WITH_KNOTS ( ( 3, 2, 2, 2, 2, 2, 3 ),
 ( 0.6500000000000000222, 0.6600000000000000311, 0.6800000000000000488, 0.6999999999999999556, 0.7199999999999999734, 0.7399999999999999911, 0.7500000000000000000 ),
 .UNSPECIFIED. ) 
 CURVE ( )  GEOMETRIC_REPRESENTATION_ITEM ( )  RATIONAL_B_SPLINE_CURVE ( ( 0.9755282581475768211, 0.9755282581475768211, 1.000000000000000000, 0.9510565162951535312, 1.000000000000000000, 0.9510565162951535312, 1.000000000000000000, 0.9510565162951535312, 1.000000000000000000, 0.9510565162951535312, 1.000000000000000000, 0.9755282581475768211, 0.9755282581475768211 ) ) 
 REPRESENTATION_ITEM ( '' )  );
#4360=CARTESIAN_POINT ( 'NONE',  ( -18.94512977948576093, 11.82499999726882578, 13.76444248337722698 ) ) ;
#4366=CARTESIAN_POINT ( 'NONE',  ( 0.000000000000000000, 80.00000000000001421, 0.000000000000000000 ) ) ;
#4367=CARTESIAN_POINT ( 'NONE',  ( -27.16883889988623935, 69.32500000273117280, 19.73931689729374739 ) ) ;
#4369=CARTESIAN_POINT ( 'NONE',  ( -24.50000000000000000, 11.00000000000001066, -3.000384657911015469E-15 ) ) ;
#4370=CARTESIAN_POINT ( 'NONE',  ( -20.75514604977248823, 3.075000002731198112, -28.56700777964554305 ) ) ;
#4371=EDGE_CURVE ( 'NONE', #23252, #29590, #22967, .T. ) ;
#4372=CARTESIAN_POINT ( 'NONE',  ( 10.37757302488624056, 10.52500000273118275, -31.93888565452638417 ) ) ;
#4375=CARTESIAN_POINT ( 'NONE',  ( 2.897257156509938333E-15, 74.50000000000000000, 15.77193336357400710 ) ) ;
#4377=CARTESIAN_POINT ( 'NONE',  ( -1.778240108872766143E-15, 20.00000000546237544, -32.49999999999999289 ) ) ;
#4379=CARTESIAN_POINT ( 'NONE',  ( -9.270509831248425314, 79.95000000546235697, -12.75976212528059861 ) ) ;
#4381=CARTESIAN_POINT ( 'NONE',  ( -33.58253175000000113, 37.22500000273119980, 10.91162601494193929 ) ) ;
#4384=CARTESIAN_POINT ( 'NONE',  ( -10.37757302488624411, 24.97500000273117493, -31.93888565452638417 ) ) ;
#4385=CARTESIAN_POINT ( 'NONE',  ( 20.08610463437158344, 40.69999999999999574, 27.64615127144129403 ) ) ;
#4387=CARTESIAN_POINT ( 'NONE',  ( -15.14183272437242778, 15.04999999453763238, 20.84094480462497856 ) ) ;
#4388=CARTESIAN_POINT ( 'NONE',  ( 10.04305231718579705, 32.59999999999998721, 30.90933677959248982 ) ) ;
#4390=CARTESIAN_POINT ( 'NONE',  ( -23.41746825000000243, 11.72499999726882969, 7.608796670333725309 ) ) ;
#4396=CARTESIAN_POINT ( 'NONE',  ( 10.37757302488624767, 15.72500000273119269, 31.93888565452638417 ) ) ;
#4397=CARTESIAN_POINT ( 'NONE',  ( -18.94512977948576093, 10.32499999726882400, 13.76444248337722698 ) ) ;
#4406=CARTESIAN_POINT ( 'NONE',  ( 1.507698388325705758E-15, 1.624999997268798735, -24.62258325217400312 ) ) ;
#4407=CARTESIAN_POINT ( 'NONE',  ( -4.523095164977116484E-15, 12.12499999726881406, 24.62258325217400312 ) ) ;
#4408=CARTESIAN_POINT ( 'NONE',  ( 20.75514604977248467, 22.67500000273119198, -28.56700777964554305 ) ) ;
#4409=CARTESIAN_POINT ( 'NONE',  ( 26.29305231718578995, 27.70000000546238184, -19.10302069950538240 ) ) ;
#4411=CARTESIAN_POINT ( 'NONE',  ( 32.50000000000000000, 67.10000000000000853, -10.55989012756945833 ) ) ;
#4412=CARTESIAN_POINT ( 'NONE',  ( 23.41746824999999887, 0.6249999972688102812, 0.000000000000000000 ) ) ;
#4415=CARTESIAN_POINT ( 'NONE',  ( 33.58253175000000113, 34.47500000273119980, -10.91162601494193751 ) ) ;
#4416=CARTESIAN_POINT ( 'NONE',  ( -4.300734207923755825, 79.77500000273118985, 13.23629886949340673 ) ) ;
#4419=CARTESIAN_POINT ( 'NONE',  ( 23.41746825000000243, 19.02499999726880375, 7.608796670333735079 ) ) ;
#4420=CARTESIAN_POINT ( 'NONE',  ( 10.04305231718578817, 9.399999999999991473, -30.90933677959249337 ) ) ;
#4423=CARTESIAN_POINT ( 'NONE',  ( -20.75514604977248823, 58.82500000273117990, -28.56700777964554305 ) ) ;
#4425=CARTESIAN_POINT ( 'NONE',  ( 27.16883889988624290, 42.17500000273119554, 19.73931689729373673 ) ) ;
#4428=CARTESIAN_POINT ( 'NONE',  ( 33.58253175000000823, 2.025000002731202287, 10.91162601494192863 ) ) ;
#4432=CARTESIAN_POINT ( 'NONE',  ( 32.50000000000000711, 66.90000000000001990, 10.55989012756945122 ) ) ;
#4434=DIRECTION ( 'NONE',  ( -0.000000000000000000, -1.000000000000000000, -0.000000000000000000 ) ) ;
#4437=CARTESIAN_POINT ( 'NONE',  ( 2.445080149700053643E-15, 70.75000000546236834, 15.00000000000000000 ) ) ;
#4438=CARTESIAN_POINT ( 'NONE',  ( -33.58253175000000113, 33.02500000273118275, -10.91162601494193041 ) ) ;
#4444=ORIENTED_EDGE ( 'NONE', *, *, #1940, .T. ) ;
#4450=CARTESIAN_POINT ( 'NONE',  ( 33.58253175000000113, 38.37500000273119838, -4.112674001490185761E-15 ) ) ;
#4451=AXIS2_PLACEMENT_3D ( 'NONE', #8093, #11012, #21482 ) ;
#4452=CARTESIAN_POINT ( 'NONE',  ( 32.50000000000000000, 43.60000000546237686, -10.55989012756945833 ) ) ;
#4454=CARTESIAN_POINT ( 'NONE',  ( -33.58253175000000113, 29.02500000273119340, -10.91162601494193218 ) ) ;
#4455=CARTESIAN_POINT ( 'NONE',  ( -5.147494310547430452, 23.55125428154684286, -32.49999999999999289 ) ) ;
#4456=CARTESIAN_POINT ( 'NONE',  ( 27.16883889988623935, 56.57500000273118701, -19.73931689729374384 ) ) ;
#4457=EDGE_CURVE ( 'NONE', #21929, #17393, #8466, .T. ) ;
#4460=CARTESIAN_POINT ( 'NONE',  ( 20.08610463437157279, 33.29999999999999716, -27.64615127144129758 ) ) ;
#4462=CARTESIAN_POINT ( 'NONE',  ( 20.75514604977248467, 74.42500000273119554, -28.56700777964554305 ) ) ;
#4465=VECTOR ( 'NONE', #17075, 1000.000000000000000 ) ;
#4467=CARTESIAN_POINT ( 'NONE',  ( -10.37757302488623701, 65.77500000273117564, 31.93888565452638417 ) ) ;
#4470=CARTESIAN_POINT ( 'NONE',  ( -2.162160676586881955E-15, 20.62500000273119483, -35.31076352940723240 ) ) ;
#4471=CARTESIAN_POINT ( 'NONE',  ( -24.50000000000000000, 8.749999994537628112, -3.000384657911015469E-15 ) ) ;
#4473=CARTESIAN_POINT ( 'NONE',  ( -5.147494310547430452, 25.55125428154685352, -32.49999999999999289 ) ) ;
#4484=CARTESIAN_POINT ( 'NONE',  ( 32.50000000000000711, 77.40000000546240244, 10.55989012756945122 ) ) ;
#4488=ORIENTED_EDGE ( 'NONE', *, *, #25226, .T. ) ;
#4489=CARTESIAN_POINT ( 'NONE',  ( 20.75514604977248467, 74.67500000273118133, -28.56700777964554305 ) ) ;
#4492=CARTESIAN_POINT ( 'NONE',  ( -20.08610463437156923, 62.80000000546237970, 27.64615127144130113 ) ) ;
#4493=VERTEX_POINT ( 'NONE', #11814 ) ;
#4494=CARTESIAN_POINT ( 'NONE',  ( -32.50000000000000000, 56.10000000000000142, 10.55989012756946366 ) ) ;
#4495=CARTESIAN_POINT ( 'NONE',  ( -27.16883889988624290, 48.92500000273120264, -19.73931689729374028 ) ) ;
#4496=CARTESIAN_POINT ( 'NONE',  ( 23.41746825000000243, 16.52499999726882152, 7.608796670333735079 ) ) ;
#4497=CARTESIAN_POINT ( 'NONE',  ( 26.29305231718578995, 7.700000005462392494, -19.10302069950538240 ) ) ;
#4499=DIRECTION ( 'NONE',  ( -0.000000000000000000, -1.000000000000000000, -0.000000000000000000 ) ) ;
#4500=CARTESIAN_POINT ( 'NONE',  ( 26.29305231718579350, 54.80000000000001847, 19.10302069950537529 ) ) ;
#4502=CARTESIAN_POINT ( 'NONE',  ( 20.75514604977249178, 20.07500000273118346, 28.56700777964553950 ) ) ;
#4504=LINE ( 'NONE', #9477, #18959 ) ;
#4506=CARTESIAN_POINT ( 'NONE',  ( -8.601468415847518756, 81.07500000273120122, -11.83890561707634781 ) ) ;
#4512=CYLINDRICAL_SURFACE ( 'NONE', #20590, 32.50000000000000000 ) ;
#4522=CARTESIAN_POINT ( 'NONE',  ( 32.50000000000000000, 3.099999999999989431, -10.55989012756945833 ) ) ;
#4524=CARTESIAN_POINT ( 'NONE',  ( 10.37757302488624056, 42.52500000273118275, -31.93888565452638417 ) ) ;
#4527=CARTESIAN_POINT ( 'NONE',  ( 32.50000000000000000, 21.60000000546237331, -10.55989012756945833 ) ) ;
#4528=ORIENTED_EDGE ( 'NONE', *, *, #4748, .T. ) ;
#4530=CARTESIAN_POINT ( 'NONE',  ( 32.50000000000000711, 42.90000000000001279, 10.55989012756945122 ) ) ;
#4532=CARTESIAN_POINT ( 'NONE',  ( -7.236395654485763274, 12.02499999726880375, 22.27133577429736633 ) ) ;
#4537=CARTESIAN_POINT ( 'NONE',  ( 19.82091636218621034, 5.799999999999999822, 14.40073868116559730 ) ) ;
#4540=CARTESIAN_POINT ( 'NONE',  ( 33.58253175000000113, 70.12500000273119838, -4.112674001490185761E-15 ) ) ;
#4542=CARTESIAN_POINT ( 'NONE',  ( 1.577395562988744260E-15, 10.49999999999998757, -25.76082449383753925 ) ) ;
#4543=CARTESIAN_POINT ( 'NONE',  ( 18.94512977948575738, 2.924999997268806773, 13.76444248337723408 ) ) ;
#4544=CARTESIAN_POINT ( 'NONE',  ( -33.58253175000000113, 7.225000002731182924, 10.91162601494193929 ) ) ;
#4546=CARTESIAN_POINT ( 'NONE',  ( 15.00000000000000355, 74.90000000000000568, 4.873795443493592394 ) ) ;
#4549=CARTESIAN_POINT ( 'NONE',  ( -15.00000000000000000, 74.15000000546237402, -4.873795443493594171 ) ) ;
#4551=CARTESIAN_POINT ( 'NONE',  ( 2.897257156509938333E-15, 78.75000000546236834, 15.77193336357400710 ) ) ;
#4553=CARTESIAN_POINT ( 'NONE',  ( -10.37757302488624411, 30.72500000273117848, -31.93888565452638417 ) ) ;
#4554=DIRECTION ( 'NONE',  ( -0.000000000000000000, -1.000000000000000000, -0.000000000000000000 ) ) ;
#4556=CARTESIAN_POINT ( 'NONE',  ( 10.37757302488624767, 19.97500000273119625, 31.93888565452638417 ) ) ;
#4557=CARTESIAN_POINT ( 'NONE',  ( 5.779280353836490358E-15, 68.49999999999998579, 32.49999999999999289 ) ) ;
#4558=VECTOR ( 'NONE', #9899, 1000.000000000000000 ) ;
#4560=CARTESIAN_POINT ( 'NONE',  ( -8.446640517145639571E-15, 78.49999999999998579, 32.49999999999999289 ) ) ;
#4561=( BOUNDED_CURVE ( )  B_SPLINE_CURVE ( 2, ( #12992, #31844, #15916, #20893, #15747, #15400, #270, #26202, #31342, #26372, #18662, #18493, #2523 ),
 .UNSPECIFIED., .F., .T. ) 
 B_SPLINE_CURVE_WITH_KNOTS ( ( 3, 2, 2, 2, 2, 2, 3 ),
 ( 0.09615384615384615918, 0.09743589743589743668, 0.1000000000000000056, 0.1025641025641025605, 0.1051282051282051294, 0.1076923076923076983, 0.1089743589743589758 ),
 .UNSPECIFIED. ) 
 CURVE ( )  GEOMETRIC_REPRESENTATION_ITEM ( )  RATIONAL_B_SPLINE_CURVE ( ( 0.9755282581475767101, 0.9755282581475768211, 1.000000000000000000, 0.9510565162951535312, 1.000000000000000000, 0.9510565162951535312, 1.000000000000000000, 0.9510565162951535312, 1.000000000000000000, 0.9510565162951535312, 1.000000000000000000, 0.9755282581475768211, 0.9755282581475768211 ) ) 
 REPRESENTATION_ITEM ( '' )  );
#4563=CARTESIAN_POINT ( 'NONE',  ( -18.94512977948576093, 11.82499999726882578, 13.76444248337722698 ) ) ;
#4564=CARTESIAN_POINT ( 'NONE',  ( -27.16883889988623935, 61.32500000273119412, 19.73931689729374739 ) ) ;
#4568=CARTESIAN_POINT ( 'NONE',  ( 20.75514604977249178, 15.82500000273117102, 28.56700777964553950 ) ) ;
#4569=CARTESIAN_POINT ( 'NONE',  ( 14.47279130897151767, 13.42499999726880411, -19.92008829642072598 ) ) ;
#4571=ORIENTED_EDGE ( 'NONE', *, *, #31652, .F. ) ;
#4578=CARTESIAN_POINT ( 'NONE',  ( -32.50000000000000000, 72.50000000546236834, 0.000000000000000000 ) ) ;
#4579=CARTESIAN_POINT ( 'NONE',  ( -7.236395654485763274, 6.524999997268826846, 22.27133577429736633 ) ) ;
#4580=AXIS2_PLACEMENT_3D ( 'NONE', #13019, #31369, #5120 ) ;
#4581=CARTESIAN_POINT ( 'NONE',  ( -7.236395654485763274, 12.02499999726880375, 22.27133577429736633 ) ) ;
#4582=CARTESIAN_POINT ( 'NONE',  ( -27.16883889988624290, 17.17500000273119909, -19.73931689729374028 ) ) ;
#4583=CARTESIAN_POINT ( 'NONE',  ( 32.50000000000000000, 21.50000000546237189, -3.980102097228898626E-15 ) ) ;
#4584=CARTESIAN_POINT ( 'NONE',  ( 26.29305231718579350, 68.79999999999999716, 19.10302069950537529 ) ) ;
#4588=CARTESIAN_POINT ( 'NONE',  ( -27.16883889988623935, 27.57500000273119412, 19.73931689729374739 ) ) ;
#4591=CARTESIAN_POINT ( 'NONE',  ( -23.41746825000000243, 18.02499999726880731, -7.608796670333730638 ) ) ;
#4592=CARTESIAN_POINT ( 'NONE',  ( 32.50000000000000000, 7.100000000000007638, -10.55989012756945833 ) ) ;
#4595=CARTESIAN_POINT ( 'NONE',  ( 33.58253175000000113, 54.22500000273117848, -10.91162601494193751 ) ) ;
#4597=CARTESIAN_POINT ( 'NONE',  ( 20.75514604977249178, 44.07500000273117990, 28.56700777964553950 ) ) ;
#4598=FACE_OUTER_BOUND ( 'NONE', #15219, .T. ) ;
#4599=LINE ( 'NONE', #4257, #29797 ) ;
#4604=CYLINDRICAL_SURFACE ( 'NONE', #9465, 26.50000000000000355 ) ;
#4610=CARTESIAN_POINT ( 'NONE',  ( -10.04305231718578462, 60.90000000546235981, 30.90933677959249337 ) ) ;
#4611=CARTESIAN_POINT ( 'NONE',  ( 10.37757302488624056, 30.52500000273117209, -31.93888565452638417 ) ) ;
#4613=EDGE_CURVE ( 'NONE', #9319, #7495, #22494, .T. ) ;
#4617=CARTESIAN_POINT ( 'NONE',  ( -1.778240108872766143E-15, 31.49999999999998579, -32.49999999999999289 ) ) ;
#4624=CARTESIAN_POINT ( 'NONE',  ( 20.75514604977249178, 38.07500000273116569, 28.56700777964553950 ) ) ;
#4625=CARTESIAN_POINT ( 'NONE',  ( 26.29305231718579350, 41.30000000546238681, 19.10302069950537529 ) ) ;
#4627=CARTESIAN_POINT ( 'NONE',  ( -20.75514604977248823, 20.82500000273119412, -28.56700777964554305 ) ) ;
#4629=CARTESIAN_POINT ( 'NONE',  ( -10.37757302488624411, 52.97500000273119980, -31.93888565452638417 ) ) ;
#4632=CARTESIAN_POINT ( 'NONE',  ( -20.08610463437156923, 28.30000000000000782, 27.64615127144130113 ) ) ;
#4634=CARTESIAN_POINT ( 'NONE',  ( 27.16883889988623935, 76.32500000273118701, -19.73931689729374384 ) ) ;
#4637=CARTESIAN_POINT ( 'NONE',  ( -20.75514604977248112, 61.67500000273117422, 28.56700777964554661 ) ) ;
#4640=CARTESIAN_POINT ( 'NONE',  ( -10.37757302488624411, 16.72500000273119269, -31.93888565452638417 ) ) ;
#4641=CARTESIAN_POINT ( 'NONE',  ( 19.82091636218621389, 7.949999994537631842, -14.40073868116559197 ) ) ;
#4643=CARTESIAN_POINT ( 'NONE',  ( 19.82091636218621034, 7.549999994537620829, 14.40073868116559730 ) ) ;
#4648=CARTESIAN_POINT ( 'NONE',  ( -1.778240108872766143E-15, 51.50000000000000711, -32.49999999999999289 ) ) ;
#4651=EDGE_CURVE ( 'NONE', #24994, #33572, #16797, .T. ) ;
#4653=CARTESIAN_POINT ( 'NONE',  ( 0.000000000000000000, 82.00000000000001421, 0.000000000000000000 ) ) ;
#4655=CARTESIAN_POINT ( 'NONE',  ( -23.41746825000000598, 2.224999997268808816, 7.608796670333726198 ) ) ;
#4656=CARTESIAN_POINT ( 'NONE',  ( 10.04305231718579705, 77.10000000546237686, 30.90933677959248982 ) ) ;
#4660=ORIENTED_EDGE ( 'NONE', *, *, #11534, .T. ) ;
#4661=CARTESIAN_POINT ( 'NONE',  ( 33.58253175000000113, 74.37500000273116996, -4.112674001490185761E-15 ) ) ;
#4664=CARTESIAN_POINT ( 'NONE',  ( -32.50000000000000000, 64.50000000546238255, 0.000000000000000000 ) ) ;
#4667=CARTESIAN_POINT ( 'NONE',  ( 33.58253175000000113, 46.22500000273119269, -10.91162601494193751 ) ) ;
#4668=CARTESIAN_POINT ( 'NONE',  ( 18.94512977948576093, 16.82499999726880091, -13.76444248337722875 ) ) ;
#4669=CARTESIAN_POINT ( 'NONE',  ( 10.04305231718578817, 5.900000005462368691, -30.90933677959249337 ) ) ;
#4670=DIRECTION ( 'NONE',  ( 0.000000000000000000, 0.000000000000000000, 1.000000000000000000 ) ) ;
#4671=DIRECTION ( 'NONE',  ( -0.000000000000000000, -1.000000000000000000, -0.000000000000000000 ) ) ;
#4672=VECTOR ( 'NONE', #28262, 1000.000000000000000 ) ;
#4673=CARTESIAN_POINT ( 'NONE',  ( -10.04305231718579172, 49.60000000000000853, -30.90933677959248982 ) ) ;
#4674=CARTESIAN_POINT ( 'NONE',  ( 2.067204126564591252E-14, 2.500000000000004885, -24.50000000000000000 ) ) ;
#4675=CARTESIAN_POINT ( 'NONE',  ( -20.75514604977248112, 17.67500000273117422, 28.56700777964554661 ) ) ;
#4676=CARTESIAN_POINT ( 'NONE',  ( 7.570916362186213000, 0.4000000000000114575, -23.30088464923126423 ) ) ;
#4678=CARTESIAN_POINT ( 'NONE',  ( -4.300734207923755825, 75.77500000273118985, 13.23629886949340673 ) ) ;
#4693=CARTESIAN_POINT ( 'NONE',  ( 5.147494310547434893, 68.55125428154684641, 32.49999999999999289 ) ) ;
#4695=CARTESIAN_POINT ( 'NONE',  ( 6.486482029760648627E-15, 43.62500000273116996, 35.31076352940722529 ) ) ;
#4698=ORIENTED_EDGE ( 'NONE', *, *, #4457, .T. ) ;
#4700=LINE ( 'NONE', #23246, #19569 ) ;
#4702=CARTESIAN_POINT ( 'NONE',  ( 10.37757302488624767, 73.97500000273119269, 31.93888565452638417 ) ) ;
#4703=ORIENTED_EDGE ( 'NONE', *, *, #20979, .F. ) ;
#4709=CARTESIAN_POINT ( 'NONE',  ( 33.58253175000000113, 70.22500000273120691, -10.91162601494193751 ) ) ;
#4711=CARTESIAN_POINT ( 'NONE',  ( 15.14183272437241889, 13.70000000000000462, 20.84094480462498211 ) ) ;
#4712=DIRECTION ( 'NONE',  ( -0.000000000000000000, -1.000000000000000000, -0.000000000000000000 ) ) ;
#4713=CARTESIAN_POINT ( 'NONE',  ( -2.162160676586881955E-15, 8.625000002731169957, -35.31076352940723240 ) ) ;
#4716=CARTESIAN_POINT ( 'NONE',  ( 4.635254915624209993, 75.40000000000001990, -14.26584774442730463 ) ) ;
#4718=CARTESIAN_POINT ( 'NONE',  ( -26.29305231718578995, 70.19999999999998863, 19.10302069950538595 ) ) ;
#4719=CARTESIAN_POINT ( 'NONE',  ( 32.50000000000000000, 23.09999999999999432, -10.55989012756945833 ) ) ;
#4721=CARTESIAN_POINT ( 'NONE',  ( -11.25946833292375793, 78.67500000273119554, -8.180482586598733619 ) ) ;
#4723=CARTESIAN_POINT ( 'NONE',  ( 27.16883889988623935, 32.32500000273119412, -19.73931689729374384 ) ) ;
#4725=CARTESIAN_POINT ( 'NONE',  ( -33.58253175000000113, 21.37500000273118062, 0.000000000000000000 ) ) ;
#4726=CARTESIAN_POINT ( 'NONE',  ( -1.778240108872766143E-15, 12.00000000546238077, -32.49999999999999289 ) ) ;
#4727=CARTESIAN_POINT ( 'NONE',  ( 20.75514604977249178, 73.82500000273120122, 28.56700777964553950 ) ) ;
#4728=CARTESIAN_POINT ( 'NONE',  ( -32.50000000000000000, 65.89999999999999147, -10.55989012756945300 ) ) ;
#4730=CYLINDRICAL_SURFACE ( 'NONE', #25949, 32.50000000000000000 ) ;
#4731=CARTESIAN_POINT ( 'NONE',  ( 20.75514604977249178, 65.82500000273115859, 28.56700777964553950 ) ) ;
#4735=CARTESIAN_POINT ( 'NONE',  ( 20.75514604977248467, 8.425000002731204418, -28.56700777964554305 ) ) ;
#4736=CARTESIAN_POINT ( 'NONE',  ( 23.41746825000000243, 11.02499999726882152, 7.608796670333735079 ) ) ;
#4739=ORIENTED_EDGE ( 'NONE', *, *, #2377, .T. ) ;
#4741=ORIENTED_EDGE ( 'NONE', *, *, #12302, .T. ) ;
#4744=CARTESIAN_POINT ( 'NONE',  ( -1.778240108872766143E-15, 59.50000000000000711, -32.49999999999999289 ) ) ;
#4746=CARTESIAN_POINT ( 'NONE',  ( 0.000000000000000000, 80.00000000000001421, -32.50000000000000000 ) ) ;
#4747=CARTESIAN_POINT ( 'NONE',  ( -23.41746825000000598, 4.224999997268803931, 7.608796670333726198 ) ) ;
#4748=EDGE_CURVE ( 'NONE', #14496, #21334, #23824, .T. ) ;
#4749=EDGE_CURVE ( 'NONE', #10964, #27108, #31197, .T. ) ;
#4750=CARTESIAN_POINT ( 'NONE',  ( -7.236395654485757944, 11.22499999726880837, -22.27133577429736988 ) ) ;
#4751=CARTESIAN_POINT ( 'NONE',  ( -33.58253175000000113, 13.27500000273119518, -10.91162601494193218 ) ) ;
#4752=CARTESIAN_POINT ( 'NONE',  ( 20.08610463437157279, 21.80000000546236549, -27.64615127144129758 ) ) ;
#4753=CARTESIAN_POINT ( 'NONE',  ( -32.50000000000000000, 63.89999999999998437, -10.55989012756945478 ) ) ;
#4754=CARTESIAN_POINT ( 'NONE',  ( 12.13525491562420910, 77.45000000546237118, -8.816778784387098611 ) ) ;
#4755=FACE_OUTER_BOUND ( 'NONE', #16535, .T. ) ;
#4757=CARTESIAN_POINT ( 'NONE',  ( -20.75514604977248823, 29.07500000273119056, -28.56700777964554305 ) ) ;
#4758=CARTESIAN_POINT ( 'NONE',  ( -13.91746824999999887, 81.37500000273118417, 0.000000000000000000 ) ) ;
#4761=CARTESIAN_POINT ( 'NONE',  ( 7.236395654485760609, 15.52499999726880731, -22.27133577429736633 ) ) ;
#4762=CARTESIAN_POINT ( 'NONE',  ( 32.50000000000000000, 9.100000000000004974, -10.55989012756945833 ) ) ;
#4763=CARTESIAN_POINT ( 'NONE',  ( -5.147494310547430452, 51.55125428154684641, -32.49999999999999289 ) ) ;
#4765=CARTESIAN_POINT ( 'NONE',  ( -27.16883889988623935, 47.32500000273117990, 19.73931689729374739 ) ) ;
#4767=CARTESIAN_POINT ( 'NONE',  ( 10.37757302488624056, 42.77500000273118275, -31.93888565452638417 ) ) ;
#4769=AXIS2_PLACEMENT_3D ( 'NONE', #30087, #14492, #19479 ) ;
#4772=CARTESIAN_POINT ( 'NONE',  ( 10.04305231718578817, 51.90000000546238113, -30.90933677959249337 ) ) ;
#4776=FACE_OUTER_BOUND ( 'NONE', #26198, .T. ) ;
#4780=CARTESIAN_POINT ( 'NONE',  ( -5.147494310547377161, 60.05125428700924317, -32.50000000000002132 ) ) ;
#4781=CARTESIAN_POINT ( 'NONE',  ( 20.75514604977248467, 26.42500000273118843, -28.56700777964554305 ) ) ;
#4783=ORIENTED_EDGE ( 'NONE', *, *, #24050, .T. ) ;
#4786=CARTESIAN_POINT ( 'NONE',  ( -1.778240108872766143E-15, 16.00000000546237899, -32.49999999999999289 ) ) ;
#4787=ORIENTED_EDGE ( 'NONE', *, *, #33841, .T. ) ;
#4791=CIRCLE ( 'NONE', #26729, 24.50000000000000000 ) ;
#4793=CARTESIAN_POINT ( 'NONE',  ( 3.980102097228898626E-15, 80.00000000000001421, 32.50000000000000000 ) ) ;
#4794=CARTESIAN_POINT ( 'NONE',  ( -33.58253175000000113, 37.37500000273119838, 0.000000000000000000 ) ) ;
#4795=CARTESIAN_POINT ( 'NONE',  ( -10.04305231718578462, 44.90000000546237402, 30.90933677959249337 ) ) ;
#4797=CARTESIAN_POINT ( 'NONE',  ( 6.486482029760649416E-15, 23.62500000273119127, 35.31076352940723240 ) ) ;
#4799=CARTESIAN_POINT ( 'NONE',  ( 33.58253175000000823, 52.27500000273118985, 10.91162601494192863 ) ) ;
#4801=CARTESIAN_POINT ( 'NONE',  ( 10.04305231718578817, 27.40000000000000924, -30.90933677959249337 ) ) ;
#4804=CARTESIAN_POINT ( 'NONE',  ( 27.16883889988624290, 67.92500000273119554, 19.73931689729373673 ) ) ;
#4807=CARTESIAN_POINT ( 'NONE',  ( -33.58253175000000113, 63.47500000273117848, 10.91162601494193929 ) ) ;
#4809=CARTESIAN_POINT ( 'NONE',  ( 32.50000000000000000, 7.600000005462378638, -10.55989012756945833 ) ) ;
#4810=CARTESIAN_POINT ( 'NONE',  ( 20.75514604977248467, 18.42500000273117422, -28.56700777964554305 ) ) ;
#4811=CARTESIAN_POINT ( 'NONE',  ( 24.50000000000000000, 11.74999999453762989, 0.000000000000000000 ) ) ;
#4813=CARTESIAN_POINT ( 'NONE',  ( 32.50000000000000711, 46.90000000000000568, 10.55989012756945122 ) ) ;
#4822=CARTESIAN_POINT ( 'NONE',  ( 26.29305231718579350, 62.79999999999999716, 19.10302069950537529 ) ) ;
#4824=CARTESIAN_POINT ( 'NONE',  ( -32.50000000000000000, 53.90000000000001279, -10.55989012756945300 ) ) ;
#4825=CARTESIAN_POINT ( 'NONE',  ( 32.50000000000000000, 75.60000000546236265, -10.55989012756945833 ) ) ;
#4829=EDGE_LOOP ( 'NONE', ( #850, #10070, #28426, #24088 ) ) ;
#4830=CARTESIAN_POINT ( 'NONE',  ( -2.162160676586881955E-15, 76.87500000273115575, -35.31076352940723240 ) ) ;
#4834=CARTESIAN_POINT ( 'NONE',  ( 27.16883889988623935, 52.57500000273118701, -19.73931689729374384 ) ) ;
#4835=CARTESIAN_POINT ( 'NONE',  ( -26.29305231718578995, 60.70000000546238539, 19.10302069950538595 ) ) ;
#4838=CARTESIAN_POINT ( 'NONE',  ( 27.16883889988624290, 43.92500000273119554, 19.73931689729373673 ) ) ;
#4839=CYLINDRICAL_SURFACE ( 'NONE', #14868, 32.50000000000000000 ) ;
#4840=CARTESIAN_POINT ( 'NONE',  ( 27.16883889988624290, 66.17500000273118133, 19.73931689729373673 ) ) ;
#4841=CARTESIAN_POINT ( 'NONE',  ( -20.08610463437156923, 6.800000005462376151, 27.64615127144130113 ) ) ;
#4843=CARTESIAN_POINT ( 'NONE',  ( 0.000000000000000000, 80.00000000000001421, 0.000000000000000000 ) ) ;
#4844=CARTESIAN_POINT ( 'NONE',  ( 26.29305231718578995, 45.19999999999998863, -19.10302069950538240 ) ) ;
#4845=EDGE_CURVE ( 'NONE', #24499, #3193, #545, .T. ) ;
#4846=CARTESIAN_POINT ( 'NONE',  ( -32.50000000000000000, 13.89999999999999680, -10.55989012756945300 ) ) ;
#4847=CARTESIAN_POINT ( 'NONE',  ( 20.75514604977248467, 14.67500000273117955, -28.56700777964554305 ) ) ;
#4848=CARTESIAN_POINT ( 'NONE',  ( -5.147494310547403806, 73.55125428154681799, -32.50000000000000711 ) ) ;
#4850=CARTESIAN_POINT ( 'NONE',  ( -13.91746824999999532, 77.47500000273120691, 4.522059556121122093 ) ) ;
#4851=DIRECTION ( 'NONE',  ( 0.000000000000000000, 0.000000000000000000, -1.000000000000000000 ) ) ;
#4852=CARTESIAN_POINT ( 'NONE',  ( 5.779280353836490358E-15, 22.49999999999999645, 32.49999999999999289 ) ) ;
#4866=( BOUNDED_CURVE ( )  B_SPLINE_CURVE ( 2, ( #9645, #22691, #30396, #20127, #184, #13593, #5523, #31431, #21321, #26627, #28514, #8253, #12908 ),
 .UNSPECIFIED., .F., .T. ) 
 B_SPLINE_CURVE_WITH_KNOTS ( ( 3, 2, 2, 2, 2, 2, 3 ),
 ( 0.6500000000000000222, 0.6600000000000000311, 0.6800000000000000488, 0.6999999999999999556, 0.7199999999999999734, 0.7399999999999999911, 0.7500000000000000000 ),
 .UNSPECIFIED. ) 
 CURVE ( )  GEOMETRIC_REPRESENTATION_ITEM ( )  RATIONAL_B_SPLINE_CURVE ( ( 0.9755282581475768211, 0.9755282581475768211, 1.000000000000000000, 0.9510565162951535312, 1.000000000000000000, 0.9510565162951535312, 1.000000000000000000, 0.9510565162951535312, 1.000000000000000000, 0.9510565162951535312, 1.000000000000000000, 0.9755282581475768211, 0.9755282581475768211 ) ) 
 REPRESENTATION_ITEM ( '' )  );
#4867=CARTESIAN_POINT ( 'NONE',  ( 11.25946833292375793, 72.57500000273120122, -8.180482586598735395 ) ) ;
#4869=CARTESIAN_POINT ( 'NONE',  ( 20.75514604977248467, 48.42500000273119554, -28.56700777964554305 ) ) ;
#4872=EDGE_LOOP ( 'NONE', ( #18774, #31877, #27282, #19398 ) ) ;
#4874=CARTESIAN_POINT ( 'NONE',  ( -10.04305231718578462, 4.900000005462368691, 30.90933677959249337 ) ) ;
#4876=CARTESIAN_POINT ( 'NONE',  ( 20.75514604977249178, 76.07500000273118701, 28.56700777964553950 ) ) ;
#4877=ORIENTED_EDGE ( 'NONE', *, *, #21121, .T. ) ;
#4881=LINE ( 'NONE', #15872, #680 ) ;
#4882=CARTESIAN_POINT ( 'NONE',  ( -10.37757302488624411, 58.72500000273117848, -31.93888565452638417 ) ) ;
#4885=CARTESIAN_POINT ( 'NONE',  ( -14.47279130897152299, 4.424999997268826313, 19.92008829642072243 ) ) ;
#4886=CARTESIAN_POINT ( 'NONE',  ( -27.16883889988623935, 13.32500000273117990, 19.73931689729374739 ) ) ;
#4889=CARTESIAN_POINT ( 'NONE',  ( 9.270509831248423538, 73.29999999999996874, -12.75976212528059861 ) ) ;
#4891=CARTESIAN_POINT ( 'NONE',  ( 5.147494310547434893, 19.05125428700922185, 32.49999999999999289 ) ) ;
#4895=CARTESIAN_POINT ( 'NONE',  ( -8.601468415847515203, 79.17500000273120975, 11.83890561707634959 ) ) ;
#4897=CARTESIAN_POINT ( 'NONE',  ( 33.58253175000000823, 32.02500000273118275, 10.91162601494192863 ) ) ;
#4898=CARTESIAN_POINT ( 'NONE',  ( 0.000000000000000000, 80.00000000000001421, 0.000000000000000000 ) ) ;
#4900=CARTESIAN_POINT ( 'NONE',  ( 33.58253175000000113, 20.47500000273119980, -10.91162601494193574 ) ) ;
#4901=CARTESIAN_POINT ( 'NONE',  ( -4.635254915624208216, 80.40000000000000568, 14.26584774442730463 ) ) ;
#4902=CARTESIAN_POINT ( 'NONE',  ( -33.58253175000000113, 75.02500000273117564, -10.91162601494193041 ) ) ;
#4903=CARTESIAN_POINT ( 'NONE',  ( 26.29305231718578995, 59.70000000546238539, -19.10302069950538240 ) ) ;
#4905=CARTESIAN_POINT ( 'NONE',  ( 18.94512977948576093, 16.82499999726880091, -13.76444248337722875 ) ) ;
#4906=CARTESIAN_POINT ( 'NONE',  ( -33.58253175000000113, 63.02500000273118985, -10.91162601494193041 ) ) ;
#4910=CARTESIAN_POINT ( 'NONE',  ( -20.75514604977248823, 6.825000002731195892, -28.56700777964554305 ) ) ;
#4911=CARTESIAN_POINT ( 'NONE',  ( 14.47279130897151589, 16.82499999726881512, 19.92008829642072953 ) ) ;
#4916=ORIENTED_EDGE ( 'NONE', *, *, #32529, .T. ) ;
#4921=CARTESIAN_POINT ( 'NONE',  ( -23.41746825000000598, 2.224999997268808816, 7.608796670333726198 ) ) ;
#4922=CARTESIAN_POINT ( 'NONE',  ( -23.41746825000000598, 9.724999997268804819, 7.608796670333726198 ) ) ;
#4923=CARTESIAN_POINT ( 'NONE',  ( 10.37757302488624056, 14.77500000273118630, -31.93888565452638417 ) ) ;
#4924=CARTESIAN_POINT ( 'NONE',  ( 10.04305231718578817, 15.90000000546237757, -30.90933677959249337 ) ) ;
#4925=CARTESIAN_POINT ( 'NONE',  ( -2.092463501923844636E-15, 63.50000000000000000, -34.17252228774368916 ) ) ;
#4926=CARTESIAN_POINT ( 'NONE',  ( 15.14183272437242067, 11.44999999453763095, 20.84094480462498211 ) ) ;
#4927=CARTESIAN_POINT ( 'NONE',  ( 3.445340210940985210E-14, 5.499999999999997335, 24.50000000000000000 ) ) ;
#4929=CARTESIAN_POINT ( 'NONE',  ( -32.50000000000000000, 32.50000000546238255, 0.000000000000000000 ) ) ;
#4932=CARTESIAN_POINT ( 'NONE',  ( 23.41746824999999887, 17.12499999726882649, 0.000000000000000000 ) ) ;
#4933=CARTESIAN_POINT ( 'NONE',  ( -32.50000000000000000, 8.100000000000006750, 10.55989012756946366 ) ) ;
#4934=CARTESIAN_POINT ( 'NONE',  ( -4.635254915624208216, 74.40000000000001990, 14.26584774442730463 ) ) ;
#4936=CARTESIAN_POINT ( 'NONE',  ( 27.16883889988623935, 52.32500000273118701, -19.73931689729374384 ) ) ;
#4938=CARTESIAN_POINT ( 'NONE',  ( -27.16883889988623935, 39.57500000273117280, 19.73931689729374739 ) ) ;
#4941=CARTESIAN_POINT ( 'NONE',  ( -5.147494310547423346, 62.44874571845315359, 32.50000000000000000 ) ) ;
#4943=CARTESIAN_POINT ( 'NONE',  ( -32.50000000000000000, 27.99999999999999645, 0.000000000000000000 ) ) ;
#4945=CARTESIAN_POINT ( 'NONE',  ( -26.29305231718578995, 62.70000000546238539, 19.10302069950538595 ) ) ;
#4948=DIRECTION ( 'NONE',  ( 0.000000000000000000, 0.000000000000000000, -1.000000000000000000 ) ) ;
#4953=CARTESIAN_POINT ( 'NONE',  ( 33.58253175000000823, 24.02500000273117919, 10.91162601494192685 ) ) ;
#4962=ORIENTED_EDGE ( 'NONE', *, *, #17336, .F. ) ;
#4964=( BOUNDED_CURVE ( )  B_SPLINE_CURVE ( 2, ( #23967, #8167, #16082, #26536, #26867, #13832, #10921, #13669, #16743, #32176, #437, #29265, #5768 ),
 .UNSPECIFIED., .F., .T. ) 
 B_SPLINE_CURVE_WITH_KNOTS ( ( 3, 2, 2, 2, 2, 2, 3 ),
 ( 0.4551282051282051211, 0.4564102564102563986, 0.4589743589743589536, 0.4615384615384615641, 0.4641025641025641191, 0.4666666666666666741, 0.4679487179487179516 ),
 .UNSPECIFIED. ) 
 CURVE ( )  GEOMETRIC_REPRESENTATION_ITEM ( )  RATIONAL_B_SPLINE_CURVE ( ( 0.9755282581475768211, 0.9755282581475768211, 1.000000000000000000, 0.9510565162951535312, 1.000000000000000000, 0.9510565162951535312, 1.000000000000000000, 0.9510565162951535312, 1.000000000000000000, 0.9510565162951535312, 1.000000000000000000, 0.9755282581475768211, 0.9755282581475768211 ) ) 
 REPRESENTATION_ITEM ( '' )  );
#4967=CARTESIAN_POINT ( 'NONE',  ( -20.08610463437157989, 45.69999999999998153, -27.64615127144129758 ) ) ;
#4968=CARTESIAN_POINT ( 'NONE',  ( 27.16883889988624290, 36.17500000273118843, 19.73931689729373673 ) ) ;
#4969=CARTESIAN_POINT ( 'NONE',  ( -32.50000000000000000, 40.60000000546239107, 10.55989012756946366 ) ) ;
#4970=( BOUNDED_CURVE ( )  B_SPLINE_CURVE ( 2, ( #9863, #10043, #28055, #15193, #20172, #30615, #33188, #7798, #28396, #20858, #33888, #31304, #25992, #31139, #18287, #22911, #2486, #12954, #4543, #28732, #12784, #17593, #33720, #15711, #25656, #7464, #15017, #26167, #30965, #23428, #17947, #20340, #2659, #4885, #7111, #23257, #25487, #1966, #10217, #20697, #7630, #12441, #33367, #30790, #5056, #15540, #15876, #3168, #23935, #13638, #21695, #570, #736, #31639, #31477, #5738, #26333, #2996, #11061, #2821, #8298, #230, #23764, #18790, #16542, #21364, #16048, #21526, #404, #26995, #10717, #7969, #26503, #18455, #8469, #13469, #28898, #60, #24269, #10890, #5400, #5567, #13290, #21196, #24102, #31974, #26673, #18957, #29402, #29233, #8137, #29062, #10547, #18626, #31807, #5904, #16218, #16381, #26834, #3330, #13800, #19121, #11221, #32142, #8636, #29558, #6058, #13120, #23595, #21028, #30061, #6399, #30401, #32307, #6901, #3657, #29897, #16709, #27164, #14464, #3991, #11709, #1571, #6567, #11883, #16874, #17382, #9473, #9134, #19615, #12048, #14296, #27501, #6730, #17041, #6230, #19954, #27337, #22518, #14133, #17213, #32639, #3823, #21859, #8799, #24589, #32969, #24920, #1405, #3493, #22354, #19779, #1061, #32801, #11384, #11542, #9294, #27671, #30228, #902, #4161, #19282, #19451, #24425, #29725, #13962, #22024, #14634, #25093, #32468, #8969, #24754, #1230, #22192, #28012, #7593, #18070, #33144, #15496, #20474, #7238 ),
 .UNSPECIFIED., .F., .T. ) 
 B_SPLINE_CURVE_WITH_KNOTS ( ( 3, 2, 2, 2, 2, 2, 2, 2, 2, 2, 2, 2, 2, 2, 2, 2, 2, 2, 2, 2, 2, 2, 2, 2, 2, 2, 2, 2, 2, 2, 2, 2, 2, 2, 2, 2, 2, 2, 2, 2, 2, 2, 2, 2, 2, 2, 2, 2, 2, 2, 2, 2, 2, 2, 2, 2, 2, 2, 2, 2, 2, 2, 2, 2, 2, 2, 2, 2, 2, 2, 2, 2, 2, 2, 2, 2, 2, 2, 2, 2, 2, 2, 2, 2, 2, 2, 2, 2, 2, 2, 3 ),
 ( 0.000000000000000000, 0.01111111111111111154, 0.02222222222222222307, 0.03333333333333333287, 0.04444444444444444614, 0.05555555555555555247, 0.06666666666666666574, 0.07777777777777777901, 0.08888888888888889228, 0.1000000000000000056, 0.1111111111111111049, 0.1222222222222222182, 0.1333333333333333315, 0.1444444444444444309, 0.1555555555555555580, 0.1666666666666666574, 0.1777777777777777846, 0.1888888888888888840, 0.2000000000000000111, 0.2111111111111111105, 0.2222222222222222099, 0.2333333333333333370, 0.2444444444444444364, 0.2555555555555555358, 0.2666666666666666630, 0.2777777777777777901, 0.2888888888888888618, 0.2999999999999999889, 0.3111111111111111160, 0.3222222222222222432, 0.3333333333333333148, 0.3444444444444444420, 0.3555555555555555691, 0.3666666666666666408, 0.3777777777777777679, 0.3888888888888888951, 0.4000000000000000222, 0.4111111111111110938, 0.4222222222222222210, 0.4333333333333333481, 0.4444444444444444198, 0.4555555555555555469, 0.4666666666666666741, 0.4777777777777778012, 0.4888888888888888729, 0.5000000000000000000, 0.5111111111111110716, 0.5222222222222222543, 0.5333333333333333259, 0.5444444444444443976, 0.5555555555555555802, 0.5666666666666666519, 0.5777777777777777235, 0.5888888888888889062, 0.5999999999999999778, 0.6111111111111111605, 0.6222222222222222321, 0.6333333333333333037, 0.6444444444444444864, 0.6555555555555555580, 0.6666666666666666297, 0.6777777777777778123, 0.6888888888888888840, 0.6999999999999999556, 0.7111111111111111382, 0.7222222222222222099, 0.7333333333333332815, 0.7444444444444444642, 0.7555555555555555358, 0.7666666666666667185, 0.7777777777777777901, 0.7888888888888888618, 0.8000000000000000444, 0.8111111111111111160, 0.8222222222222221877, 0.8333333333333333703, 0.8444444444444444420, 0.8555555555555555136, 0.8666666666666666963, 0.8777777777777777679, 0.8888888888888888395, 0.9000000000000000222, 0.9111111111111110938, 0.9222222222222222765, 0.9333333333333333481, 0.9444444444444444198, 0.9555555555555556024, 0.9666666666666666741, 0.9777777777777777457, 0.9888888888888889284, 1.000000000000000000 ),
 .UNSPECIFIED. ) 
 CURVE ( )  GEOMETRIC_REPRESENTATION_ITEM ( )  RATIONAL_B_SPLINE_CURVE ( ( 1.000000000000000000, 0.9510565162951535312, 1.000000000000000000, 0.9510565162951535312, 1.000000000000000000, 0.9510565162951535312, 1.000000000000000000, 0.9510565162951535312, 1.000000000000000000, 0.9510565162951535312, 1.000000000000000000, 0.9510565162951535312, 1.000000000000000000, 0.9510565162951535312, 1.000000000000000000, 0.9510565162951535312, 1.000000000000000000, 0.9510565162951535312, 1.000000000000000000, 0.9510565162951535312, 1.000000000000000000, 0.9510565162951535312, 1.000000000000000000, 0.9510565162951535312, 1.000000000000000000, 0.9510565162951535312, 1.000000000000000000, 0.9510565162951535312, 1.000000000000000000, 0.9510565162951535312, 1.000000000000000000, 0.9510565162951535312, 1.000000000000000000, 0.9510565162951535312, 1.000000000000000000, 0.9510565162951535312, 1.000000000000000000, 0.9510565162951535312, 1.000000000000000000, 0.9510565162951535312, 1.000000000000000000, 0.9510565162951535312, 1.000000000000000000, 0.9510565162951535312, 1.000000000000000000, 0.9510565162951535312, 1.000000000000000000, 0.9510565162951535312, 1.000000000000000000, 0.9510565162951535312, 1.000000000000000000, 0.9510565162951535312, 1.000000000000000000, 0.9510565162951535312, 1.000000000000000000, 0.9510565162951535312, 1.000000000000000000, 0.9510565162951535312, 1.000000000000000000, 0.9510565162951535312, 1.000000000000000000, 0.9510565162951535312, 1.000000000000000000, 0.9510565162951535312, 1.000000000000000000, 0.9510565162951535312, 1.000000000000000000, 0.9510565162951535312, 1.000000000000000000, 0.9510565162951535312, 1.000000000000000000, 0.9510565162951535312, 1.000000000000000000, 0.9510565162951535312, 1.000000000000000000, 0.9510565162951535312, 1.000000000000000000, 0.9510565162951535312, 1.000000000000000000, 0.9510565162951535312, 1.000000000000000000, 0.9510565162951535312, 1.000000000000000000, 0.9510565162951535312, 1.000000000000000000, 0.9510565162951535312, 1.000000000000000000, 0.9510565162951535312, 1.000000000000000000, 0.9510565162951535312, 1.000000000000000000, 0.9510565162951535312, 1.000000000000000000, 0.9510565162951535312, 1.000000000000000000, 0.9510565162951535312, 1.000000000000000000, 0.9510565162951535312, 1.000000000000000000, 0.9510565162951535312, 1.000000000000000000, 0.9510565162951535312, 1.000000000000000000, 0.9510565162951535312, 1.000000000000000000, 0.9510565162951535312, 1.000000000000000000, 0.9510565162951535312, 1.000000000000000000, 0.9510565162951535312, 1.000000000000000000, 0.9510565162951535312, 1.000000000000000000, 0.9510565162951535312, 1.000000000000000000, 0.9510565162951535312, 1.000000000000000000, 0.9510565162951535312, 1.000000000000000000, 0.9510565162951535312, 1.000000000000000000, 0.9510565162951535312, 1.000000000000000000, 0.9510565162951535312, 1.000000000000000000, 0.9510565162951535312, 1.000000000000000000, 0.9510565162951535312, 1.000000000000000000, 0.9510565162951535312, 1.000000000000000000, 0.9510565162951535312, 1.000000000000000000, 0.9510565162951535312, 1.000000000000000000, 0.9510565162951535312, 1.000000000000000000, 0.9510565162951535312, 1.000000000000000000, 0.9510565162951535312, 1.000000000000000000, 0.9510565162951535312, 1.000000000000000000, 0.9510565162951535312, 1.000000000000000000, 0.9510565162951535312, 1.000000000000000000, 0.9510565162951535312, 1.000000000000000000, 0.9510565162951535312, 1.000000000000000000, 0.9510565162951535312, 1.000000000000000000, 0.9510565162951535312, 1.000000000000000000, 0.9510565162951535312, 1.000000000000000000, 0.9510565162951535312, 1.000000000000000000, 0.9510565162951535312, 1.000000000000000000, 0.9510565162951535312, 1.000000000000000000, 0.9510565162951535312, 1.000000000000000000, 0.9510565162951535312, 1.000000000000000000, 0.9510565162951535312, 1.000000000000000000, 0.9510565162951535312, 1.000000000000000000, 0.9510565162951535312, 1.000000000000000000, 0.9510565162951535312, 1.000000000000000000, 0.9510565162951535312, 1.000000000000000000, 0.9510565162951535312, 1.000000000000000000, 0.9510565162951535312, 1.000000000000000000 ) ) 
 REPRESENTATION_ITEM ( '' )  );
#4972=CARTESIAN_POINT ( 'NONE',  ( -20.08610463437156923, 48.30000000000001847, 27.64615127144130113 ) ) ;
#4973=CARTESIAN_POINT ( 'NONE',  ( -2.162160676586881955E-15, 22.62500000273119127, -35.31076352940723240 ) ) ;
#4975=CARTESIAN_POINT ( 'NONE',  ( 6.486482029760649416E-15, 49.87500000273119838, 35.31076352940723240 ) ) ;
#4977=CARTESIAN_POINT ( 'NONE',  ( -10.04305231718578462, 30.39999999999998437, 30.90933677959249337 ) ) ;
#4979=CARTESIAN_POINT ( 'NONE',  ( -20.75514604977248823, 70.82500000273117280, -28.56700777964554305 ) ) ;
#4981=CARTESIAN_POINT ( 'NONE',  ( -5.147494310547423346, 38.44874571845315359, 32.50000000000000000 ) ) ;
#4982=CARTESIAN_POINT ( 'NONE',  ( -33.58253175000000113, 63.37500000273119127, 0.000000000000000000 ) ) ;
#4983=CARTESIAN_POINT ( 'NONE',  ( 32.50000000000000711, 72.89999999999999147, 10.55989012756945122 ) ) ;
#4984=CARTESIAN_POINT ( 'NONE',  ( -10.37757302488624411, 10.72500000273118914, -31.93888565452638417 ) ) ;
#4989=CARTESIAN_POINT ( 'NONE',  ( 5.147494310547434893, 18.55125428154684286, 32.49999999999999289 ) ) ;
#4996=CARTESIAN_POINT ( 'NONE',  ( -10.04305231718578462, 76.90000000546237402, 30.90933677959249337 ) ) ;
#5001=CARTESIAN_POINT ( 'NONE',  ( -2.162160676586881955E-15, 74.87500000273116996, -35.31076352940723240 ) ) ;
#5005=CARTESIAN_POINT ( 'NONE',  ( 20.75514604977249178, 56.07500000273117990, 28.56700777964553950 ) ) ;
#5006=CARTESIAN_POINT ( 'NONE',  ( -32.50000000000000000, 56.50000000546237544, 0.000000000000000000 ) ) ;
#5008=CARTESIAN_POINT ( 'NONE',  ( 20.75514604977248467, 42.42500000273117422, -28.56700777964554305 ) ) ;
#5009=CARTESIAN_POINT ( 'NONE',  ( -2.375766604868041476, 72.44874571845316780, 14.99999999999999822 ) ) ;
#5011=CARTESIAN_POINT ( 'NONE',  ( -20.75514604977248823, 69.07500000273115859, -28.56700777964554305 ) ) ;
#5012=CARTESIAN_POINT ( 'NONE',  ( 20.08610463437157279, 5.800000005462378816, -27.64615127144129758 ) ) ;
#5015=CARTESIAN_POINT ( 'NONE',  ( -10.04305231718578462, 48.39999999999999858, 30.90933677959249337 ) ) ;
#5016=DIRECTION ( 'NONE',  ( -0.000000000000000000, -1.000000000000000000, -0.000000000000000000 ) ) ;
#5017=CARTESIAN_POINT ( 'NONE',  ( 27.16883889988624290, 12.17500000273119554, 19.73931689729373673 ) ) ;
#5018=CARTESIAN_POINT ( 'NONE',  ( -3.880418787951124493, 7.448745718453147369, 24.50000000000000355 ) ) ;
#5020=CARTESIAN_POINT ( 'NONE',  ( -11.25946833292375793, 71.07500000273120122, 8.180482586598737171 ) ) ;
#5022=CARTESIAN_POINT ( 'NONE',  ( -20.08610463437157989, 21.69999999999998153, -27.64615127144129758 ) ) ;
#5024=VERTEX_POINT ( 'NONE', #6290 ) ;
#5038=CARTESIAN_POINT ( 'NONE',  ( -33.58253175000000113, 45.22500000273117848, 10.91162601494193929 ) ) ;
#5041=ORIENTED_EDGE ( 'NONE', *, *, #16366, .T. ) ;
#5046=CARTESIAN_POINT ( 'NONE',  ( 27.16883889988624290, 76.17500000273119554, 19.73931689729373673 ) ) ;
#5047=EDGE_CURVE ( 'NONE', #22185, #17375, #29293, .T. ) ;
#5048=ORIENTED_EDGE ( 'NONE', *, *, #16975, .F. ) ;
#5051=VERTEX_POINT ( 'NONE', #6118 ) ;
#5052=DIRECTION ( 'NONE',  ( 0.000000000000000000, 0.000000000000000000, 1.000000000000000000 ) ) ;
#5053=CARTESIAN_POINT ( 'NONE',  ( -33.58253175000000113, 59.12500000273118417, 0.000000000000000000 ) ) ;
#5055=CARTESIAN_POINT ( 'NONE',  ( 7.570916362186213000, 16.39999999999999858, -23.30088464923126423 ) ) ;
#5056=CARTESIAN_POINT ( 'NONE',  ( 7.236395654485760609, 5.524999997268825958, -22.27133577429736633 ) ) ;
#5057=CARTESIAN_POINT ( 'NONE',  ( -33.58253175000000113, 3.125000002731193049, 0.000000000000000000 ) ) ;
#5059=CARTESIAN_POINT ( 'NONE',  ( -10.37757302488624411, 78.97500000273119269, -31.93888565452638417 ) ) ;
#5061=CARTESIAN_POINT ( 'NONE',  ( 32.50000000000000711, 75.40000000546238823, 10.55989012756945122 ) ) ;
#5065=CARTESIAN_POINT ( 'NONE',  ( 15.00000000000000355, 73.15000000546240244, 4.873795443493592394 ) ) ;
#5067=( BOUNDED_SURFACE ( )  B_SPLINE_SURFACE ( 1, 2, ( 
 ( #6783, #7120, #22242, #4379, #17777, #19829, #30111, #1282, #27724, #20349, #22920, #9182, #9346, #11761, #4212, #4551, #30281, #33376, #11934, #22403, #22570, #1455, #17093, #17435, #9871, #14854, #6951, #30799, #6615, #17261, #14684, #25320, #7292, #9700, #1621, #15030, #32687, #33020, #17602, #12450, #28235, #32851, #4040, #1794, #30624, #9526, #24804, #19666, #27552, #12272, #27896, #14514, #25495, #1975, #24973, #20007, #30454, #22746, #33197, #20180, #12964, #15375, #23604, #7978, #10559, #18124, #18464, #71, #2144, #28908, #25665, #5065, #25830, #5409, #10227, #10050, #26002, #15888, #2495, #12619, #20707, #26344, #23438, #2671, #28569, #23086, #23267, #33549, #2320, #7474, #7808, #13302, #28742, #31316, #23777, #20531, #31149, #7640, #15722, #31650, #21038 ),
 ( #33899, #31488, #26177, #12793, #15550, #15201, #5238, #10390, #33729, #2833, #20868, #30974, #18297, #17956, #13130, #28405, #243, #4895, #10729, #21206, #8148, #18637, #4721, #11069, #13809, #414, #14143, #5913, #29735, #24111, #26682, #32318, #26843, #3008, #31983, #8980, #29074, #745, #3338, #32479, #3178, #3669, #27004, #24277, #3502, #579, #16228, #11230, #6068, #13647, #912, #6240, #19292, #1073, #21535, #21706, #8480, #5578, #27176, #13972, #18967, #16721, #22035, #24599, #32152, #24435, #8645, #19130, #10900, #16059, #29567, #23945, #16551, #11391, #29411, #21868, #8809, #11553, #26514, #13480, #21373, #31817, #8308, #18799, #29243, #16390, #5747, #25107, #27684, #12410, #19790, #7083, #14308, #6744, #9485, #6578, #19462, #4341, #19627, #1583, #20143 ) ),
 .UNSPECIFIED., .F., .F., .F. ) 
 B_SPLINE_SURFACE_WITH_KNOTS ( ( 2, 2 ),
 ( 3, 2, 2, 2, 2, 2, 2, 2, 2, 2, 2, 2, 2, 2, 2, 2, 2, 2, 2, 2, 2, 2, 2, 2, 2, 2, 2, 2, 2, 2, 2, 2, 2, 2, 2, 2, 2, 2, 2, 2, 2, 2, 2, 2, 2, 2, 2, 2, 2, 2, 3 ),
 ( 0.000000000000000000, 1.000000000000000000 ),
 ( 0.000000000000000000, 0.02000000000000000042, 0.04000000000000000083, 0.05999999999999999778, 0.08000000000000000167, 0.1000000000000000056, 0.1199999999999999956, 0.1400000000000000133, 0.1600000000000000033, 0.1799999999999999933, 0.2000000000000000111, 0.2200000000000000011, 0.2399999999999999911, 0.2600000000000000089, 0.2800000000000000266, 0.2999999999999999889, 0.3200000000000000067, 0.3400000000000000244, 0.3599999999999999867, 0.3800000000000000044, 0.4000000000000000222, 0.4199999999999999845, 0.4400000000000000022, 0.4600000000000000200, 0.4799999999999999822, 0.5000000000000000000, 0.5200000000000000178, 0.5400000000000000355, 0.5600000000000000533, 0.5799999999999999600, 0.5999999999999999778, 0.6199999999999999956, 0.6400000000000000133, 0.6600000000000000311, 0.6800000000000000488, 0.6999999999999999556, 0.7199999999999999734, 0.7399999999999999911, 0.7600000000000000089, 0.7800000000000000266, 0.8000000000000000444, 0.8199999999999999512, 0.8399999999999999689, 0.8599999999999999867, 0.8800000000000000044, 0.9000000000000000222, 0.9200000000000000400, 0.9399999999999999467, 0.9599999999999999645, 0.9799999999999999822, 1.000000000000000000 ),
 .UNSPECIFIED. ) 
 GEOMETRIC_REPRESENTATION_ITEM ( )  RATIONAL_B_SPLINE_SURFACE ( (
 ( 1.000000000000000000, 0.9510565162951535312, 1.000000000000000000, 0.9510565162951535312, 1.000000000000000000, 0.9510565162951535312, 1.000000000000000000, 0.9510565162951535312, 1.000000000000000000, 0.9510565162951535312, 1.000000000000000000, 0.9510565162951535312, 1.000000000000000000, 0.9510565162951535312, 1.000000000000000000, 0.9510565162951535312, 1.000000000000000000, 0.9510565162951535312, 1.000000000000000000, 0.9510565162951535312, 1.000000000000000000, 0.9510565162951535312, 1.000000000000000000, 0.9510565162951535312, 1.000000000000000000, 0.9510565162951535312, 1.000000000000000000, 0.9510565162951535312, 1.000000000000000000, 0.9510565162951535312, 1.000000000000000000, 0.9510565162951535312, 1.000000000000000000, 0.9510565162951535312, 1.000000000000000000, 0.9510565162951535312, 1.000000000000000000, 0.9510565162951535312, 1.000000000000000000, 0.9510565162951535312, 1.000000000000000000, 0.9510565162951535312, 1.000000000000000000, 0.9510565162951535312, 1.000000000000000000, 0.9510565162951535312, 1.000000000000000000, 0.9510565162951535312, 1.000000000000000000, 0.9510565162951535312, 1.000000000000000000, 0.9510565162951535312, 1.000000000000000000, 0.9510565162951535312, 1.000000000000000000, 0.9510565162951535312, 1.000000000000000000, 0.9510565162951535312, 1.000000000000000000, 0.9510565162951535312, 1.000000000000000000, 0.9510565162951535312, 1.000000000000000000, 0.9510565162951535312, 1.000000000000000000, 0.9510565162951535312, 1.000000000000000000, 0.9510565162951535312, 1.000000000000000000, 0.9510565162951535312, 1.000000000000000000, 0.9510565162951535312, 1.000000000000000000, 0.9510565162951535312, 1.000000000000000000, 0.9510565162951535312, 1.000000000000000000, 0.9510565162951535312, 1.000000000000000000, 0.9510565162951535312, 1.000000000000000000, 0.9510565162951535312, 1.000000000000000000, 0.9510565162951535312, 1.000000000000000000, 0.9510565162951535312, 1.000000000000000000, 0.9510565162951535312, 1.000000000000000000, 0.9510565162951535312, 1.000000000000000000, 0.9510565162951535312, 1.000000000000000000, 0.9510565162951535312, 1.000000000000000000, 0.9510565162951535312, 1.000000000000000000, 0.9510565162951535312, 1.000000000000000000, 0.9510565162951535312, 1.000000000000000000),
 ( 1.000000000000000000, 0.9510565162951535312, 1.000000000000000000, 0.9510565162951535312, 1.000000000000000000, 0.9510565162951535312, 1.000000000000000000, 0.9510565162951535312, 1.000000000000000000, 0.9510565162951535312, 1.000000000000000000, 0.9510565162951535312, 1.000000000000000000, 0.9510565162951535312, 1.000000000000000000, 0.9510565162951535312, 1.000000000000000000, 0.9510565162951535312, 1.000000000000000000, 0.9510565162951535312, 1.000000000000000000, 0.9510565162951535312, 1.000000000000000000, 0.9510565162951535312, 1.000000000000000000, 0.9510565162951535312, 1.000000000000000000, 0.9510565162951535312, 1.000000000000000000, 0.9510565162951535312, 1.000000000000000000, 0.9510565162951535312, 1.000000000000000000, 0.9510565162951535312, 1.000000000000000000, 0.9510565162951535312, 1.000000000000000000, 0.9510565162951535312, 1.000000000000000000, 0.9510565162951535312, 1.000000000000000000, 0.9510565162951535312, 1.000000000000000000, 0.9510565162951535312, 1.000000000000000000, 0.9510565162951535312, 1.000000000000000000, 0.9510565162951535312, 1.000000000000000000, 0.9510565162951535312, 1.000000000000000000, 0.9510565162951535312, 1.000000000000000000, 0.9510565162951535312, 1.000000000000000000, 0.9510565162951535312, 1.000000000000000000, 0.9510565162951535312, 1.000000000000000000, 0.9510565162951535312, 1.000000000000000000, 0.9510565162951535312, 1.000000000000000000, 0.9510565162951535312, 1.000000000000000000, 0.9510565162951535312, 1.000000000000000000, 0.9510565162951535312, 1.000000000000000000, 0.9510565162951535312, 1.000000000000000000, 0.9510565162951535312, 1.000000000000000000, 0.9510565162951535312, 1.000000000000000000, 0.9510565162951535312, 1.000000000000000000, 0.9510565162951535312, 1.000000000000000000, 0.9510565162951535312, 1.000000000000000000, 0.9510565162951535312, 1.000000000000000000, 0.9510565162951535312, 1.000000000000000000, 0.9510565162951535312, 1.000000000000000000, 0.9510565162951535312, 1.000000000000000000, 0.9510565162951535312, 1.000000000000000000, 0.9510565162951535312, 1.000000000000000000, 0.9510565162951535312, 1.000000000000000000, 0.9510565162951535312, 1.000000000000000000, 0.9510565162951535312, 1.000000000000000000, 0.9510565162951535312, 1.000000000000000000) ) ) 
 REPRESENTATION_ITEM ( '' )  SURFACE ( )  );
#5068=CARTESIAN_POINT ( 'NONE',  ( -10.37757302488624411, 28.72500000273120335, -31.93888565452638417 ) ) ;
#5071=CARTESIAN_POINT ( 'NONE',  ( -10.37757302488623701, 23.77500000273119340, 31.93888565452638417 ) ) ;
#5074=CARTESIAN_POINT ( 'NONE',  ( 27.16883889988624290, 77.92500000273116711, 19.73931689729373673 ) ) ;
#5075=CARTESIAN_POINT ( 'NONE',  ( -32.50000000000000000, 26.40000000546236691, -10.55989012756945300 ) ) ;
#5077=FACE_OUTER_BOUND ( 'NONE', #6052, .T. ) ;
#5078=CARTESIAN_POINT ( 'NONE',  ( -33.58253175000000113, 63.22500000273119269, 10.91162601494193929 ) ) ;
#5079=VECTOR ( 'NONE', #2791, 1000.000000000000000 ) ;
#5082=CARTESIAN_POINT ( 'NONE',  ( 10.37757302488624056, 6.525000002731207616, -31.93888565452638417 ) ) ;
#5084=CARTESIAN_POINT ( 'NONE',  ( -23.41746825000000598, 16.22499999726880304, 7.608796670333726198 ) ) ;
#5088=ORIENTED_EDGE ( 'NONE', *, *, #12201, .F. ) ;
#5092=CARTESIAN_POINT ( 'NONE',  ( 32.50000000000000711, 27.40000000546239534, 10.55989012756945122 ) ) ;
#5093=CARTESIAN_POINT ( 'NONE',  ( -7.236395654485757944, 3.724999997268802154, -22.27133577429736988 ) ) ;
#5094=CARTESIAN_POINT ( 'NONE',  ( -23.41746824999999887, 15.62499999726882294, -2.867812753649727150E-15 ) ) ;
#5095=CARTESIAN_POINT ( 'NONE',  ( 27.16883889988623935, 16.57500000273118346, -19.73931689729374384 ) ) ;
#5096=CARTESIAN_POINT ( 'NONE',  ( 26.29305231718579350, 21.30000000546239391, 19.10302069950537529 ) ) ;
#5098=CARTESIAN_POINT ( 'NONE',  ( -20.08610463437156923, 64.29999999999996874, 27.64615127144130113 ) ) ;
#5099=CARTESIAN_POINT ( 'NONE',  ( -4.223320258572819786E-15, 11.24999999453763344, 24.50000000000000000 ) ) ;
#5101=CARTESIAN_POINT ( 'NONE',  ( 13.91746825000000065, 80.27500000273117564, 4.522059556121114987 ) ) ;
#5105=DIRECTION ( 'NONE',  ( -0.000000000000000000, 1.000000000000000000, -0.000000000000000000 ) ) ;
#5106=CARTESIAN_POINT ( 'NONE',  ( 7.236395654485755280, 14.72499999726881192, 22.27133577429736988 ) ) ;
#5107=CARTESIAN_POINT ( 'NONE',  ( -26.29305231718578995, 10.19999999999998685, 19.10302069950538595 ) ) ;
#5108=CARTESIAN_POINT ( 'NONE',  ( 5.147494310547434893, 17.05125428700922541, 32.49999999999999289 ) ) ;
#5110=CARTESIAN_POINT ( 'NONE',  ( -10.37757302488624411, 52.72500000273119980, -31.93888565452638417 ) ) ;
#5112=CARTESIAN_POINT ( 'NONE',  ( -10.37757302488623701, 43.77500000273118275, 31.93888565452638417 ) ) ;
#5113=CARTESIAN_POINT ( 'NONE',  ( 5.779280353836490358E-15, 23.00000000546237899, 32.49999999999999289 ) ) ;
#5114=CARTESIAN_POINT ( 'NONE',  ( 2.445080149700053643E-15, 74.50000000000001421, 15.00000000000000000 ) ) ;
#5115=CARTESIAN_POINT ( 'NONE',  ( -7.570916362186210335, 8.599999999999996092, -23.30088464923126779 ) ) ;
#5119=CARTESIAN_POINT ( 'NONE',  ( 10.04305231718578817, 7.400000000000018119, -30.90933677959249337 ) ) ;
#5120=DIRECTION ( 'NONE',  ( -1.000000000000000000, 0.000000000000000000, -0.000000000000000000 ) ) ;
#5121=CARTESIAN_POINT ( 'NONE',  ( 15.14183272437242067, 11.70000000000000817, 20.84094480462498211 ) ) ;
#5124=CARTESIAN_POINT ( 'NONE',  ( -7.570916362186210335, 10.34999999453761710, -23.30088464923126779 ) ) ;
#5125=CARTESIAN_POINT ( 'NONE',  ( 27.16883889988624290, 25.92500000273118133, 19.73931689729373673 ) ) ;
#5135=CARTESIAN_POINT ( 'NONE',  ( 7.236395654485755280, 2.224999997268800378, 22.27133577429736988 ) ) ;
#5136=CARTESIAN_POINT ( 'NONE',  ( 10.37757302488624056, 36.77500000273120406, -31.93888565452638417 ) ) ;
#5137=CARTESIAN_POINT ( 'NONE',  ( -26.29305231718578995, 38.70000000546236407, 19.10302069950538595 ) ) ;
#5140=CARTESIAN_POINT ( 'NONE',  ( -33.58253175000000113, 25.12500000273118417, 0.000000000000000000 ) ) ;
#5141=CARTESIAN_POINT ( 'NONE',  ( 5.147494310547434893, 76.55125428154684641, 32.49999999999999289 ) ) ;
#5142=CARTESIAN_POINT ( 'NONE',  ( -10.37757302488624411, 48.97500000273119269, -31.93888565452638417 ) ) ;
#5145=CARTESIAN_POINT ( 'NONE',  ( -32.50000000000000000, 27.89999999999999147, -10.55989012756945478 ) ) ;
#5147=CARTESIAN_POINT ( 'NONE',  ( 33.58253175000000113, 72.12500000273119838, -4.112674001490185761E-15 ) ) ;
#5148=CARTESIAN_POINT ( 'NONE',  ( -8.446640517145639571E-15, 78.49999999999998579, 32.49999999999999289 ) ) ;
#5151=CARTESIAN_POINT ( 'NONE',  ( 33.58253175000000113, 58.47500000273119269, -10.91162601494193574 ) ) ;
#5153=CARTESIAN_POINT ( 'NONE',  ( -32.50000000000000000, 40.50000000546238965, 0.000000000000000000 ) ) ;
#5154=CARTESIAN_POINT ( 'NONE',  ( -2.162160676586881955E-15, 10.62500000273119127, -35.31076352940723240 ) ) ;
#5157=CARTESIAN_POINT ( 'NONE',  ( 33.58253175000000113, 4.475000002731182924, -10.91162601494193574 ) ) ;
#5159=CARTESIAN_POINT ( 'NONE',  ( 20.08610463437158344, 45.20000000546238539, 27.64615127144129403 ) ) ;
#5160=LINE ( 'NONE', #26436, #9498 ) ;
#5167=( BOUNDED_CURVE ( )  B_SPLINE_CURVE ( 2, ( #26912, #652, #29316, #32055, #23851, #3246, #5650, #11141, #24349, #13379, #8555, #26753, #28984 ),
 .UNSPECIFIED., .F., .T. ) 
 B_SPLINE_CURVE_WITH_KNOTS ( ( 3, 2, 2, 2, 2, 2, 3 ),
 ( 0.3012820512820512664, 0.3025641025641025439, 0.3051282051282051544, 0.3076923076923077094, 0.3102564102564102644, 0.3128205128205128194, 0.3141025641025640969 ),
 .UNSPECIFIED. ) 
 CURVE ( )  GEOMETRIC_REPRESENTATION_ITEM ( )  RATIONAL_B_SPLINE_CURVE ( ( 0.9755282581475768211, 0.9755282581475768211, 1.000000000000000000, 0.9510565162951535312, 1.000000000000000000, 0.9510565162951535312, 1.000000000000000000, 0.9510565162951535312, 1.000000000000000000, 0.9510565162951535312, 1.000000000000000000, 0.9755282581475768211, 0.9755282581475768211 ) ) 
 REPRESENTATION_ITEM ( '' )  );
#5168=CARTESIAN_POINT ( 'NONE',  ( -1.778240108872766143E-15, 64.00000000546238255, -32.49999999999999289 ) ) ;
#5169=CARTESIAN_POINT ( 'NONE',  ( -32.50000000000000000, 70.50000000546238255, 0.000000000000000000 ) ) ;
#5171=EDGE_CURVE ( 'NONE', #12166, #33526, #21422, .T. ) ;
#5173=( BOUNDED_CURVE ( )  B_SPLINE_CURVE ( 2, ( #4852, #15333, #25788, #1579, #14642, #25102, #12056, #32977, #8265, #5022, #5197, #26130, #197 ),
 .UNSPECIFIED., .F., .T. ) 
 B_SPLINE_CURVE_WITH_KNOTS ( ( 3, 2, 2, 2, 2, 2, 3 ),
 ( 0.7371794871794872250, 0.7384615384615385025, 0.7410256410256410575, 0.7435897435897436125, 0.7461538461538461675, 0.7487179487179487225, 0.7500000000000000000 ),
 .UNSPECIFIED. ) 
 CURVE ( )  GEOMETRIC_REPRESENTATION_ITEM ( )  RATIONAL_B_SPLINE_CURVE ( ( 0.9755282581475768211, 0.9755282581475768211, 1.000000000000000000, 0.9510565162951535312, 1.000000000000000000, 0.9510565162951535312, 1.000000000000000000, 0.9510565162951535312, 1.000000000000000000, 0.9510565162951535312, 1.000000000000000000, 0.9755282581475768211, 0.9755282581475768211 ) ) 
 REPRESENTATION_ITEM ( '' )  );
#5175=VERTEX_POINT ( 'NONE', #14021 ) ;
#5181=CARTESIAN_POINT ( 'NONE',  ( -2.162160676586881955E-15, 50.87500000273119838, -35.31076352940723240 ) ) ;
#5182=CARTESIAN_POINT ( 'NONE',  ( 20.08610463437158344, 59.20000000546237828, 27.64615127144129403 ) ) ;
#5183=CARTESIAN_POINT ( 'NONE',  ( 3.778760231354629433E-15, 2.249999994537632553, -24.50000000000000355 ) ) ;
#5184=CARTESIAN_POINT ( 'NONE',  ( -33.58253175000000113, 45.02500000273117564, -10.91162601494193218 ) ) ;
#5185=CARTESIAN_POINT ( 'NONE',  ( -15.00000000000000000, 72.00000000000001421, 0.000000000000000000 ) ) ;
#5186=CARTESIAN_POINT ( 'NONE',  ( 6.486482029760649416E-15, 69.87500000273121259, 35.31076352940723240 ) ) ;
#5191=CARTESIAN_POINT ( 'NONE',  ( -2.092463501923844636E-15, 49.50000000000001421, -34.17252228774368916 ) ) ;
#5193=CARTESIAN_POINT ( 'NONE',  ( -20.75514604977248823, 9.075000002731183457, -28.56700777964554305 ) ) ;
#5195=CARTESIAN_POINT ( 'NONE',  ( -13.91746824999999532, 79.47500000273117848, 4.522059556121122093 ) ) ;
#5196=CARTESIAN_POINT ( 'NONE',  ( 20.75514604977248467, 76.67500000273116711, -28.56700777964554305 ) ) ;
#5197=CARTESIAN_POINT ( 'NONE',  ( -10.04305231718579172, 21.60000000000000853, -30.90933677959248982 ) ) ;
#5199=ORIENTED_EDGE ( 'NONE', *, *, #13566, .T. ) ;
#5200=CARTESIAN_POINT ( 'NONE',  ( 0.000000000000000000, 80.00000000000001421, 0.000000000000000000 ) ) ;
#5211=CARTESIAN_POINT ( 'NONE',  ( 27.16883889988624290, 37.92500000273118843, 19.73931689729373673 ) ) ;
#5213=DIRECTION ( 'NONE',  ( -0.000000000000000000, 1.000000000000000000, -0.000000000000000000 ) ) ;
#5216=CARTESIAN_POINT ( 'NONE',  ( -2.375766604868041476, 70.69874572391553613, 14.99999999999999822 ) ) ;
#5218=CARTESIAN_POINT ( 'NONE',  ( 27.16883889988623935, 76.57500000273120122, -19.73931689729374384 ) ) ;
#5219=VERTEX_POINT ( 'NONE', #13693 ) ;
#5224=DIRECTION ( 'NONE',  ( 0.000000000000000000, -1.000000000000000000, 0.000000000000000000 ) ) ;
#5225=CARTESIAN_POINT ( 'NONE',  ( 10.37757302488624056, 58.52500000273119696, -31.93888565452638417 ) ) ;
#5229=CARTESIAN_POINT ( 'NONE',  ( -2.162160676586881955E-15, 4.625000002731208149, -35.31076352940723240 ) ) ;
#5230=CARTESIAN_POINT ( 'NONE',  ( -4.635254915624208216, 78.65000000546237402, 14.26584774442730463 ) ) ;
#5232=FACE_OUTER_BOUND ( 'NONE', #22640, .T. ) ;
#5234=CARTESIAN_POINT ( 'NONE',  ( 32.50000000000000000, 75.50000000546236834, -3.980102097228898626E-15 ) ) ;
#5238=CARTESIAN_POINT ( 'NONE',  ( 4.300734207923757602, 80.27500000273118985, -13.23629886949340673 ) ) ;
#5241=CARTESIAN_POINT ( 'NONE',  ( 20.75514604977248467, 30.42500000273117777, -28.56700777964554305 ) ) ;
#5245=CARTESIAN_POINT ( 'NONE',  ( 10.37757302488624056, 14.77500000273118630, -31.93888565452638417 ) ) ;
#5248=CARTESIAN_POINT ( 'NONE',  ( -33.58253175000000113, 73.22500000273117848, 10.91162601494193929 ) ) ;
#5252=CARTESIAN_POINT ( 'NONE',  ( -27.16883889988623935, 63.32500000273119412, 19.73931689729374739 ) ) ;
#5255=CARTESIAN_POINT ( 'NONE',  ( 33.58253175000000823, 6.025000002731191628, 10.91162601494192685 ) ) ;
#5257=CARTESIAN_POINT ( 'NONE',  ( -7.236395654485757944, 3.224999997268801266, -22.27133577429736988 ) ) ;
#5261=ORIENTED_EDGE ( 'NONE', *, *, #32118, .F. ) ;
#5263=CARTESIAN_POINT ( 'NONE',  ( 5.779280353836490358E-15, 30.49999999999999645, 32.49999999999999289 ) ) ;
#5265=FACE_OUTER_BOUND ( 'NONE', #17203, .T. ) ;
#5267=CARTESIAN_POINT ( 'NONE',  ( -19.82091636218621389, 1.200000000000006617, 14.40073868116558842 ) ) ;
#5268=CARTESIAN_POINT ( 'NONE',  ( 33.58253175000000113, 14.47500000273118737, -10.91162601494193751 ) ) ;
#5269=( BOUNDED_CURVE ( )  B_SPLINE_CURVE ( 2, ( #20754, #21423, #27226, #16275, #3059, #8359, #799, #11281, #13694, #5793, #29458, #3720, #19016 ),
 .UNSPECIFIED., .F., .T. ) 
 B_SPLINE_CURVE_WITH_KNOTS ( ( 3, 2, 2, 2, 2, 2, 3 ),
 ( 0.6217948717948718063, 0.6230769230769230838, 0.6256410256410256387, 0.6282051282051281937, 0.6307692307692307487, 0.6333333333333333037, 0.6346153846153845812 ),
 .UNSPECIFIED. ) 
 CURVE ( )  GEOMETRIC_REPRESENTATION_ITEM ( )  RATIONAL_B_SPLINE_CURVE ( ( 0.9755282581475768211, 0.9755282581475768211, 1.000000000000000000, 0.9510565162951535312, 1.000000000000000000, 0.9510565162951535312, 1.000000000000000000, 0.9510565162951535312, 1.000000000000000000, 0.9510565162951535312, 1.000000000000000000, 0.9755282581475768211, 0.9755282581475768211 ) ) 
 REPRESENTATION_ITEM ( '' )  );
#5270=CARTESIAN_POINT ( 'NONE',  ( 32.50000000000000000, 56.99999999999999289, -3.980102097228898626E-15 ) ) ;
#5272=DIRECTION ( 'NONE',  ( 0.000000000000000000, 0.000000000000000000, 1.000000000000000000 ) ) ;
#5274=CARTESIAN_POINT ( 'NONE',  ( -13.91746824999999532, 75.47500000273116427, 4.522059556121122093 ) ) ;
#5276=CARTESIAN_POINT ( 'NONE',  ( 0.000000000000000000, 0.000000000000000000, 24.50000000000000000 ) ) ;
#5277=CARTESIAN_POINT ( 'NONE',  ( -7.570916362186210335, 12.59999999999999964, -23.30088464923126779 ) ) ;
#5278=CARTESIAN_POINT ( 'NONE',  ( -20.08610463437157989, 3.699999999999999289, -27.64615127144129758 ) ) ;
#5279=CARTESIAN_POINT ( 'NONE',  ( 20.08610463437157279, 17.80000000546237615, -27.64615127144129758 ) ) ;
#5282=CARTESIAN_POINT ( 'NONE',  ( -10.37757302488624411, 50.72500000273119980, -31.93888565452638417 ) ) ;
#5284=CARTESIAN_POINT ( 'NONE',  ( -27.16883889988623935, 35.57500000273120122, 19.73931689729374739 ) ) ;
#5288=CARTESIAN_POINT ( 'NONE',  ( -10.04305231718578462, 62.40000000000001279, 30.90933677959249337 ) ) ;
#5290=CARTESIAN_POINT ( 'NONE',  ( -32.50000000000000000, 27.89999999999999147, -10.55989012756945300 ) ) ;
#5292=CARTESIAN_POINT ( 'NONE',  ( -8.601468415847518756, 81.07500000273121543, -11.83890561707634603 ) ) ;
#5293=DIRECTION ( 'NONE',  ( -0.000000000000000000, -1.000000000000000000, -0.000000000000000000 ) ) ;
#5294=CARTESIAN_POINT ( 'NONE',  ( 0.000000000000000000, 80.00000000000001421, 0.000000000000000000 ) ) ;
#5297=FACE_OUTER_BOUND ( 'NONE', #22765, .T. ) ;
#5298=CARTESIAN_POINT ( 'NONE',  ( 27.16883889988624290, 23.92500000273117777, 19.73931689729373673 ) ) ;
#5302=ORIENTED_EDGE ( 'NONE', *, *, #6221, .F. ) ;
#5307=VECTOR ( 'NONE', #15292, 1000.000000000000000 ) ;
#5308=CARTESIAN_POINT ( 'NONE',  ( -20.75514604977248112, 33.67500000273119554, 28.56700777964554661 ) ) ;
#5309=( BOUNDED_CURVE ( )  B_SPLINE_CURVE ( 2, ( #3256, #24191, #7169, #17651, #22124, #17309, #3921, #22618, #2023, #14902, #1330, #25366, #27430 ),
 .UNSPECIFIED., .F., .T. ) 
 B_SPLINE_CURVE_WITH_KNOTS ( ( 3, 2, 2, 2, 2, 2, 3 ),
 ( 0.5277777777777777901, 0.5333333333333333259, 0.5444444444444443976, 0.5555555555555555802, 0.5666666666666666519, 0.5777777777777777235, 0.5833333333333332593 ),
 .UNSPECIFIED. ) 
 CURVE ( )  GEOMETRIC_REPRESENTATION_ITEM ( )  RATIONAL_B_SPLINE_CURVE ( ( 0.9755282581475768211, 0.9755282581475768211, 1.000000000000000000, 0.9510565162951535312, 1.000000000000000000, 0.9510565162951535312, 1.000000000000000000, 0.9510565162951535312, 1.000000000000000000, 0.9510565162951535312, 1.000000000000000000, 0.9755282581475770431, 0.9755282581475768211 ) ) 
 REPRESENTATION_ITEM ( '' )  );
#5310=CARTESIAN_POINT ( 'NONE',  ( -10.04305231718579172, 40.10000000546237686, -30.90933677959248982 ) ) ;
#5311=FACE_OUTER_BOUND ( 'NONE', #33092, .T. ) ;
#5313=CARTESIAN_POINT ( 'NONE',  ( -4.635254915624211769, 81.60000000000000853, -14.26584774442730286 ) ) ;
#5314=CARTESIAN_POINT ( 'NONE',  ( -10.37757302488624411, 46.97500000273119269, -31.93888565452638417 ) ) ;
#5315=AXIS2_PLACEMENT_3D ( 'NONE', #5554, #723, #11209 ) ;
#5318=CARTESIAN_POINT ( 'NONE',  ( -10.04305231718579172, 25.60000000000001208, -30.90933677959248982 ) ) ;
#5320=CARTESIAN_POINT ( 'NONE',  ( 10.37757302488624056, 72.52500000273120406, -31.93888565452638417 ) ) ;
#5323=CARTESIAN_POINT ( 'NONE',  ( 20.75514604977249178, 60.07500000273120122, 28.56700777964553950 ) ) ;
#5324=CARTESIAN_POINT ( 'NONE',  ( 10.04305231718578817, 73.40000000000001990, -30.90933677959249337 ) ) ;
#5325=CARTESIAN_POINT ( 'NONE',  ( 20.75514604977249178, 9.825000002731188786, 28.56700777964553950 ) ) ;
#5328=CARTESIAN_POINT ( 'NONE',  ( 6.486482029760648627E-15, 5.875000002731167292, 35.31076352940722529 ) ) ;
#5330=CARTESIAN_POINT ( 'NONE',  ( 10.04305231718578817, 45.90000000546237402, -30.90933677959249337 ) ) ;
#5338=AXIS2_PLACEMENT_3D ( 'NONE', #15957, #311, #26413 ) ;
#5339=CARTESIAN_POINT ( 'NONE',  ( 32.50000000000000000, 67.50000000546238255, -3.980102097228898626E-15 ) ) ;
#5341=EDGE_CURVE ( 'NONE', #5934, #8435, #14584, .T. ) ;
#5349=CARTESIAN_POINT ( 'NONE',  ( -20.75514604977248112, 53.67500000273119554, 28.56700777964554661 ) ) ;
#5350=CARTESIAN_POINT ( 'NONE',  ( 6.277390505771533514E-15, 57.00000000546238965, 34.17252228774368916 ) ) ;
#5351=DIRECTION ( 'NONE',  ( 0.000000000000000000, -1.000000000000000000, 0.000000000000000000 ) ) ;
#5352=CARTESIAN_POINT ( 'NONE',  ( 20.75514604977249178, 39.82500000273116569, 28.56700777964553950 ) ) ;
#5354=CARTESIAN_POINT ( 'NONE',  ( -2.162160676586881955E-15, 68.87500000273118417, -35.31076352940723240 ) ) ;
#5358=CARTESIAN_POINT ( 'NONE',  ( -20.08610463437157989, 43.69999999999998863, -27.64615127144129758 ) ) ;
#5360=CARTESIAN_POINT ( 'NONE',  ( -33.58253175000000113, 9.475000002731201576, 10.91162601494193929 ) ) ;
#5361=CARTESIAN_POINT ( 'NONE',  ( 7.570916362186207671, 19.34999999453762598, 23.30088464923126779 ) ) ;
#5363=CARTESIAN_POINT ( 'NONE',  ( 8.601468415847516980, 74.67500000273118133, -11.83890561707634781 ) ) ;
#5364=CARTESIAN_POINT ( 'NONE',  ( 2.445080149700053643E-15, 74.75000000546236834, 15.00000000000000000 ) ) ;
#5365=CYLINDRICAL_SURFACE ( 'NONE', #18325, 32.50000000000000000 ) ;
#5374=( BOUNDED_CURVE ( )  B_SPLINE_CURVE ( 2, ( #14802, #22866, #17040, #20129, #6729, #11881, #12568, #33323, #4160, #17726, #14974, #9821, #23039 ),
 .UNSPECIFIED., .F., .F. ) 
 B_SPLINE_CURVE_WITH_KNOTS ( ( 3, 2, 2, 2, 2, 2, 3 ),
 ( 0.9166666666666666297, 0.9179487179487179072, 0.9205128205128204621, 0.9230769230769231282, 0.9256410256410256832, 0.9282051282051282382, 0.9294871794871795156 ),
 .UNSPECIFIED. ) 
 CURVE ( )  GEOMETRIC_REPRESENTATION_ITEM ( )  RATIONAL_B_SPLINE_CURVE ( ( 0.9755282581475768211, 0.9755282581475768211, 1.000000000000000000, 0.9510565162951535312, 1.000000000000000000, 0.9510565162951535312, 1.000000000000000000, 0.9510565162951535312, 1.000000000000000000, 0.9510565162951535312, 1.000000000000000000, 0.9755282581475768211, 0.9755282581475768211 ) ) 
 REPRESENTATION_ITEM ( '' )  );
#5380=CARTESIAN_POINT ( 'NONE',  ( -27.16883889988624290, 40.92500000273119554, -19.73931689729374028 ) ) ;
#5383=EDGE_CURVE ( 'NONE', #20887, #28718, #27305, .T. ) ;
#5384=LINE ( 'NONE', #18773, #8985 ) ;
#5387=CARTESIAN_POINT ( 'NONE',  ( -32.50000000000000000, 2.000000000000001776, 0.000000000000000000 ) ) ;
#5389=CARTESIAN_POINT ( 'NONE',  ( 33.58253175000000113, 74.47500000273116427, -10.91162601494193751 ) ) ;
#5390=ORIENTED_EDGE ( 'NONE', *, *, #32068, .F. ) ;
#5392=EDGE_CURVE ( 'NONE', #1605, #9595, #30811, .T. ) ;
#5394=AXIS2_PLACEMENT_3D ( 'NONE', #7674, #20220, #14893 ) ;
#5395=VERTEX_POINT ( 'NONE', #11941 ) ;
#5396=CARTESIAN_POINT ( 'NONE',  ( 5.779280353836490358E-15, 29.00000000546237544, 32.49999999999999289 ) ) ;
#5397=CARTESIAN_POINT ( 'NONE',  ( -27.16883889988624290, 62.92500000273118843, -19.73931689729374028 ) ) ;
#5399=CARTESIAN_POINT ( 'NONE',  ( 19.82091636218621389, 16.19999999999999218, -14.40073868116559197 ) ) ;
#5400=CARTESIAN_POINT ( 'NONE',  ( 23.41746824999999887, 9.124999997268817609, 0.000000000000000000 ) ) ;
#5401=CARTESIAN_POINT ( 'NONE',  ( 10.37757302488624767, 1.725000002731180704, 31.93888565452638417 ) ) ;
#5402=CARTESIAN_POINT ( 'NONE',  ( -10.37757302488624411, 32.97500000273117848, -31.93888565452638417 ) ) ;
#5404=LINE ( 'NONE', #19125, #17160 ) ;
#5409=CARTESIAN_POINT ( 'NONE',  ( 9.270509831248425314, 72.95000000546238539, 12.75976212528059683 ) ) ;
#5411=CARTESIAN_POINT ( 'NONE',  ( -10.37757302488623701, 23.52500000273119340, 31.93888565452638417 ) ) ;
#5414=CARTESIAN_POINT ( 'NONE',  ( -33.58253175000000113, 15.37500000273117706, 0.000000000000000000 ) ) ;
#5415=CARTESIAN_POINT ( 'NONE',  ( -2.375766604868045029, 79.55125428154684641, -14.99999999999999822 ) ) ;
#5417=CARTESIAN_POINT ( 'NONE',  ( -20.75514604977248823, 76.82500000273120122, -28.56700777964554305 ) ) ;
#5418=CARTESIAN_POINT ( 'NONE',  ( 15.14183272437242067, 7.699999999999988631, 20.84094480462498211 ) ) ;
#5420=CARTESIAN_POINT ( 'NONE',  ( 23.95873412499999944, 0.3124999986344190184, 0.000000000000000000 ) ) ;
#5421=CARTESIAN_POINT ( 'NONE',  ( -10.37757302488624411, 60.72500000273117848, -31.93888565452638417 ) ) ;
#5423=ORIENTED_EDGE ( 'NONE', *, *, #14557, .F. ) ;
#5426=CARTESIAN_POINT ( 'NONE',  ( 23.41746825000000243, 17.22499999726880304, -7.608796670333727974 ) ) ;
#5428=EDGE_LOOP ( 'NONE', ( #13998, #19602, #11131, #16509 ) ) ;
#5437=CARTESIAN_POINT ( 'NONE',  ( 23.41746824999999887, 16.62499999726882294, 0.000000000000000000 ) ) ;
#5438=CARTESIAN_POINT ( 'NONE',  ( 20.75514604977249178, 6.075000002731190563, 28.56700777964553950 ) ) ;
#5439=CARTESIAN_POINT ( 'NONE',  ( -26.29305231718578995, 62.20000000000000284, 19.10302069950538595 ) ) ;
#5440=CARTESIAN_POINT ( 'NONE',  ( -11.25946833292375793, 79.07500000273121543, 8.180482586598737171 ) ) ;
#5441=CARTESIAN_POINT ( 'NONE',  ( -20.08610463437156923, 30.30000000000000426, 27.64615127144130113 ) ) ;
#5443=CARTESIAN_POINT ( 'NONE',  ( -8.601468415847518756, 73.07500000273115859, -11.83890561707634781 ) ) ;
#5446=CARTESIAN_POINT ( 'NONE',  ( -33.58253175000000113, 1.250000002731177506, 0.000000000000000000 ) ) ;
#5447=DIRECTION ( 'NONE',  ( 0.000000000000000000, 0.000000000000000000, 1.000000000000000000 ) ) ;
#5448=CARTESIAN_POINT ( 'NONE',  ( 26.29305231718578995, 3.199999999999980638, -19.10302069950538240 ) ) ;
#5449=CARTESIAN_POINT ( 'NONE',  ( 0.000000000000000000, 80.00000000000001421, 0.000000000000000000 ) ) ;
#5451=CARTESIAN_POINT ( 'NONE',  ( 10.37757302488624056, 48.52500000273118985, -31.93888565452638417 ) ) ;
#5454=CARTESIAN_POINT ( 'NONE',  ( -20.75514604977248112, 31.67500000273119909, 28.56700777964554661 ) ) ;
#5455=CARTESIAN_POINT ( 'NONE',  ( 32.50000000000000000, 23.60000000546236976, -10.55989012756945833 ) ) ;
#5457=CARTESIAN_POINT ( 'NONE',  ( 10.04305231718579705, 15.10000000546238219, 30.90933677959248982 ) ) ;
#5458=CARTESIAN_POINT ( 'NONE',  ( 20.08610463437157279, 51.80000000546237970, -27.64615127144129758 ) ) ;
#5461=CARTESIAN_POINT ( 'NONE',  ( 1.507698388325705758E-15, 1.124999997268814722, -24.62258325217400312 ) ) ;
#5462=CYLINDRICAL_SURFACE ( 'NONE', #31839, 32.50000000000000000 ) ;
#5465=CARTESIAN_POINT ( 'NONE',  ( -26.29305231718578995, 12.19999999999998863, 19.10302069950538595 ) ) ;
#5466=CARTESIAN_POINT ( 'NONE',  ( -10.37757302488624411, 26.72500000273120335, -31.93888565452638417 ) ) ;
#5468=ORIENTED_EDGE ( 'NONE', *, *, #29543, .T. ) ;
#5471=( BOUNDED_CURVE ( )  B_SPLINE_CURVE ( 2, ( #16067, #26523, #3016, #13488, #23953, #422, #10909, #31826, #8319, #29920, #9801, #11729, #20277 ),
 .UNSPECIFIED., .F., .T. ) 
 B_SPLINE_CURVE_WITH_KNOTS ( ( 3, 2, 2, 2, 2, 2, 3 ),
 ( 0.9551282051282051766, 0.9564102564102564541, 0.9589743589743590091, 0.9615384615384615641, 0.9641025641025641191, 0.9666666666666666741, 0.9679487179487179516 ),
 .UNSPECIFIED. ) 
 CURVE ( )  GEOMETRIC_REPRESENTATION_ITEM ( )  RATIONAL_B_SPLINE_CURVE ( ( 0.9755282581475768211, 0.9755282581475768211, 1.000000000000000000, 0.9510565162951535312, 1.000000000000000000, 0.9510565162951535312, 1.000000000000000000, 0.9510565162951535312, 1.000000000000000000, 0.9510565162951535312, 1.000000000000000000, 0.9755282581475768211, 0.9755282581475768211 ) ) 
 REPRESENTATION_ITEM ( '' )  );
#5477=ORIENTED_EDGE ( 'NONE', *, *, #12464, .F. ) ;
#5479=CARTESIAN_POINT ( 'NONE',  ( 27.16883889988623935, 36.57500000273117280, -19.73931689729374384 ) ) ;
#5480=CARTESIAN_POINT ( 'NONE',  ( -20.08610463437157989, 40.20000000546235697, -27.64615127144129758 ) ) ;
#5481=CARTESIAN_POINT ( 'NONE',  ( -20.08610463437157989, 77.70000000000003126, -27.64615127144129758 ) ) ;
#5482=CARTESIAN_POINT ( 'NONE',  ( 32.50000000000000000, 53.09999999999998010, -10.55989012756945833 ) ) ;
#5483=CARTESIAN_POINT ( 'NONE',  ( -12.13525491562421088, 81.79999999999998295, -8.816778784387096835 ) ) ;
#5484=CARTESIAN_POINT ( 'NONE',  ( 33.58253175000000823, 42.27500000273118275, 10.91162601494192863 ) ) ;
#5487=CARTESIAN_POINT ( 'NONE',  ( -2.092463501923844636E-15, 23.49999999999998934, -34.17252228774368916 ) ) ;
#5489=CARTESIAN_POINT ( 'NONE',  ( -33.58253175000000113, 71.22500000273117848, 10.91162601494193929 ) ) ;
#5491=CARTESIAN_POINT ( 'NONE',  ( -10.04305231718579172, 76.10000000546237686, -30.90933677959248982 ) ) ;
#5492=CARTESIAN_POINT ( 'NONE',  ( -10.37757302488623701, 55.77500000273119696, 31.93888565452638417 ) ) ;
#5493=CARTESIAN_POINT ( 'NONE',  ( 32.50000000000000000, 73.09999999999996589, -10.55989012756945833 ) ) ;
#5494=CARTESIAN_POINT ( 'NONE',  ( -27.16883889988624290, 12.92500000273116889, -19.73931689729374028 ) ) ;
#5499=CARTESIAN_POINT ( 'NONE',  ( -2.165007332552593587E-13, 45.00000000546237544, 32.50000000000000000 ) ) ;
#5508=CARTESIAN_POINT ( 'NONE',  ( -2.092463501923844636E-15, 70.00000000546239676, -34.17252228774368916 ) ) ;
#5516=CARTESIAN_POINT ( 'NONE',  ( -32.50000000000000000, 35.89999999999999858, -10.55989012756945300 ) ) ;
#5517=EDGE_CURVE ( 'NONE', #11416, #30585, #12170, .T. ) ;
#5518=CARTESIAN_POINT ( 'NONE',  ( -2.162160676586881955E-15, 56.87500000273117706, -35.31076352940723240 ) ) ;
#5519=EDGE_CURVE ( 'NONE', #23148, #33131, #12379, .T. ) ;
#5520=CARTESIAN_POINT ( 'NONE',  ( 26.29305231718578995, 53.70000000546237828, -19.10302069950538240 ) ) ;
#5522=CARTESIAN_POINT ( 'NONE',  ( 10.37757302488624056, 44.52500000273118275, -31.93888565452638417 ) ) ;
#5523=CARTESIAN_POINT ( 'NONE',  ( 15.00000000000000000, 73.25000000546239676, -1.836970198721029589E-15 ) ) ;
#5524=CARTESIAN_POINT ( 'NONE',  ( -33.58253175000000113, 69.27500000273116143, -10.91162601494193218 ) ) ;
#5525=CARTESIAN_POINT ( 'NONE',  ( 26.29305231718578995, 1.700000005462387609, -19.10302069950538240 ) ) ;
#5528=CARTESIAN_POINT ( 'NONE',  ( -26.29305231718579350, 41.80000000000000426, -19.10302069950537884 ) ) ;
#5530=CARTESIAN_POINT ( 'NONE',  ( -20.75514604977248112, 11.67500000273118843, 28.56700777964554661 ) ) ;
#5531=CARTESIAN_POINT ( 'NONE',  ( 0.000000000000000000, 0.000000000000000000, 0.000000000000000000 ) ) ;
#5533=CARTESIAN_POINT ( 'NONE',  ( 8.601468415847516980, 72.67500000273118133, -11.83890561707634781 ) ) ;
#5534=CARTESIAN_POINT ( 'NONE',  ( 33.58253175000000113, 70.37500000273119838, -4.112674001490185761E-15 ) ) ;
#5535=CARTESIAN_POINT ( 'NONE',  ( 0.000000000000000000, 0.000000000000000000, 0.000000000000000000 ) ) ;
#5537=ORIENTED_EDGE ( 'NONE', *, *, #27607, .T. ) ;
#5538=DIRECTION ( 'NONE',  ( 0.000000000000000000, 0.000000000000000000, -1.000000000000000000 ) ) ;
#5548=CARTESIAN_POINT ( 'NONE',  ( -33.58253175000000113, 41.02500000273118985, -10.91162601494193041 ) ) ;
#5551=CARTESIAN_POINT ( 'NONE',  ( 1.555960095263670572E-15, 6.499999999999994671, -24.50000000000000000 ) ) ;
#5552=ORIENTED_EDGE ( 'NONE', *, *, #32298, .T. ) ;
#5554=CARTESIAN_POINT ( 'NONE',  ( 0.000000000000000000, 0.000000000000000000, 0.000000000000000000 ) ) ;
#5558=CARTESIAN_POINT ( 'NONE',  ( -20.75514604977248823, 69.07500000273115859, -28.56700777964554305 ) ) ;
#5563=LINE ( 'NONE', #8794, #6171 ) ;
#5564=CARTESIAN_POINT ( 'NONE',  ( 20.75514604977249178, 63.82500000273119412, 28.56700777964553950 ) ) ;
#5567=CARTESIAN_POINT ( 'NONE',  ( 23.41746824999999887, 9.224999997268820806, -7.608796670333727974 ) ) ;
#5568=CARTESIAN_POINT ( 'NONE',  ( 10.37757302488624767, 5.725000002731183812, 31.93888565452638417 ) ) ;
#5569=CARTESIAN_POINT ( 'NONE',  ( -33.58253175000000113, 29.47500000273117848, 10.91162601494193929 ) ) ;
#5572=CARTESIAN_POINT ( 'NONE',  ( 10.37757302488624056, 78.77500000273118985, -31.93888565452638417 ) ) ;
#5573=CARTESIAN_POINT ( 'NONE',  ( -11.25946833292375793, 80.67500000273119554, -8.180482586598733619 ) ) ;
#5574=CARTESIAN_POINT ( 'NONE',  ( -32.50000000000000000, 4.099999999999986322, 10.55989012756946366 ) ) ;
#5578=CARTESIAN_POINT ( 'NONE',  ( -8.601468415847515203, 75.17500000273118133, 11.83890561707634959 ) ) ;
#5580=CARTESIAN_POINT ( 'NONE',  ( 6.486482029760649416E-15, 21.62500000273119483, 35.31076352940723240 ) ) ;
#5584=CARTESIAN_POINT ( 'NONE',  ( 20.75514604977248467, 12.67500000273118488, -28.56700777964554305 ) ) ;
#5586=CARTESIAN_POINT ( 'NONE',  ( -33.58253175000000113, 69.02500000273117564, -10.91162601494193041 ) ) ;
#5587=CARTESIAN_POINT ( 'NONE',  ( 32.50000000000000711, 59.40000000546237402, 10.55989012756945122 ) ) ;
#5589=CARTESIAN_POINT ( 'NONE',  ( 12.13525491562421088, 79.05000000546236549, 8.816778784387095058 ) ) ;
#5590=CARTESIAN_POINT ( 'NONE',  ( 33.58253175000000823, 56.02500000273118275, 10.91162601494192685 ) ) ;
#5594=CARTESIAN_POINT ( 'NONE',  ( -10.04305231718579172, 15.60000000000000320, -30.90933677959248982 ) ) ;
#5595=CARTESIAN_POINT ( 'NONE',  ( 14.47279130897151589, 18.82499999726881157, 19.92008829642072953 ) ) ;
#5601=EDGE_LOOP ( 'NONE', ( #33660, #17420, #7311, #18188 ) ) ;
#5603=CARTESIAN_POINT ( 'NONE',  ( 10.04305231718579705, 4.599999999999992539, 30.90933677959248982 ) ) ;
#5607=CARTESIAN_POINT ( 'NONE',  ( -19.82091636218621034, 2.799999999999997158, -14.40073868116559552 ) ) ;
#5608=CARTESIAN_POINT ( 'NONE',  ( -27.16883889988623935, 9.575000002731204773, 19.73931689729374739 ) ) ;
#5609=CARTESIAN_POINT ( 'NONE',  ( -2.092463501923844636E-15, 57.49999999999999289, -34.17252228774368916 ) ) ;
#5610=CARTESIAN_POINT ( 'NONE',  ( 5.147494310547434893, 57.05125428700922896, 32.49999999999999289 ) ) ;
#5613=CARTESIAN_POINT ( 'NONE',  ( -8.601468415847515203, 77.67500000273119554, 11.83890561707634959 ) ) ;
#5616=CARTESIAN_POINT ( 'NONE',  ( 1.836970198721029589E-15, 82.00000000000001421, 15.00000000000000000 ) ) ;
#5617=DIRECTION ( 'NONE',  ( -0.000000000000000000, 1.000000000000000000, -0.000000000000000000 ) ) ;
#5618=CARTESIAN_POINT ( 'NONE',  ( -10.04305231718578462, 2.400000000000013234, 30.90933677959249337 ) ) ;
#5621=CARTESIAN_POINT ( 'NONE',  ( -27.16883889988624290, 42.92500000273119554, -19.73931689729374028 ) ) ;
#5624=CARTESIAN_POINT ( 'NONE',  ( -33.58253175000000113, 37.47500000273118559, 10.91162601494193929 ) ) ;
#5625=CARTESIAN_POINT ( 'NONE',  ( 26.29305231718579350, 23.30000000546236905, 19.10302069950537529 ) ) ;
#5628=CARTESIAN_POINT ( 'NONE',  ( -26.29305231718579350, 44.30000000546238681, -19.10302069950537884 ) ) ;
#5631=CARTESIAN_POINT ( 'NONE',  ( -23.41746825000000243, 1.724999997268824581, 7.608796670333725309 ) ) ;
#5634=LINE ( 'NONE', #12851, #22193 ) ;
#5635=CARTESIAN_POINT ( 'NONE',  ( -20.75514604977248823, 18.82500000273119056, -28.56700777964554305 ) ) ;
#5637=ORIENTED_EDGE ( 'NONE', *, *, #9027, .F. ) ;
#5642=AXIS2_PLACEMENT_3D ( 'NONE', #7175, #27950, #9583 ) ;
#5644=AXIS2_PLACEMENT_3D ( 'NONE', #13633, #565, #13957 ) ;
#5646=CARTESIAN_POINT ( 'NONE',  ( -18.94512977948575738, 1.424999997268805441, -13.76444248337723231 ) ) ;
#5647=CARTESIAN_POINT ( 'NONE',  ( -20.75514604977248112, 29.67500000273119909, 28.56700777964554661 ) ) ;
#5648=CARTESIAN_POINT ( 'NONE',  ( 6.277390505771533514E-15, 39.00000000546236834, 34.17252228774368916 ) ) ;
#5649=CARTESIAN_POINT ( 'NONE',  ( -32.50000000000000000, 76.00000000000001421, 0.000000000000000000 ) ) ;
#5650=CARTESIAN_POINT ( 'NONE',  ( -32.50000000000000000, 54.50000000546237544, 0.000000000000000000 ) ) ;
#5652=CARTESIAN_POINT ( 'NONE',  ( -33.58253175000000113, 45.37500000273120548, 0.000000000000000000 ) ) ;
#5655=CARTESIAN_POINT ( 'NONE',  ( 10.04305231718579705, 22.60000000000000853, 30.90933677959248982 ) ) ;
#5657=CARTESIAN_POINT ( 'NONE',  ( 20.75514604977249178, 63.82500000273119412, 28.56700777964553950 ) ) ;
#5659=CARTESIAN_POINT ( 'NONE',  ( -20.08610463437156923, 76.80000000546239391, 27.64615127144130113 ) ) ;
#5660=CARTESIAN_POINT ( 'NONE',  ( 27.16883889988623935, 52.57500000273118701, -19.73931689729374384 ) ) ;
#5663=CARTESIAN_POINT ( 'NONE',  ( 33.58253175000000823, 12.02500000273117742, 10.91162601494192863 ) ) ;
#5665=EDGE_CURVE ( 'NONE', #13370, #11893, #26017, .T. ) ;
#5670=CARTESIAN_POINT ( 'NONE',  ( 0.000000000000000000, 0.000000000000000000, 0.000000000000000000 ) ) ;
#5677=( BOUNDED_CURVE ( )  B_SPLINE_CURVE ( 2, ( #127, #28969, #28460, #8202, #5465, #21267, #15947, #20588, #26402, #2895, #18692, #33790, #29132 ),
 .UNSPECIFIED., .F., .T. ) 
 B_SPLINE_CURVE_WITH_KNOTS ( ( 3, 2, 2, 2, 2, 2, 3 ),
 ( 0.8653846153846154188, 0.8666666666666666963, 0.8692307692307692513, 0.8717948717948718063, 0.8743589743589743613, 0.8769230769230769162, 0.8782051282051281937 ),
 .UNSPECIFIED. ) 
 CURVE ( )  GEOMETRIC_REPRESENTATION_ITEM ( )  RATIONAL_B_SPLINE_CURVE ( ( 0.9755282581475768211, 0.9755282581475768211, 1.000000000000000000, 0.9510565162951535312, 1.000000000000000000, 0.9510565162951535312, 1.000000000000000000, 0.9510565162951535312, 1.000000000000000000, 0.9510565162951535312, 1.000000000000000000, 0.9755282581475768211, 0.9755282581475768211 ) ) 
 REPRESENTATION_ITEM ( '' )  );
#5680=CARTESIAN_POINT ( 'NONE',  ( 26.29305231718578995, 71.70000000546239960, -19.10302069950538240 ) ) ;
#5688=CARTESIAN_POINT ( 'NONE',  ( 20.08610463437157279, 75.30000000000001137, -27.64615127144129758 ) ) ;
#5689=CARTESIAN_POINT ( 'NONE',  ( -20.75514604977248823, 49.07500000273117280, -28.56700777964554305 ) ) ;
#5690=CARTESIAN_POINT ( 'NONE',  ( 32.50000000000000000, 55.50000000546237544, -3.980102097228898626E-15 ) ) ;
#5692=CARTESIAN_POINT ( 'NONE',  ( 20.75514604977248467, 36.42500000273118843, -28.56700777964554305 ) ) ;
#5694=CARTESIAN_POINT ( 'NONE',  ( -27.16883889988624290, 59.17500000273118133, -19.73931689729374028 ) ) ;
#5695=CARTESIAN_POINT ( 'NONE',  ( 10.04305231718579705, 1.100000005462370423, 30.90933677959248982 ) ) ;
#5699=CARTESIAN_POINT ( 'NONE',  ( -10.04305231718579172, 39.59999999999999432, -30.90933677959248982 ) ) ;
#5701=CARTESIAN_POINT ( 'NONE',  ( 33.58253175000000113, 8.375000002731169957, -4.112674001490185761E-15 ) ) ;
#5704=CARTESIAN_POINT ( 'NONE',  ( 6.486482029760648627E-15, 75.87500000273119838, 35.31076352940722529 ) ) ;
#5705=CARTESIAN_POINT ( 'NONE',  ( 0.000000000000000000, 82.00000000000001421, 0.000000000000000000 ) ) ;
#5709=DIRECTION ( 'NONE',  ( -0.000000000000000000, -1.000000000000000000, -0.000000000000000000 ) ) ;
#5720=CARTESIAN_POINT ( 'NONE',  ( 10.37757302488624767, 39.72500000273118559, 31.93888565452638417 ) ) ;
#5724=ORIENTED_EDGE ( 'NONE', *, *, #19597, .T. ) ;
#5728=CARTESIAN_POINT ( 'NONE',  ( 33.58253175000000113, 70.47500000273117848, -10.91162601494193751 ) ) ;
#5729=ORIENTED_EDGE ( 'NONE', *, *, #26149, .T. ) ;
#5732=ORIENTED_EDGE ( 'NONE', *, *, #32911, .T. ) ;
#5733=CARTESIAN_POINT ( 'NONE',  ( -10.04305231718579172, 48.10000000546238397, -30.90933677959248982 ) ) ;
#5734=CARTESIAN_POINT ( 'NONE',  ( 20.75514604977249178, 55.82500000273119412, 28.56700777964553950 ) ) ;
#5736=CARTESIAN_POINT ( 'NONE',  ( -20.08610463437157989, 16.20000000546237118, -27.64615127144129758 ) ) ;
#5738=CARTESIAN_POINT ( 'NONE',  ( -4.523095164977117273E-15, 6.624999997268815832, 24.62258325217400312 ) ) ;
#5740=CARTESIAN_POINT ( 'NONE',  ( -20.75514604977248112, 27.67500000273118133, 28.56700777964554661 ) ) ;
#5742=CARTESIAN_POINT ( 'NONE',  ( 8.601468415847516980, 80.17500000273116711, -11.83890561707634781 ) ) ;
#5743=CARTESIAN_POINT ( 'NONE',  ( -5.147494310547430452, 3.551254281546844194, -32.49999999999999289 ) ) ;
#5747=CARTESIAN_POINT ( 'NONE',  ( 4.300734207923757602, 72.27500000273117564, -13.23629886949340673 ) ) ;
#5749=CARTESIAN_POINT ( 'NONE',  ( 20.75514604977248467, 26.42500000273118843, -28.56700777964554305 ) ) ;
#5752=CARTESIAN_POINT ( 'NONE',  ( -20.75514604977248823, 13.07500000273120300, -28.56700777964554305 ) ) ;
#5754=CARTESIAN_POINT ( 'NONE',  ( -33.58253175000000113, 69.12500000273119838, 0.000000000000000000 ) ) ;
#5757=CARTESIAN_POINT ( 'NONE',  ( -12.13525491562421088, 72.05000000546237970, -8.816778784387096835 ) ) ;
#5758=CARTESIAN_POINT ( 'NONE',  ( -2.162160676586882350E-15, 56.62500000273116996, -35.31076352940722529 ) ) ;
#5760=VECTOR ( 'NONE', #14913, 1000.000000000000000 ) ;
#5761=ORIENTED_EDGE ( 'NONE', *, *, #25175, .T. ) ;
#5763=CARTESIAN_POINT ( 'NONE',  ( -10.37757302488623701, 3.525000002731204507, 31.93888565452638417 ) ) ;
#5764=CARTESIAN_POINT ( 'NONE',  ( 1.507698388325705758E-15, 7.124999997268799845, -24.62258325217400312 ) ) ;
#5768=CARTESIAN_POINT ( 'NONE',  ( -1.778240108872766143E-15, 42.00000000546236834, -32.49999999999999289 ) ) ;
#5771=CARTESIAN_POINT ( 'NONE',  ( 20.08610463437158344, 4.699999999999996625, 27.64615127144129403 ) ) ;
#5772=CARTESIAN_POINT ( 'NONE',  ( -24.50000000000000000, 3.000000000000002665, -3.000384657911015469E-15 ) ) ;
#5773=CARTESIAN_POINT ( 'NONE',  ( -20.75514604977248112, 75.42500000273120975, 28.56700777964554661 ) ) ;
#5775=CARTESIAN_POINT ( 'NONE',  ( 14.47279130897151589, 18.32499999726882578, 19.92008829642072953 ) ) ;
#5776=CARTESIAN_POINT ( 'NONE',  ( 27.16883889988623935, 6.575000002731201221, -19.73931689729374384 ) ) ;
#5777=CARTESIAN_POINT ( 'NONE',  ( 27.16883889988624290, 21.92500000273117777, 19.73931689729373673 ) ) ;
#5778=CARTESIAN_POINT ( 'NONE',  ( 13.91746825000000065, 77.77500000273118985, 4.522059556121115875 ) ) ;
#5781=CARTESIAN_POINT ( 'NONE',  ( 13.91746824999999532, 74.47500000273116427, -4.522059556121118540 ) ) ;
#5786=CARTESIAN_POINT ( 'NONE',  ( 33.58253175000000823, 44.02500000273118275, 10.91162601494192863 ) ) ;
#5789=CARTESIAN_POINT ( 'NONE',  ( -20.75514604977248112, 33.67500000273119554, 28.56700777964554661 ) ) ;
#5792=DIRECTION ( 'NONE',  ( -0.000000000000000000, -1.000000000000000000, -0.000000000000000000 ) ) ;
#5793=CARTESIAN_POINT ( 'NONE',  ( 20.08610463437158344, 30.69999999999999218, 27.64615127144129403 ) ) ;
#5796=CARTESIAN_POINT ( 'NONE',  ( -23.41746824999999887, 3.624999997268813168, -2.867812753649727150E-15 ) ) ;
#5797=AXIS2_PLACEMENT_3D ( 'NONE', #26353, #33739, #21048 ) ;
#5798=EDGE_CURVE ( 'NONE', #21432, #28216, #28339, .T. ) ;
#5801=CARTESIAN_POINT ( 'NONE',  ( -5.147494310547423346, 60.44874571845313938, 32.50000000000000000 ) ) ;
#5802=CARTESIAN_POINT ( 'NONE',  ( -2.162160676586882350E-15, 22.62500000273119127, -35.31076352940722529 ) ) ;
#5804=EDGE_CURVE ( 'NONE', #8435, #13370, #10887, .T. ) ;
#5805=VERTEX_POINT ( 'NONE', #17240 ) ;
#5808=ORIENTED_EDGE ( 'NONE', *, *, #29497, .F. ) ;
#5812=EDGE_CURVE ( 'NONE', #10957, #6411, #32116, .T. ) ;
#5813=ORIENTED_EDGE ( 'NONE', *, *, #3983, .T. ) ;
#5814=CYLINDRICAL_SURFACE ( 'NONE', #16323, 24.50000000000000000 ) ;
#5815=CARTESIAN_POINT ( 'NONE',  ( 20.75514604977248467, 30.67500000273119909, -28.56700777964554305 ) ) ;
#5816=CARTESIAN_POINT ( 'NONE',  ( 6.277390505771533514E-15, 33.00000000546238255, 34.17252228774368916 ) ) ;
#5818=CARTESIAN_POINT ( 'NONE',  ( -32.50000000000000000, 78.10000000000000853, 10.55989012756946366 ) ) ;
#5820=CARTESIAN_POINT ( 'NONE',  ( -3.880418787951099180, 10.55125428154683753, -24.50000000000001421 ) ) ;
#5821=CARTESIAN_POINT ( 'NONE',  ( -27.16883889988623935, 45.57500000273117990, 19.73931689729374739 ) ) ;
#5823=CARTESIAN_POINT ( 'NONE',  ( 20.08610463437157279, 19.30000000000000426, -27.64615127144129758 ) ) ;
#5825=CARTESIAN_POINT ( 'NONE',  ( 33.58253175000000113, 60.22500000273119980, -10.91162601494193751 ) ) ;
#5828=CARTESIAN_POINT ( 'NONE',  ( 20.75514604977249178, 54.07500000273118701, 28.56700777964553950 ) ) ;
#5831=CARTESIAN_POINT ( 'NONE',  ( -33.58253175000000113, 3.025000002731199622, -10.91162601494193218 ) ) ;
#5844=ORIENTED_EDGE ( 'NONE', *, *, #21954, .T. ) ;
#5845=CARTESIAN_POINT ( 'NONE',  ( 32.50000000000000711, 69.40000000546235981, 10.55989012756945122 ) ) ;
#5848=ORIENTED_EDGE ( 'NONE', *, *, #27277, .T. ) ;
#5852=CARTESIAN_POINT ( 'NONE',  ( 32.50000000000000711, 74.89999999999999147, 10.55989012756945122 ) ) ;
#5853=CARTESIAN_POINT ( 'NONE',  ( -33.58253175000000113, 45.37500000273120548, 0.000000000000000000 ) ) ;
#5854=CARTESIAN_POINT ( 'NONE',  ( 20.08610463437157279, 49.80000000546238681, -27.64615127144129758 ) ) ;
#5855=EDGE_CURVE ( 'NONE', #12435, #14813, #32666, .T. ) ;
#5857=CARTESIAN_POINT ( 'NONE',  ( -20.75514604977248112, 33.42500000273120264, 28.56700777964554661 ) ) ;
#5859=CARTESIAN_POINT ( 'NONE',  ( 20.75514604977248467, 60.67500000273118133, -28.56700777964554305 ) ) ;
#5860=CARTESIAN_POINT ( 'NONE',  ( 6.277390505771533514E-15, 1.000000005462384323, 34.17252228774368916 ) ) ;
#5862=CARTESIAN_POINT ( 'NONE',  ( -10.04305231718579172, 41.60000000000000142, -30.90933677959248982 ) ) ;
#5864=CARTESIAN_POINT ( 'NONE',  ( 27.16883889988623935, 2.575000002731198112, -19.73931689729374384 ) ) ;
#5866=CARTESIAN_POINT ( 'NONE',  ( -8.601468415847515203, 73.67500000273120975, 11.83890561707634959 ) ) ;
#5867=CARTESIAN_POINT ( 'NONE',  ( 20.75514604977249178, 76.07500000273118701, 28.56700777964553950 ) ) ;
#5868=CARTESIAN_POINT ( 'NONE',  ( -19.82091636218621389, 18.94999999453761319, 14.40073868116558842 ) ) ;
#5874=DIRECTION ( 'NONE',  ( -0.000000000000000000, -1.000000000000000000, -0.000000000000000000 ) ) ;
#5880=VECTOR ( 'NONE', #24867, 1000.000000000000000 ) ;
#5884=CARTESIAN_POINT ( 'NONE',  ( 10.37757302488624767, 35.72500000273118559, 31.93888565452638417 ) ) ;
#5890=CARTESIAN_POINT ( 'NONE',  ( -10.04305231718579172, 50.10000000546238397, -30.90933677959248982 ) ) ;
#5892=CARTESIAN_POINT ( 'NONE',  ( 6.486482029760649416E-15, 67.87500000273116996, 35.31076352940723240 ) ) ;
#5893=VERTEX_POINT ( 'NONE', #3686 ) ;
#5896=VERTEX_POINT ( 'NONE', #14834 ) ;
#5898=CARTESIAN_POINT ( 'NONE',  ( 33.58253175000000113, 56.12500000273118417, -4.112674001490185761E-15 ) ) ;
#5902=CARTESIAN_POINT ( 'NONE',  ( -20.08610463437156923, 16.80000000546237970, 27.64615127144130113 ) ) ;
#5903=CARTESIAN_POINT ( 'NONE',  ( 7.570916362186207671, 15.34999999453762243, 23.30088464923126779 ) ) ;
#5904=CARTESIAN_POINT ( 'NONE',  ( -4.523095164977117273E-15, 10.62499999726880517, 24.62258325217400312 ) ) ;
#5905=CARTESIAN_POINT ( 'NONE',  ( -33.58253175000000113, 25.47500000273118914, 10.91162601494193929 ) ) ;
#5908=CARTESIAN_POINT ( 'NONE',  ( 13.91746824999999887, 79.87500000273118417, -1.704398294459741270E-15 ) ) ;
#5909=CARTESIAN_POINT ( 'NONE',  ( -26.29305231718578995, 34.20000000000000995, 19.10302069950538595 ) ) ;
#5911=ORIENTED_EDGE ( 'NONE', *, *, #26858, .T. ) ;
#5913=CARTESIAN_POINT ( 'NONE',  ( 8.601468415847516980, 78.17500000273118133, -11.83890561707634781 ) ) ;
#5915=CARTESIAN_POINT ( 'NONE',  ( -20.75514604977248823, 26.82500000273117280, -28.56700777964554305 ) ) ;
#5919=CARTESIAN_POINT ( 'NONE',  ( 20.75514604977248467, 14.67500000273117955, -28.56700777964554305 ) ) ;
#5921=CARTESIAN_POINT ( 'NONE',  ( 27.16883889988624290, 69.92500000273119554, 19.73931689729373673 ) ) ;
#5922=FACE_OUTER_BOUND ( 'NONE', #29848, .T. ) ;
#5923=CARTESIAN_POINT ( 'NONE',  ( -4.300734207923759378, 76.97500000273119269, -13.23629886949340495 ) ) ;
#5925=CARTESIAN_POINT ( 'NONE',  ( 3.980102097228898626E-15, 80.00000000000001421, 32.50000000000000000 ) ) ;
#5926=CARTESIAN_POINT ( 'NONE',  ( -27.16883889988624290, 54.92500000273120264, -19.73931689729374028 ) ) ;
#5932=CARTESIAN_POINT ( 'NONE',  ( 18.94512977948576093, 6.824999997268821339, -13.76444248337722875 ) ) ;
#5934=VERTEX_POINT ( 'NONE', #32831 ) ;
#5936=VERTEX_POINT ( 'NONE', #27875 ) ;
#5939=CARTESIAN_POINT ( 'NONE',  ( 10.37757302488624056, 76.52500000273118985, -31.93888565452638417 ) ) ;
#5941=CARTESIAN_POINT ( 'NONE',  ( 1.577395562988744260E-15, 6.499999999999998224, -25.76082449383753925 ) ) ;
#5942=ADVANCED_FACE ( 'NONE', ( #14160 ), #9321, .T. ) ;
#5943=CARTESIAN_POINT ( 'NONE',  ( -20.75514604977248823, 9.075000002731183457, -28.56700777964554305 ) ) ;
#5944=ADVANCED_FACE ( 'NONE', ( #9161 ), #1769, .T. ) ;
#5945=CARTESIAN_POINT ( 'NONE',  ( 6.486482029760649416E-15, 13.62500000273118417, 35.31076352940723240 ) ) ;
#5946=CARTESIAN_POINT ( 'NONE',  ( -8.960552108402744065E-16, 80.37500000273116996, -14.63369212191046209 ) ) ;
#5947=CARTESIAN_POINT ( 'NONE',  ( 0.000000000000000000, 80.00000000000001421, 0.000000000000000000 ) ) ;
#5949=CARTESIAN_POINT ( 'NONE',  ( -4.635254915624208216, 78.39999999999999147, 14.26584774442730463 ) ) ;
#5953=CARTESIAN_POINT ( 'NONE',  ( -20.75514604977248823, 44.82500000273117990, -28.56700777964554305 ) ) ;
#5956=CARTESIAN_POINT ( 'NONE',  ( 10.37757302488624056, 32.77500000273120406, -31.93888565452638417 ) ) ;
#5960=ADVANCED_FACE ( 'NONE', ( #22727 ), #11573, .T. ) ;
#5964=CARTESIAN_POINT ( 'NONE',  ( 14.47279130897151767, 4.324999997268800911, 19.92008829642072953 ) ) ;
#5965=LINE ( 'NONE', #1124, #25328 ) ;
#5967=( BOUNDED_CURVE ( )  B_SPLINE_CURVE ( 2, ( #14739, #15255, #9403, #19719, #30166, #6670, #27608, #30339, #11985, #17317, #1678, #25200, #22627 ),
 .UNSPECIFIED., .F., .T. ) 
 B_SPLINE_CURVE_WITH_KNOTS ( ( 3, 2, 2, 2, 2, 2, 3 ),
 ( 0.4679487179487179516, 0.4692307692307692291, 0.4717948717948717841, 0.4743589743589743390, 0.4769230769230769496, 0.4794871794871795045, 0.4807692307692307820 ),
 .UNSPECIFIED. ) 
 CURVE ( )  GEOMETRIC_REPRESENTATION_ITEM ( )  RATIONAL_B_SPLINE_CURVE ( ( 0.9755282581475768211, 0.9755282581475768211, 1.000000000000000000, 0.9510565162951535312, 1.000000000000000000, 0.9510565162951535312, 1.000000000000000000, 0.9510565162951535312, 1.000000000000000000, 0.9510565162951535312, 1.000000000000000000, 0.9755282581475768211, 0.9755282581475768211 ) ) 
 REPRESENTATION_ITEM ( '' )  );
#5969=CARTESIAN_POINT ( 'NONE',  ( 27.16883889988623935, 18.32500000273118346, -19.73931689729374384 ) ) ;
#5970=CARTESIAN_POINT ( 'NONE',  ( -18.94512977948576093, 8.324999997268822227, 13.76444248337722698 ) ) ;
#5978=CARTESIAN_POINT ( 'NONE',  ( -23.41746825000000243, 7.524999997268816188, -7.608796670333730638 ) ) ;
#5979=CARTESIAN_POINT ( 'NONE',  ( -10.37757302488623701, 29.77500000273120051, 31.93888565452638417 ) ) ;
#5980=CARTESIAN_POINT ( 'NONE',  ( -20.08610463437156923, 28.80000000546238326, 27.64615127144130113 ) ) ;
#5981=CARTESIAN_POINT ( 'NONE',  ( 32.50000000000000000, 77.09999999999998010, -10.55989012756945833 ) ) ;
#5982=CARTESIAN_POINT ( 'NONE',  ( 20.08610463437158344, 52.69999999999998863, 27.64615127144129403 ) ) ;
#5983=DIRECTION ( 'NONE',  ( -0.000000000000000000, -1.000000000000000000, -0.000000000000000000 ) ) ;
#5984=CARTESIAN_POINT ( 'NONE',  ( -33.58253175000000113, 43.27500000273117564, -10.91162601494193218 ) ) ;
#5986=CARTESIAN_POINT ( 'NONE',  ( 20.08610463437158344, 18.69999999999998863, 27.64615127144129403 ) ) ;
#5988=CARTESIAN_POINT ( 'NONE',  ( 33.58253175000000823, 66.02500000273118985, 10.91162601494192863 ) ) ;
#5989=CARTESIAN_POINT ( 'NONE',  ( -33.58253175000000113, 55.37500000273118417, 0.000000000000000000 ) ) ;
#5991=ADVANCED_FACE ( 'NONE', ( #33176 ), #1090, .T. ) ;
#5992=CARTESIAN_POINT ( 'NONE',  ( 26.29305231718579350, 39.30000000546237970, 19.10302069950537529 ) ) ;
#5993=CARTESIAN_POINT ( 'NONE',  ( -2.162160676586881955E-15, 8.625000002731169957, -35.31076352940723240 ) ) ;
#5998=CARTESIAN_POINT ( 'NONE',  ( -10.04305231718579172, 18.10000000546238397, -30.90933677959248982 ) ) ;
#5999=CARTESIAN_POINT ( 'NONE',  ( -1.778240108872766143E-15, 39.50000000000000000, -32.49999999999999289 ) ) ;
#6000=EDGE_CURVE ( 'NONE', #16286, #19940, #15709, .T. ) ;
#6001=CARTESIAN_POINT ( 'NONE',  ( -26.29305231718578995, 30.70000000546238539, 19.10302069950538595 ) ) ;
#6005=FACE_OUTER_BOUND ( 'NONE', #24619, .T. ) ;
#6015=CARTESIAN_POINT ( 'NONE',  ( 0.000000000000000000, 82.00000000000001421, -15.00000000000000000 ) ) ;
#6016=CARTESIAN_POINT ( 'NONE',  ( 33.58253175000000113, 44.47500000273119269, -10.91162601494193751 ) ) ;
#6017=CARTESIAN_POINT ( 'NONE',  ( 20.08610463437157279, 51.80000000546238681, -27.64615127144129758 ) ) ;
#6019=CARTESIAN_POINT ( 'NONE',  ( 27.16883889988624290, 33.92500000273118843, 19.73931689729373673 ) ) ;
#6021=CARTESIAN_POINT ( 'NONE',  ( -27.16883889988624290, 61.17500000273118133, -19.73931689729374028 ) ) ;
#6022=CARTESIAN_POINT ( 'NONE',  ( -2.092463501923844636E-15, 41.49999999999999289, -34.17252228774368916 ) ) ;
#6024=CARTESIAN_POINT ( 'NONE',  ( -27.16883889988624290, 7.175000002731191096, -19.73931689729374028 ) ) ;
#6025=CARTESIAN_POINT ( 'NONE',  ( -1.778240108872766143E-15, 13.50000000000000355, -32.49999999999999289 ) ) ;
#6026=CARTESIAN_POINT ( 'NONE',  ( -11.25946833292375793, 73.17500000273119554, -8.180482586598733619 ) ) ;
#6027=CARTESIAN_POINT ( 'NONE',  ( -2.162160676586882350E-15, 70.87500000273118417, -35.31076352940722529 ) ) ;
#6030=EDGE_LOOP ( 'NONE', ( #6257, #20026, #21017, #16041 ) ) ;
#6031=CARTESIAN_POINT ( 'NONE',  ( -19.82091636218621389, 6.949999994537630954, 14.40073868116558842 ) ) ;
#6043=CARTESIAN_POINT ( 'NONE',  ( 5.779280353836490358E-15, 58.49999999999999289, 32.49999999999999289 ) ) ;
#6044=VERTEX_POINT ( 'NONE', #15005 ) ;
#6046=LINE ( 'NONE', #10537, #22310 ) ;
#6048=CARTESIAN_POINT ( 'NONE',  ( 20.75514604977248467, 66.67500000273119554, -28.56700777964554305 ) ) ;
#6052=EDGE_LOOP ( 'NONE', ( #5813, #19315, #32477, #20167 ) ) ;
#6054=CARTESIAN_POINT ( 'NONE',  ( 33.58253175000000823, 54.02500000273118275, 10.91162601494192863 ) ) ;
#6056=CARTESIAN_POINT ( 'NONE',  ( -26.29305231718578995, 12.70000000546239782, 19.10302069950538595 ) ) ;
#6057=CARTESIAN_POINT ( 'NONE',  ( -10.04305231718579172, 66.10000000546237686, -30.90933677959248982 ) ) ;
#6058=CARTESIAN_POINT ( 'NONE',  ( -7.236395654485757944, 11.72499999726880837, -22.27133577429736988 ) ) ;
#6059=( BOUNDED_CURVE ( )  B_SPLINE_CURVE ( 2, ( #21452, #13048, #26426, #5659, #10473, #10978, #16142, #20951, #29153, #23860, #5491, #8223, #2919 ),
 .UNSPECIFIED., .F., .T. ) 
 B_SPLINE_CURVE_WITH_KNOTS ( ( 3, 2, 2, 2, 2, 2, 3 ),
 ( 0.01923076923076923184, 0.02051282051282051280, 0.02307692307692307820, 0.02564102564102564014, 0.02820512820512820554, 0.03076923076923077094, 0.03205128205128205537 ),
 .UNSPECIFIED. ) 
 CURVE ( )  GEOMETRIC_REPRESENTATION_ITEM ( )  RATIONAL_B_SPLINE_CURVE ( ( 0.9755282581475768211, 0.9755282581475768211, 1.000000000000000000, 0.9510565162951535312, 1.000000000000000000, 0.9510565162951535312, 1.000000000000000000, 0.9510565162951535312, 1.000000000000000000, 0.9510565162951535312, 1.000000000000000000, 0.9755282581475767101, 0.9755282581475768211 ) ) 
 REPRESENTATION_ITEM ( '' )  );
#6060=CARTESIAN_POINT ( 'NONE',  ( 20.75514604977248467, 20.67500000273119909, -28.56700777964554305 ) ) ;
#6061=CARTESIAN_POINT ( 'NONE',  ( 9.270509831248421762, 77.30000000000001137, -12.75976212528059861 ) ) ;
#6063=CARTESIAN_POINT ( 'NONE',  ( -32.50000000000000000, 31.90000000000001279, -10.55989012756945300 ) ) ;
#6064=CARTESIAN_POINT ( 'NONE',  ( 32.50000000000000000, 15.00000000000001421, -3.980102097228898626E-15 ) ) ;
#6066=EDGE_LOOP ( 'NONE', ( #24212, #28178, #1818, #30429 ) ) ;
#6068=CARTESIAN_POINT ( 'NONE',  ( 11.25946833292375793, 76.07500000273120122, -8.180482586598735395 ) ) ;
#6070=CARTESIAN_POINT ( 'NONE',  ( 33.58253175000000823, 26.02500000273120406, 10.91162601494192863 ) ) ;
#6074=CARTESIAN_POINT ( 'NONE',  ( -20.75514604977248823, 9.075000002731183457, -28.56700777964554305 ) ) ;
#6076=CARTESIAN_POINT ( 'NONE',  ( -33.58253175000000113, 71.12500000273119838, 0.000000000000000000 ) ) ;
#6080=CARTESIAN_POINT ( 'NONE',  ( -8.601468415847515203, 77.67500000273119554, 11.83890561707634959 ) ) ;
#6083=CARTESIAN_POINT ( 'NONE',  ( 20.75514604977249178, 57.82500000273119412, 28.56700777964553950 ) ) ;
#6084=EDGE_CURVE ( 'NONE', #22217, #28718, #4700, .T. ) ;
#6086=ORIENTED_EDGE ( 'NONE', *, *, #3699, .T. ) ;
#6088=CARTESIAN_POINT ( 'NONE',  ( 6.486482029760648627E-15, 3.625000002731181059, 35.31076352940722529 ) ) ;
#6089=CARTESIAN_POINT ( 'NONE',  ( -23.41746824999999887, 5.624999997268814944, -2.867812753649727150E-15 ) ) ;
#6091=EDGE_LOOP ( 'NONE', ( #31801, #8832, #9717, #730 ) ) ;
#6093=CARTESIAN_POINT ( 'NONE',  ( -1.778240108872766143E-15, 55.49999999999999289, -32.49999999999999289 ) ) ;
#6095=ORIENTED_EDGE ( 'NONE', *, *, #9343, .T. ) ;
#6098=DIRECTION ( 'NONE',  ( 0.000000000000000000, 1.000000000000000000, 0.000000000000000000 ) ) ;
#6099=CARTESIAN_POINT ( 'NONE',  ( 33.58253175000000823, 72.02500000273118985, 10.91162601494192863 ) ) ;
#6101=CARTESIAN_POINT ( 'NONE',  ( 7.570916362186213000, 8.399999999999991473, -23.30088464923126423 ) ) ;
#6102=CARTESIAN_POINT ( 'NONE',  ( 6.486482029760649416E-15, 11.87500000273118062, 35.31076352940723240 ) ) ;
#6103=CARTESIAN_POINT ( 'NONE',  ( -33.58253175000000113, 17.02500000273118985, -10.91162601494193218 ) ) ;
#6104=CARTESIAN_POINT ( 'NONE',  ( 8.601468415847520532, 75.57500000273120122, 11.83890561707634603 ) ) ;
#6108=CARTESIAN_POINT ( 'NONE',  ( 8.601468415847516980, 72.67500000273118133, -11.83890561707634781 ) ) ;
#6112=CARTESIAN_POINT ( 'NONE',  ( -2.162160676586881955E-15, 46.62500000273119127, -35.31076352940723240 ) ) ;
#6115=CARTESIAN_POINT ( 'NONE',  ( -33.58253175000000113, 31.37500000273119127, 0.000000000000000000 ) ) ;
#6116=LINE ( 'NONE', #11767, #18567 ) ;
#6118=CARTESIAN_POINT ( 'NONE',  ( 6.001560367445586717E-15, 1.500000000000005995, 24.50000000000000000 ) ) ;
#6119=EDGE_CURVE ( 'NONE', #6044, #5934, #12427, .T. ) ;
#6120=CARTESIAN_POINT ( 'NONE',  ( -4.635254915624208216, 76.40000000000001990, 14.26584774442730463 ) ) ;
#6123=CARTESIAN_POINT ( 'NONE',  ( -18.94512977948576093, 5.824999997268820451, 13.76444248337722698 ) ) ;
#6126=CARTESIAN_POINT ( 'NONE',  ( -32.50000000000000000, 59.89999999999999147, -10.55989012756945300 ) ) ;
#6127=CARTESIAN_POINT ( 'NONE',  ( -10.37757302488623701, 19.52500000273118985, 31.93888565452638417 ) ) ;
#6128=CARTESIAN_POINT ( 'NONE',  ( -23.41746825000000243, 4.024999997268810858, -7.608796670333730638 ) ) ;
#6132=ORIENTED_EDGE ( 'NONE', *, *, #19308, .T. ) ;
#6137=CARTESIAN_POINT ( 'NONE',  ( 1.507698388325705758E-15, 3.124999997268809615, -24.62258325217400312 ) ) ;
#6138=CARTESIAN_POINT ( 'NONE',  ( 6.486482029760649416E-15, 29.87500000273119838, 35.31076352940723240 ) ) ;
#6139=CARTESIAN_POINT ( 'NONE',  ( -10.04305231718579172, 32.10000000546236976, -30.90933677959248982 ) ) ;
#6140=CARTESIAN_POINT ( 'NONE',  ( -26.29305231718579350, 71.79999999999999716, -19.10302069950537884 ) ) ;
#6142=CYLINDRICAL_SURFACE ( 'NONE', #32382, 32.50000000000000000 ) ;
#6144=CARTESIAN_POINT ( 'NONE',  ( -20.75514604977248112, 41.67500000273117422, 28.56700777964554661 ) ) ;
#6145=CARTESIAN_POINT ( 'NONE',  ( 1.507698388325705758E-15, 11.62499999726880340, -24.62258325217400312 ) ) ;
#6146=CARTESIAN_POINT ( 'NONE',  ( -26.29305231718578995, 18.19999999999999574, 19.10302069950538595 ) ) ;
#6149=CARTESIAN_POINT ( 'NONE',  ( -20.75514604977248112, 65.42500000273118133, 28.56700777964554661 ) ) ;
#6150=CARTESIAN_POINT ( 'NONE',  ( 10.37757302488624767, 53.97500000273119980, 31.93888565452638417 ) ) ;
#6151=VECTOR ( 'NONE', #5983, 1000.000000000000000 ) ;
#6153=CARTESIAN_POINT ( 'NONE',  ( 5.779280353836490358E-15, 39.00000000546237544, 32.49999999999999289 ) ) ;
#6154=CARTESIAN_POINT ( 'NONE',  ( -20.75514604977248823, 6.825000002731195892, -28.56700777964554305 ) ) ;
#6156=( BOUNDED_CURVE ( )  B_SPLINE_CURVE ( 2, ( #5168, #10153, #15478, #10489, #17709, #20635, #33479, #9980, #2425, #23368, #18394, #25763, #13062 ),
 .UNSPECIFIED., .F., .T. ) 
 B_SPLINE_CURVE_WITH_KNOTS ( ( 3, 2, 2, 2, 2, 2, 3 ),
 ( 0.1858974358974359031, 0.1871794871794871806, 0.1897435897435897356, 0.1923076923076923184, 0.1948717948717948734, 0.1974358974358974284, 0.1987179487179487336 ),
 .UNSPECIFIED. ) 
 CURVE ( )  GEOMETRIC_REPRESENTATION_ITEM ( )  RATIONAL_B_SPLINE_CURVE ( ( 0.9755282581475768211, 0.9755282581475768211, 1.000000000000000000, 0.9510565162951535312, 1.000000000000000000, 0.9510565162951535312, 1.000000000000000000, 0.9510565162951535312, 1.000000000000000000, 0.9510565162951535312, 1.000000000000000000, 0.9755282581475764880, 0.9755282581475768211 ) ) 
 REPRESENTATION_ITEM ( '' )  );
#6157=FACE_OUTER_BOUND ( 'NONE', #6091, .T. ) ;
#6158=CYLINDRICAL_SURFACE ( 'NONE', #30257, 32.50000000000000000 ) ;
#6164=CARTESIAN_POINT ( 'NONE',  ( -1.778240108872766143E-15, 2.000000005462374997, -32.49999999999999289 ) ) ;
#6167=CARTESIAN_POINT ( 'NONE',  ( -32.50000000000000000, 79.25000000273118417, 0.000000000000000000 ) ) ;
#6171=VECTOR ( 'NONE', #16704, 1000.000000000000114 ) ;
#6175=ORIENTED_EDGE ( 'NONE', *, *, #30303, .T. ) ;
#6179=CARTESIAN_POINT ( 'NONE',  ( -10.04305231718578462, 46.90000000546238113, 30.90933677959249337 ) ) ;
#6180=CARTESIAN_POINT ( 'NONE',  ( 27.16883889988623935, 46.57500000273117990, -19.73931689729374384 ) ) ;
#6181=CARTESIAN_POINT ( 'NONE',  ( -20.08610463437157989, 48.20000000546237828, -27.64615127144129758 ) ) ;
#6183=CARTESIAN_POINT ( 'NONE',  ( -33.58253175000000113, 35.12500000273119127, 0.000000000000000000 ) ) ;
#6185=CARTESIAN_POINT ( 'NONE',  ( 27.16883889988624290, 62.17500000273118133, 19.73931689729373673 ) ) ;
#6186=CARTESIAN_POINT ( 'NONE',  ( 0.000000000000000000, 0.000000000000000000, 0.000000000000000000 ) ) ;
#6187=CARTESIAN_POINT ( 'NONE',  ( -32.50000000000000000, 38.09999999999999432, 10.55989012756946366 ) ) ;
#6189=CARTESIAN_POINT ( 'NONE',  ( -27.16883889988624290, 3.175000002731187543, -19.73931689729374028 ) ) ;
#6191=CARTESIAN_POINT ( 'NONE',  ( 32.50000000000000000, 13.09999999999999432, -10.55989012756945833 ) ) ;
#6193=CARTESIAN_POINT ( 'NONE',  ( 33.58253175000000823, 76.27500000273118985, 10.91162601494192685 ) ) ;
#6194=CARTESIAN_POINT ( 'NONE',  ( -15.14183272437242067, 4.699999999999996625, -20.84094480462497856 ) ) ;
#6198=CARTESIAN_POINT ( 'NONE',  ( 15.14183272437241889, 3.449999994537620296, 20.84094480462498211 ) ) ;
#6212=CARTESIAN_POINT ( 'NONE',  ( -3.880418787951099180, 16.55125428154684286, -24.50000000000001421 ) ) ;
#6213=ORIENTED_EDGE ( 'NONE', *, *, #15322, .T. ) ;
#6218=VERTEX_POINT ( 'NONE', #20507 ) ;
#6221=EDGE_CURVE ( 'NONE', #15956, #21689, #28417, .T. ) ;
#6225=CARTESIAN_POINT ( 'NONE',  ( -32.50000000000000000, 48.60000000546235555, 10.55989012756946366 ) ) ;
#6226=CARTESIAN_POINT ( 'NONE',  ( -20.75514604977248112, 53.42500000273117422, 28.56700777964554661 ) ) ;
#6228=CARTESIAN_POINT ( 'NONE',  ( 6.277390505771533514E-15, 9.000000005462364783, 34.17252228774368916 ) ) ;
#6229=CARTESIAN_POINT ( 'NONE',  ( 3.880418787951134707, 15.30125427608446742, 24.50000000000000000 ) ) ;
#6230=CARTESIAN_POINT ( 'NONE',  ( -4.523095164977117273E-15, 14.62499999726882649, 24.62258325217400312 ) ) ;
#6231=CARTESIAN_POINT ( 'NONE',  ( -32.50000000000000000, 57.89999999999999858, -10.55989012756945478 ) ) ;
#6232=CARTESIAN_POINT ( 'NONE',  ( -2.162160676586881955E-15, 22.87500000273118062, -35.31076352940723240 ) ) ;
#6234=CARTESIAN_POINT ( 'NONE',  ( -13.91746824999999532, 76.77500000273117564, -4.522059556121115875 ) ) ;
#6235=CARTESIAN_POINT ( 'NONE',  ( 19.82091636218621389, 16.19999999999999218, -14.40073868116559197 ) ) ;
#6236=CARTESIAN_POINT ( 'NONE',  ( 5.779280353836490358E-15, 14.50000000000000178, 32.49999999999999289 ) ) ;
#6238=ORIENTED_EDGE ( 'NONE', *, *, #25807, .T. ) ;
#6240=CARTESIAN_POINT ( 'NONE',  ( 13.91746825000000065, 75.77500000273120406, 4.522059556121114987 ) ) ;
#6242=CARTESIAN_POINT ( 'NONE',  ( -20.75514604977248823, 18.82500000273119767, -28.56700777964554305 ) ) ;
#6247=CARTESIAN_POINT ( 'NONE',  ( 33.58253175000000113, 10.37500000273117173, -4.112674001490185761E-15 ) ) ;
#6251=CARTESIAN_POINT ( 'NONE',  ( 3.735172737399427541E-15, 80.00000000000001421, 30.50000000000000000 ) ) ;
#6252=CARTESIAN_POINT ( 'NONE',  ( -4.300734207923759378, 74.97500000273119269, -13.23629886949340495 ) ) ;
#6254=CARTESIAN_POINT ( 'NONE',  ( 8.891200544363830713E-16, 79.75000000546236834, -15.00000000000000000 ) ) ;
#6255=CARTESIAN_POINT ( 'NONE',  ( 20.75514604977249178, 53.82500000273119412, 28.56700777964553950 ) ) ;
#6257=ORIENTED_EDGE ( 'NONE', *, *, #9555, .F. ) ;
#6259=CARTESIAN_POINT ( 'NONE',  ( 0.000000000000000000, 0.000000000000000000, 0.000000000000000000 ) ) ;
#6260=CARTESIAN_POINT ( 'NONE',  ( 7.236395654485755280, 4.224999997268802154, 22.27133577429736988 ) ) ;
#6262=( BOUNDED_CURVE ( )  B_SPLINE_CURVE ( 2, ( #23922, #558, #32128, #24090, #7957, #19107, #18444, #8125, #13625, #8456, #5890, #16204, #31794 ),
 .UNSPECIFIED., .F., .T. ) 
 B_SPLINE_CURVE_WITH_KNOTS ( ( 3, 2, 2, 2, 2, 2, 3 ),
 ( 0.3525641025641025883, 0.3538461538461538658, 0.3564102564102564208, 0.3589743589743589758, 0.3615384615384615308, 0.3641025641025640858, 0.3653846153846153633 ),
 .UNSPECIFIED. ) 
 CURVE ( )  GEOMETRIC_REPRESENTATION_ITEM ( )  RATIONAL_B_SPLINE_CURVE ( ( 0.9755282581475768211, 0.9755282581475772652, 1.000000000000000000, 0.9510565162951535312, 1.000000000000000000, 0.9510565162951535312, 1.000000000000000000, 0.9510565162951535312, 1.000000000000000000, 0.9510565162951535312, 1.000000000000000000, 0.9755282581475768211, 0.9755282581475768211 ) ) 
 REPRESENTATION_ITEM ( '' )  );
#6263=ORIENTED_EDGE ( 'NONE', *, *, #33483, .F. ) ;
#6269=CARTESIAN_POINT ( 'NONE',  ( -33.58253175000000113, 59.37500000273118417, 0.000000000000000000 ) ) ;
#6270=CARTESIAN_POINT ( 'NONE',  ( 2.067204126564591252E-14, 4.499999999999996447, -24.50000000000000000 ) ) ;
#6271=CARTESIAN_POINT ( 'NONE',  ( -33.58253175000000113, 71.12500000273119838, 0.000000000000000000 ) ) ;
#6273=CARTESIAN_POINT ( 'NONE',  ( 19.82091636218621389, 4.200000000000009059, -14.40073868116559197 ) ) ;
#6274=CARTESIAN_POINT ( 'NONE',  ( -33.58253175000000113, 3.475000002731185589, 10.91162601494193929 ) ) ;
#6276=CARTESIAN_POINT ( 'NONE',  ( 6.486482029760649416E-15, 19.62500000273116996, 35.31076352940723240 ) ) ;
#6277=CARTESIAN_POINT ( 'NONE',  ( -13.91746824999999532, 74.77500000273117564, -4.522059556121115875 ) ) ;
#6279=CARTESIAN_POINT ( 'NONE',  ( 9.270509831248423538, 79.30000000000003979, -12.75976212528059861 ) ) ;
#6282=CARTESIAN_POINT ( 'NONE',  ( 5.147494310547426899, 71.44874571845316780, -32.50000000000000000 ) ) ;
#6284=CARTESIAN_POINT ( 'NONE',  ( -10.37757302488624411, 42.72500000273119269, -31.93888565452638417 ) ) ;
#6287=CARTESIAN_POINT ( 'NONE',  ( 33.58253175000000823, 30.27500000273118275, 10.91162601494192685 ) ) ;
#6290=CARTESIAN_POINT ( 'NONE',  ( 24.50000000000000000, 18.00000000000001421, 0.000000000000000000 ) ) ;
#6291=CARTESIAN_POINT ( 'NONE',  ( -9.270509831248423538, 75.69999999999998863, -12.75976212528059861 ) ) ;
#6294=CARTESIAN_POINT ( 'NONE',  ( 23.41746824999999887, 6.724999997268811924, -7.608796670333727974 ) ) ;
#6298=CARTESIAN_POINT ( 'NONE',  ( -12.13525491562420910, 76.45000000546237118, 8.816778784387098611 ) ) ;
#6299=CARTESIAN_POINT ( 'NONE',  ( 33.58253175000000113, 22.22500000273117493, -10.91162601494193574 ) ) ;
#6300=CARTESIAN_POINT ( 'NONE',  ( -4.523095164977116484E-15, 6.624999997268815832, 24.62258325217400312 ) ) ;
#6302=ORIENTED_EDGE ( 'NONE', *, *, #8037, .F. ) ;
#6308=CARTESIAN_POINT ( 'NONE',  ( 5.147494310547426899, 39.44874571845314648, -32.50000000000000000 ) ) ;
#6309=CARTESIAN_POINT ( 'NONE',  ( -19.82091636218621389, 14.94999999453763806, 14.40073868116558842 ) ) ;
#6310=CARTESIAN_POINT ( 'NONE',  ( -23.41746824999999887, 3.624999997268813168, -2.867812753649727150E-15 ) ) ;
#6311=CARTESIAN_POINT ( 'NONE',  ( 27.16883889988623935, 28.57500000273119412, -19.73931689729374384 ) ) ;
#6313=CARTESIAN_POINT ( 'NONE',  ( 26.29305231718579350, 33.30000000546237970, 19.10302069950537529 ) ) ;
#6314=EDGE_CURVE ( 'NONE', #13788, #969, #1633, .T. ) ;
#6315=CARTESIAN_POINT ( 'NONE',  ( -32.50000000000000000, 74.00000000000001421, 0.000000000000000000 ) ) ;
#6316=LINE ( 'NONE', #19698, #10504 ) ;
#6317=CARTESIAN_POINT ( 'NONE',  ( -1.778240108872766143E-15, 38.00000000546237544, -32.49999999999999289 ) ) ;
#6319=CARTESIAN_POINT ( 'NONE',  ( -33.58253175000000113, 39.27500000273118275, -10.91162601494193218 ) ) ;
#6322=EDGE_CURVE ( 'NONE', #28763, #17393, #3154, .T. ) ;
#6323=CARTESIAN_POINT ( 'NONE',  ( -14.47279130897152122, 10.42499999726881299, 19.92008829642072243 ) ) ;
#6324=CARTESIAN_POINT ( 'NONE',  ( -10.04305231718578462, 12.39999999999999503, 30.90933677959249337 ) ) ;
#6327=CARTESIAN_POINT ( 'NONE',  ( -10.37757302488623701, 63.52500000273120406, 31.93888565452638417 ) ) ;
#6328=CARTESIAN_POINT ( 'NONE',  ( -33.58253175000000113, 45.37500000273120548, 0.000000000000000000 ) ) ;
#6331=CARTESIAN_POINT ( 'NONE',  ( 6.486482029760649416E-15, 5.625000002731175286, 35.31076352940723240 ) ) ;
#6334=DIRECTION ( 'NONE',  ( -0.000000000000000000, -1.000000000000000000, -0.000000000000000000 ) ) ;
#6341=PRESENTATION_STYLE_ASSIGNMENT (( #8406 ) ) ;
#6347=ORIENTED_EDGE ( 'NONE', *, *, #29971, .T. ) ;
#6349=AXIS2_PLACEMENT_3D ( 'NONE', #10680, #31603, #30030 ) ;
#6352=CARTESIAN_POINT ( 'NONE',  ( -20.08610463437157989, 46.20000000546237828, -27.64615127144129758 ) ) ;
#6353=CARTESIAN_POINT ( 'NONE',  ( -33.58253175000000113, 47.37500000273120548, 0.000000000000000000 ) ) ;
#6354=CARTESIAN_POINT ( 'NONE',  ( 26.29305231718579350, 49.30000000546236549, 19.10302069950537529 ) ) ;
#6356=CARTESIAN_POINT ( 'NONE',  ( -20.75514604977248823, 28.82500000273116569, -28.56700777964554305 ) ) ;
#6357=CARTESIAN_POINT ( 'NONE',  ( 32.50000000000000000, 77.60000000546237686, -10.55989012756945833 ) ) ;
#6358=CARTESIAN_POINT ( 'NONE',  ( 6.486482029760649416E-15, 61.87500000273117706, 35.31076352940723240 ) ) ;
#6360=CARTESIAN_POINT ( 'NONE',  ( 32.50000000000000000, 35.10000000000000142, -10.55989012756945833 ) ) ;
#6362=( BOUNDED_CURVE ( )  B_SPLINE_CURVE ( 2, ( #27434, #3925, #14399, #25370, #25196, #12149, #30504, #14232, #9581, #3760, #1506, #1849, #22293 ),
 .UNSPECIFIED., .F., .T. ) 
 B_SPLINE_CURVE_WITH_KNOTS ( ( 3, 2, 2, 2, 2, 2, 3 ),
 ( 0.4807692307692307820, 0.4820512820512820595, 0.4846153846153846145, 0.4871794871794871695, 0.4897435897435897245, 0.4923076923076923350, 0.4935897435897436125 ),
 .UNSPECIFIED. ) 
 CURVE ( )  GEOMETRIC_REPRESENTATION_ITEM ( )  RATIONAL_B_SPLINE_CURVE ( ( 0.9755282581475768211, 0.9755282581475768211, 1.000000000000000000, 0.9510565162951535312, 1.000000000000000000, 0.9510565162951535312, 1.000000000000000000, 0.9510565162951535312, 1.000000000000000000, 0.9510565162951535312, 1.000000000000000000, 0.9755282581475768211, 0.9755282581475768211 ) ) 
 REPRESENTATION_ITEM ( '' )  );
#6363=CARTESIAN_POINT ( 'NONE',  ( -27.16883889988623935, 7.575000002731202997, 19.73931689729374739 ) ) ;
#6364=CYLINDRICAL_SURFACE ( 'NONE', #17306, 32.50000000000000000 ) ;
#6366=CARTESIAN_POINT ( 'NONE',  ( -33.58253175000000113, 65.27500000273117564, -10.91162601494193041 ) ) ;
#6367=CARTESIAN_POINT ( 'NONE',  ( 19.82091636218621034, 3.549999994537617276, 14.40073868116559730 ) ) ;
#6370=CARTESIAN_POINT ( 'NONE',  ( 24.50000000000000000, 1.749999994537621006, 0.000000000000000000 ) ) ;
#6372=CARTESIAN_POINT ( 'NONE',  ( 2.375766604868046361, 74.55125428154683220, 14.99999999999999822 ) ) ;
#6381=FACE_BOUND ( 'NONE', #19606, .T. ) ;
#6384=CARTESIAN_POINT ( 'NONE',  ( -19.82091636218621034, 16.80000000000000782, -14.40073868116559552 ) ) ;
#6387=DIRECTION ( 'NONE',  ( 0.000000000000000000, -1.000000000000000000, 0.000000000000000000 ) ) ;
#6389=ORIENTED_EDGE ( 'NONE', *, *, #19964, .T. ) ;
#6394=CARTESIAN_POINT ( 'NONE',  ( 20.75514604977248467, 56.42500000273120264, -28.56700777964554305 ) ) ;
#6396=CARTESIAN_POINT ( 'NONE',  ( -32.50000000000000000, 12.50000000546236478, 0.000000000000000000 ) ) ;
#6399=CARTESIAN_POINT ( 'NONE',  ( -23.41746825000000243, 12.22499999726881370, 7.608796670333725309 ) ) ;
#6401=CARTESIAN_POINT ( 'NONE',  ( 10.04305231718579705, 62.59999999999998721, 30.90933677959248982 ) ) ;
#6402=CARTESIAN_POINT ( 'NONE',  ( -20.75514604977248823, 21.07500000273118346, -28.56700777964554305 ) ) ;
#6403=CARTESIAN_POINT ( 'NONE',  ( 2.375766604868046361, 76.55125428154684641, 14.99999999999999822 ) ) ;
#6405=CARTESIAN_POINT ( 'NONE',  ( -8.601468415847518756, 72.57500000273117280, -11.83890561707634781 ) ) ;
#6406=CYLINDRICAL_SURFACE ( 'NONE', #18984, 32.50000000000000000 ) ;
#6408=EDGE_CURVE ( 'NONE', #10494, #28763, #6262, .T. ) ;
#6411=VERTEX_POINT ( 'NONE', #5387 ) ;
#6415=CARTESIAN_POINT ( 'NONE',  ( 27.16883889988623935, 16.32500000273118346, -19.73931689729374384 ) ) ;
#6419=CARTESIAN_POINT ( 'NONE',  ( 33.58253175000000823, 10.27500000273117386, 10.91162601494192685 ) ) ;
#6421=EDGE_CURVE ( 'NONE', #18399, #21929, #11969, .T. ) ;
#6424=CARTESIAN_POINT ( 'NONE',  ( -8.960552108402744065E-16, 74.87500000273116996, -14.63369212191046209 ) ) ;
#6426=CARTESIAN_POINT ( 'NONE',  ( -33.58253175000000113, 49.22500000273119269, 10.91162601494193929 ) ) ;
#6428=ADVANCED_FACE ( 'NONE', ( #21682 ), #24253, .F. ) ;
#6431=CARTESIAN_POINT ( 'NONE',  ( -26.29305231718578995, 2.199999999999979750, 19.10302069950538595 ) ) ;
#6432=CARTESIAN_POINT ( 'NONE',  ( -7.236395654485763274, 6.024999997268825958, 22.27133577429736633 ) ) ;
#6434=EDGE_LOOP ( 'NONE', ( #972, #26025, #15008, #11207 ) ) ;
#6440=CARTESIAN_POINT ( 'NONE',  ( 10.37757302488624767, 57.97500000273119980, 31.93888565452638417 ) ) ;
#6442=CARTESIAN_POINT ( 'NONE',  ( 27.16883889988623935, 72.32500000273117280, -19.73931689729374384 ) ) ;
#6444=CARTESIAN_POINT ( 'NONE',  ( -7.570916362186215665, 3.400000000000014122, 23.30088464923126423 ) ) ;
#6445=CARTESIAN_POINT ( 'NONE',  ( -27.16883889988623935, 1.575000002731197224, 19.73931689729374739 ) ) ;
#6446=CARTESIAN_POINT ( 'NONE',  ( -27.16883889988624290, 14.92500000273117067, -19.73931689729374028 ) ) ;
#6447=CARTESIAN_POINT ( 'NONE',  ( -4.300734207923755825, 75.27500000273118985, 13.23629886949340673 ) ) ;
#6449=CARTESIAN_POINT ( 'NONE',  ( 11.25946833292375793, 72.17500000273119554, 8.180482586598731842 ) ) ;
#6453=FACE_OUTER_BOUND ( 'NONE', #15705, .T. ) ;
#6455=CARTESIAN_POINT ( 'NONE',  ( -33.58253175000000113, 39.12500000273119838, 0.000000000000000000 ) ) ;
#6458=CARTESIAN_POINT ( 'NONE',  ( 6.486482029760648627E-15, 29.87500000273119483, 35.31076352940722529 ) ) ;
#6461=CARTESIAN_POINT ( 'NONE',  ( -15.14183272437242067, 14.44999999453762207, -20.84094480462497856 ) ) ;
#6465=CARTESIAN_POINT ( 'NONE',  ( -14.47279130897152299, 7.924999997268802332, 19.92008829642072243 ) ) ;
#6467=( BOUNDED_CURVE ( )  B_SPLINE_CURVE ( 2, ( #6025, #3956, #16503, #19414, #19747, #6191, #11676, #14097, #700, #26956, #3790, #13927, #19582 ),
 .UNSPECIFIED., .F., .T. ) 
 B_SPLINE_CURVE_WITH_KNOTS ( ( 3, 2, 2, 2, 2, 2, 3 ),
 ( 0.8525641025641025328, 0.8538461538461538103, 0.8564102564102563653, 0.8589743589743589203, 0.8615384615384615863, 0.8641025641025641413, 0.8653846153846154188 ),
 .UNSPECIFIED. ) 
 CURVE ( )  GEOMETRIC_REPRESENTATION_ITEM ( )  RATIONAL_B_SPLINE_CURVE ( ( 0.9755282581475768211, 0.9755282581475768211, 1.000000000000000000, 0.9510565162951535312, 1.000000000000000000, 0.9510565162951535312, 1.000000000000000000, 0.9510565162951535312, 1.000000000000000000, 0.9510565162951535312, 1.000000000000000000, 0.9755282581475768211, 0.9755282581475768211 ) ) 
 REPRESENTATION_ITEM ( '' )  );
#6471=( BOUNDED_CURVE ( )  B_SPLINE_CURVE ( 2, ( #31135, #10376, #10544, #23423, #28893, #2307, #7965, #10713, #12780, #23075, #28221, #7626, #5396 ),
 .UNSPECIFIED., .F., .T. ) 
 B_SPLINE_CURVE_WITH_KNOTS ( ( 3, 2, 2, 2, 2, 2, 3 ),
 ( 0.6217948717948718063, 0.6230769230769230838, 0.6256410256410256387, 0.6282051282051281937, 0.6307692307692307487, 0.6333333333333333037, 0.6346153846153845812 ),
 .UNSPECIFIED. ) 
 CURVE ( )  GEOMETRIC_REPRESENTATION_ITEM ( )  RATIONAL_B_SPLINE_CURVE ( ( 0.9755282581475768211, 0.9755282581475768211, 1.000000000000000000, 0.9510565162951535312, 1.000000000000000000, 0.9510565162951535312, 1.000000000000000000, 0.9510565162951535312, 1.000000000000000000, 0.9510565162951535312, 1.000000000000000000, 0.9755282581475768211, 0.9755282581475768211 ) ) 
 REPRESENTATION_ITEM ( '' )  );
#6472=CARTESIAN_POINT ( 'NONE',  ( 10.37757302488624056, 12.52500000273118452, -31.93888565452638417 ) ) ;
#6473=CARTESIAN_POINT ( 'NONE',  ( 14.47279130897151589, 6.824999997268808904, 19.92008829642072953 ) ) ;
#6475=ORIENTED_EDGE ( 'NONE', *, *, #17076, .T. ) ;
#6478=ORIENTED_EDGE ( 'NONE', *, *, #423, .F. ) ;
#6482=CARTESIAN_POINT ( 'NONE',  ( -7.570916362186210335, 16.34999999453762243, -23.30088464923126779 ) ) ;
#6483=CARTESIAN_POINT ( 'NONE',  ( 18.94512977948575738, 4.424999997268807661, 13.76444248337723408 ) ) ;
#6484=CARTESIAN_POINT ( 'NONE',  ( -10.37757302488624411, 22.97500000273117138, -31.93888565452638417 ) ) ;
#6485=CARTESIAN_POINT ( 'NONE',  ( -20.08610463437157989, 30.20000000546236407, -27.64615127144129758 ) ) ;
#6486=CARTESIAN_POINT ( 'NONE',  ( 10.04305231718578817, 73.40000000000001990, -30.90933677959249337 ) ) ;
#6487=CARTESIAN_POINT ( 'NONE',  ( 20.08610463437157279, 37.80000000546237970, -27.64615127144129758 ) ) ;
#6489=CARTESIAN_POINT ( 'NONE',  ( 20.75514604977249178, 34.07500000273117990, 28.56700777964553950 ) ) ;
#6492=CARTESIAN_POINT ( 'NONE',  ( -4.523095164977116484E-15, 10.62499999726880695, 24.62258325217400312 ) ) ;
#6493=CARTESIAN_POINT ( 'NONE',  ( 32.50000000000000711, 14.89999999999999680, 10.55989012756945122 ) ) ;
#6496=CARTESIAN_POINT ( 'NONE',  ( 20.75514604977249178, 53.82500000273119412, 28.56700777964553950 ) ) ;
#6497=CARTESIAN_POINT ( 'NONE',  ( 10.37757302488624056, 44.77500000273118275, -31.93888565452638417 ) ) ;
#6499=FACE_OUTER_BOUND ( 'NONE', #27494, .T. ) ;
#6500=CARTESIAN_POINT ( 'NONE',  ( -20.75514604977248823, 2.825000002731177240, -28.56700777964554305 ) ) ;
#6506=CARTESIAN_POINT ( 'NONE',  ( 1.836970198721029589E-15, 82.00000000000001421, 15.00000000000000000 ) ) ;
#6507=FACE_BOUND ( 'NONE', #30305, .T. ) ;
#6508=CARTESIAN_POINT ( 'NONE',  ( 1.555960095263670572E-15, 14.50000000000000178, -24.50000000000000000 ) ) ;
#6511=EDGE_CURVE ( 'NONE', #27108, #9001, #6046, .T. ) ;
#6513=CARTESIAN_POINT ( 'NONE',  ( 33.58253175000000113, 34.12500000273119127, -4.112674001490185761E-15 ) ) ;
#6523=CARTESIAN_POINT ( 'NONE',  ( 26.29305231718578995, 21.19999999999999574, -19.10302069950538240 ) ) ;
#6524=CARTESIAN_POINT ( 'NONE',  ( 33.58253175000000823, 40.27500000273118985, 10.91162601494192863 ) ) ;
#6525=CARTESIAN_POINT ( 'NONE',  ( -10.04305231718579172, 48.10000000546238397, -30.90933677959248982 ) ) ;
#6527=CARTESIAN_POINT ( 'NONE',  ( 10.37757302488624056, 28.52500000273120051, -31.93888565452638417 ) ) ;
#6528=LINE ( 'NONE', #11839, #28560 ) ;
#6529=CARTESIAN_POINT ( 'NONE',  ( 33.58253175000000113, 54.47500000273117138, -10.91162601494193751 ) ) ;
#6532=CARTESIAN_POINT ( 'NONE',  ( -10.04305231718578462, 36.39999999999999147, 30.90933677959249337 ) ) ;
#6534=CARTESIAN_POINT ( 'NONE',  ( -20.75514604977248823, 74.82500000273115859, -28.56700777964554305 ) ) ;
#6535=CARTESIAN_POINT ( 'NONE',  ( 0.000000000000000000, 80.00000000000001421, 0.000000000000000000 ) ) ;
#6537=CARTESIAN_POINT ( 'NONE',  ( 10.37757302488624767, 65.97500000273120691, 31.93888565452638417 ) ) ;
#6538=CARTESIAN_POINT ( 'NONE',  ( -15.14183272437242778, 5.300000000000006040, 20.84094480462497856 ) ) ;
#6540=CARTESIAN_POINT ( 'NONE',  ( 1.577395562988744260E-15, 2.249999994537629444, -25.76082449383753925 ) ) ;
#6553=ORIENTED_EDGE ( 'NONE', *, *, #427, .F. ) ;
#6555=CARTESIAN_POINT ( 'NONE',  ( -26.29305231718578995, 76.19999999999998863, 19.10302069950538595 ) ) ;
#6557=ORIENTED_EDGE ( 'NONE', *, *, #12835, .T. ) ;
#6560=( BOUNDED_CURVE ( )  B_SPLINE_CURVE ( 2, ( #28288, #23490, #5119, #28621, #33605, #12670, #28793, #20583, #10103, #15253, #31368, #2719, #25714 ),
 .UNSPECIFIED., .F., .T. ) 
 B_SPLINE_CURVE_WITH_KNOTS ( ( 3, 2, 2, 2, 2, 2, 3 ),
 ( 0.9294871794871795156, 0.9307692307692307931, 0.9333333333333333481, 0.9358974358974359031, 0.9384615384615384581, 0.9410256410256410131, 0.9423076923076922906 ),
 .UNSPECIFIED. ) 
 CURVE ( )  GEOMETRIC_REPRESENTATION_ITEM ( )  RATIONAL_B_SPLINE_CURVE ( ( 0.9755282581475768211, 0.9755282581475768211, 1.000000000000000000, 0.9510565162951535312, 1.000000000000000000, 0.9510565162951535312, 1.000000000000000000, 0.9510565162951535312, 1.000000000000000000, 0.9510565162951535312, 1.000000000000000000, 0.9755282581475768211, 0.9755282581475768211 ) ) 
 REPRESENTATION_ITEM ( '' )  );
#6561=CARTESIAN_POINT ( 'NONE',  ( -5.147494310547423346, 56.44874571845314648, 32.50000000000000000 ) ) ;
#6562=CARTESIAN_POINT ( 'NONE',  ( 20.75514604977248467, 50.42500000273118843, -28.56700777964554305 ) ) ;
#6565=CARTESIAN_POINT ( 'NONE',  ( -32.50000000000000000, 14.50000000546236478, 0.000000000000000000 ) ) ;
#6566=CARTESIAN_POINT ( 'NONE',  ( -4.635254915624208216, 78.39999999999999147, 14.26584774442730463 ) ) ;
#6567=CARTESIAN_POINT ( 'NONE',  ( 14.47279130897151944, 13.42499999726880411, -19.92008829642072598 ) ) ;
#6568=CARTESIAN_POINT ( 'NONE',  ( 26.29305231718579350, 52.80000000000001137, 19.10302069950537529 ) ) ;
#6569=CARTESIAN_POINT ( 'NONE',  ( 33.58253175000000823, 26.27500000273119340, 10.91162601494192863 ) ) ;
#6570=CARTESIAN_POINT ( 'NONE',  ( 3.980102097228898626E-15, 80.00000000000001421, 32.50000000000000000 ) ) ;
#6572=CARTESIAN_POINT ( 'NONE',  ( 4.300734207923761154, 73.47500000273119269, 13.23629886949340495 ) ) ;
#6573=CARTESIAN_POINT ( 'NONE',  ( 15.00000000000000000, 75.35000000546239107, -4.873795443493596835 ) ) ;
#6576=EDGE_LOOP ( 'NONE', ( #31124, #2559, #1773, #1439 ) ) ;
#6578=CARTESIAN_POINT ( 'NONE',  ( 2.688165632520823219E-15, 71.37500000273119838, 14.63369212191046387 ) ) ;
#6583=CARTESIAN_POINT ( 'NONE',  ( -10.37757302488623701, 11.77500000273118452, 31.93888565452638417 ) ) ;
#6586=CARTESIAN_POINT ( 'NONE',  ( 8.601468415847516980, 76.67500000273116711, -11.83890561707634603 ) ) ;
#6589=CARTESIAN_POINT ( 'NONE',  ( 6.486482029760648627E-15, 49.62500000273117706, 35.31076352940722529 ) ) ;
#6591=ORIENTED_EDGE ( 'NONE', *, *, #11041, .F. ) ;
#6594=CARTESIAN_POINT ( 'NONE',  ( -4.523095164977116484E-15, 12.12499999726881406, 24.62258325217400312 ) ) ;
#6602=CARTESIAN_POINT ( 'NONE',  ( -10.37757302488624411, 58.97500000273120691, -31.93888565452638417 ) ) ;
#6603=CARTESIAN_POINT ( 'NONE',  ( -32.50000000000000000, 36.40000000546236691, -10.55989012756945300 ) ) ;
#6604=CARTESIAN_POINT ( 'NONE',  ( -27.16883889988624290, 64.92500000273118133, -19.73931689729374028 ) ) ;
#6606=CARTESIAN_POINT ( 'NONE',  ( 19.82091636218621389, 8.200000000000013500, -14.40073868116559197 ) ) ;
#6608=CARTESIAN_POINT ( 'NONE',  ( 6.486482029760649416E-15, 15.62500000273117884, 35.31076352940723240 ) ) ;
#6609=CARTESIAN_POINT ( 'NONE',  ( 11.25946833292375793, 74.07500000273120122, -8.180482586598735395 ) ) ;
#6611=CARTESIAN_POINT ( 'NONE',  ( -15.00000000000000000, 81.90000000000000568, -4.873795443493594171 ) ) ;
#6613=CARTESIAN_POINT ( 'NONE',  ( -9.270509831248419985, 74.55000000546237970, 12.75976212528060039 ) ) ;
#6615=CARTESIAN_POINT ( 'NONE',  ( 12.13525491562420910, 77.45000000546237118, -8.816778784387098611 ) ) ;
#6617=CARTESIAN_POINT ( 'NONE',  ( -33.58253175000000113, 37.12500000273119838, 0.000000000000000000 ) ) ;
#6620=CARTESIAN_POINT ( 'NONE',  ( -33.58253175000000113, 27.27500000273118985, -10.91162601494193041 ) ) ;
#6621=CARTESIAN_POINT ( 'NONE',  ( -7.570916362186215665, 17.14999999453761959, 23.30088464923126423 ) ) ;
#6623=CARTESIAN_POINT ( 'NONE',  ( -32.50000000000000000, 18.09999999999998010, 10.55989012756946366 ) ) ;
#6624=CARTESIAN_POINT ( 'NONE',  ( 5.147494310547426899, 33.44874571845315359, -32.50000000000000000 ) ) ;
#6626=CARTESIAN_POINT ( 'NONE',  ( -7.236395654485763274, 14.02499999726880553, 22.27133577429736633 ) ) ;
#6630=ADVANCED_FACE ( 'NONE', ( #6888 ), #14452, .T. ) ;
#6631=CARTESIAN_POINT ( 'NONE',  ( -10.37757302488623701, 13.52500000273118630, 31.93888565452638417 ) ) ;
#6632=CARTESIAN_POINT ( 'NONE',  ( -7.236395654485757944, 9.724999997268806595, -22.27133577429736988 ) ) ;
#6634=ORIENTED_EDGE ( 'NONE', *, *, #19623, .F. ) ;
#6637=VERTEX_POINT ( 'NONE', #17201 ) ;
#6641=CARTESIAN_POINT ( 'NONE',  ( -20.08610463437156923, 72.80000000546236549, 27.64615127144130113 ) ) ;
#6642=CARTESIAN_POINT ( 'NONE',  ( 19.82091636218621034, 13.54999999453762527, 14.40073868116559730 ) ) ;
#6643=CARTESIAN_POINT ( 'NONE',  ( -14.47279130897151589, 5.324999997268799135, -19.92008829642072598 ) ) ;
#6644=CARTESIAN_POINT ( 'NONE',  ( -20.75514604977248823, 25.07500000273120122, -28.56700777964554305 ) ) ;
#6645=CARTESIAN_POINT ( 'NONE',  ( -20.08610463437156923, 24.80000000546235839, 27.64615127144130113 ) ) ;
#6646=CARTESIAN_POINT ( 'NONE',  ( -26.29305231718578995, 72.19999999999998863, 19.10302069950538595 ) ) ;
#6650=CARTESIAN_POINT ( 'NONE',  ( 20.75514604977248467, 36.67500000273118843, -28.56700777964554305 ) ) ;
#6654=CARTESIAN_POINT ( 'NONE',  ( 23.41746824999999887, 9.124999997268817609, 0.000000000000000000 ) ) ;
#6655=CARTESIAN_POINT ( 'NONE',  ( 20.08610463437157279, 17.30000000000000782, -27.64615127144129758 ) ) ;
#6658=CARTESIAN_POINT ( 'NONE',  ( 20.75514604977249178, 57.82500000273118701, 28.56700777964553950 ) ) ;
#6659=CARTESIAN_POINT ( 'NONE',  ( 10.37757302488624767, 47.97500000273119269, 31.93888565452638417 ) ) ;
#6660=( BOUNDED_CURVE ( )  B_SPLINE_CURVE ( 2, ( #28826, #15972, #2921, #10645, #23178, #4809, #329, #2412, #10815, #20953, #12878, #31402, #7385 ),
 .UNSPECIFIED., .F., .F. ) 
 B_SPLINE_CURVE_WITH_KNOTS ( ( 3, 2, 2, 2, 2, 2, 3 ),
 ( 0.9038461538461538547, 0.9051282051282051322, 0.9076923076923076872, 0.9102564102564102422, 0.9128205128205127972, 0.9153846153846153522, 0.9166666666666666297 ),
 .UNSPECIFIED. ) 
 CURVE ( )  GEOMETRIC_REPRESENTATION_ITEM ( )  RATIONAL_B_SPLINE_CURVE ( ( 0.9755282581475768211, 0.9755282581475768211, 1.000000000000000000, 0.9510565162951535312, 1.000000000000000000, 0.9510565162951535312, 1.000000000000000000, 0.9510565162951535312, 1.000000000000000000, 0.9510565162951535312, 1.000000000000000000, 0.9755282581475768211, 0.9755282581475768211 ) ) 
 REPRESENTATION_ITEM ( '' )  );
#6663=CARTESIAN_POINT ( 'NONE',  ( 33.58253175000000113, 2.125000002731192161, -4.112674001490185761E-15 ) ) ;
#6670=CARTESIAN_POINT ( 'NONE',  ( 32.50000000000000000, 41.60000000546236976, -10.55989012756945833 ) ) ;
#6673=CARTESIAN_POINT ( 'NONE',  ( -8.891200544363830713E-16, 71.75000000546238255, -15.00000000000000000 ) ) ;
#6674=CARTESIAN_POINT ( 'NONE',  ( 33.58253175000000113, 32.22500000273117848, -10.91162601494193574 ) ) ;
#6676=ORIENTED_EDGE ( 'NONE', *, *, #26197, .T. ) ;
#6680=EDGE_LOOP ( 'NONE', ( #29263, #8499, #24698, #8128 ) ) ;
#6684=CARTESIAN_POINT ( 'NONE',  ( 5.779280353836490358E-15, 65.00000000546236834, 32.49999999999999289 ) ) ;
#6685=CARTESIAN_POINT ( 'NONE',  ( -10.37757302488623701, 39.77500000273118275, 31.93888565452638417 ) ) ;
#6686=CARTESIAN_POINT ( 'NONE',  ( 32.50000000000000000, 41.60000000546238397, -10.55989012756945833 ) ) ;
#6688=CARTESIAN_POINT ( 'NONE',  ( -2.162160676586881955E-15, 28.62500000273118062, -35.31076352940723240 ) ) ;
#6689=CARTESIAN_POINT ( 'NONE',  ( -20.08610463437157989, 23.70000000000000639, -27.64615127144129758 ) ) ;
#6690=CARTESIAN_POINT ( 'NONE',  ( -20.75514604977248823, 53.07500000273118701, -28.56700777964554305 ) ) ;
#6692=CARTESIAN_POINT ( 'NONE',  ( -26.29305231718578995, 36.20000000000000995, 19.10302069950538595 ) ) ;
#6694=EDGE_CURVE ( 'NONE', #33755, #31336, #17368, .T. ) ;
#6695=CARTESIAN_POINT ( 'NONE',  ( 33.58253175000000113, 78.22500000273119269, -10.91162601494193751 ) ) ;
#6698=CARTESIAN_POINT ( 'NONE',  ( -33.58253175000000113, 67.47500000273116427, 10.91162601494193929 ) ) ;
#6700=EDGE_CURVE ( 'NONE', #8211, #6218, #15908, .T. ) ;
#6702=CARTESIAN_POINT ( 'NONE',  ( 1.577395562988744260E-15, 6.249999994537619230, -25.76082449383753925 ) ) ;
#6704=CARTESIAN_POINT ( 'NONE',  ( 15.14183272437242422, 8.049999994537621717, -20.84094480462497856 ) ) ;
#6705=AXIS2_PLACEMENT_3D ( 'NONE', #9035, #32037, #18851 ) ;
#6711=AXIS2_PLACEMENT_3D ( 'NONE', #16675, #18922, #13605 ) ;
#6716=CYLINDRICAL_SURFACE ( 'NONE', #12746, 24.50000000000000000 ) ;
#6723=VERTEX_POINT ( 'NONE', #4314 ) ;
#6725=CARTESIAN_POINT ( 'NONE',  ( 20.75514604977248467, 48.42500000273119554, -28.56700777964554305 ) ) ;
#6727=CARTESIAN_POINT ( 'NONE',  ( 32.50000000000000000, 13.60000000546239285, -10.55989012756945833 ) ) ;
#6729=CARTESIAN_POINT ( 'NONE',  ( -26.29305231718578995, 8.199999999999985079, 19.10302069950538595 ) ) ;
#6730=CARTESIAN_POINT ( 'NONE',  ( -14.47279130897152299, 14.42499999726880056, 19.92008829642072243 ) ) ;
#6731=CARTESIAN_POINT ( 'NONE',  ( -26.29305231718578995, 54.19999999999999574, 19.10302069950538595 ) ) ;
#6733=DIRECTION ( 'NONE',  ( -0.000000000000000000, -1.000000000000000000, -0.000000000000000000 ) ) ;
#6734=CARTESIAN_POINT ( 'NONE',  ( 33.58253175000000823, 14.27500000273119340, 10.91162601494192863 ) ) ;
#6735=CARTESIAN_POINT ( 'NONE',  ( 15.00000000000000000, 77.00000000000001421, -1.836970198721029589E-15 ) ) ;
#6737=CARTESIAN_POINT ( 'NONE',  ( 8.601468415847516980, 76.17500000273116711, -11.83890561707634781 ) ) ;
#6740=ADVANCED_FACE ( 'NONE', ( #26448 ), #349, .T. ) ;
#6742=EDGE_LOOP ( 'NONE', ( #14126, #10623, #87 ) ) ;
#6744=CARTESIAN_POINT ( 'NONE',  ( 8.601468415847520532, 71.57500000273118701, 11.83890561707634781 ) ) ;
#6749=CARTESIAN_POINT ( 'NONE',  ( 6.486482029760648627E-15, 7.875000002731192161, 35.31076352940722529 ) ) ;
#6752=CARTESIAN_POINT ( 'NONE',  ( -13.91746824999999532, 73.27500000273120406, -4.522059556121115875 ) ) ;
#6755=CARTESIAN_POINT ( 'NONE',  ( -33.58253175000000113, 49.02500000273116854, -10.91162601494193041 ) ) ;
#6758=ORIENTED_EDGE ( 'NONE', *, *, #16049, .T. ) ;
#6761=DIRECTION ( 'NONE',  ( 0.000000000000000000, 0.000000000000000000, -1.000000000000000000 ) ) ;
#6762=CARTESIAN_POINT ( 'NONE',  ( 14.47279130897151589, 14.32499999726880624, 19.92008829642072953 ) ) ;
#6764=EDGE_LOOP ( 'NONE', ( #23457, #19923, #19586, #20768 ) ) ;
#6766=ORIENTED_EDGE ( 'NONE', *, *, #8408, .T. ) ;
#6768=CARTESIAN_POINT ( 'NONE',  ( -27.16883889988624290, 59.17500000273118133, -19.73931689729374028 ) ) ;
#6770=CARTESIAN_POINT ( 'NONE',  ( 20.75514604977248467, 66.42500000273120975, -28.56700777964554305 ) ) ;
#6772=CARTESIAN_POINT ( 'NONE',  ( -15.14183272437242600, 15.30000000000001137, 20.84094480462497856 ) ) ;
#6773=CARTESIAN_POINT ( 'NONE',  ( -33.58253175000000113, 1.375000002731191495, 0.000000000000000000 ) ) ;
#6774=CARTESIAN_POINT ( 'NONE',  ( 33.58253175000000113, 12.12500000273120193, -4.112674001490185761E-15 ) ) ;
#6775=CARTESIAN_POINT ( 'NONE',  ( -10.04305231718578462, 0.9000000054623646939, 30.90933677959249337 ) ) ;
#6777=CARTESIAN_POINT ( 'NONE',  ( 12.13525491562421088, 74.80000000000001137, 8.816778784387095058 ) ) ;
#6781=CARTESIAN_POINT ( 'NONE',  ( 20.08610463437157279, 23.29999999999999005, -27.64615127144129758 ) ) ;
#6783=CARTESIAN_POINT ( 'NONE',  ( -15.00000000000000000, 80.25000000546239676, 0.000000000000000000 ) ) ;
#6785=CARTESIAN_POINT ( 'NONE',  ( 10.37757302488624767, 39.72500000273118559, 31.93888565452638417 ) ) ;
#6788=CARTESIAN_POINT ( 'NONE',  ( 27.16883889988623935, 26.57500000273119056, -19.73931689729374384 ) ) ;
#6789=CARTESIAN_POINT ( 'NONE',  ( 32.50000000000000000, 41.10000000000000853, -10.55989012756945833 ) ) ;
#6793=CARTESIAN_POINT ( 'NONE',  ( 7.236395654485760609, 11.02499999726880375, -22.27133577429736633 ) ) ;
#6798=CARTESIAN_POINT ( 'NONE',  ( 27.16883889988623935, 14.32500000273117990, -19.73931689729374384 ) ) ;
#6799=CARTESIAN_POINT ( 'NONE',  ( -18.94512977948575738, 9.924999997268812990, -13.76444248337723231 ) ) ;
#6801=VERTEX_POINT ( 'NONE', #29668 ) ;
#6808=CARTESIAN_POINT ( 'NONE',  ( 19.82091636218621389, 13.94999999453763806, -14.40073868116559197 ) ) ;
#6809=CARTESIAN_POINT ( 'NONE',  ( 23.41746825000000243, 10.52499999726880731, 7.608796670333735079 ) ) ;
#6810=CARTESIAN_POINT ( 'NONE',  ( 10.37757302488624056, 22.77500000273119340, -31.93888565452638417 ) ) ;
#6811=CARTESIAN_POINT ( 'NONE',  ( 20.08610463437158344, 23.20000000546238539, 27.64615127144129403 ) ) ;
#6812=CARTESIAN_POINT ( 'NONE',  ( 20.08610463437157279, 73.29999999999996874, -27.64615127144129758 ) ) ;
#6813=CARTESIAN_POINT ( 'NONE',  ( -26.29305231718579350, 6.300000005462380592, -19.10302069950537884 ) ) ;
#6816=CARTESIAN_POINT ( 'NONE',  ( 33.58253175000000113, 36.37500000273119838, -4.112674001490185761E-15 ) ) ;
#6819=CARTESIAN_POINT ( 'NONE',  ( -7.236395654485757944, 7.724999997268805707, -22.27133577429736988 ) ) ;
#6820=CARTESIAN_POINT ( 'NONE',  ( 32.50000000000000711, 12.90000000000000036, 10.55989012756945122 ) ) ;
#6821=CARTESIAN_POINT ( 'NONE',  ( 32.50000000000000000, 9.600000005462375086, -10.55989012756945833 ) ) ;
#6823=CARTESIAN_POINT ( 'NONE',  ( -27.16883889988623935, 57.32500000273119412, 19.73931689729374739 ) ) ;
#6824=CARTESIAN_POINT ( 'NONE',  ( 33.58253175000000113, 50.37500000273120548, -4.112674001490185761E-15 ) ) ;
#6826=EDGE_CURVE ( 'NONE', #1603, #30131, #11995, .T. ) ;
#6827=LINE ( 'NONE', #22289, #24879 ) ;
#6828=CARTESIAN_POINT ( 'NONE',  ( -27.16883889988623935, 1.325000002731169246, 19.73931689729374739 ) ) ;
#6831=CARTESIAN_POINT ( 'NONE',  ( 15.14183272437242067, 3.699999999999999289, 20.84094480462498211 ) ) ;
#6833=DIRECTION ( 'NONE',  ( 0.000000000000000000, -0.000000000000000000, -1.000000000000000000 ) ) ;
#6836=CARTESIAN_POINT ( 'NONE',  ( 3.980102097228898626E-15, 80.00000000000001421, 32.50000000000000000 ) ) ;
#6841=CARTESIAN_POINT ( 'NONE',  ( 20.75514604977249178, 31.82500000273119056, 28.56700777964553950 ) ) ;
#6842=CARTESIAN_POINT ( 'NONE',  ( 6.486482029760649416E-15, 65.87500000273119838, 35.31076352940723240 ) ) ;
#6850=ORIENTED_EDGE ( 'NONE', *, *, #8451, .F. ) ;
#6855=CARTESIAN_POINT ( 'NONE',  ( -26.29305231718579350, 64.30000000546237970, -19.10302069950537884 ) ) ;
#6856=CARTESIAN_POINT ( 'NONE',  ( 33.58253175000000113, 42.47500000273119980, -10.91162601494193751 ) ) ;
#6857=CARTESIAN_POINT ( 'NONE',  ( -32.50000000000000000, 46.50000000546239676, 0.000000000000000000 ) ) ;
#6859=CARTESIAN_POINT ( 'NONE',  ( 6.486482029760649416E-15, 27.62500000273118062, 35.31076352940723240 ) ) ;
#6860=CARTESIAN_POINT ( 'NONE',  ( -26.29305231718578995, 24.19999999999999929, 19.10302069950538595 ) ) ;
#6861=CARTESIAN_POINT ( 'NONE',  ( 10.37757302488624056, 54.77500000273119696, -31.93888565452638417 ) ) ;
#6863=CARTESIAN_POINT ( 'NONE',  ( -10.04305231718579172, 33.59999999999999432, -30.90933677959248982 ) ) ;
#6865=CARTESIAN_POINT ( 'NONE',  ( -27.16883889988624290, 74.92500000273119554, -19.73931689729374028 ) ) ;
#6868=CARTESIAN_POINT ( 'NONE',  ( -33.58253175000000113, 69.27500000273116143, -10.91162601494193041 ) ) ;
#6870=CARTESIAN_POINT ( 'NONE',  ( -19.82091636218621034, 8.549999994537621717, -14.40073868116559552 ) ) ;
#6871=COLOUR_RGB ( '', 0.09019608, 0.27058824, 0.51372549) ;
#6873=CARTESIAN_POINT ( 'NONE',  ( 7.570916362186207671, 7.349999994537615322, 23.30088464923126779 ) ) ;
#6881=VECTOR ( 'NONE', #1924, 1000.000000000000000 ) ;
#6883=CARTESIAN_POINT ( 'NONE',  ( 5.779280353836490358E-15, 42.49999999999999289, 32.49999999999999289 ) ) ;
#6884=CARTESIAN_POINT ( 'NONE',  ( 10.04305231718579705, 73.10000000546237686, 30.90933677959248982 ) ) ;
#6886=ADVANCED_FACE ( 'NONE', ( #27448 ), #14078, .F. ) ;
#6888=FACE_OUTER_BOUND ( 'NONE', #18526, .T. ) ;
#6889=ORIENTED_EDGE ( 'NONE', *, *, #24376, .F. ) ;
#6893=CARTESIAN_POINT ( 'NONE',  ( 26.29305231718578995, 61.70000000546238539, -19.10302069950538240 ) ) ;
#6894=ORIENTED_EDGE ( 'NONE', *, *, #5383, .T. ) ;
#6896=CARTESIAN_POINT ( 'NONE',  ( -10.37757302488623701, 49.52500000273118985, 31.93888565452638417 ) ) ;
#6897=CARTESIAN_POINT ( 'NONE',  ( 1.507698388325705758E-15, 17.12499999726880517, -24.62258325217400312 ) ) ;
#6898=DIRECTION ( 'NONE',  ( -1.000000000000000000, 0.000000000000000000, 0.000000000000000000 ) ) ;
#6899=CARTESIAN_POINT ( 'NONE',  ( -10.04305231718578462, 4.900000005462368691, 30.90933677959249337 ) ) ;
#6901=CARTESIAN_POINT ( 'NONE',  ( -7.236395654485763274, 12.52499999726880375, 22.27133577429736633 ) ) ;
#6902=CARTESIAN_POINT ( 'NONE',  ( 6.277390505771533514E-15, 52.50000000000000000, 34.17252228774368916 ) ) ;
#6904=CARTESIAN_POINT ( 'NONE',  ( 20.75514604977248467, 16.67500000273117777, -28.56700777964554305 ) ) ;
#6908=CARTESIAN_POINT ( 'NONE',  ( 11.25946833292375793, 74.07500000273120122, -8.180482586598735395 ) ) ;
#6910=CARTESIAN_POINT ( 'NONE',  ( -10.04305231718579172, 43.60000000000000142, -30.90933677959248982 ) ) ;
#6918=CARTESIAN_POINT ( 'NONE',  ( -5.147494310547423346, 20.44874571845315003, 32.50000000000000000 ) ) ;
#6922=CARTESIAN_POINT ( 'NONE',  ( 32.50000000000000000, 69.09999999999998010, -10.55989012756945833 ) ) ;
#6924=CARTESIAN_POINT ( 'NONE',  ( 33.58253175000000113, 50.22500000273118559, -10.91162601494193574 ) ) ;
#6927=ORIENTED_EDGE ( 'NONE', *, *, #26774, .F. ) ;
#6928=ADVANCED_FACE ( 'NONE', ( #1521, #29847 ), #21805, .T. ) ;
#6930=CARTESIAN_POINT ( 'NONE',  ( 10.04305231718579705, 16.60000000000000497, 30.90933677959248982 ) ) ;
#6931=CARTESIAN_POINT ( 'NONE',  ( 18.94512977948575738, 10.42499999726881299, 13.76444248337723408 ) ) ;
#6934=ORIENTED_EDGE ( 'NONE', *, *, #23790, .F. ) ;
#6939=FACE_OUTER_BOUND ( 'NONE', #26804, .T. ) ;
#6940=CARTESIAN_POINT ( 'NONE',  ( -2.162160676586881955E-15, 68.62500000273119838, -35.31076352940723240 ) ) ;
#6942=CARTESIAN_POINT ( 'NONE',  ( -15.14183272437241889, 14.70000000000000107, -20.84094480462497856 ) ) ;
#6943=CARTESIAN_POINT ( 'NONE',  ( -2.162160676586881955E-15, 4.875000002731200155, -35.31076352940723240 ) ) ;
#6944=CARTESIAN_POINT ( 'NONE',  ( -33.58253175000000113, 11.22500000273120335, 10.91162601494193929 ) ) ;
#6945=CARTESIAN_POINT ( 'NONE',  ( 11.25946833292375793, 71.67500000273119554, 8.180482586598731842 ) ) ;
#6947=CARTESIAN_POINT ( 'NONE',  ( 15.00000000000000000, 77.00000000000001421, -1.836970198721029589E-15 ) ) ;
#6949=CARTESIAN_POINT ( 'NONE',  ( 5.779280353836490358E-15, 61.00000000546238255, 32.49999999999999289 ) ) ;
#6951=CARTESIAN_POINT ( 'NONE',  ( 4.635254915624209993, 77.65000000546237402, -14.26584774442730463 ) ) ;
#6953=CARTESIAN_POINT ( 'NONE',  ( 20.75514604977249178, 35.82500000273117990, 28.56700777964553950 ) ) ;
#6956=CARTESIAN_POINT ( 'NONE',  ( 10.37757302488624767, 21.97500000273119980, 31.93888565452638417 ) ) ;
#6957=CARTESIAN_POINT ( 'NONE',  ( 5.147494310547426899, 41.44874571845314648, -32.50000000000000000 ) ) ;
#6959=CARTESIAN_POINT ( 'NONE',  ( 26.29305231718578995, 79.19999999999998863, -19.10302069950538240 ) ) ;
#6960=( BOUNDED_CURVE ( )  B_SPLINE_CURVE ( 2, ( #24829, #32711, #9207, #6641, #33048, #31001, #4578, #9900, #15056, #22772, #33225, #17462, #25688 ),
 .UNSPECIFIED., .F., .T. ) 
 B_SPLINE_CURVE_WITH_KNOTS ( ( 3, 2, 2, 2, 2, 2, 3 ),
 ( 0.07051282051282051211, 0.07179487179487178961, 0.07435897435897435848, 0.07692307692307692735, 0.07948717948717948234, 0.08205128205128205121, 0.08333333333333334259 ),
 .UNSPECIFIED. ) 
 CURVE ( )  GEOMETRIC_REPRESENTATION_ITEM ( )  RATIONAL_B_SPLINE_CURVE ( ( 0.9755282581475768211, 0.9755282581475768211, 1.000000000000000000, 0.9510565162951535312, 1.000000000000000000, 0.9510565162951535312, 1.000000000000000000, 0.9510565162951535312, 1.000000000000000000, 0.9510565162951535312, 1.000000000000000000, 0.9755282581475765991, 0.9755282581475767101 ) ) 
 REPRESENTATION_ITEM ( '' )  );
#6962=CARTESIAN_POINT ( 'NONE',  ( 7.236395654485755280, 8.224999997268806595, 22.27133577429736988 ) ) ;
#6964=VECTOR ( 'NONE', #27967, 1000.000000000000000 ) ;
#6968=CARTESIAN_POINT ( 'NONE',  ( -10.37757302488623701, 11.52500000273118452, 31.93888565452638417 ) ) ;
#6969=CARTESIAN_POINT ( 'NONE',  ( 23.41746824999999887, 9.124999997268817609, 0.000000000000000000 ) ) ;
#6971=ORIENTED_EDGE ( 'NONE', *, *, #6421, .F. ) ;
#6979=CARTESIAN_POINT ( 'NONE',  ( 0.000000000000000000, 82.00000000000001421, 0.000000000000000000 ) ) ;
#6980=CARTESIAN_POINT ( 'NONE',  ( 7.236395654485755280, 4.724999997268803043, 22.27133577429736988 ) ) ;
#6981=CARTESIAN_POINT ( 'NONE',  ( -7.236395654485757944, 9.224999997268806595, -22.27133577429736988 ) ) ;
#6982=CARTESIAN_POINT ( 'NONE',  ( 27.16883889988624290, 24.17500000273117777, 19.73931689729373673 ) ) ;
#6983=CARTESIAN_POINT ( 'NONE',  ( -26.29305231718579350, 26.30000000546236905, -19.10302069950537884 ) ) ;
#6984=CARTESIAN_POINT ( 'NONE',  ( -32.50000000000000000, 66.10000000000000853, 10.55989012756946366 ) ) ;
#6985=CARTESIAN_POINT ( 'NONE',  ( 32.50000000000000000, 47.60000000546239818, -10.55989012756945833 ) ) ;
#6986=CARTESIAN_POINT ( 'NONE',  ( -1.778240108872766143E-15, 4.000000005462373664, -32.49999999999999289 ) ) ;
#6988=CARTESIAN_POINT ( 'NONE',  ( -27.16883889988624290, 37.17500000273118843, -19.73931689729374028 ) ) ;
#6989=CARTESIAN_POINT ( 'NONE',  ( 13.91746824999999532, 80.47500000273119269, -4.522059556121118540 ) ) ;
#6992=CARTESIAN_POINT ( 'NONE',  ( -23.41746825000000243, 16.02499999726881086, -7.608796670333730638 ) ) ;
#6993=CARTESIAN_POINT ( 'NONE',  ( 26.29305231718578995, 15.19999999999999218, -19.10302069950538240 ) ) ;
#6996=CARTESIAN_POINT ( 'NONE',  ( -33.58253175000000113, 55.02500000273118985, -10.91162601494193218 ) ) ;
#6998=CARTESIAN_POINT ( 'NONE',  ( 6.486482029760648627E-15, 49.87500000273119838, 35.31076352940722529 ) ) ;
#7000=CARTESIAN_POINT ( 'NONE',  ( 3.245314017740486554E-15, 70.00000000000000000, -26.50000000000000355 ) ) ;
#7001=CARTESIAN_POINT ( 'NONE',  ( -10.04305231718579172, 49.60000000000000853, -30.90933677959248982 ) ) ;
#7004=CARTESIAN_POINT ( 'NONE',  ( 3.880418787951134707, 3.551254281546844194, 24.50000000000000000 ) ) ;
#7006=CARTESIAN_POINT ( 'NONE',  ( 26.29305231718579350, 66.79999999999999716, 19.10302069950537529 ) ) ;
#7007=LINE ( 'NONE', #6836, #33561 ) ;
#7010=CARTESIAN_POINT ( 'NONE',  ( 2.375766604868043252, 71.69874572391555034, -14.99999999999999822 ) ) ;
#7011=CARTESIAN_POINT ( 'NONE',  ( -27.16883889988624290, 30.92500000273118488, -19.73931689729374028 ) ) ;
#7013=VERTEX_POINT ( 'NONE', #8914 ) ;
#7017=CARTESIAN_POINT ( 'NONE',  ( 5.779280353836490358E-15, 3.000000005462374109, 32.49999999999999289 ) ) ;
#7018=ORIENTED_EDGE ( 'NONE', *, *, #2332, .T. ) ;
#7024=CARTESIAN_POINT ( 'NONE',  ( 10.37757302488624767, 39.97500000273118559, 31.93888565452638417 ) ) ;
#7025=CARTESIAN_POINT ( 'NONE',  ( -26.29305231718578995, 42.70000000546237118, 19.10302069950538595 ) ) ;
#7027=CARTESIAN_POINT ( 'NONE',  ( 33.58253175000000113, 30.12500000273118772, -4.112674001490185761E-15 ) ) ;
#7029=CARTESIAN_POINT ( 'NONE',  ( -33.58253175000000113, 55.47500000273119980, 10.91162601494193929 ) ) ;
#7031=CARTESIAN_POINT ( 'NONE',  ( -26.29305231718578995, 34.20000000000000995, 19.10302069950538595 ) ) ;
#7033=CARTESIAN_POINT ( 'NONE',  ( -33.58253175000000113, 77.22500000273117848, 10.91162601494193929 ) ) ;
#7035=CARTESIAN_POINT ( 'NONE',  ( -10.04305231718579172, 20.10000000546238752, -30.90933677959248982 ) ) ;
#7036=CARTESIAN_POINT ( 'NONE',  ( 27.16883889988624290, 66.17500000273118133, 19.73931689729373673 ) ) ;
#7038=EDGE_CURVE ( 'NONE', #15614, #24433, #11329, .T. ) ;
#7040=CARTESIAN_POINT ( 'NONE',  ( -33.58253175000000113, 17.02500000273118985, -10.91162601494193218 ) ) ;
#7041=CARTESIAN_POINT ( 'NONE',  ( -7.570916362186215665, 9.149999994537639125, 23.30088464923126423 ) ) ;
#7043=CARTESIAN_POINT ( 'NONE',  ( 20.08610463437157279, 47.29999999999999005, -27.64615127144129758 ) ) ;
#7053=DIRECTION ( 'NONE',  ( 0.000000000000000000, 0.000000000000000000, 1.000000000000000000 ) ) ;
#7054=CARTESIAN_POINT ( 'NONE',  ( -26.29305231718579350, 74.30000000546237970, -19.10302069950537884 ) ) ;
#7059=ORIENTED_EDGE ( 'NONE', *, *, #8037, .T. ) ;
#7060=CARTESIAN_POINT ( 'NONE',  ( 10.37757302488624056, 76.77500000273118985, -31.93888565452638417 ) ) ;
#7062=ORIENTED_EDGE ( 'NONE', *, *, #1694, .F. ) ;
#7064=CARTESIAN_POINT ( 'NONE',  ( -20.08610463437157989, 64.20000000546238539, -27.64615127144129758 ) ) ;
#7065=VERTEX_POINT ( 'NONE', #11829 ) ;
#7066=CARTESIAN_POINT ( 'NONE',  ( 2.489536152421872915E-14, 74.00000000546238255, -32.49999999999999289 ) ) ;
#7067=CARTESIAN_POINT ( 'NONE',  ( -10.37757302488624411, 50.72500000273119980, -31.93888565452638417 ) ) ;
#7068=DIRECTION ( 'NONE',  ( -0.000000000000000000, -1.000000000000000000, -0.000000000000000000 ) ) ;
#7069=CARTESIAN_POINT ( 'NONE',  ( 10.04305231718578817, 7.900000005462370467, -30.90933677959249337 ) ) ;
#7070=CARTESIAN_POINT ( 'NONE',  ( -15.00000000000000000, 78.00000000000001421, 0.000000000000000000 ) ) ;
#7071=CYLINDRICAL_SURFACE ( 'NONE', #10057, 32.50000000000000000 ) ;
#7072=CARTESIAN_POINT ( 'NONE',  ( 6.277390505771533514E-15, 54.49999999999999289, 34.17252228774368916 ) ) ;
#7073=CARTESIAN_POINT ( 'NONE',  ( -20.08610463437157989, 13.70000000000000462, -27.64615127144129758 ) ) ;
#7074=CARTESIAN_POINT ( 'NONE',  ( 33.58253175000000823, 16.27500000273118630, 10.91162601494192863 ) ) ;
#7075=CARTESIAN_POINT ( 'NONE',  ( -1.778240108872766143E-15, 62.00000000546238255, -32.49999999999999289 ) ) ;
#7077=CARTESIAN_POINT ( 'NONE',  ( 8.601468415847520532, 76.07500000273118701, 11.83890561707634781 ) ) ;
#7081=EDGE_LOOP ( 'NONE', ( #14832, #31510, #31038, #3606 ) ) ;
#7083=CARTESIAN_POINT ( 'NONE',  ( 13.91746825000000065, 71.77500000273120406, 4.522059556121114987 ) ) ;
#7088=CARTESIAN_POINT ( 'NONE',  ( -27.16883889988624290, 3.175000002731187543, -19.73931689729374028 ) ) ;
#7092=CARTESIAN_POINT ( 'NONE',  ( 3.980102097228898626E-15, 80.00000000000001421, 32.50000000000000000 ) ) ;
#7094=CARTESIAN_POINT ( 'NONE',  ( -20.75514604977248823, 42.82500000273120122, -28.56700777964554305 ) ) ;
#7097=CARTESIAN_POINT ( 'NONE',  ( 9.270509831248421762, 79.30000000000003979, -12.75976212528059861 ) ) ;
#7098=EDGE_LOOP ( 'NONE', ( #263, #21688, #16240, #27202 ) ) ;
#7100=CARTESIAN_POINT ( 'NONE',  ( 20.08610463437157279, 43.30000000000000426, -27.64615127144129758 ) ) ;
#7101=CARTESIAN_POINT ( 'NONE',  ( -23.41746825000000598, 9.724999997268804819, 7.608796670333726198 ) ) ;
#7105=CARTESIAN_POINT ( 'NONE',  ( 0.000000000000000000, 80.00000000000001421, 0.000000000000000000 ) ) ;
#7106=EDGE_LOOP ( 'NONE', ( #29800, #13825, #19104, #26534, #8996, #33088, #13540, #13742, #646, #6132, #21227, #23735, #21601, #23397, #23755, #21533, #24778, #19027, #27832, #29931, #3526, #13990 ) ) ;
#7108=CARTESIAN_POINT ( 'NONE',  ( 33.58253175000000113, 68.12500000273119838, -4.112674001490185761E-15 ) ) ;
#7110=CARTESIAN_POINT ( 'NONE',  ( 24.50000000000000355, 11.90000000000000391, 7.960532557706212486 ) ) ;
#7111=CARTESIAN_POINT ( 'NONE',  ( -7.236395654485763274, 4.524999997268825069, 22.27133577429736633 ) ) ;
#7112=CARTESIAN_POINT ( 'NONE',  ( -20.75514604977248112, 7.425000002731177773, 28.56700777964554661 ) ) ;
#7113=CARTESIAN_POINT ( 'NONE',  ( -3.880418787951127602, 6.301254276084462091, -24.50000000000000000 ) ) ;
#7115=CARTESIAN_POINT ( 'NONE',  ( -12.13525491562421088, 73.80000000000001137, -8.816778784387096835 ) ) ;
#7118=CARTESIAN_POINT ( 'NONE',  ( -15.00000000000000000, 74.35000000546236265, 4.873795443493597723 ) ) ;
#7120=CARTESIAN_POINT ( 'NONE',  ( -15.00000000000000000, 80.15000000546234560, -4.873795443493594171 ) ) ;
#7123=CARTESIAN_POINT ( 'NONE',  ( 6.486482029760649416E-15, 31.62500000273119483, 35.31076352940723240 ) ) ;
#7124=FACE_OUTER_BOUND ( 'NONE', #28383, .T. ) ;
#7126=CARTESIAN_POINT ( 'NONE',  ( 20.75514604977248467, 24.67500000273118488, -28.56700777964554305 ) ) ;
#7129=CARTESIAN_POINT ( 'NONE',  ( -32.50000000000000000, 8.600000005462376862, 10.55989012756946366 ) ) ;
#7130=CARTESIAN_POINT ( 'NONE',  ( 8.891200544363830713E-16, 81.50000000000001421, -15.00000000000000000 ) ) ;
#7132=CARTESIAN_POINT ( 'NONE',  ( -23.41746824999999887, 11.52499999726880553, -7.608796670333730638 ) ) ;
#7133=CARTESIAN_POINT ( 'NONE',  ( 33.58253175000000113, 66.12500000273119838, -4.112674001490185761E-15 ) ) ;
#7136=CARTESIAN_POINT ( 'NONE',  ( -33.58253175000000113, 1.125000002731191273, 0.000000000000000000 ) ) ;
#7137=CARTESIAN_POINT ( 'NONE',  ( 33.58253175000000113, 16.22500000273118914, -10.91162601494193574 ) ) ;
#7138=CARTESIAN_POINT ( 'NONE',  ( -23.41746825000000598, 12.22499999726881370, 7.608796670333726198 ) ) ;
#7143=EDGE_LOOP ( 'NONE', ( #3770, #3199, #16290, #18594 ) ) ;
#7147=CARTESIAN_POINT ( 'NONE',  ( -8.891200544363830713E-16, 77.50000000000000000, -15.00000000000000000 ) ) ;
#7148=CARTESIAN_POINT ( 'NONE',  ( -18.94512977948576093, 2.324999997268817342, 13.76444248337722698 ) ) ;
#7149=CARTESIAN_POINT ( 'NONE',  ( -23.41746824999999887, 11.62499999726881938, -2.867812753649727150E-15 ) ) ;
#7150=CARTESIAN_POINT ( 'NONE',  ( -20.75514604977248823, 21.07500000273118346, -28.56700777964554305 ) ) ;
#7151=CARTESIAN_POINT ( 'NONE',  ( 26.29305231718578995, 23.70000000546237828, -19.10302069950538240 ) ) ;
#7152=CARTESIAN_POINT ( 'NONE',  ( 32.50000000000000000, 65.10000000000000853, -10.55989012756945833 ) ) ;
#7153=CARTESIAN_POINT ( 'NONE',  ( 7.570916362186207671, 11.34999999453761887, 23.30088464923126779 ) ) ;
#7156=CARTESIAN_POINT ( 'NONE',  ( -20.75514604977248823, 33.07500000273117990, -28.56700777964554305 ) ) ;
#7157=CARTESIAN_POINT ( 'NONE',  ( -1.778240108872766143E-15, 32.00000000546237544, -32.49999999999999289 ) ) ;
#7160=CARTESIAN_POINT ( 'NONE',  ( -7.570916362186210335, 0.5999999999999894307, -23.30088464923126779 ) ) ;
#7161=CARTESIAN_POINT ( 'NONE',  ( -10.04305231718578462, 8.400000000000018119, 30.90933677959249337 ) ) ;
#7163=EDGE_CURVE ( 'NONE', #16413, #29502, #32254, .T. ) ;
#7165=CARTESIAN_POINT ( 'NONE',  ( -27.16883889988623935, 59.32500000273119412, 19.73931689729374739 ) ) ;
#7167=CARTESIAN_POINT ( 'NONE',  ( 6.486482029760648627E-15, 43.87500000273118417, 35.31076352940722529 ) ) ;
#7169=CARTESIAN_POINT ( 'NONE',  ( 7.570916362186207671, 9.599999999999997868, 23.30088464923126779 ) ) ;
#7170=DIRECTION ( 'NONE',  ( -0.000000000000000000, -1.000000000000000000, -0.000000000000000000 ) ) ;
#7175=CARTESIAN_POINT ( 'NONE',  ( 0.000000000000000000, 80.00000000000001421, 0.000000000000000000 ) ) ;
#7180=CARTESIAN_POINT ( 'NONE',  ( 0.000000000000000000, 80.00000000000001421, -32.50000000000000000 ) ) ;
#7181=CARTESIAN_POINT ( 'NONE',  ( -33.58253175000000113, 35.12500000273119127, 0.000000000000000000 ) ) ;
#7182=CARTESIAN_POINT ( 'NONE',  ( -20.75514604977248112, 63.67500000273116711, 28.56700777964554661 ) ) ;
#7184=ORIENTED_EDGE ( 'NONE', *, *, #26475, .T. ) ;
#7188=ORIENTED_EDGE ( 'NONE', *, *, #16049, .F. ) ;
#7193=CARTESIAN_POINT ( 'NONE',  ( -5.147494310547430452, 45.55125428154684641, -32.49999999999999289 ) ) ;
#7194=CARTESIAN_POINT ( 'NONE',  ( -10.37757302488623701, 41.77500000273118275, 31.93888565452638417 ) ) ;
#7195=VECTOR ( 'NONE', #19077, 1000.000000000000000 ) ;
#7196=CARTESIAN_POINT ( 'NONE',  ( 20.08610463437157279, 45.80000000546240102, -27.64615127144129758 ) ) ;
#7198=CARTESIAN_POINT ( 'NONE',  ( -20.75514604977248823, 22.82500000273118701, -28.56700777964554305 ) ) ;
#7199=CARTESIAN_POINT ( 'NONE',  ( 24.50000000000000000, 13.64999999453761781, 7.960532557706212486 ) ) ;
#7200=CARTESIAN_POINT ( 'NONE',  ( 10.37757302488624056, 58.77500000273119696, -31.93888565452638417 ) ) ;
#7202=CARTESIAN_POINT ( 'NONE',  ( 32.50000000000000000, 26.99999999999999645, -3.980102097228898626E-15 ) ) ;
#7204=CARTESIAN_POINT ( 'NONE',  ( 20.75514604977249178, 73.82500000273121543, 28.56700777964553950 ) ) ;
#7206=VECTOR ( 'NONE', #27584, 1000.000000000000000 ) ;
#7207=CARTESIAN_POINT ( 'NONE',  ( -24.50000000000000000, 15.00000000000001421, -3.000384657911015469E-15 ) ) ;
#7208=CARTESIAN_POINT ( 'NONE',  ( 10.37757302488624056, 60.77500000273117564, -31.93888565452638417 ) ) ;
#7210=ORIENTED_EDGE ( 'NONE', *, *, #15759, .T. ) ;
#7211=CARTESIAN_POINT ( 'NONE',  ( -27.16883889988624290, 20.92500000273117422, -19.73931689729374028 ) ) ;
#7212=CARTESIAN_POINT ( 'NONE',  ( 24.50000000000000000, 7.749999994537626336, 0.000000000000000000 ) ) ;
#7223=CARTESIAN_POINT ( 'NONE',  ( -23.41746824999999887, 2.124999997268811391, -2.867812753649727150E-15 ) ) ;
#7224=CARTESIAN_POINT ( 'NONE',  ( -33.58253175000000113, 1.125000002731191273, 0.000000000000000000 ) ) ;
#7228=EDGE_LOOP ( 'NONE', ( #12075, #31969, #7184, #936 ) ) ;
#7229=CARTESIAN_POINT ( 'NONE',  ( -10.37757302488623701, 77.77500000273118985, 31.93888565452638417 ) ) ;
#7232=CARTESIAN_POINT ( 'NONE',  ( -2.092463501923844636E-15, 62.00000000546238255, -34.17252228774368916 ) ) ;
#7234=CARTESIAN_POINT ( 'NONE',  ( -33.58253175000000113, 47.02500000273116854, -10.91162601494193218 ) ) ;
#7235=CARTESIAN_POINT ( 'NONE',  ( 7.236395654485755280, 18.22499999726881370, 22.27133577429736988 ) ) ;
#7236=CARTESIAN_POINT ( 'NONE',  ( -20.08610463437157989, 4.200000005462371178, -27.64615127144129758 ) ) ;
#7237=LINE ( 'NONE', #28183, #22903 ) ;
#7238=CARTESIAN_POINT ( 'NONE',  ( 23.41746824999999887, 19.12499999726882649, 0.000000000000000000 ) ) ;
#7239=CARTESIAN_POINT ( 'NONE',  ( -32.50000000000000000, 49.99999999999998579, 0.000000000000000000 ) ) ;
#7240=CARTESIAN_POINT ( 'NONE',  ( 24.50000000000000000, 2.000000000000001776, 0.000000000000000000 ) ) ;
#7241=CARTESIAN_POINT ( 'NONE',  ( -27.16883889988623935, 19.57500000273118701, 19.73931689729374739 ) ) ;
#7245=CARTESIAN_POINT ( 'NONE',  ( -13.91746824999999887, 81.37500000273118417, 0.000000000000000000 ) ) ;
#7246=CARTESIAN_POINT ( 'NONE',  ( -1.089172066684569321E-14, 76.75000000546238255, 15.00000000000000000 ) ) ;
#7247=CARTESIAN_POINT ( 'NONE',  ( -32.50000000000000000, 44.10000000000000142, 10.55989012756946366 ) ) ;
#7249=ORIENTED_EDGE ( 'NONE', *, *, #33483, .T. ) ;
#7261=( BOUNDED_CURVE ( )  B_SPLINE_CURVE ( 2, ( #2912, #23679, #23852, #31556, #26418, #2400, #8053, #16133, #2576, #144, #13380, #5141, #316 ),
 .UNSPECIFIED., .F., .T. ) 
 B_SPLINE_CURVE_WITH_KNOTS ( ( 3, 2, 2, 2, 2, 2, 3 ),
 ( 0.03205128205128205537, 0.03333333333333333287, 0.03589743589743589480, 0.03846153846153846367, 0.04102564102564102561, 0.04358974358974358754, 0.04487179487179487197 ),
 .UNSPECIFIED. ) 
 CURVE ( )  GEOMETRIC_REPRESENTATION_ITEM ( )  RATIONAL_B_SPLINE_CURVE ( ( 0.9755282581475768211, 0.9755282581475768211, 1.000000000000000000, 0.9510565162951535312, 1.000000000000000000, 0.9510565162951535312, 1.000000000000000000, 0.9510565162951535312, 1.000000000000000000, 0.9510565162951535312, 1.000000000000000000, 0.9755282581475768211, 0.9755282581475768211 ) ) 
 REPRESENTATION_ITEM ( '' )  );
#7262=CARTESIAN_POINT ( 'NONE',  ( 32.50000000000000711, 68.90000000000000568, 10.55989012756945122 ) ) ;
#7264=CARTESIAN_POINT ( 'NONE',  ( 33.58253175000000113, 42.12500000273116996, -4.112674001490185761E-15 ) ) ;
#7266=ADVANCED_FACE ( 'NONE', ( #13910 ), #849, .F. ) ;
#7267=EDGE_CURVE ( 'NONE', #26901, #24499, #7572, .T. ) ;
#7269=EDGE_LOOP ( 'NONE', ( #26860, #29431, #13623, #3561 ) ) ;
#7271=CARTESIAN_POINT ( 'NONE',  ( 26.29305231718579350, 42.80000000000000426, 19.10302069950537529 ) ) ;
#7274=CARTESIAN_POINT ( 'NONE',  ( 33.58253175000000113, 76.37500000273116996, -4.112674001490185761E-15 ) ) ;
#7275=EDGE_LOOP ( 'NONE', ( #1130, #10922, #15683, #27621 ) ) ;
#7280=CARTESIAN_POINT ( 'NONE',  ( -33.58253175000000113, 67.22500000273117848, 10.91162601494193929 ) ) ;
#7282=CARTESIAN_POINT ( 'NONE',  ( 7.570916362186207671, 13.60000000000000142, 23.30088464923126779 ) ) ;
#7284=CARTESIAN_POINT ( 'NONE',  ( 20.75514604977249178, 9.825000002731188786, 28.56700777964553950 ) ) ;
#7287=CARTESIAN_POINT ( 'NONE',  ( 12.13525491562421088, 76.80000000000001137, 8.816778784387095058 ) ) ;
#7290=CARTESIAN_POINT ( 'NONE',  ( 20.08610463437157279, 61.80000000546237970, -27.64615127144129758 ) ) ;
#7292=CARTESIAN_POINT ( 'NONE',  ( 12.13525491562421088, 77.05000000546239391, 8.816778784387095058 ) ) ;
#7294=CARTESIAN_POINT ( 'NONE',  ( 20.75514604977248467, 32.42500000273116711, -28.56700777964554305 ) ) ;
#7297=CARTESIAN_POINT ( 'NONE',  ( -33.58253175000000113, 21.47500000273120335, 10.91162601494193929 ) ) ;
#7298=CARTESIAN_POINT ( 'NONE',  ( -20.08610463437156923, 68.29999999999998295, 27.64615127144130113 ) ) ;
#7300=CARTESIAN_POINT ( 'NONE',  ( 10.37757302488624056, 76.52500000273118985, -31.93888565452638417 ) ) ;
#7301=CARTESIAN_POINT ( 'NONE',  ( -5.147494310547430452, 65.55125428154684641, -32.49999999999999289 ) ) ;
#7303=CARTESIAN_POINT ( 'NONE',  ( 23.41746824999999887, 14.62499999726882294, 0.000000000000000000 ) ) ;
#7304=CARTESIAN_POINT ( 'NONE',  ( -27.16883889988623935, 67.32500000273117280, 19.73931689729374739 ) ) ;
#7308=CARTESIAN_POINT ( 'NONE',  ( 20.75514604977249178, 3.825000002731174575, 28.56700777964553950 ) ) ;
#7309=CARTESIAN_POINT ( 'NONE',  ( -23.41746824999999887, 10.12499999726881938, -2.867812753649727150E-15 ) ) ;
#7311=ORIENTED_EDGE ( 'NONE', *, *, #9439, .F. ) ;
#7314=ORIENTED_EDGE ( 'NONE', *, *, #17702, .T. ) ;
#7319=DIRECTION ( 'NONE',  ( 0.000000000000000000, 0.000000000000000000, -1.000000000000000000 ) ) ;
#7320=CARTESIAN_POINT ( 'NONE',  ( 14.47279130897151589, 2.824999997268819119, 19.92008829642072953 ) ) ;
#7322=CARTESIAN_POINT ( 'NONE',  ( 7.236395654485760609, 11.02499999726880375, -22.27133577429736633 ) ) ;
#7323=CARTESIAN_POINT ( 'NONE',  ( 20.75514604977248467, 14.67500000273117955, -28.56700777964554305 ) ) ;
#7324=CARTESIAN_POINT ( 'NONE',  ( -26.29305231718578995, 26.70000000546238184, 19.10302069950538595 ) ) ;
#7325=CARTESIAN_POINT ( 'NONE',  ( 20.08610463437158344, 68.70000000000001705, 27.64615127144129403 ) ) ;
#7329=CARTESIAN_POINT ( 'NONE',  ( 27.16883889988623935, 32.57500000273119412, -19.73931689729374384 ) ) ;
#7330=CARTESIAN_POINT ( 'NONE',  ( 2.688165632520823219E-15, 79.87500000273118417, 14.63369212191046387 ) ) ;
#7333=CARTESIAN_POINT ( 'NONE',  ( -14.47279130897151589, 15.82499999726881335, -19.92008829642072598 ) ) ;
#7334=CARTESIAN_POINT ( 'NONE',  ( -10.04305231718579172, 9.599999999999997868, -30.90933677959248982 ) ) ;
#7337=CARTESIAN_POINT ( 'NONE',  ( 6.486482029760649416E-15, 47.62500000273118417, 35.31076352940723240 ) ) ;
#7339=CARTESIAN_POINT ( 'NONE',  ( -27.16883889988624290, 41.17500000273119554, -19.73931689729374028 ) ) ;
#7341=CYLINDRICAL_SURFACE ( 'NONE', #31457, 15.00000000000000000 ) ;
#7342=CARTESIAN_POINT ( 'NONE',  ( -32.50000000000000000, 49.89999999999999147, -10.55989012756945300 ) ) ;
#7346=DIRECTION ( 'NONE',  ( 1.000000000000000000, 0.000000000000000000, 0.000000000000000000 ) ) ;
#7352=CARTESIAN_POINT ( 'NONE',  ( 20.08610463437158344, 34.70000000000000995, 27.64615127144129403 ) ) ;
#7353=CARTESIAN_POINT ( 'NONE',  ( -33.58253175000000113, 29.12500000273118772, 0.000000000000000000 ) ) ;
#7360=VERTEX_POINT ( 'NONE', #25211 ) ;
#7363=ORIENTED_EDGE ( 'NONE', *, *, #9567, .F. ) ;
#7365=( BOUNDED_CURVE ( )  B_SPLINE_CURVE ( 2, ( #15921, #3372, #23976, #24309, #32017, #5946, #2868, #8513, #27041, #26545, #16258, #16425, #16094, #26877, #21070, #3211, #13161, #18667, #5440, #31519, #3041, #13843, #13513, #29105, #8013, #32187, #26377, #24143, #447, #29277, #10929, #5778, #21404, #18498, #13337, #26715, #23810, #611, #275, #11102, #21571, #21240, #783, #31683, #18999, #19165, #31849, #11265, #21741, #23637, #8177, #8681, #29603, #6104, #32513, #9176, #6447, #27546, #30275, #11755, #22561, #6277, #24470, #21900, #19660, #32846, #17428, #16919, #6609, #32352, #3535, #22069, #14007, #30103, #22236, #30447, #3868, #25138, #8844, #24798, #4033, #945, #22398, #3703, #17086, #4205, #14340, #27379, #11425, #17256, #27717, #14508, #6945, #32681, #14677, #19327, #1614, #11928, #14175, #20000, #1275 ),
 .UNSPECIFIED., .F., .T. ) 
 B_SPLINE_CURVE_WITH_KNOTS ( ( 3, 2, 2, 2, 2, 2, 2, 2, 2, 2, 2, 2, 2, 2, 2, 2, 2, 2, 2, 2, 2, 2, 2, 2, 2, 2, 2, 2, 2, 2, 2, 2, 2, 2, 2, 2, 2, 2, 2, 2, 2, 2, 2, 2, 2, 2, 2, 2, 2, 2, 3 ),
 ( 0.000000000000000000, 0.02000000000000000042, 0.04000000000000000083, 0.05999999999999999778, 0.08000000000000000167, 0.1000000000000000056, 0.1199999999999999956, 0.1400000000000000133, 0.1600000000000000033, 0.1799999999999999933, 0.2000000000000000111, 0.2200000000000000011, 0.2399999999999999911, 0.2600000000000000089, 0.2800000000000000266, 0.2999999999999999889, 0.3200000000000000067, 0.3400000000000000244, 0.3599999999999999867, 0.3800000000000000044, 0.4000000000000000222, 0.4199999999999999845, 0.4400000000000000022, 0.4600000000000000200, 0.4799999999999999822, 0.5000000000000000000, 0.5200000000000000178, 0.5400000000000000355, 0.5600000000000000533, 0.5799999999999999600, 0.5999999999999999778, 0.6199999999999999956, 0.6400000000000000133, 0.6600000000000000311, 0.6800000000000000488, 0.6999999999999999556, 0.7199999999999999734, 0.7399999999999999911, 0.7600000000000000089, 0.7800000000000000266, 0.8000000000000000444, 0.8199999999999999512, 0.8399999999999999689, 0.8599999999999999867, 0.8800000000000000044, 0.9000000000000000222, 0.9200000000000000400, 0.9399999999999999467, 0.9599999999999999645, 0.9799999999999999822, 1.000000000000000000 ),
 .UNSPECIFIED. ) 
 CURVE ( )  GEOMETRIC_REPRESENTATION_ITEM ( )  RATIONAL_B_SPLINE_CURVE ( ( 1.000000000000000000, 0.9510565162951535312, 1.000000000000000000, 0.9510565162951535312, 1.000000000000000000, 0.9510565162951535312, 1.000000000000000000, 0.9510565162951535312, 1.000000000000000000, 0.9510565162951535312, 1.000000000000000000, 0.9510565162951535312, 1.000000000000000000, 0.9510565162951535312, 1.000000000000000000, 0.9510565162951535312, 1.000000000000000000, 0.9510565162951535312, 1.000000000000000000, 0.9510565162951535312, 1.000000000000000000, 0.9510565162951535312, 1.000000000000000000, 0.9510565162951535312, 1.000000000000000000, 0.9510565162951535312, 1.000000000000000000, 0.9510565162951535312, 1.000000000000000000, 0.9510565162951535312, 1.000000000000000000, 0.9510565162951535312, 1.000000000000000000, 0.9510565162951535312, 1.000000000000000000, 0.9510565162951535312, 1.000000000000000000, 0.9510565162951535312, 1.000000000000000000, 0.9510565162951535312, 1.000000000000000000, 0.9510565162951535312, 1.000000000000000000, 0.9510565162951535312, 1.000000000000000000, 0.9510565162951535312, 1.000000000000000000, 0.9510565162951535312, 1.000000000000000000, 0.9510565162951535312, 1.000000000000000000, 0.9510565162951535312, 1.000000000000000000, 0.9510565162951535312, 1.000000000000000000, 0.9510565162951535312, 1.000000000000000000, 0.9510565162951535312, 1.000000000000000000, 0.9510565162951535312, 1.000000000000000000, 0.9510565162951535312, 1.000000000000000000, 0.9510565162951535312, 1.000000000000000000, 0.9510565162951535312, 1.000000000000000000, 0.9510565162951535312, 1.000000000000000000, 0.9510565162951535312, 1.000000000000000000, 0.9510565162951535312, 1.000000000000000000, 0.9510565162951535312, 1.000000000000000000, 0.9510565162951535312, 1.000000000000000000, 0.9510565162951535312, 1.000000000000000000, 0.9510565162951535312, 1.000000000000000000, 0.9510565162951535312, 1.000000000000000000, 0.9510565162951535312, 1.000000000000000000, 0.9510565162951535312, 1.000000000000000000, 0.9510565162951535312, 1.000000000000000000, 0.9510565162951535312, 1.000000000000000000, 0.9510565162951535312, 1.000000000000000000, 0.9510565162951535312, 1.000000000000000000, 0.9510565162951535312, 1.000000000000000000, 0.9510565162951535312, 1.000000000000000000, 0.9510565162951535312, 1.000000000000000000 ) ) 
 REPRESENTATION_ITEM ( '' )  );
#7368=CARTESIAN_POINT ( 'NONE',  ( 33.58253175000000113, 36.47500000273119269, -10.91162601494193751 ) ) ;
#7370=CARTESIAN_POINT ( 'NONE',  ( 26.29305231718578995, 45.70000000546237118, -19.10302069950538240 ) ) ;
#7371=( BOUNDED_CURVE ( )  B_SPLINE_CURVE ( 2, ( #19288, #29731, #14139, #16881, #16386, #22199, #6064, #11549, #26839, #16547, #22031, #11890, #6236 ),
 .UNSPECIFIED., .F., .T. ) 
 B_SPLINE_CURVE_WITH_KNOTS ( ( 3, 2, 2, 2, 2, 2, 3 ),
 ( 0.8269230769230769829, 0.8282051282051282604, 0.8307692307692308153, 0.8333333333333333703, 0.8358974358974359253, 0.8384615384615384803, 0.8397435897435897578 ),
 .UNSPECIFIED. ) 
 CURVE ( )  GEOMETRIC_REPRESENTATION_ITEM ( )  RATIONAL_B_SPLINE_CURVE ( ( 0.9755282581475768211, 0.9755282581475778203, 1.000000000000000000, 0.9510565162951535312, 1.000000000000000000, 0.9510565162951535312, 1.000000000000000000, 0.9510565162951535312, 1.000000000000000000, 0.9510565162951535312, 1.000000000000000000, 0.9755282581475768211, 0.9755282581475768211 ) ) 
 REPRESENTATION_ITEM ( '' )  );
#7373=CARTESIAN_POINT ( 'NONE',  ( 20.75514604977249178, 23.82500000273118701, 28.56700777964553950 ) ) ;
#7375=CARTESIAN_POINT ( 'NONE',  ( 27.16883889988624290, 46.17500000273119554, 19.73931689729373673 ) ) ;
#7378=CARTESIAN_POINT ( 'NONE',  ( -2.092463501923844636E-15, 29.49999999999999645, -34.17252228774368916 ) ) ;
#7380=CARTESIAN_POINT ( 'NONE',  ( -10.37757302488624411, 72.72500000273119269, -31.93888565452638417 ) ) ;
#7383=CARTESIAN_POINT ( 'NONE',  ( -20.75514604977248112, 57.67500000273118843, 28.56700777964554661 ) ) ;
#7385=CARTESIAN_POINT ( 'NONE',  ( 5.779280353836490358E-15, 7.000000005462371000, 32.49999999999999289 ) ) ;
#7386=CARTESIAN_POINT ( 'NONE',  ( -10.37757302488623701, 19.52500000273118985, 31.93888565452638417 ) ) ;
#7387=CARTESIAN_POINT ( 'NONE',  ( -15.14183272437241889, 10.44999999453763095, -20.84094480462497856 ) ) ;
#7396=CIRCLE ( 'NONE', #16188, 24.50000000000000000 ) ;
#7400=CARTESIAN_POINT ( 'NONE',  ( -7.236395654485763274, 2.524999997268823293, 22.27133577429736633 ) ) ;
#7401=CARTESIAN_POINT ( 'NONE',  ( 20.08610463437158344, 73.20000000546235697, 27.64615127144129403 ) ) ;
#7406=CARTESIAN_POINT ( 'NONE',  ( -10.37757302488624411, 72.97500000273119269, -31.93888565452638417 ) ) ;
#7409=CARTESIAN_POINT ( 'NONE',  ( -33.58253175000000113, 51.47500000273118559, 10.91162601494193929 ) ) ;
#7410=CARTESIAN_POINT ( 'NONE',  ( -2.092463501923844636E-15, 66.00000000546239676, -34.17252228774368916 ) ) ;
#7413=CARTESIAN_POINT ( 'NONE',  ( -33.58253175000000113, 39.02500000273118985, -10.91162601494193218 ) ) ;
#7414=CARTESIAN_POINT ( 'NONE',  ( -18.94512977948575738, 17.42499999726882010, -13.76444248337723231 ) ) ;
#7415=CARTESIAN_POINT ( 'NONE',  ( -20.75514604977248112, 69.67500000273119554, 28.56700777964554661 ) ) ;
#7416=CARTESIAN_POINT ( 'NONE',  ( 26.29305231718579350, 3.300000005462377928, 19.10302069950537529 ) ) ;
#7418=DIRECTION ( 'NONE',  ( 0.000000000000000000, 0.000000000000000000, -1.000000000000000000 ) ) ;
#7419=CARTESIAN_POINT ( 'NONE',  ( 6.277390505771533514E-15, 46.50000000000001421, 34.17252228774368916 ) ) ;
#7420=CARTESIAN_POINT ( 'NONE',  ( 24.50000000000000000, 1.899999999999998135, 7.960532557706212486 ) ) ;
#7421=CARTESIAN_POINT ( 'NONE',  ( -10.37757302488624411, 16.97500000273119269, -31.93888565452638417 ) ) ;
#7422=CARTESIAN_POINT ( 'NONE',  ( 19.82091636218621389, 0.2000000000000057288, -14.40073868116559197 ) ) ;
#7424=CARTESIAN_POINT ( 'NONE',  ( -13.91746824999999887, 77.37500000273116996, 0.000000000000000000 ) ) ;
#7425=CARTESIAN_POINT ( 'NONE',  ( -33.58253175000000113, 77.47500000273120691, 10.91162601494193929 ) ) ;
#7428=VERTEX_POINT ( 'NONE', #4617 ) ;
#7433=CIRCLE ( 'NONE', #26618, 32.50000000000000000 ) ;
#7443=CARTESIAN_POINT ( 'NONE',  ( 13.91746824999999532, 72.47500000273119269, -4.522059556121118540 ) ) ;
#7445=CARTESIAN_POINT ( 'NONE',  ( 10.37757302488624767, 47.72500000273119269, 31.93888565452638417 ) ) ;
#7452=CARTESIAN_POINT ( 'NONE',  ( 33.58253175000000113, 78.47500000273116427, -10.91162601494193751 ) ) ;
#7453=ORIENTED_EDGE ( 'NONE', *, *, #14536, .F. ) ;
#7459=CARTESIAN_POINT ( 'NONE',  ( 4.445600272181915325E-13, 14.00000000546237544, -32.50000000000000000 ) ) ;
#7460=CARTESIAN_POINT ( 'NONE',  ( 6.486482029760649416E-15, 59.62500000273118417, 35.31076352940723240 ) ) ;
#7463=CARTESIAN_POINT ( 'NONE',  ( 7.570916362186207671, 11.59999999999999964, 23.30088464923126779 ) ) ;
#7464=CARTESIAN_POINT ( 'NONE',  ( 1.507698388325705758E-15, 3.624999997268822938, -24.62258325217400312 ) ) ;
#7465=CARTESIAN_POINT ( 'NONE',  ( -33.58253175000000113, 11.02500000273117919, -10.91162601494193218 ) ) ;
#7466=CARTESIAN_POINT ( 'NONE',  ( 5.147494310547434893, 28.55125428154685352, 32.49999999999999289 ) ) ;
#7468=CARTESIAN_POINT ( 'NONE',  ( 10.04305231718578817, 37.39999999999999147, -30.90933677959249337 ) ) ;
#7469=DIRECTION ( 'NONE',  ( 0.000000000000000000, 0.000000000000000000, -1.000000000000000000 ) ) ;
#7470=CARTESIAN_POINT ( 'NONE',  ( 26.29305231718578995, 19.70000000546237473, -19.10302069950538240 ) ) ;
#7474=CARTESIAN_POINT ( 'NONE',  ( 15.00000000000000000, 71.35000000546237686, -4.873795443493596835 ) ) ;
#7476=( BOUNDED_CURVE ( )  B_SPLINE_CURVE ( 2, ( #11108, #14180, #29449, #24149, #8687, #11595, #16591, #8348, #24315, #24636, #27048, #29949, #3541 ),
 .UNSPECIFIED., .F., .F. ) 
 B_SPLINE_CURVE_WITH_KNOTS ( ( 3, 2, 2, 2, 2, 2, 3 ),
 ( 0.5064102564102563875, 0.5076923076923076650, 0.5102564102564102200, 0.5128205128205127750, 0.5153846153846153300, 0.5179487179487179960, 0.5192307692307692735 ),
 .UNSPECIFIED. ) 
 CURVE ( )  GEOMETRIC_REPRESENTATION_ITEM ( )  RATIONAL_B_SPLINE_CURVE ( ( 0.9755282581475768211, 0.9755282581475768211, 1.000000000000000000, 0.9510565162951535312, 1.000000000000000000, 0.9510565162951535312, 1.000000000000000000, 0.9510565162951535312, 1.000000000000000000, 0.9510565162951535312, 1.000000000000000000, 0.9755282581475768211, 0.9755282581475768211 ) ) 
 REPRESENTATION_ITEM ( '' )  );
#7477=CARTESIAN_POINT ( 'NONE',  ( 33.58253175000000113, 34.12500000273119127, -4.112674001490185761E-15 ) ) ;
#7480=CARTESIAN_POINT ( 'NONE',  ( -33.58253175000000113, 19.47500000273117493, 10.91162601494193929 ) ) ;
#7481=CARTESIAN_POINT ( 'NONE',  ( -12.13525491562421088, 79.80000000000001137, -8.816778784387096835 ) ) ;
#7483=CARTESIAN_POINT ( 'NONE',  ( 27.16883889988623935, 76.32500000273118701, -19.73931689729374384 ) ) ;
#7484=CARTESIAN_POINT ( 'NONE',  ( 20.08610463437157279, 59.80000000546235839, -27.64615127144129758 ) ) ;
#7486=CARTESIAN_POINT ( 'NONE',  ( -7.236395654485763274, 16.02499999726880731, 22.27133577429736633 ) ) ;
#7487=CARTESIAN_POINT ( 'NONE',  ( -20.75514604977248112, 67.42500000273118133, 28.56700777964554661 ) ) ;
#7490=CARTESIAN_POINT ( 'NONE',  ( -33.58253175000000113, 5.225000002731188253, 10.91162601494193929 ) ) ;
#7491=CARTESIAN_POINT ( 'NONE',  ( 23.41746825000000243, 2.524999997268798868, 7.608796670333735079 ) ) ;
#7493=ORIENTED_EDGE ( 'NONE', *, *, #15171, .T. ) ;
#7495=VERTEX_POINT ( 'NONE', #25561 ) ;
#7497=CARTESIAN_POINT ( 'NONE',  ( -5.147494310547427787, 79.55125428154684641, -32.49999999999999289 ) ) ;
#7499=CARTESIAN_POINT ( 'NONE',  ( 7.236395654485755280, 2.724999997268801266, 22.27133577429736988 ) ) ;
#7500=CARTESIAN_POINT ( 'NONE',  ( 14.47279130897151767, 12.92499999726881832, -19.92008829642072598 ) ) ;
#7501=CARTESIAN_POINT ( 'NONE',  ( -10.37757302488624411, 12.97500000273119092, -31.93888565452638417 ) ) ;
#7502=CARTESIAN_POINT ( 'NONE',  ( -2.092463501923844636E-15, 20.00000000546236834, -34.17252228774368916 ) ) ;
#7503=CARTESIAN_POINT ( 'NONE',  ( 20.08610463437158344, 66.69999999999997442, 27.64615127144129403 ) ) ;
#7504=CARTESIAN_POINT ( 'NONE',  ( 4.635254915624212657, 76.85000000546237686, 14.26584774442730286 ) ) ;
#7507=CARTESIAN_POINT ( 'NONE',  ( -20.75514604977248823, 31.07500000273118701, -28.56700777964554305 ) ) ;
#7508=CARTESIAN_POINT ( 'NONE',  ( 5.147494310547434893, 43.05125428700922185, 32.49999999999999289 ) ) ;
#7510=AXIS2_PLACEMENT_3D ( 'NONE', #23474, #21076, #31689 ) ;
#7511=CARTESIAN_POINT ( 'NONE',  ( -4.523095164977116484E-15, 16.62499999726881583, 24.62258325217400312 ) ) ;
#7512=CARTESIAN_POINT ( 'NONE',  ( 6.277390505771533514E-15, 6.499999999999998224, 34.17252228774368916 ) ) ;
#7513=DIRECTION ( 'NONE',  ( 0.000000000000000000, 0.000000000000000000, -1.000000000000000000 ) ) ;
#7515=CARTESIAN_POINT ( 'NONE',  ( 27.16883889988624290, 49.92500000273120264, 19.73931689729373673 ) ) ;
#7517=CARTESIAN_POINT ( 'NONE',  ( 10.37757302488624767, 39.97500000273118559, 31.93888565452638417 ) ) ;
#7518=CARTESIAN_POINT ( 'NONE',  ( 10.04305231718578817, 45.39999999999999858, -30.90933677959249337 ) ) ;
#7521=CARTESIAN_POINT ( 'NONE',  ( -24.50000000000000711, 9.100000000000003197, 7.960532557706201828 ) ) ;
#7522=CARTESIAN_POINT ( 'NONE',  ( -5.147494310547430452, 22.05125428700922185, -32.49999999999999289 ) ) ;
#7525=CARTESIAN_POINT ( 'NONE',  ( 0.000000000000000000, 0.000000000000000000, 0.000000000000000000 ) ) ;
#7526=DIRECTION ( 'NONE',  ( 0.000000000000000000, -1.000000000000000000, 0.000000000000000000 ) ) ;
#7527=CYLINDRICAL_SURFACE ( 'NONE', #17053, 32.50000000000000000 ) ;
#7531=CARTESIAN_POINT ( 'NONE',  ( -33.58253175000000113, 25.12500000273118417, 0.000000000000000000 ) ) ;
#7536=VERTEX_POINT ( 'NONE', #7017 ) ;
#7542=CARTESIAN_POINT ( 'NONE',  ( 20.75514604977248467, 34.67500000273118843, -28.56700777964554305 ) ) ;
#7543=CARTESIAN_POINT ( 'NONE',  ( -32.50000000000000000, 34.40000000546236691, -10.55989012756945478 ) ) ;
#7546=CARTESIAN_POINT ( 'NONE',  ( 33.58253175000000113, 22.12500000273118062, -4.112674001490185761E-15 ) ) ;
#7547=CARTESIAN_POINT ( 'NONE',  ( -2.375766604868044141, 81.55125428154683220, -14.99999999999999822 ) ) ;
#7548=CARTESIAN_POINT ( 'NONE',  ( -33.58253175000000113, 47.37500000273120548, 0.000000000000000000 ) ) ;
#7551=CARTESIAN_POINT ( 'NONE',  ( 32.50000000000000711, 28.89999999999998792, 10.55989012756945122 ) ) ;
#7553=CARTESIAN_POINT ( 'NONE',  ( -20.75514604977248112, 71.42500000273119554, 28.56700777964554661 ) ) ;
#7554=DIRECTION ( 'NONE',  ( -0.000000000000000000, -1.000000000000000000, -0.000000000000000000 ) ) ;
#7555=CARTESIAN_POINT ( 'NONE',  ( 4.023268246324634798E-14, 10.24999999453763166, -24.50000000000000355 ) ) ;
#7556=CARTESIAN_POINT ( 'NONE',  ( -10.37757302488624411, 62.97500000273120691, -31.93888565452638417 ) ) ;
#7557=CARTESIAN_POINT ( 'NONE',  ( -26.29305231718579350, 40.30000000546237970, -19.10302069950537884 ) ) ;
#7558=CARTESIAN_POINT ( 'NONE',  ( 33.58253175000000113, 14.12500000273120193, -4.112674001490185761E-15 ) ) ;
#7564=CARTESIAN_POINT ( 'NONE',  ( 26.29305231718579350, 18.79999999999998295, 19.10302069950537529 ) ) ;
#7572=( BOUNDED_CURVE ( )  B_SPLINE_CURVE ( 2, ( #33616, #14749, #15911, #14920, #20075, #28130, #12516, #22983, #25387, #17499, #20415, #17668, #4786 ),
 .UNSPECIFIED., .F., .T. ) 
 B_SPLINE_CURVE_WITH_KNOTS ( ( 3, 2, 2, 2, 2, 2, 3 ),
 ( 0.7884615384615384359, 0.7897435897435897134, 0.7923076923076922684, 0.7948717948717948234, 0.7974358974358974894, 0.8000000000000000444, 0.8012820512820513219 ),
 .UNSPECIFIED. ) 
 CURVE ( )  GEOMETRIC_REPRESENTATION_ITEM ( )  RATIONAL_B_SPLINE_CURVE ( ( 0.9755282581475768211, 0.9755282581475768211, 1.000000000000000000, 0.9510565162951535312, 1.000000000000000000, 0.9510565162951535312, 1.000000000000000000, 0.9510565162951535312, 1.000000000000000000, 0.9510565162951535312, 1.000000000000000000, 0.9755282581475768211, 0.9755282581475768211 ) ) 
 REPRESENTATION_ITEM ( '' )  );
#7573=DIRECTION ( 'NONE',  ( 0.000000000000000000, 0.000000000000000000, -1.000000000000000000 ) ) ;
#7574=CARTESIAN_POINT ( 'NONE',  ( -26.29305231718578995, 76.70000000546239960, 19.10302069950538595 ) ) ;
#7579=ORIENTED_EDGE ( 'NONE', *, *, #20795, .F. ) ;
#7580=CARTESIAN_POINT ( 'NONE',  ( 10.37757302488624767, 73.97500000273119269, 31.93888565452638417 ) ) ;
#7585=CARTESIAN_POINT ( 'NONE',  ( 10.37757302488624056, 54.77500000273119696, -31.93888565452638417 ) ) ;
#7586=CARTESIAN_POINT ( 'NONE',  ( 32.50000000000000000, 63.50000000546238255, -3.980102097228898626E-15 ) ) ;
#7587=CARTESIAN_POINT ( 'NONE',  ( -32.50000000000000000, 10.40000000546237757, -10.55989012756945300 ) ) ;
#7588=CARTESIAN_POINT ( 'NONE',  ( 20.75514604977249178, 41.82500000273119412, 28.56700777964553950 ) ) ;
#7589=CARTESIAN_POINT ( 'NONE',  ( 32.50000000000000711, 54.90000000000001279, 10.55989012756945122 ) ) ;
#7590=CARTESIAN_POINT ( 'NONE',  ( 6.486482029760649416E-15, 67.87500000273116996, 35.31076352940723240 ) ) ;
#7591=CARTESIAN_POINT ( 'NONE',  ( 20.08610463437158344, 3.200000005462373398, 27.64615127144129403 ) ) ;
#7593=CARTESIAN_POINT ( 'NONE',  ( -4.523095164977117273E-15, 18.62499999726881583, 24.62258325217400312 ) ) ;
#7594=CARTESIAN_POINT ( 'NONE',  ( -10.04305231718578462, 44.39999999999999147, 30.90933677959249337 ) ) ;
#7595=DIRECTION ( 'NONE',  ( -0.000000000000000000, 1.000000000000000000, -0.000000000000000000 ) ) ;
#7596=CARTESIAN_POINT ( 'NONE',  ( 27.16883889988623935, 10.57500000273120477, -19.73931689729374384 ) ) ;
#7598=CARTESIAN_POINT ( 'NONE',  ( -8.960552108402742093E-16, 80.87500000273116996, -14.63369212191046387 ) ) ;
#7599=CARTESIAN_POINT ( 'NONE',  ( 10.37757302488624056, 76.77500000273118985, -31.93888565452638417 ) ) ;
#7614=CARTESIAN_POINT ( 'NONE',  ( -20.75514604977248823, 44.82500000273118701, -28.56700777964554305 ) ) ;
#7616=CARTESIAN_POINT ( 'NONE',  ( 20.08610463437158344, 21.20000000546238894, 27.64615127144129403 ) ) ;
#7619=CARTESIAN_POINT ( 'NONE',  ( -32.50000000000000000, 4.400000005462393560, -10.55989012756945300 ) ) ;
#7621=CARTESIAN_POINT ( 'NONE',  ( 10.37757302488624056, 78.77500000273118985, -31.93888565452638417 ) ) ;
#7625=ORIENTED_EDGE ( 'NONE', *, *, #17634, .T. ) ;
#7626=CARTESIAN_POINT ( 'NONE',  ( 5.147494310547434893, 29.05125428700921475, 32.49999999999999289 ) ) ;
#7627=CARTESIAN_POINT ( 'NONE',  ( 33.58253175000000113, 62.12500000273119127, -4.112674001490185761E-15 ) ) ;
#7630=CARTESIAN_POINT ( 'NONE',  ( 23.41746824999999887, 5.124999997268814056, 0.000000000000000000 ) ) ;
#7631=CARTESIAN_POINT ( 'NONE',  ( -20.75514604977248112, 3.425000002731186655, 28.56700777964554661 ) ) ;
#7634=CARTESIAN_POINT ( 'NONE',  ( 0.000000000000000000, 80.00000000000001421, 0.000000000000000000 ) ) ;
#7636=CARTESIAN_POINT ( 'NONE',  ( 4.023268246324634798E-14, 8.499999999999992895, -24.50000000000000355 ) ) ;
#7640=CARTESIAN_POINT ( 'NONE',  ( -9.270509831248421762, 70.55000000546237970, 12.75976212528060039 ) ) ;
#7642=CARTESIAN_POINT ( 'NONE',  ( -27.16883889988624290, 28.92500000273118133, -19.73931689729374028 ) ) ;
#7645=CARTESIAN_POINT ( 'NONE',  ( -27.16883889988623935, 21.57500000273118701, 19.73931689729374739 ) ) ;
#7648=CARTESIAN_POINT ( 'NONE',  ( -10.37757302488623701, 75.52500000273118985, 31.93888565452638417 ) ) ;
#7649=CARTESIAN_POINT ( 'NONE',  ( -20.08610463437156923, 26.80000000546238326, 27.64615127144130113 ) ) ;
#7651=DIRECTION ( 'NONE',  ( -0.000000000000000000, -1.000000000000000000, -0.000000000000000000 ) ) ;
#7652=CARTESIAN_POINT ( 'NONE',  ( 20.75514604977248467, 66.42500000273119554, -28.56700777964554305 ) ) ;
#7655=CARTESIAN_POINT ( 'NONE',  ( 10.37757302488624767, 9.725000002731187365, 31.93888565452638417 ) ) ;
#7656=CARTESIAN_POINT ( 'NONE',  ( 7.236395654485760609, 17.52499999726880731, -22.27133577429736633 ) ) ;
#7660=VERTEX_POINT ( 'NONE', #4275 ) ;
#7662=CARTESIAN_POINT ( 'NONE',  ( 2.667360163309149608E-15, 79.50000000000001421, -32.50000000000000000 ) ) ;
#7664=CARTESIAN_POINT ( 'NONE',  ( 27.16883889988624290, 77.92500000273116711, 19.73931689729373673 ) ) ;
#7665=CARTESIAN_POINT ( 'NONE',  ( 18.94512977948575738, 4.924999997268808549, 13.76444248337723408 ) ) ;
#7666=CARTESIAN_POINT ( 'NONE',  ( 14.47279130897151767, 16.92499999726880944, -19.92008829642072598 ) ) ;
#7667=CARTESIAN_POINT ( 'NONE',  ( 10.37757302488624767, 13.97500000273119092, 31.93888565452638417 ) ) ;
#7668=CARTESIAN_POINT ( 'NONE',  ( 10.04305231718579705, 17.10000000546238397, 30.90933677959248982 ) ) ;
#7670=CARTESIAN_POINT ( 'NONE',  ( 6.277390505771533514E-15, 68.50000000000002842, 34.17252228774368916 ) ) ;
#7671=CARTESIAN_POINT ( 'NONE',  ( 4.635254915624209993, 77.65000000546237402, -14.26584774442730463 ) ) ;
#7672=LINE ( 'NONE', #15232, #9934 ) ;
#7674=CARTESIAN_POINT ( 'NONE',  ( 0.000000000000000000, 80.00000000000001421, 0.000000000000000000 ) ) ;
#7676=SHAPE_DEFINITION_REPRESENTATION ( #23580, #22108 ) ;
#7678=CARTESIAN_POINT ( 'NONE',  ( 23.41746824999999887, 15.12499999726882294, 0.000000000000000000 ) ) ;
#7679=CARTESIAN_POINT ( 'NONE',  ( -32.50000000000000000, 9.899999999999979039, -10.55989012756945478 ) ) ;
#7682=CARTESIAN_POINT ( 'NONE',  ( -10.37757302488624411, 48.72500000273119269, -31.93888565452638417 ) ) ;
#7684=CARTESIAN_POINT ( 'NONE',  ( 27.16883889988623935, 40.57500000273117280, -19.73931689729374384 ) ) ;
#7685=CARTESIAN_POINT ( 'NONE',  ( 10.04305231718578817, 23.90000000546238468, -30.90933677959249337 ) ) ;
#7687=CARTESIAN_POINT ( 'NONE',  ( -24.50000000000000000, 9.000000000000007105, -3.000384657911015469E-15 ) ) ;
#7697=CYLINDRICAL_SURFACE ( 'NONE', #10687, 32.50000000000000000 ) ;
#7698=CARTESIAN_POINT ( 'NONE',  ( -2.162160676586882350E-15, 28.62500000273117706, -35.31076352940722529 ) ) ;
#7700=ORIENTED_EDGE ( 'NONE', *, *, #19161, .F. ) ;
#7702=EDGE_CURVE ( 'NONE', #1605, #24457, #31673, .T. ) ;
#7704=VERTEX_POINT ( 'NONE', #6093 ) ;
#7707=EDGE_LOOP ( 'NONE', ( #19523, #8826, #10165, #21519, #10914, #6095, #27150, #19146 ) ) ;
#7710=CARTESIAN_POINT ( 'NONE',  ( 33.58253175000000113, 34.37500000273119127, -4.112674001490185761E-15 ) ) ;
#7711=CARTESIAN_POINT ( 'NONE',  ( -32.50000000000000000, 38.50000000546238965, 0.000000000000000000 ) ) ;
#7714=CARTESIAN_POINT ( 'NONE',  ( 33.58253175000000823, 24.02500000273117564, 10.91162601494192863 ) ) ;
#7716=CARTESIAN_POINT ( 'NONE',  ( -20.75514604977248823, 49.07500000273117280, -28.56700777964554305 ) ) ;
#7719=CARTESIAN_POINT ( 'NONE',  ( -26.29305231718578995, 26.20000000000000284, 19.10302069950538595 ) ) ;
#7721=CARTESIAN_POINT ( 'NONE',  ( -10.37757302488623701, 71.52500000273120406, 31.93888565452638417 ) ) ;
#7723=CARTESIAN_POINT ( 'NONE',  ( -20.08610463437156923, 38.29999999999999005, 27.64615127144130113 ) ) ;
#7724=CARTESIAN_POINT ( 'NONE',  ( -2.162160676586882350E-15, 58.87500000273117706, -35.31076352940722529 ) ) ;
#7726=CARTESIAN_POINT ( 'NONE',  ( 27.16883889988624290, 11.92500000273116711, 19.73931689729373673 ) ) ;
#7729=CARTESIAN_POINT ( 'NONE',  ( -27.16883889988623935, 3.575000002731199000, 19.73931689729374739 ) ) ;
#7731=CARTESIAN_POINT ( 'NONE',  ( 5.147494310547426899, 45.94874572391552903, -32.50000000000000000 ) ) ;
#7736=CARTESIAN_POINT ( 'NONE',  ( 20.08610463437157279, 61.30000000000001137, -27.64615127144129758 ) ) ;
#7738=CARTESIAN_POINT ( 'NONE',  ( 23.41746824999999887, 1.124999997268810725, 0.000000000000000000 ) ) ;
#7739=CARTESIAN_POINT ( 'NONE',  ( -32.50000000000000000, 68.60000000546237686, 10.55989012756946366 ) ) ;
#7748=CARTESIAN_POINT ( 'NONE',  ( -20.75514604977248823, 51.07500000273116569, -28.56700777964554305 ) ) ;
#7749=CARTESIAN_POINT ( 'NONE',  ( 32.50000000000000000, 59.60000000546236976, -10.55989012756945833 ) ) ;
#7753=CARTESIAN_POINT ( 'NONE',  ( -2.162160676586881955E-15, 44.62500000273119838, -35.31076352940723240 ) ) ;
#7755=CARTESIAN_POINT ( 'NONE',  ( -33.58253175000000113, 65.47500000273117848, 10.91162601494193929 ) ) ;
#7756=EDGE_CURVE ( 'NONE', #14241, #12812, #18989, .T. ) ;
#7757=CARTESIAN_POINT ( 'NONE',  ( 20.08610463437157279, 1.800000005462388364, -27.64615127144129758 ) ) ;
#7760=CARTESIAN_POINT ( 'NONE',  ( -32.50000000000000000, 43.90000000000001279, -10.55989012756945478 ) ) ;
#7762=CARTESIAN_POINT ( 'NONE',  ( -27.16883889988624290, 9.175000002731191984, -19.73931689729374028 ) ) ;
#7763=CYLINDRICAL_SURFACE ( 'NONE', #4142, 26.50000000000000355 ) ;
#7765=CARTESIAN_POINT ( 'NONE',  ( 2.688165632520823219E-15, 71.37500000273119838, 14.63369212191046387 ) ) ;
#7766=CARTESIAN_POINT ( 'NONE',  ( 9.270509831248425314, 74.95000000546237118, 12.75976212528059683 ) ) ;
#7767=CYLINDRICAL_SURFACE ( 'NONE', #7893, 32.50000000000000000 ) ;
#7781=CARTESIAN_POINT ( 'NONE',  ( -10.37757302488623701, 43.52500000273118275, 31.93888565452638417 ) ) ;
#7783=CARTESIAN_POINT ( 'NONE',  ( -32.50000000000000000, 2.500000005462382546, 0.000000000000000000 ) ) ;
#7787=CARTESIAN_POINT ( 'NONE',  ( 10.37757302488624767, 75.97500000273119269, 31.93888565452638417 ) ) ;
#7791=EDGE_CURVE ( 'NONE', #2565, #12293, #4964, .T. ) ;
#7792=ORIENTED_EDGE ( 'NONE', *, *, #6314, .T. ) ;
#7794=CARTESIAN_POINT ( 'NONE',  ( -33.58253175000000113, 61.02500000273118985, -10.91162601494193218 ) ) ;
#7796=EDGE_CURVE ( 'NONE', #18361, #12435, #33209, .T. ) ;
#7798=CARTESIAN_POINT ( 'NONE',  ( -14.47279130897151767, 1.824999997268821783, -19.92008829642072598 ) ) ;
#7799=CARTESIAN_POINT ( 'NONE',  ( 33.58253175000000823, 2.025000002731202287, 10.91162601494192863 ) ) ;
#7802=CARTESIAN_POINT ( 'NONE',  ( 5.147494310547434893, 36.55125428154683220, 32.49999999999999289 ) ) ;
#7804=CARTESIAN_POINT ( 'NONE',  ( 26.29305231718579350, 75.30000000546237970, 19.10302069950537529 ) ) ;
#7808=CARTESIAN_POINT ( 'NONE',  ( 15.00000000000000000, 71.25000000546238255, -1.836970198721029589E-15 ) ) ;
#7810=CARTESIAN_POINT ( 'NONE',  ( 33.58253175000000113, 34.22500000273117848, -10.91162601494193751 ) ) ;
#7813=CARTESIAN_POINT ( 'NONE',  ( -33.58253175000000113, 13.37500000273117351, 0.000000000000000000 ) ) ;
#7814=CARTESIAN_POINT ( 'NONE',  ( -10.04305231718578462, 64.40000000000000568, 30.90933677959249337 ) ) ;
#7816=CARTESIAN_POINT ( 'NONE',  ( -20.75514604977248112, 75.42500000273120975, 28.56700777964554661 ) ) ;
#7817=CARTESIAN_POINT ( 'NONE',  ( -5.147494310547423346, 26.94874572391553613, 32.50000000000000000 ) ) ;
#7821=CARTESIAN_POINT ( 'NONE',  ( -10.37757302488623701, 61.52500000273120406, 31.93888565452638417 ) ) ;
#7825=CARTESIAN_POINT ( 'NONE',  ( 6.486482029760648627E-15, 7.625000002731170845, 35.31076352940722529 ) ) ;
#7826=CARTESIAN_POINT ( 'NONE',  ( -4.523095164977116484E-15, 2.124999997268812280, 24.62258325217400312 ) ) ;
#7830=ORIENTED_EDGE ( 'NONE', *, *, #16499, .T. ) ;
#7834=CARTESIAN_POINT ( 'NONE',  ( 32.50000000000000000, 27.60000000546238752, -10.55989012756945833 ) ) ;
#7836=CARTESIAN_POINT ( 'NONE',  ( -23.41746825000000243, 17.52499999726881796, -7.608796670333730638 ) ) ;
#7837=CARTESIAN_POINT ( 'NONE',  ( 27.16883889988624290, 14.17500000273119731, 19.73931689729373673 ) ) ;
#7839=CARTESIAN_POINT ( 'NONE',  ( 6.277390505771533514E-15, 62.50000000000000000, 34.17252228774368916 ) ) ;
#7840=CARTESIAN_POINT ( 'NONE',  ( 2.375766604868040144, 76.80125428700922896, 15.00000000000000178 ) ) ;
#7843=CARTESIAN_POINT ( 'NONE',  ( -13.91746824999999887, 79.37500000273118417, 0.000000000000000000 ) ) ;
#7847=CARTESIAN_POINT ( 'NONE',  ( 15.14183272437242067, 15.69999999999999929, 20.84094480462498211 ) ) ;
#7848=CARTESIAN_POINT ( 'NONE',  ( 26.29305231718578995, 5.199999999999982414, -19.10302069950538240 ) ) ;
#7851=CARTESIAN_POINT ( 'NONE',  ( -10.37757302488623701, 49.52500000273118985, 31.93888565452638417 ) ) ;
#7853=CARTESIAN_POINT ( 'NONE',  ( -2.162160676586882350E-15, 38.87500000273120548, -35.31076352940722529 ) ) ;
#7854=DIRECTION ( 'NONE',  ( 0.000000000000000000, 0.000000000000000000, 1.000000000000000000 ) ) ;
#7861=CARTESIAN_POINT ( 'NONE',  ( -1.778240108872766143E-15, 2.000000005462374997, -32.49999999999999289 ) ) ;
#7864=CARTESIAN_POINT ( 'NONE',  ( 3.880418787951178228, 18.19874571299077104, -24.49999999999998224 ) ) ;
#7865=CARTESIAN_POINT ( 'NONE',  ( 33.58253175000000823, 26.02500000273120406, 10.91162601494192685 ) ) ;
#7870=( BOUNDED_CURVE ( )  B_SPLINE_CURVE ( 2, ( #9534, #6624, #20016, #1629, #20190, #32859, #1983, #27732, #12107, #30633, #4388, #15039, #22579 ),
 .UNSPECIFIED., .F., .T. ) 
 B_SPLINE_CURVE_WITH_KNOTS ( ( 3, 2, 2, 2, 2, 2, 3 ),
 ( 0.5961538461538461453, 0.5974358974358974228, 0.5999999999999999778, 0.6025641025641025328, 0.6051282051282050878, 0.6076923076923076428, 0.6089743589743590313 ),
 .UNSPECIFIED. ) 
 CURVE ( )  GEOMETRIC_REPRESENTATION_ITEM ( )  RATIONAL_B_SPLINE_CURVE ( ( 0.9755282581475768211, 0.9755282581475768211, 1.000000000000000000, 0.9510565162951535312, 1.000000000000000000, 0.9510565162951535312, 1.000000000000000000, 0.9510565162951535312, 1.000000000000000000, 0.9510565162951535312, 1.000000000000000000, 0.9755282581475757109, 0.9755282581475768211 ) ) 
 REPRESENTATION_ITEM ( '' )  );
#7871=ORIENTED_EDGE ( 'NONE', *, *, #9567, .T. ) ;
#7874=EDGE_LOOP ( 'NONE', ( #5423, #14037, #6758, #31965 ) ) ;
#7876=CARTESIAN_POINT ( 'NONE',  ( 7.236395654485760609, 1.024999997268821739, -22.27133577429736633 ) ) ;
#7877=CARTESIAN_POINT ( 'NONE',  ( -33.58253175000000113, 37.27500000273119696, -10.91162601494193218 ) ) ;
#7878=CARTESIAN_POINT ( 'NONE',  ( -26.29305231718579350, 36.30000000546237970, -19.10302069950537884 ) ) ;
#7879=CARTESIAN_POINT ( 'NONE',  ( -20.08610463437157989, 75.69999999999998863, -27.64615127144129758 ) ) ;
#7881=CARTESIAN_POINT ( 'NONE',  ( 27.16883889988624290, 19.92500000273117422, 19.73931689729373673 ) ) ;
#7882=CARTESIAN_POINT ( 'NONE',  ( 3.880418787951150694, 6.198745712990782586, -24.49999999999999645 ) ) ;
#7883=CARTESIAN_POINT ( 'NONE',  ( -33.58253175000000113, 51.47500000273118559, 10.91162601494193929 ) ) ;
#7886=CARTESIAN_POINT ( 'NONE',  ( 26.29305231718579350, 28.79999999999999361, 19.10302069950537529 ) ) ;
#7888=CARTESIAN_POINT ( 'NONE',  ( -20.75514604977248112, 67.42500000273118133, 28.56700777964554661 ) ) ;
#7890=AXIS2_PLACEMENT_3D ( 'NONE', #31624, #8122, #16032 ) ;
#7892=CARTESIAN_POINT ( 'NONE',  ( 10.37757302488624767, 59.97500000273120691, 31.93888565452638417 ) ) ;
#7893=AXIS2_PLACEMENT_3D ( 'NONE', #10517, #18253, #18424 ) ;
#7896=CARTESIAN_POINT ( 'NONE',  ( -1.778240108872766143E-15, 36.00000000546238255, -32.49999999999999289 ) ) ;
#7897=CARTESIAN_POINT ( 'NONE',  ( -20.75514604977248112, 11.42500000273116711, 28.56700777964554661 ) ) ;
#7899=CARTESIAN_POINT ( 'NONE',  ( -33.58253175000000113, 5.475000002731180260, 10.91162601494193929 ) ) ;
#7901=CYLINDRICAL_SURFACE ( 'NONE', #8375, 32.50000000000000000 ) ;
#7910=CARTESIAN_POINT ( 'NONE',  ( 23.41746825000000243, 1.224999997268811480, -7.608796670333727974 ) ) ;
#7911=CARTESIAN_POINT ( 'NONE',  ( -32.50000000000000000, 68.40000000546237402, -10.55989012756945478 ) ) ;
#7919=CYLINDRICAL_SURFACE ( 'NONE', #933, 32.50000000000000000 ) ;
#7920=CARTESIAN_POINT ( 'NONE',  ( 27.16883889988623935, 56.57500000273118701, -19.73931689729374384 ) ) ;
#7921=CARTESIAN_POINT ( 'NONE',  ( 32.50000000000000711, 59.40000000546237402, 10.55989012756945122 ) ) ;
#7923=CARTESIAN_POINT ( 'NONE',  ( -10.37757302488623701, 41.52500000273118275, 31.93888565452638417 ) ) ;
#7924=CARTESIAN_POINT ( 'NONE',  ( 26.29305231718579350, 54.80000000000001847, 19.10302069950537529 ) ) ;
#7925=CARTESIAN_POINT ( 'NONE',  ( 20.75514604977248467, 70.67500000273118133, -28.56700777964554305 ) ) ;
#7929=CARTESIAN_POINT ( 'NONE',  ( 10.04305231718579705, 46.60000000000000142, 30.90933677959248982 ) ) ;
#7931=CARTESIAN_POINT ( 'NONE',  ( -33.58253175000000113, 9.375000002731169957, 0.000000000000000000 ) ) ;
#7932=LINE ( 'NONE', #18420, #8532 ) ;
#7936=LINE ( 'NONE', #26638, #11116 ) ;
#7938=VERTEX_POINT ( 'NONE', #27880 ) ;
#7939=LINE ( 'NONE', #14435, #31018 ) ;
#7951=CARTESIAN_POINT ( 'NONE',  ( 20.75514604977249178, 39.82500000273116569, 28.56700777964553950 ) ) ;
#7955=VERTEX_POINT ( 'NONE', #30609 ) ;
#7957=CARTESIAN_POINT ( 'NONE',  ( -26.29305231718578995, 50.70000000546237828, 19.10302069950538595 ) ) ;
#7959=CARTESIAN_POINT ( 'NONE',  ( -27.16883889988624290, 75.17500000273119554, -19.73931689729374028 ) ) ;
#7960=EDGE_LOOP ( 'NONE', ( #9858, #8046, #27487, #896 ) ) ;
#7965=CARTESIAN_POINT ( 'NONE',  ( 32.50000000000000000, 29.50000000546237899, -3.980102097228898626E-15 ) ) ;
#7966=CARTESIAN_POINT ( 'NONE',  ( 33.58253175000000113, 58.22500000273116427, -10.91162601494193751 ) ) ;
#7968=CARTESIAN_POINT ( 'NONE',  ( -24.50000000000000355, 16.89999999999998437, -7.960532557706207157 ) ) ;
#7969=CARTESIAN_POINT ( 'NONE',  ( -23.41746825000000243, 8.224999997268822582, 7.608796670333725309 ) ) ;
#7970=CARTESIAN_POINT ( 'NONE',  ( 33.58253175000000113, 4.225000002731190030, -10.91162601494193751 ) ) ;
#7972=CARTESIAN_POINT ( 'NONE',  ( 20.08610463437158344, 36.70000000000000284, 27.64615127144129403 ) ) ;
#7974=CARTESIAN_POINT ( 'NONE',  ( 26.29305231718578995, 9.199999999999985079, -19.10302069950538240 ) ) ;
#7978=CARTESIAN_POINT ( 'NONE',  ( -9.270509831248425314, 73.95000000546238539, -12.75976212528059861 ) ) ;
#7980=CARTESIAN_POINT ( 'NONE',  ( 33.58253175000000113, 24.12500000273118417, -4.112674001490185761E-15 ) ) ;
#7983=CARTESIAN_POINT ( 'NONE',  ( 27.16883889988623935, 14.57500000273120833, -19.73931689729374384 ) ) ;
#7986=CARTESIAN_POINT ( 'NONE',  ( -33.58253175000000113, 79.12500000273119838, 0.000000000000000000 ) ) ;
#7988=CARTESIAN_POINT ( 'NONE',  ( 7.570916362186207671, 7.599999999999996092, 23.30088464923126779 ) ) ;
#7989=ADVANCED_FACE ( 'NONE', ( #27706 ), #3856, .T. ) ;
#7991=CARTESIAN_POINT ( 'NONE',  ( -18.94512977948576093, 17.82499999726880446, 13.76444248337722698 ) ) ;
#7992=CARTESIAN_POINT ( 'NONE',  ( -10.37757302488623701, 57.52500000273119696, 31.93888565452638417 ) ) ;
#7995=ORIENTED_EDGE ( 'NONE', *, *, #20351, .F. ) ;
#7997=CARTESIAN_POINT ( 'NONE',  ( 10.37757302488624056, 4.525000002731205839, -31.93888565452638417 ) ) ;
#7999=CARTESIAN_POINT ( 'NONE',  ( 18.94512977948575738, 16.92499999726882010, 13.76444248337723408 ) ) ;
#8008=CARTESIAN_POINT ( 'NONE',  ( 26.29305231718579350, 27.30000000546237260, 19.10302069950537529 ) ) ;
#8010=CARTESIAN_POINT ( 'NONE',  ( 14.47279130897151589, 16.32499999726879736, 19.92008829642072953 ) ) ;
#8011=CARTESIAN_POINT ( 'NONE',  ( 33.58253175000000823, 6.275000002731184523, 10.91162601494192863 ) ) ;
#8012=CARTESIAN_POINT ( 'NONE',  ( 20.08610463437158344, 60.70000000000000284, 27.64615127144129403 ) ) ;
#8013=CARTESIAN_POINT ( 'NONE',  ( -4.300734207923759378, 78.47500000273119269, -13.23629886949340495 ) ) ;
#8014=CARTESIAN_POINT ( 'NONE',  ( 10.04305231718579705, 73.10000000546237686, 30.90933677959248982 ) ) ;
#8016=CARTESIAN_POINT ( 'NONE',  ( -13.91746824999999532, 73.47500000273117848, 4.522059556121122093 ) ) ;
#8019=CARTESIAN_POINT ( 'NONE',  ( -15.14183272437242778, 13.29999999999998650, 20.84094480462497856 ) ) ;
#8020=CARTESIAN_POINT ( 'NONE',  ( -26.29305231718579350, 3.799999999999998046, -19.10302069950537884 ) ) ;
#8023=CARTESIAN_POINT ( 'NONE',  ( 33.58253175000000823, 52.02500000273118985, 10.91162601494192863 ) ) ;
#8026=CARTESIAN_POINT ( 'NONE',  ( 27.16883889988624290, 32.17500000273118843, 19.73931689729373673 ) ) ;
#8027=CARTESIAN_POINT ( 'NONE',  ( 5.147494310547434893, 24.55125428154685707, 32.49999999999999289 ) ) ;
#8028=LINE ( 'NONE', #31363, #13921 ) ;
#8029=CARTESIAN_POINT ( 'NONE',  ( 10.04305231718578817, 15.90000000546237757, -30.90933677959249337 ) ) ;
#8030=CARTESIAN_POINT ( 'NONE',  ( -10.04305231718578462, 22.90000000546238468, 30.90933677959249337 ) ) ;
#8033=CARTESIAN_POINT ( 'NONE',  ( 23.41746824999999887, 0.7249999972688272454, -7.608796670333727974 ) ) ;
#8037=EDGE_CURVE ( 'NONE', #23284, #15393, #27510, .T. ) ;
#8038=CARTESIAN_POINT ( 'NONE',  ( -27.16883889988623935, 23.32500000273118701, 19.73931689729374739 ) ) ;
#8046=ORIENTED_EDGE ( 'NONE', *, *, #7796, .T. ) ;
#8047=CYLINDRICAL_SURFACE ( 'NONE', #5338, 32.50000000000000000 ) ;
#8048=AXIS2_PLACEMENT_3D ( 'NONE', #2875, #10428, #15413 ) ;
#8049=CARTESIAN_POINT ( 'NONE',  ( 27.16883889988624290, 32.17500000273118843, 19.73931689729373673 ) ) ;
#8050=CARTESIAN_POINT ( 'NONE',  ( 32.50000000000000000, 35.50000000546238255, -3.980102097228898626E-15 ) ) ;
#8052=DIRECTION ( 'NONE',  ( 0.000000000000000000, 1.000000000000000000, 0.000000000000000000 ) ) ;
#8053=CARTESIAN_POINT ( 'NONE',  ( 32.50000000000000000, 77.00000000000001421, -3.980102097228898626E-15 ) ) ;
#8054=CARTESIAN_POINT ( 'NONE',  ( -33.58253175000000113, 47.27500000273116143, -10.91162601494193218 ) ) ;
#8057=CARTESIAN_POINT ( 'NONE',  ( -10.04305231718579172, 21.60000000000000853, -30.90933677959248982 ) ) ;
#8059=CARTESIAN_POINT ( 'NONE',  ( -27.16883889988624290, 66.92500000273119554, -19.73931689729374028 ) ) ;
#8062=CARTESIAN_POINT ( 'NONE',  ( -33.58253175000000113, 55.27500000273121117, -10.91162601494193041 ) ) ;
#8064=CARTESIAN_POINT ( 'NONE',  ( 6.486482029760649416E-15, 9.625000002731196602, 35.31076352940723240 ) ) ;
#8067=CARTESIAN_POINT ( 'NONE',  ( -10.37757302488624411, 4.975000002731183812, -31.93888565452638417 ) ) ;
#8069=CARTESIAN_POINT ( 'NONE',  ( 32.50000000000000711, 45.40000000546237402, 10.55989012756945122 ) ) ;
#8076=CARTESIAN_POINT ( 'NONE',  ( 26.29305231718579350, 60.79999999999999005, 19.10302069950537529 ) ) ;
#8078=CARTESIAN_POINT ( 'NONE',  ( -23.41746824999999887, 8.124999997268817609, -2.867812753649727150E-15 ) ) ;
#8080=CARTESIAN_POINT ( 'NONE',  ( 10.04305231718579705, 67.10000000546237686, 30.90933677959248982 ) ) ;
#8088=CARTESIAN_POINT ( 'NONE',  ( -32.50000000000000000, 36.00000000000000711, 0.000000000000000000 ) ) ;
#8089=CARTESIAN_POINT ( 'NONE',  ( 20.75514604977248467, 52.67500000273116711, -28.56700777964554305 ) ) ;
#8090=CARTESIAN_POINT ( 'NONE',  ( -32.50000000000000000, 58.40000000546237402, -10.55989012756945478 ) ) ;
#8092=CARTESIAN_POINT ( 'NONE',  ( -33.58253175000000113, 39.22500000273119269, 10.91162601494193929 ) ) ;
#8093=CARTESIAN_POINT ( 'NONE',  ( 0.000000000000000000, 80.00000000000001421, 0.000000000000000000 ) ) ;
#8094=CARTESIAN_POINT ( 'NONE',  ( 27.16883889988624290, 68.17500000273119554, 19.73931689729373673 ) ) ;
#8098=CARTESIAN_POINT ( 'NONE',  ( -10.04305231718579172, 47.60000000000000142, -30.90933677959248982 ) ) ;
#8100=CARTESIAN_POINT ( 'NONE',  ( -10.37757302488624411, 8.975000002731187365, -31.93888565452638417 ) ) ;
#8101=CARTESIAN_POINT ( 'NONE',  ( 20.08610463437158344, 35.20000000546238539, 27.64615127144129403 ) ) ;
#8103=CARTESIAN_POINT ( 'NONE',  ( -13.91746824999999532, 71.47500000273119269, 4.522059556121122093 ) ) ;
#8104=CARTESIAN_POINT ( 'NONE',  ( 33.58253175000000113, 78.37500000273116996, -4.112674001490185761E-15 ) ) ;
#8108=CYLINDRICAL_SURFACE ( 'NONE', #23366, 15.00000000000000000 ) ;
#8117=EDGE_CURVE ( 'NONE', #21143, #33174, #11578, .T. ) ;
#8118=CARTESIAN_POINT ( 'NONE',  ( -20.08610463437156923, 56.80000000546240102, 27.64615127144130113 ) ) ;
#8119=CARTESIAN_POINT ( 'NONE',  ( 10.37757302488624767, 41.72500000273118559, 31.93888565452638417 ) ) ;
#8122=DIRECTION ( 'NONE',  ( -0.000000000000000000, -1.000000000000000000, -0.000000000000000000 ) ) ;
#8125=CARTESIAN_POINT ( 'NONE',  ( -32.50000000000000000, 50.40000000546236691, -10.55989012756945300 ) ) ;
#8127=CARTESIAN_POINT ( 'NONE',  ( 10.37757302488624767, 69.97500000273119269, 31.93888565452638417 ) ) ;
#8128=ORIENTED_EDGE ( 'NONE', *, *, #17702, .F. ) ;
#8132=ORIENTED_EDGE ( 'NONE', *, *, #5517, .F. ) ;
#8133=CARTESIAN_POINT ( 'NONE',  ( -20.08610463437157989, 48.20000000546237118, -27.64615127144129758 ) ) ;
#8134=CARTESIAN_POINT ( 'NONE',  ( 6.486482029760649416E-15, 63.62500000273117706, 35.31076352940723240 ) ) ;
#8136=CARTESIAN_POINT ( 'NONE',  ( -26.29305231718578995, 66.70000000546238539, 19.10302069950538595 ) ) ;
#8137=CARTESIAN_POINT ( 'NONE',  ( -23.41746824999999887, 10.12499999726881938, -2.867812753649727150E-15 ) ) ;
#8138=CARTESIAN_POINT ( 'NONE',  ( -33.58253175000000113, 5.025000002731194293, -10.91162601494193218 ) ) ;
#8139=CARTESIAN_POINT ( 'NONE',  ( 33.58253175000000823, 28.27500000273118985, 10.91162601494192863 ) ) ;
#8142=CARTESIAN_POINT ( 'NONE',  ( 8.891200544363830713E-16, 79.75000000546236834, -15.00000000000000000 ) ) ;
#8143=CARTESIAN_POINT ( 'NONE',  ( -1.778240108872766143E-15, 31.49999999999998579, -32.49999999999999289 ) ) ;
#8148=CARTESIAN_POINT ( 'NONE',  ( -13.91746824999999887, 78.87500000273118417, 0.000000000000000000 ) ) ;
#8150=CARTESIAN_POINT ( 'NONE',  ( 33.58253175000000823, 22.02500000273117919, 10.91162601494192863 ) ) ;
#8153=CARTESIAN_POINT ( 'NONE',  ( 33.58253175000000113, 16.37500000273117706, -4.112674001490185761E-15 ) ) ;
#8155=CARTESIAN_POINT ( 'NONE',  ( 33.58253175000000113, 68.22500000273116427, -10.91162601494193574 ) ) ;
#8158=CARTESIAN_POINT ( 'NONE',  ( -27.16883889988623935, 57.32500000273119412, 19.73931689729374739 ) ) ;
#8162=CARTESIAN_POINT ( 'NONE',  ( -27.16883889988623935, 1.325000002731169246, 19.73931689729374739 ) ) ;
#8163=CARTESIAN_POINT ( 'NONE',  ( 14.47279130897151589, 2.324999997268805796, 19.92008829642072953 ) ) ;
#8165=ORIENTED_EDGE ( 'NONE', *, *, #21677, .T. ) ;
#8167=CARTESIAN_POINT ( 'NONE',  ( -5.147494310547423346, 42.94874572391552192, 32.50000000000000000 ) ) ;
#8168=ORIENTED_EDGE ( 'NONE', *, *, #16781, .F. ) ;
#8171=CARTESIAN_POINT ( 'NONE',  ( 27.16883889988623935, 78.32500000273118701, -19.73931689729374384 ) ) ;
#8173=CARTESIAN_POINT ( 'NONE',  ( -14.47279130897151589, 15.32499999726880269, -19.92008829642072598 ) ) ;
#8174=CARTESIAN_POINT ( 'NONE',  ( 27.16883889988623935, 10.57500000273120477, -19.73931689729374384 ) ) ;
#8175=EDGE_CURVE ( 'NONE', #3689, #3647, #9327, .T. ) ;
#8176=CARTESIAN_POINT ( 'NONE',  ( -10.04305231718579172, 59.59999999999998721, -30.90933677959248982 ) ) ;
#8177=CARTESIAN_POINT ( 'NONE',  ( 13.91746824999999887, 75.87500000273116996, -1.704398294459741270E-15 ) ) ;
#8178=CARTESIAN_POINT ( 'NONE',  ( 19.82091636218621034, 1.799999999999996048, 14.40073868116559730 ) ) ;
#8180=CARTESIAN_POINT ( 'NONE',  ( -11.25946833292375793, 75.17500000273119554, -8.180482586598733619 ) ) ;
#8182=EDGE_CURVE ( 'NONE', #21850, #1559, #11088, .T. ) ;
#8184=CARTESIAN_POINT ( 'NONE',  ( 24.50000000000000000, 16.00000000000001421, 0.000000000000000000 ) ) ;
#8185=CARTESIAN_POINT ( 'NONE',  ( 10.04305231718578817, 3.400000000000014122, -30.90933677959249337 ) ) ;
#8186=CARTESIAN_POINT ( 'NONE',  ( 32.50000000000000711, 17.40000000546238823, 10.55989012756945122 ) ) ;
#8188=CARTESIAN_POINT ( 'NONE',  ( 33.58253175000000113, 44.12500000273117706, -4.112674001490185761E-15 ) ) ;
#8191=CARTESIAN_POINT ( 'NONE',  ( 10.37757302488624056, 34.77500000273120406, -31.93888565452638417 ) ) ;
#8198=CARTESIAN_POINT ( 'NONE',  ( 1.507698388325705758E-15, 5.124999997268805174, -24.62258325217400312 ) ) ;
#8199=CARTESIAN_POINT ( 'NONE',  ( -5.147494310547423346, 40.44874571845314648, 32.50000000000000000 ) ) ;
#8202=CARTESIAN_POINT ( 'NONE',  ( -20.08610463437156923, 12.29999999999999183, 27.64615127144130113 ) ) ;
#8203=CARTESIAN_POINT ( 'NONE',  ( -20.75514604977248112, 19.42500000273117777, 28.56700777964554661 ) ) ;
#8205=ORIENTED_EDGE ( 'NONE', *, *, #31314, .F. ) ;
#8211=VERTEX_POINT ( 'NONE', #11916 ) ;
#8212=CARTESIAN_POINT ( 'NONE',  ( -33.58253175000000113, 27.27500000273119340, -10.91162601494193218 ) ) ;
#8213=CARTESIAN_POINT ( 'NONE',  ( 10.04305231718578817, 39.90000000546237402, -30.90933677959249337 ) ) ;
#8215=CARTESIAN_POINT ( 'NONE',  ( -26.29305231718578995, 78.19999999999998863, 19.10302069950538595 ) ) ;
#8217=CARTESIAN_POINT ( 'NONE',  ( -10.37757302488623701, 39.77500000273118275, 31.93888565452638417 ) ) ;
#8219=CARTESIAN_POINT ( 'NONE',  ( -20.08610463437156923, 20.30000000000000071, 27.64615127144130113 ) ) ;
#8221=CARTESIAN_POINT ( 'NONE',  ( -10.37757302488624411, 64.72500000273117848, -31.93888565452638417 ) ) ;
#8223=CARTESIAN_POINT ( 'NONE',  ( -5.147494310547418017, 76.05125428700922896, -32.50000000000000000 ) ) ;
#8224=CARTESIAN_POINT ( 'NONE',  ( -2.162160676586882350E-15, 52.87500000273119838, -35.31076352940722529 ) ) ;
#8227=CARTESIAN_POINT ( 'NONE',  ( -20.75514604977248112, 13.42500000273119198, 28.56700777964554661 ) ) ;
#8232=CARTESIAN_POINT ( 'NONE',  ( -5.147494310547430452, 18.05125428700922541, -32.49999999999999289 ) ) ;
#8238=CARTESIAN_POINT ( 'NONE',  ( -8.446640517145639571E-15, 77.00000000546236834, 32.49999999999999289 ) ) ;
#8240=CARTESIAN_POINT ( 'NONE',  ( 32.50000000000000711, 71.40000000546241665, 10.55989012756945122 ) ) ;
#8244=ORIENTED_EDGE ( 'NONE', *, *, #12201, .T. ) ;
#8249=CARTESIAN_POINT ( 'NONE',  ( 27.16883889988623935, 50.57500000273118701, -19.73931689729374384 ) ) ;
#8250=CARTESIAN_POINT ( 'NONE',  ( 20.08610463437157279, 59.80000000546235839, -27.64615127144129758 ) ) ;
#8252=CARTESIAN_POINT ( 'NONE',  ( -20.75514604977248823, 38.82500000273120122, -28.56700777964554305 ) ) ;
#8253=CARTESIAN_POINT ( 'NONE',  ( 2.375766604868046361, 72.80125428700920054, 14.99999999999999822 ) ) ;
#8254=CARTESIAN_POINT ( 'NONE',  ( -33.58253175000000113, 59.37500000273118417, 0.000000000000000000 ) ) ;
#8256=CARTESIAN_POINT ( 'NONE',  ( 32.50000000000000000, 1.500000005462381880, -3.980102097228898626E-15 ) ) ;
#8259=CARTESIAN_POINT ( 'NONE',  ( 20.08610463437158344, 42.69999999999998863, 27.64615127144129403 ) ) ;
#8261=CARTESIAN_POINT ( 'NONE',  ( 6.486482029760649416E-15, 13.87500000273117529, 35.31076352940723240 ) ) ;
#8262=CARTESIAN_POINT ( 'NONE',  ( -2.165007332552593587E-13, 51.00000000546238255, 32.50000000000000000 ) ) ;
#8263=CARTESIAN_POINT ( 'NONE',  ( 8.601468415847520532, 74.07500000273120122, 11.83890561707634781 ) ) ;
#8264=CARTESIAN_POINT ( 'NONE',  ( -27.16883889988624290, 75.17500000273119554, -19.73931689729374028 ) ) ;
#8265=CARTESIAN_POINT ( 'NONE',  ( -26.29305231718579350, 21.79999999999998650, -19.10302069950537884 ) ) ;
#8278=CARTESIAN_POINT ( 'NONE',  ( 33.58253175000000113, 36.22500000273119980, -10.91162601494193574 ) ) ;
#8288=CARTESIAN_POINT ( 'NONE',  ( 33.58253175000000113, 72.47500000273119269, -10.91162601494193751 ) ) ;
#8294=CARTESIAN_POINT ( 'NONE',  ( 27.16883889988624290, 51.92500000273120264, 19.73931689729373673 ) ) ;
#8296=CARTESIAN_POINT ( 'NONE',  ( -20.08610463437157989, 18.20000000546239605, -27.64615127144129758 ) ) ;
#8298=CARTESIAN_POINT ( 'NONE',  ( 23.41746824999999887, 7.124999997268815832, 0.000000000000000000 ) ) ;
#8299=CARTESIAN_POINT ( 'NONE',  ( -20.75514604977248112, 31.67500000273119909, 28.56700777964554661 ) ) ;
#8303=CARTESIAN_POINT ( 'NONE',  ( -20.08610463437157989, 3.699999999999999289, -27.64615127144129758 ) ) ;
#8308=CARTESIAN_POINT ( 'NONE',  ( -11.25946833292375793, 72.67500000273119554, -8.180482586598733619 ) ) ;
#8310=CARTESIAN_POINT ( 'NONE',  ( 20.75514604977249178, 23.82500000273118701, 28.56700777964553950 ) ) ;
#8314=CARTESIAN_POINT ( 'NONE',  ( 6.486482029760648627E-15, 15.87500000273120015, 35.31076352940722529 ) ) ;
#8317=CARTESIAN_POINT ( 'NONE',  ( 33.58253175000000113, 68.12500000273119838, -4.112674001490185761E-15 ) ) ;
#8319=CARTESIAN_POINT ( 'NONE',  ( 26.29305231718579350, 3.300000005462377928, 19.10302069950537529 ) ) ;
#8322=CARTESIAN_POINT ( 'NONE',  ( -33.58253175000000113, 57.12500000273118417, 0.000000000000000000 ) ) ;
#8327=CARTESIAN_POINT ( 'NONE',  ( -20.75514604977248112, 3.425000002731186655, 28.56700777964554661 ) ) ;
#8328=CARTESIAN_POINT ( 'NONE',  ( 23.41746824999999887, 8.624999997268817609, 0.000000000000000000 ) ) ;
#8332=CARTESIAN_POINT ( 'NONE',  ( -20.08610463437157989, 68.20000000546239960, -27.64615127144129758 ) ) ;
#8333=ORIENTED_EDGE ( 'NONE', *, *, #14071, .T. ) ;
#8335=CARTESIAN_POINT ( 'NONE',  ( 26.29305231718579350, 4.799999999999998934, 19.10302069950537529 ) ) ;
#8337=LINE ( 'NONE', #26540, #3049 ) ;
#8339=CARTESIAN_POINT ( 'NONE',  ( -24.50000000000000355, 2.899999999999995470, -7.960532557706207157 ) ) ;
#8340=CARTESIAN_POINT ( 'NONE',  ( -33.58253175000000113, 7.475000002731175819, 10.91162601494193929 ) ) ;
#8341=CARTESIAN_POINT ( 'NONE',  ( -20.08610463437157989, 59.70000000000000284, -27.64615127144129758 ) ) ;
#8342=CARTESIAN_POINT ( 'NONE',  ( 32.50000000000000000, 57.60000000546236976, -10.55989012756945833 ) ) ;
#8343=CARTESIAN_POINT ( 'NONE',  ( 3.245314017740486554E-15, 0.000000000000000000, -26.50000000000000355 ) ) ;
#8345=CARTESIAN_POINT ( 'NONE',  ( 13.91746825000000065, 74.27500000273117564, 4.522059556121114987 ) ) ;
#8348=CARTESIAN_POINT ( 'NONE',  ( -32.50000000000000000, 38.40000000546235981, -10.55989012756945300 ) ) ;
#8350=CARTESIAN_POINT ( 'NONE',  ( 33.58253175000000823, 46.02500000273118275, 10.91162601494192863 ) ) ;
#8354=CARTESIAN_POINT ( 'NONE',  ( -20.75514604977248823, 35.07500000273120833, -28.56700777964554305 ) ) ;
#8356=AXIS2_PLACEMENT_3D ( 'NONE', #5535, #10182, #21332 ) ;
#8359=CARTESIAN_POINT ( 'NONE',  ( 32.50000000000000000, 31.10000000000000497, -10.55989012756945833 ) ) ;
#8362=CARTESIAN_POINT ( 'NONE',  ( 14.47279130897151944, 2.924999997268816099, -19.92008829642072598 ) ) ;
#8365=ADVANCED_FACE ( 'NONE', ( #12044 ), #15794, .T. ) ;
#8367=CARTESIAN_POINT ( 'NONE',  ( -10.04305231718578462, 60.40000000000000568, 30.90933677959249337 ) ) ;
#8368=CARTESIAN_POINT ( 'NONE',  ( -27.16883889988623935, 19.32500000273118701, 19.73931689729374739 ) ) ;
#8375=AXIS2_PLACEMENT_3D ( 'NONE', #2754, #9970, #13219 ) ;
#8377=VECTOR ( 'NONE', #1999, 1000.000000000000000 ) ;
#8378=ORIENTED_EDGE ( 'NONE', *, *, #29484, .T. ) ;
#8380=CARTESIAN_POINT ( 'NONE',  ( -33.58253175000000113, 25.27500000273119696, -10.91162601494193218 ) ) ;
#8381=CARTESIAN_POINT ( 'NONE',  ( 26.29305231718579350, 29.30000000546237260, 19.10302069950537529 ) ) ;
#8383=CARTESIAN_POINT ( 'NONE',  ( 10.04305231718579705, 52.60000000000000853, 30.90933677959248982 ) ) ;
#8384=CARTESIAN_POINT ( 'NONE',  ( -15.14183272437242067, 10.70000000000001172, -20.84094480462497856 ) ) ;
#8385=CARTESIAN_POINT ( 'NONE',  ( 6.486482029760649416E-15, 41.87500000273119127, 35.31076352940723240 ) ) ;
#8387=CARTESIAN_POINT ( 'NONE',  ( 26.29305231718579350, 20.79999999999998650, 19.10302069950537529 ) ) ;
#8389=CARTESIAN_POINT ( 'NONE',  ( 10.37757302488624767, 65.72500000273117848, 31.93888565452638417 ) ) ;
#8392=CARTESIAN_POINT ( 'NONE',  ( -27.16883889988624290, 55.17500000273118133, -19.73931689729374028 ) ) ;
#8394=CARTESIAN_POINT ( 'NONE',  ( 20.75514604977249178, 7.825000002731194115, 28.56700777964553950 ) ) ;
#8400=DIRECTION ( 'NONE',  ( -0.000000000000000000, -1.000000000000000000, -0.000000000000000000 ) ) ;
#8405=CARTESIAN_POINT ( 'NONE',  ( -1.778240108872766143E-15, 49.50000000000000000, -32.49999999999999289 ) ) ;
#8406=SURFACE_STYLE_USAGE ( .BOTH. , #22136 ) ;
#8408=EDGE_CURVE ( 'NONE', #30686, #17243, #26222, .T. ) ;
#8409=CARTESIAN_POINT ( 'NONE',  ( 20.08610463437157279, 69.80000000546240813, -27.64615127144129758 ) ) ;
#8416=LINE ( 'NONE', #6015, #31105 ) ;
#8417=CARTESIAN_POINT ( 'NONE',  ( 10.37757302488624767, 45.97500000273119269, 31.93888565452638417 ) ) ;
#8418=CARTESIAN_POINT ( 'NONE',  ( 26.29305231718578995, 55.70000000546237828, -19.10302069950538240 ) ) ;
#8419=LINE ( 'NONE', #13419, #28666 ) ;
#8420=CARTESIAN_POINT ( 'NONE',  ( 20.75514604977248467, 34.42500000273117422, -28.56700777964554305 ) ) ;
#8422=CARTESIAN_POINT ( 'NONE',  ( -27.16883889988624290, 63.17500000273118843, -19.73931689729374028 ) ) ;
#8423=CARTESIAN_POINT ( 'NONE',  ( -20.08610463437156923, 0.8000000054623617185, 27.64615127144130113 ) ) ;
#8427=CARTESIAN_POINT ( 'NONE',  ( -2.092463501923844636E-15, 39.50000000000000000, -34.17252228774368916 ) ) ;
#8429=CARTESIAN_POINT ( 'NONE',  ( -10.37757302488624411, 2.975000002731182036, -31.93888565452638417 ) ) ;
#8430=CARTESIAN_POINT ( 'NONE',  ( 19.82091636218621034, 19.54999999453763238, 14.40073868116559730 ) ) ;
#8431=CARTESIAN_POINT ( 'NONE',  ( -11.25946833292375793, 75.17500000273119554, -8.180482586598733619 ) ) ;
#8432=CARTESIAN_POINT ( 'NONE',  ( 20.75514604977248467, 70.67500000273119554, -28.56700777964554305 ) ) ;
#8433=CYLINDRICAL_SURFACE ( 'NONE', #6711, 32.50000000000000000 ) ;
#8435=VERTEX_POINT ( 'NONE', #17379 ) ;
#8436=CARTESIAN_POINT ( 'NONE',  ( 0.000000000000000000, 80.00000000000001421, 0.000000000000000000 ) ) ;
#8438=CARTESIAN_POINT ( 'NONE',  ( -8.891200544363830713E-16, 75.50000000000001421, -15.00000000000000000 ) ) ;
#8447=VECTOR ( 'NONE', #23654, 1000.000000000000114 ) ;
#8448=CARTESIAN_POINT ( 'NONE',  ( -10.37757302488623701, 39.52500000273118275, 31.93888565452638417 ) ) ;
#8451=EDGE_CURVE ( 'NONE', #14454, #7660, #31021, .T. ) ;
#8454=ORIENTED_EDGE ( 'NONE', *, *, #18889, .T. ) ;
#8456=CARTESIAN_POINT ( 'NONE',  ( -20.08610463437157989, 50.20000000546237118, -27.64615127144129758 ) ) ;
#8458=CARTESIAN_POINT ( 'NONE',  ( -2.162160676586881955E-15, 68.87500000273118417, -35.31076352940723240 ) ) ;
#8459=ORIENTED_EDGE ( 'NONE', *, *, #12464, .T. ) ;
#8462=ORIENTED_EDGE ( 'NONE', *, *, #10902, .T. ) ;
#8464=CARTESIAN_POINT ( 'NONE',  ( -33.58253175000000113, 57.12500000273118417, 0.000000000000000000 ) ) ;
#8466=( BOUNDED_CURVE ( )  B_SPLINE_CURVE ( 2, ( #1671, #22619, #17145, #33072, #11980, #9578, #2024, #7342, #22448, #15077, #7001, #1845, #14396 ),
 .UNSPECIFIED., .F., .T. ) 
 B_SPLINE_CURVE_WITH_KNOTS ( ( 3, 2, 2, 2, 2, 2, 3 ),
 ( 0.3782051282051281937, 0.3794871794871794712, 0.3820512820512820262, 0.3846153846153846367, 0.3871794871794871917, 0.3897435897435897467, 0.3910256410256410242 ),
 .UNSPECIFIED. ) 
 CURVE ( )  GEOMETRIC_REPRESENTATION_ITEM ( )  RATIONAL_B_SPLINE_CURVE ( ( 0.9755282581475768211, 0.9755282581475768211, 1.000000000000000000, 0.9510565162951535312, 1.000000000000000000, 0.9510565162951535312, 1.000000000000000000, 0.9510565162951535312, 1.000000000000000000, 0.9510565162951535312, 1.000000000000000000, 0.9755282581475768211, 0.9755282581475768211 ) ) 
 REPRESENTATION_ITEM ( '' )  );
#8467=CARTESIAN_POINT ( 'NONE',  ( -26.29305231718578995, 20.70000000546237828, 19.10302069950538595 ) ) ;
#8468=FACE_OUTER_BOUND ( 'NONE', #9635, .T. ) ;
#8469=CARTESIAN_POINT ( 'NONE',  ( -7.236395654485763274, 8.524999997268800200, 22.27133577429736633 ) ) ;
#8473=CARTESIAN_POINT ( 'NONE',  ( 20.75514604977248467, 24.67500000273118843, -28.56700777964554305 ) ) ;
#8475=CARTESIAN_POINT ( 'NONE',  ( 8.601468415847520532, 79.57500000273120122, 11.83890561707634781 ) ) ;
#8476=CARTESIAN_POINT ( 'NONE',  ( -10.04305231718578462, 28.90000000546238823, 30.90933677959249337 ) ) ;
#8478=ORIENTED_EDGE ( 'NONE', *, *, #9780, .T. ) ;
#8480=CARTESIAN_POINT ( 'NONE',  ( -4.300734207923755825, 75.27500000273118985, 13.23629886949340673 ) ) ;
#8482=CARTESIAN_POINT ( 'NONE',  ( -20.75514604977248112, 27.42500000273118488, 28.56700777964554661 ) ) ;
#8485=CARTESIAN_POINT ( 'NONE',  ( 10.37757302488624767, 15.97500000273119269, 31.93888565452638417 ) ) ;
#8487=CARTESIAN_POINT ( 'NONE',  ( -33.58253175000000113, 69.22500000273116427, 10.91162601494193929 ) ) ;
#8489=CARTESIAN_POINT ( 'NONE',  ( -4.300734207923759378, 78.97500000273119269, -13.23629886949340495 ) ) ;
#8492=CARTESIAN_POINT ( 'NONE',  ( -33.58253175000000113, 59.12500000273118417, 0.000000000000000000 ) ) ;
#8497=CARTESIAN_POINT ( 'NONE',  ( -7.236395654485763274, 4.024999997268824181, 22.27133577429736633 ) ) ;
#8499=ORIENTED_EDGE ( 'NONE', *, *, #3387, .T. ) ;
#8505=CARTESIAN_POINT ( 'NONE',  ( -4.223320258572819786E-15, 3.500000000000004441, 24.50000000000000000 ) ) ;
#8506=CARTESIAN_POINT ( 'NONE',  ( 10.37757302488624767, 71.72500000273119269, 31.93888565452638417 ) ) ;
#8508=EDGE_CURVE ( 'NONE', #2126, #33755, #9935, .T. ) ;
#8509=CARTESIAN_POINT ( 'NONE',  ( -15.14183272437241889, 8.699999999999986855, -20.84094480462497856 ) ) ;
#8510=CARTESIAN_POINT ( 'NONE',  ( 20.75514604977249178, 10.07500000273118168, 28.56700777964553950 ) ) ;
#8511=CARTESIAN_POINT ( 'NONE',  ( -20.75514604977248112, 15.42500000273118843, 28.56700777964554661 ) ) ;
#8513=CARTESIAN_POINT ( 'NONE',  ( 8.601468415847516980, 80.17500000273116711, -11.83890561707634603 ) ) ;
#8516=CARTESIAN_POINT ( 'NONE',  ( 4.300734207923761154, 75.97500000273119269, 13.23629886949340495 ) ) ;
#8518=EDGE_CURVE ( 'NONE', #20335, #31666, #18538, .T. ) ;
#8519=CARTESIAN_POINT ( 'NONE',  ( -24.50000000000000000, 8.749999994537628112, -3.000384657911015469E-15 ) ) ;
#8520=VECTOR ( 'NONE', #15225, 1000.000000000000000 ) ;
#8521=CARTESIAN_POINT ( 'NONE',  ( 26.29305231718578995, 49.70000000546237118, -19.10302069950538240 ) ) ;
#8523=CARTESIAN_POINT ( 'NONE',  ( -10.37757302488623701, 45.52500000273118985, 31.93888565452638417 ) ) ;
#8526=CARTESIAN_POINT ( 'NONE',  ( 33.58253175000000823, 36.27500000273119696, 10.91162601494192685 ) ) ;
#8530=CARTESIAN_POINT ( 'NONE',  ( -20.08610463437157989, 44.20000000546238539, -27.64615127144129758 ) ) ;
#8532=VECTOR ( 'NONE', #21161, 1000.000000000000000 ) ;
#8534=CARTESIAN_POINT ( 'NONE',  ( 23.41746824999999887, 2.724999997268822138, -7.608796670333727974 ) ) ;
#8536=CARTESIAN_POINT ( 'NONE',  ( -5.147494310547423346, 52.94874572391552903, 32.50000000000000000 ) ) ;
#8538=CARTESIAN_POINT ( 'NONE',  ( -5.147494310547430452, 59.55125428154684641, -32.49999999999999289 ) ) ;
#8540=CARTESIAN_POINT ( 'NONE',  ( 33.58253175000000823, 20.02500000273118275, 10.91162601494192685 ) ) ;
#8544=VERTEX_POINT ( 'NONE', #29638 ) ;
#8549=ORIENTED_EDGE ( 'NONE', *, *, #1168, .T. ) ;
#8550=CARTESIAN_POINT ( 'NONE',  ( -7.236395654485763274, 2.024999997268822405, 22.27133577429736633 ) ) ;
#8551=CARTESIAN_POINT ( 'NONE',  ( 33.58253175000000113, 30.37500000273119127, -4.112674001490185761E-15 ) ) ;
#8552=CARTESIAN_POINT ( 'NONE',  ( -10.04305231718578462, 28.90000000546238823, 30.90933677959249337 ) ) ;
#8553=AXIS2_PLACEMENT_3D ( 'NONE', #10350, #20828, #4851 ) ;
#8554=CARTESIAN_POINT ( 'NONE',  ( 26.29305231718579350, 76.80000000000001137, 19.10302069950537529 ) ) ;
#8555=CARTESIAN_POINT ( 'NONE',  ( -10.04305231718579172, 54.10000000546239107, -30.90933677959248982 ) ) ;
#8556=CARTESIAN_POINT ( 'NONE',  ( 26.29305231718578995, 37.70000000546236407, -19.10302069950538240 ) ) ;
#8557=CARTESIAN_POINT ( 'NONE',  ( -27.16883889988623935, 41.57500000273117990, 19.73931689729374739 ) ) ;
#8560=CARTESIAN_POINT ( 'NONE',  ( -26.29305231718578995, 22.19999999999999574, 19.10302069950538595 ) ) ;
#8562=CARTESIAN_POINT ( 'NONE',  ( -33.58253175000000113, 65.22500000273117848, 10.91162601494193929 ) ) ;
#8563=CARTESIAN_POINT ( 'NONE',  ( -33.58253175000000113, 51.37500000273120548, 0.000000000000000000 ) ) ;
#8565=DIRECTION ( 'NONE',  ( -0.000000000000000000, -1.000000000000000000, -0.000000000000000000 ) ) ;
#8566=CARTESIAN_POINT ( 'NONE',  ( -2.162160676586881955E-15, 2.625000002731183724, -35.31076352940723240 ) ) ;
#8570=CARTESIAN_POINT ( 'NONE',  ( 0.000000000000000000, 80.00000000000001421, 0.000000000000000000 ) ) ;
#8574=CARTESIAN_POINT ( 'NONE',  ( -10.04305231718578462, 58.90000000546238823, 30.90933677959249337 ) ) ;
#8578=CARTESIAN_POINT ( 'NONE',  ( 24.50000000000000000, 0.000000000000000000, 0.000000000000000000 ) ) ;
#8583=VERTEX_POINT ( 'NONE', #16295 ) ;
#8588=CARTESIAN_POINT ( 'NONE',  ( -20.75514604977248112, 49.67500000273118133, 28.56700777964554661 ) ) ;
#8589=CARTESIAN_POINT ( 'NONE',  ( -10.04305231718578462, 52.90000000546238113, 30.90933677959249337 ) ) ;
#8591=CARTESIAN_POINT ( 'NONE',  ( -20.75514604977248823, 34.82500000273118701, -28.56700777964554305 ) ) ;
#8593=CARTESIAN_POINT ( 'NONE',  ( -27.16883889988624290, 65.17500000273118133, -19.73931689729374028 ) ) ;
#8595=CARTESIAN_POINT ( 'NONE',  ( -26.29305231718578995, 42.20000000000001705, 19.10302069950538595 ) ) ;
#8598=CARTESIAN_POINT ( 'NONE',  ( -27.16883889988623935, 1.575000002731197224, 19.73931689729374739 ) ) ;
#8599=DIRECTION ( 'NONE',  ( -0.000000000000000000, -1.000000000000000000, -0.000000000000000000 ) ) ;
#8600=CARTESIAN_POINT ( 'NONE',  ( -8.601468415847518756, 75.07500000273118701, -11.83890561707634781 ) ) ;
#8601=CARTESIAN_POINT ( 'NONE',  ( 10.37757302488624767, 75.97500000273119269, 31.93888565452638417 ) ) ;
#8603=EDGE_CURVE ( 'NONE', #22348, #33045, #5167, .T. ) ;
#8609=CARTESIAN_POINT ( 'NONE',  ( 4.635254915624209993, 75.40000000000001990, -14.26584774442730463 ) ) ;
#8621=CARTESIAN_POINT ( 'NONE',  ( 20.08610463437158344, 13.20000000546237651, 27.64615127144129403 ) ) ;
#8622=ORIENTED_EDGE ( 'NONE', *, *, #132, .F. ) ;
#8624=CARTESIAN_POINT ( 'NONE',  ( 20.08610463437157279, 51.29999999999997584, -27.64615127144129758 ) ) ;
#8626=CARTESIAN_POINT ( 'NONE',  ( -33.58253175000000113, 67.27500000273117564, -10.91162601494193218 ) ) ;
#8632=CARTESIAN_POINT ( 'NONE',  ( 6.486482029760649416E-15, 57.62500000273119127, 35.31076352940723240 ) ) ;
#8635=CARTESIAN_POINT ( 'NONE',  ( 20.08610463437158344, 19.20000000546236052, 27.64615127144129403 ) ) ;
#8636=CARTESIAN_POINT ( 'NONE',  ( 7.236395654485760609, 11.52499999726880375, -22.27133577429736633 ) ) ;
#8637=CARTESIAN_POINT ( 'NONE',  ( -33.58253175000000113, 21.37500000273118062, 0.000000000000000000 ) ) ;
#8641=CARTESIAN_POINT ( 'NONE',  ( -10.04305231718579172, 33.59999999999999432, -30.90933677959248982 ) ) ;
#8643=ORIENTED_EDGE ( 'NONE', *, *, #30311, .T. ) ;
#8645=CARTESIAN_POINT ( 'NONE',  ( 4.300734207923757602, 74.27500000273118985, -13.23629886949340673 ) ) ;
#8647=CARTESIAN_POINT ( 'NONE',  ( -27.16883889988624290, 26.92500000273118133, -19.73931689729374028 ) ) ;
#8651=CARTESIAN_POINT ( 'NONE',  ( -27.16883889988623935, 11.57500000273120655, 19.73931689729374739 ) ) ;
#8653=CARTESIAN_POINT ( 'NONE',  ( 20.75514604977248467, 72.42500000273119554, -28.56700777964554305 ) ) ;
#8655=CARTESIAN_POINT ( 'NONE',  ( 0.000000000000000000, 0.000000000000000000, 0.000000000000000000 ) ) ;
#8656=CARTESIAN_POINT ( 'NONE',  ( -8.960552108402744065E-16, 78.87500000273118417, -14.63369212191046209 ) ) ;
#8659=CARTESIAN_POINT ( 'NONE',  ( -20.75514604977248823, 58.82500000273117990, -28.56700777964554305 ) ) ;
#8664=CARTESIAN_POINT ( 'NONE',  ( -32.50000000000000000, 16.10000000000001208, 10.55989012756946366 ) ) ;
#8665=CARTESIAN_POINT ( 'NONE',  ( -18.94512977948576093, 3.824999997268818674, 13.76444248337722698 ) ) ;
#8667=( BOUNDED_CURVE ( )  B_SPLINE_CURVE ( 2, ( #5099, #12826, #7153, #4926, #9906, #30834, #10083, #20562, #23298, #31007, #20216, #20898, #20738 ),
 .UNSPECIFIED., .F., .F. ) 
 B_SPLINE_CURVE_WITH_KNOTS ( ( 3, 2, 2, 2, 2, 2, 3 ),
 ( 0.5277777777777777901, 0.5333333333333333259, 0.5444444444444443976, 0.5555555555555555802, 0.5666666666666666519, 0.5777777777777777235, 0.5833333333333332593 ),
 .UNSPECIFIED. ) 
 CURVE ( )  GEOMETRIC_REPRESENTATION_ITEM ( )  RATIONAL_B_SPLINE_CURVE ( ( 0.9755282581475768211, 0.9755282581475768211, 1.000000000000000000, 0.9510565162951535312, 1.000000000000000000, 0.9510565162951535312, 1.000000000000000000, 0.9510565162951535312, 1.000000000000000000, 0.9510565162951535312, 1.000000000000000000, 0.9755282581475770431, 0.9755282581475768211 ) ) 
 REPRESENTATION_ITEM ( '' )  );
#8668=ORIENTED_EDGE ( 'NONE', *, *, #30311, .F. ) ;
#8670=CARTESIAN_POINT ( 'NONE',  ( -32.50000000000000000, 68.60000000546237686, 10.55989012756946366 ) ) ;
#8671=ORIENTED_EDGE ( 'NONE', *, *, #23447, .F. ) ;
#8672=( BOUNDED_CURVE ( )  B_SPLINE_CURVE ( 2, ( #31634, #3325, #29397, #1056, #29228, #6225, #21521, #24097, #19115, #8133, #5733, #13795, #29553 ),
 .UNSPECIFIED., .F., .T. ) 
 B_SPLINE_CURVE_WITH_KNOTS ( ( 3, 2, 2, 2, 2, 2, 3 ),
 ( 0.3782051282051281937, 0.3794871794871794712, 0.3820512820512820262, 0.3846153846153846367, 0.3871794871794871917, 0.3897435897435897467, 0.3910256410256410242 ),
 .UNSPECIFIED. ) 
 CURVE ( )  GEOMETRIC_REPRESENTATION_ITEM ( )  RATIONAL_B_SPLINE_CURVE ( ( 0.9755282581475768211, 0.9755282581475768211, 1.000000000000000000, 0.9510565162951535312, 1.000000000000000000, 0.9510565162951535312, 1.000000000000000000, 0.9510565162951535312, 1.000000000000000000, 0.9510565162951535312, 1.000000000000000000, 0.9755282581475768211, 0.9755282581475768211 ) ) 
 REPRESENTATION_ITEM ( '' )  );
#8675=CARTESIAN_POINT ( 'NONE',  ( -7.570916362186210335, 2.599999999999991207, -23.30088464923126779 ) ) ;
#8676=CARTESIAN_POINT ( 'NONE',  ( -20.75514604977248112, 71.42500000273119554, 28.56700777964554661 ) ) ;
#8678=CARTESIAN_POINT ( 'NONE',  ( 24.50000000000000355, 4.099999999999986322, -7.960532557706203605 ) ) ;
#8679=CARTESIAN_POINT ( 'NONE',  ( -10.37757302488624411, 6.975000002731185589, -31.93888565452638417 ) ) ;
#8680=CARTESIAN_POINT ( 'NONE',  ( 27.16883889988623935, 18.32500000273118346, -19.73931689729374384 ) ) ;
#8681=CARTESIAN_POINT ( 'NONE',  ( 13.91746825000000065, 75.77500000273120406, 4.522059556121115875 ) ) ;
#8684=CARTESIAN_POINT ( 'NONE',  ( 4.635254915624212657, 80.60000000000000853, 14.26584774442730286 ) ) ;
#8687=CARTESIAN_POINT ( 'NONE',  ( -26.29305231718578995, 38.70000000546236407, 19.10302069950538595 ) ) ;
#8689=CARTESIAN_POINT ( 'NONE',  ( 6.486482029760649416E-15, 41.62500000273116996, 35.31076352940723240 ) ) ;
#8692=CARTESIAN_POINT ( 'NONE',  ( 6.486482029760648627E-15, 33.87500000273118417, 35.31076352940722529 ) ) ;
#8695=CARTESIAN_POINT ( 'NONE',  ( 0.000000000000000000, 82.00000000000001421, -15.00000000000000000 ) ) ;
#8696=CARTESIAN_POINT ( 'NONE',  ( -26.29305231718578995, 44.70000000546237118, 19.10302069950538595 ) ) ;
#8699=CARTESIAN_POINT ( 'NONE',  ( -18.94512977948575738, 5.424999997268809437, -13.76444248337723231 ) ) ;
#8700=CARTESIAN_POINT ( 'NONE',  ( -10.04305231718579172, 52.10000000546239107, -30.90933677959248982 ) ) ;
#8702=CARTESIAN_POINT ( 'NONE',  ( 0.000000000000000000, 80.00000000000001421, 0.000000000000000000 ) ) ;
#8703=CARTESIAN_POINT ( 'NONE',  ( 27.16883889988624290, 21.92500000273117777, 19.73931689729373673 ) ) ;
#8704=CARTESIAN_POINT ( 'NONE',  ( 23.41746825000000243, 9.024999997268826846, 7.608796670333735079 ) ) ;
#8708=ORIENTED_EDGE ( 'NONE', *, *, #25136, .T. ) ;
#8711=CARTESIAN_POINT ( 'NONE',  ( 32.50000000000000000, 39.10000000000001563, -10.55989012756945833 ) ) ;
#8712=CARTESIAN_POINT ( 'NONE',  ( -7.236395654485763274, 8.024999997268800200, 22.27133577429736633 ) ) ;
#8713=CARTESIAN_POINT ( 'NONE',  ( -27.16883889988623935, 27.57500000273119412, 19.73931689729374739 ) ) ;
#8714=CARTESIAN_POINT ( 'NONE',  ( -26.29305231718579350, 28.30000000546237260, -19.10302069950537884 ) ) ;
#8715=CARTESIAN_POINT ( 'NONE',  ( -32.50000000000000000, 70.00000000000000000, 0.000000000000000000 ) ) ;
#8717=CARTESIAN_POINT ( 'NONE',  ( 7.313012447739250820E-14, 11.49999999999999112, 24.50000000000000000 ) ) ;
#8719=CARTESIAN_POINT ( 'NONE',  ( 20.75514604977249178, 44.07500000273117990, 28.56700777964553950 ) ) ;
#8721=CARTESIAN_POINT ( 'NONE',  ( 18.94512977948575738, 10.92499999726881299, 13.76444248337723408 ) ) ;
#8722=CARTESIAN_POINT ( 'NONE',  ( -10.04305231718578462, 18.39999999999999858, 30.90933677959249337 ) ) ;
#8724=EDGE_CURVE ( 'NONE', #19688, #30562, #19039, .T. ) ;
#8726=CARTESIAN_POINT ( 'NONE',  ( -33.58253175000000113, 63.12500000273119127, 0.000000000000000000 ) ) ;
#8727=CARTESIAN_POINT ( 'NONE',  ( 20.75514604977249178, 56.07500000273117990, 28.56700777964553950 ) ) ;
#8731=CARTESIAN_POINT ( 'NONE',  ( 10.37757302488624767, 3.725000002731182480, 31.93888565452638417 ) ) ;
#8733=CARTESIAN_POINT ( 'NONE',  ( 5.147494310547434893, 25.05125428700921830, 32.49999999999999289 ) ) ;
#8734=CARTESIAN_POINT ( 'NONE',  ( -32.50000000000000000, 19.99999999999998934, 0.000000000000000000 ) ) ;
#8738=CARTESIAN_POINT ( 'NONE',  ( 32.50000000000000711, 1.400000005462371799, 10.55989012756945122 ) ) ;
#8739=EDGE_CURVE ( 'NONE', #15393, #1219, #1434, .T. ) ;
#8752=CARTESIAN_POINT ( 'NONE',  ( 0.000000000000000000, 80.00000000000001421, 0.000000000000000000 ) ) ;
#8753=CARTESIAN_POINT ( 'NONE',  ( 10.37757302488624056, 50.77500000273118985, -31.93888565452638417 ) ) ;
#8754=CARTESIAN_POINT ( 'NONE',  ( -32.50000000000000000, 52.50000000546236834, 0.000000000000000000 ) ) ;
#8756=CARTESIAN_POINT ( 'NONE',  ( -27.16883889988624290, 38.92500000273118843, -19.73931689729374028 ) ) ;
#8757=CARTESIAN_POINT ( 'NONE',  ( 5.779280353836490358E-15, 27.00000000546237544, 32.49999999999999289 ) ) ;
#8758=CARTESIAN_POINT ( 'NONE',  ( -2.162160676586881955E-15, 64.87500000273119838, -35.31076352940723240 ) ) ;
#8760=CARTESIAN_POINT ( 'NONE',  ( 32.50000000000000711, 38.89999999999999147, 10.55989012756945122 ) ) ;
#8762=( BOUNDED_CURVE ( )  B_SPLINE_CURVE ( 2, ( #20663, #26129, #15504, #2103, #12576, #18252, #33505, #28867, #20481, #25787, #8104, #28699, #15844, #2452, #23730, #26301, #30932, #2276, #21164, #7425, #31606, #31103, #31272, #12750, #23223, #33682, #7599, #5196, #12918, #25958, #23563, #6193, #13431, #5867, #8601, #5704, #18591, #3458, #18756, #24231, #19248, #23899, #8264, #29199, #14099, #21331, #8765, #29367, #29687, #13929, #11348, #16182, #24393, #21989, #31939, #21658, #21825, #11022, #32272, #26469, #19084, #26637, #29031, #867, #3131, #702, #16674, #18921, #16345, #11188, #27130, #26958, #29524, #11509, #3295, #3625, #370, #24555, #1028, #13604, #32437, #24069, #535, #26801, #32103, #6027, #21492, #8432, #16505, #13761, #5534, #16015, #10856, #2962, #31772, #22326, #22657, #22161, #4294, #8936, #29865, #6868, #14941, #27639, #19919, #27980, #14602, #4127, #25059, #25406, #1884, #33111, #25234, #22485, #27300, #1540, #12016, #32936, #19584, #6698, #9434, #14769, #9613, #1709, #30367, #17347, #24887, #27810, #20095, #12187, #30540, #30032, #7036, #17519, #6537, #14263, #4467, #17010, #27469, #12362, #3958, #6366, #32771, #22830, #19416, #16844, #3792, #24721, #32604, #1197, #11678, #9103, #14432, #9265, #1371, #11847, #19749, #30197, #17181, #4807, #4982, #13211, #23354, #26088, #7556, #18379, #23521, #28151, #18041, #31062, #18212, #20266, #15461, #28654, #33290, #2228, #2410, #4637, #9788, #17867, #30713, #12705, #12877, #2585, #25746, #13049, #7208, #33816, #2747, #15286, #15116, #17691, #23176, #5323, #7892, #25580, #23005, #33980, #33638, #2060, #10137, #28485, #10474, #12536, #20952, #7724, #9962, #15803, #20619, #5151, #20437, #33462, #30887, #10309, #25916, #20787, #31232, #7383, #15637, #28319, #31401, #28825, #26259, #3417, #2920, #19047, #23688, #10643, #153, #21453, #26921, #13891, #24189, #8727, #24358, #3254, #5492, #18877, #21293, #29326, #5989, #8062, #8392, #26762, #13724, #326, #31896, #661, #10979, #21120, #21787, #21620, #26427, #5828, #6150, #828, #29154, #18547, #19211, #13389, #11149, #31733, #28993, #11309, #10813, #8224, #32063, #18718, #5660, #16143, #29648, #29486, #16466, #32235, #15971, #16635, #31564, #16307, #27091, #26596, #8563, #23861, #3093, #3585, #13564, #24027, #496, #11638, #27942, #4086, #6824, #22287, #9225, #19709, #20052, #6998, #27769, #30328, #27595, #32399, #32732, #17480, #14057, #24519, #32565, #25190, #9391, #4254, #19875, #1500, #14561, #29993, #30155, #1668, #6659, #17142, #24682, #17307, #22616, #22122, #19378, #25020, #24848, #8894, #29824, #11977, #11474, #3919, #22445, #14729, #32892, #9575, #12143, #3752, #33069, #30497, #989, #21948, #14392, #14226, #6328, #16805, #27261, #1156, #9064, #19545, #6497, #16970, #27428, #1328, #11811, #28612, #33245, #4597, #33944, #7167, #5112, #15245, #15596, #23313, #31194, #22964, #14900, #10097, #12662, #31361, #4767, #26050, #9743, #25707, #28447, #25542, #4425, #33778, #15074, #20576, #2544, #2188, #23131, #31020, #20751, #25364, #7339, #30848, #28110, #1842, #13010, #10435, #7684, #22792, #23482, #33422, #2020, #33597, #7517, #18002, #9920, #12495, #4938, #15420, #12839, #20229, #20397, #20910, #25874, #7853, #12322, #18341, #17649, #30669, #17824, #2366, #18170, #28281, #10269, #13855, #32029, #18682, #10943, #5624, #21418, #26391, #26727, #2884, #13350, #23823, #24321, #24154, #11114, #19010, #13175, #8526, #26221, #461, #794, #21254, #3222, #29121, #5284, #23652, #18843, #31861, #289, #8354, #10777, #16436, #8191, #13690, #15767, #3055, #26559, #625, #2713, #29289, #21583, #8692, #31698, #5789, #114, #28786, #16108, #32198, #13526, #16270, #29454, #23989, #5956, #10606, #26888, #21084, #3385, #31533, #8026, #11277, #21753, #18512, #28958, #5454, #15935, #1115, #6115, #12104, #3879, #19834, #24481, #9352, #27557, #29782, #1626, #9025, #14519, #6287, #19338, #16763, #22248, #6458, #16932, #27390, #29613, #14352, #3546, #17099, #11766, #32525, #19507, #9187, #17266, #21912, #16598, #27053, #24809, #22408, #30287, #19671, #4217, #32856, #32692, #955, #1287, #27222, #30116, #6620, #14018, #4045, #24978, #1461, #3715, #11939, #6788, #27729, #11435, #14691, #25150, #32362, #22575, #33026, #19176, #24641, #8856, #14185, #11600, #22081, #29954, #33555, #4384, #15381, #20012, #7126, #23443, #10055, #2325, #17782, #28575, #33735, #14859, #9705, #5071, #12278, #10232, #20357, #20712, #25325, #9531, #28069, #30459, #15206, #28240, #2501, #9877, #31154, #1800, #30804, #20536, #30629, #6956, #28410, #20185, #25670, #7645, #7297, #4725, #25837, #17961, #30980, #12969, #2149, #18131, #22751, #15555, #4900, #17607, #26008, #33381, #12799, #4556, #15035, #25500, #12624, #23092, #7480, #23272, #17440, #27902, #33202, #1980, #12455, #22925, #13307, #23950, #31989, #2677, #20874, #10395, #31656, #3183, #24117, #419, #18972, #13652, #13485, #15727, #26849, #584, #16233, #10906, #18302, #18642, #3013, #21378, #10564, #8153, #31823, #21211, #31322, #8485, #8314, #13135, #29079, #16396, #11075, #5414, #26519, #21043, #21540, #29417, #31493, #5245, #5919, #7983, #18471, #18804, #28913, #15893, #26349, #3346, #29248, #26687, #13816, #28747, #33904, #7813, #26182, #23609, #5752, #249, #77, #2839, #5584, #23782, #10734, #16064, #19468, #29917, #30244, #17229, #4007, #6583, #3839, #8651, #8987, #27354, #27689, #752, #8815, #1422, #19632, #14481, #30077, #11726, #14314, #6247, #6419, #11900, #16891, #24769, #918, #27520, #32819, #21874, #29573, #24937, #1079, #19136, #6074, #1247, #21712, #14149, #32655, #22372, #22208, #19796, #9150, #13978, #17058, #9311, #6749, #4179, #24605, #24441, #24283, #11236, #16558, #32158, #27011, #32324, #3508, #11397, #19298, #32485, #29742, #16727, #27182, #3675, #11559, #22041, #5328, #25463, #26264, #33986, #7899, #4346, #25113, #20318, #22886, #8067, #14993, #2752, #9490, #1938, #5157, #1758, #14653, #10479, #14821, #30767, #15809, #12416, #33343, #7729, #31406, #23526, #17572, #7088, #25286, #12065, #23693, #10649, #18384, #32986, #159, #33164, #12238, #9840, #18218, #28662, #9667, #22714, #15642, #26093, #20957, #28830 ),
 .UNSPECIFIED., .F., .F. ) 
 B_SPLINE_CURVE_WITH_KNOTS ( ( 3, 2, 2, 2, 2, 2, 2, 2, 2, 2, 2, 2, 2, 2, 2, 2, 2, 2, 2, 2, 2, 2, 2, 2, 2, 2, 2, 2, 2, 2, 2, 2, 2, 2, 2, 2, 2, 2, 2, 2, 2, 2, 2, 2, 2, 2, 2, 2, 2, 2, 2, 2, 2, 2, 2, 2, 2, 2, 2, 2, 2, 2, 2, 2, 2, 2, 2, 2, 2, 2, 2, 2, 2, 2, 2, 2, 2, 2, 2, 2, 2, 2, 2, 2, 2, 2, 2, 2, 2, 2, 2, 2, 2, 2, 2, 2, 2, 2, 2, 2, 2, 2, 2, 2, 2, 2, 2, 2, 2, 2, 2, 2, 2, 2, 2, 2, 2, 2, 2, 2, 2, 2, 2, 2, 2, 2, 2, 2, 2, 2, 2, 2, 2, 2, 2, 2, 2, 2, 2, 2, 2, 2, 2, 2, 2, 2, 2, 2, 2, 2, 2, 2, 2, 2, 2, 2, 2, 2, 2, 2, 2, 2, 2, 2, 2, 2, 2, 2, 2, 2, 2, 2, 2, 2, 2, 2, 2, 2, 2, 2, 2, 2, 2, 2, 2, 2, 2, 2, 2, 2, 2, 2, 2, 2, 2, 2, 2, 2, 2, 2, 2, 2, 2, 2, 2, 2, 2, 2, 2, 2, 2, 2, 2, 2, 2, 2, 2, 2, 2, 2, 2, 2, 2, 2, 2, 2, 2, 2, 2, 2, 2, 2, 2, 2, 2, 2, 2, 2, 2, 2, 2, 2, 2, 2, 2, 2, 2, 2, 2, 2, 2, 2, 2, 2, 2, 2, 2, 2, 2, 2, 2, 2, 2, 2, 2, 2, 2, 2, 2, 2, 2, 2, 2, 2, 2, 2, 2, 2, 2, 2, 2, 2, 2, 2, 2, 2, 2, 2, 2, 2, 2, 2, 2, 2, 2, 2, 2, 2, 2, 2, 2, 2, 2, 2, 2, 2, 2, 2, 2, 2, 2, 2, 2, 2, 2, 2, 2, 2, 2, 2, 2, 2, 2, 2, 2, 2, 2, 2, 2, 2, 2, 2, 2, 2, 2, 2, 2, 2, 2, 2, 2, 2, 2, 2, 2, 2, 2, 2, 2, 2, 2, 2, 2, 2, 2, 2, 2, 2, 2, 2, 2, 2, 2, 2, 2, 2, 2, 2, 2, 2, 2, 2, 2, 2, 2, 2, 2, 2, 2, 2, 2, 2, 2, 2, 2, 2, 2, 2, 2, 2, 3 ),
 ( 0.000000000000000000, 0.002564102564102564100, 0.005128205128205128201, 0.007692307692307692735, 0.01025641025641025640, 0.01282051282051282007, 0.01538461538461538547, 0.01794871794871794740, 0.02051282051282051280, 0.02307692307692307820, 0.02564102564102564014, 0.02820512820512820554, 0.03076923076923077094, 0.03333333333333333287, 0.03589743589743589480, 0.03846153846153846367, 0.04102564102564102561, 0.04358974358974358754, 0.04615384615384615641, 0.04871794871794871834, 0.05128205128205128027, 0.05384615384615384914, 0.05641025641025641107, 0.05897435897435897301, 0.06153846153846154188, 0.06410256410256409687, 0.06666666666666666574, 0.06923076923076923461, 0.07179487179487178961, 0.07435897435897435848, 0.07692307692307692735, 0.07948717948717948234, 0.08205128205128205121, 0.08461538461538462008, 0.08717948717948717507, 0.08974358974358974395, 0.09230769230769231282, 0.09487179487179486781, 0.09743589743589743668, 0.1000000000000000056, 0.1025641025641025605, 0.1051282051282051294, 0.1076923076923076983, 0.1102564102564102533, 0.1128205128205128221, 0.1153846153846153910, 0.1179487179487179460, 0.1205128205128205149, 0.1230769230769230838, 0.1256410256410256387, 0.1282051282051281937, 0.1307692307692307765, 0.1333333333333333315, 0.1358974358974358865, 0.1384615384615384692, 0.1410256410256410242, 0.1435897435897435792, 0.1461538461538461620, 0.1487179487179487170, 0.1512820512820512719, 0.1538461538461538547, 0.1564102564102564097, 0.1589743589743589647, 0.1615384615384615474, 0.1641025641025641024, 0.1666666666666666574, 0.1692307692307692402, 0.1717948717948717952, 0.1743589743589743501, 0.1769230769230769329, 0.1794871794871794879, 0.1820512820512820429, 0.1846153846153846256, 0.1871794871794871806, 0.1897435897435897356, 0.1923076923076923184, 0.1948717948717948734, 0.1974358974358974284, 0.2000000000000000111, 0.2025641025641025661, 0.2051282051282051211, 0.2076923076923077038, 0.2102564102564102588, 0.2128205128205128138, 0.2153846153846153966, 0.2179487179487179516, 0.2205128205128205066, 0.2230769230769230893, 0.2256410256410256443, 0.2282051282051281993, 0.2307692307692307820, 0.2333333333333333370, 0.2358974358974358920, 0.2384615384615384748, 0.2410256410256410298, 0.2435897435897435848, 0.2461538461538461675, 0.2487179487179487225, 0.2512820512820512775, 0.2538461538461538325, 0.2564102564102563875, 0.2589743589743589980, 0.2615384615384615530, 0.2641025641025641080, 0.2666666666666666630, 0.2692307692307692180, 0.2717948717948717730, 0.2743589743589743835, 0.2769230769230769384, 0.2794871794871794934, 0.2820512820512820484, 0.2846153846153846034, 0.2871794871794871584, 0.2897435897435897689, 0.2923076923076923239, 0.2948717948717948789, 0.2974358974358974339, 0.2999999999999999889, 0.3025641025641025439, 0.3051282051282051544, 0.3076923076923077094, 0.3102564102564102644, 0.3128205128205128194, 0.3153846153846153744, 0.3179487179487179294, 0.3205128205128205399, 0.3230769230769230949, 0.3256410256410256499, 0.3282051282051282048, 0.3307692307692307598, 0.3333333333333333148, 0.3358974358974358698, 0.3384615384615384803, 0.3410256410256410353, 0.3435897435897435903, 0.3461538461538461453, 0.3487179487179487003, 0.3512820512820512553, 0.3538461538461538658, 0.3564102564102564208, 0.3589743589743589758, 0.3615384615384615308, 0.3641025641025640858, 0.3666666666666666408, 0.3692307692307692513, 0.3717948717948718063, 0.3743589743589743613, 0.3769230769230769162, 0.3794871794871794712, 0.3820512820512820262, 0.3846153846153846367, 0.3871794871794871917, 0.3897435897435897467, 0.3923076923076923017, 0.3948717948717948567, 0.3974358974358974117, 0.4000000000000000222, 0.4025641025641025772, 0.4051282051282051322, 0.4076923076923076872, 0.4102564102564102422, 0.4128205128205127972, 0.4153846153846154077, 0.4179487179487179627, 0.4205128205128205177, 0.4230769230769230727, 0.4256410256410256276, 0.4282051282051281826, 0.4307692307692307931, 0.4333333333333333481, 0.4358974358974359031, 0.4384615384615384581, 0.4410256410256410131, 0.4435897435897435681, 0.4461538461538461786, 0.4487179487179487336, 0.4512820512820512886, 0.4538461538461538436, 0.4564102564102563986, 0.4589743589743589536, 0.4615384615384615641, 0.4641025641025641191, 0.4666666666666666741, 0.4692307692307692291, 0.4717948717948717841, 0.4743589743589743390, 0.4769230769230769496, 0.4794871794871795045, 0.4820512820512820595, 0.4846153846153846145, 0.4871794871794871695, 0.4897435897435897245, 0.4923076923076923350, 0.4948717948717948900, 0.4974358974358974450, 0.5000000000000000000, 0.5025641025641025550, 0.5051282051282051100, 0.5076923076923076650, 0.5102564102564102200, 0.5128205128205127750, 0.5153846153846153300, 0.5179487179487179960, 0.5205128205128205510, 0.5230769230769231060, 0.5256410256410256610, 0.5282051282051282159, 0.5307692307692307709, 0.5333333333333333259, 0.5358974358974358809, 0.5384615384615384359, 0.5410256410256409909, 0.5435897435897435459, 0.5461538461538461009, 0.5487179487179487669, 0.5512820512820513219, 0.5538461538461538769, 0.5564102564102564319, 0.5589743589743589869, 0.5615384615384615419, 0.5641025641025640969, 0.5666666666666666519, 0.5692307692307692069, 0.5717948717948717618, 0.5743589743589743168, 0.5769230769230768718, 0.5794871794871795379, 0.5820512820512820928, 0.5846153846153846478, 0.5871794871794872028, 0.5897435897435897578, 0.5923076923076923128, 0.5948717948717948678, 0.5974358974358974228, 0.5999999999999999778, 0.6025641025641025328, 0.6051282051282050878, 0.6076923076923076428, 0.6102564102564103088, 0.6128205128205128638, 0.6153846153846154188, 0.6179487179487179738, 0.6205128205128205288, 0.6230769230769230838, 0.6256410256410256387, 0.6282051282051281937, 0.6307692307692307487, 0.6333333333333333037, 0.6358974358974358587, 0.6384615384615384137, 0.6410256410256410797, 0.6435897435897436347, 0.6461538461538461897, 0.6487179487179487447, 0.6512820512820512997, 0.6538461538461538547, 0.6564102564102564097, 0.6589743589743589647, 0.6615384615384615197, 0.6641025641025640747, 0.6666666666666666297, 0.6692307692307691847, 0.6717948717948717396, 0.6743589743589744057, 0.6769230769230769607, 0.6794871794871795156, 0.6820512820512820706, 0.6846153846153846256, 0.6871794871794871806, 0.6897435897435897356, 0.6923076923076922906, 0.6948717948717948456, 0.6974358974358974006, 0.6999999999999999556, 0.7025641025641025106, 0.7051282051282051766, 0.7076923076923077316, 0.7102564102564102866, 0.7128205128205128416, 0.7153846153846153966, 0.7179487179487179516, 0.7205128205128205066, 0.7230769230769230616, 0.7256410256410256165, 0.7282051282051281715, 0.7307692307692307265, 0.7333333333333332815, 0.7358974358974359475, 0.7384615384615385025, 0.7410256410256410575, 0.7435897435897436125, 0.7461538461538461675, 0.7487179487179487225, 0.7512820512820512775, 0.7538461538461538325, 0.7564102564102563875, 0.7589743589743589425, 0.7615384615384614975, 0.7641025641025640525, 0.7666666666666667185, 0.7692307692307692735, 0.7717948717948718285, 0.7743589743589743835, 0.7769230769230769384, 0.7794871794871794934, 0.7820512820512820484, 0.7846153846153846034, 0.7871794871794871584, 0.7897435897435897134, 0.7923076923076922684, 0.7948717948717948234, 0.7974358974358974894, 0.8000000000000000444, 0.8025641025641025994, 0.8051282051282051544, 0.8076923076923077094, 0.8102564102564102644, 0.8128205128205128194, 0.8153846153846153744, 0.8179487179487179294, 0.8205128205128204844, 0.8230769230769230393, 0.8256410256410255943, 0.8282051282051282604, 0.8307692307692308153, 0.8333333333333333703, 0.8358974358974359253, 0.8384615384615384803, 0.8410256410256410353, 0.8435897435897435903, 0.8461538461538461453, 0.8487179487179487003, 0.8512820512820512553, 0.8538461538461538103, 0.8564102564102563653, 0.8589743589743589203, 0.8615384615384615863, 0.8641025641025641413, 0.8666666666666666963, 0.8692307692307692513, 0.8717948717948718063, 0.8743589743589743613, 0.8769230769230769162, 0.8794871794871794712, 0.8820512820512820262, 0.8846153846153845812, 0.8871794871794871362, 0.8897435897435896912, 0.8923076923076923572, 0.8948717948717949122, 0.8974358974358974672, 0.9000000000000000222, 0.9025641025641025772, 0.9051282051282051322, 0.9076923076923076872, 0.9102564102564102422, 0.9128205128205127972, 0.9153846153846153522, 0.9179487179487179072, 0.9205128205128204621, 0.9230769230769231282, 0.9256410256410256832, 0.9282051282051282382, 0.9307692307692307931, 0.9333333333333333481, 0.9358974358974359031, 0.9384615384615384581, 0.9410256410256410131, 0.9435897435897435681, 0.9461538461538461231, 0.9487179487179486781, 0.9512820512820512331, 0.9538461538461538991, 0.9564102564102564541, 0.9589743589743590091, 0.9615384615384615641, 0.9641025641025641191, 0.9666666666666666741, 0.9692307692307692291, 0.9717948717948717841, 0.9743589743589743390, 0.9769230769230768940, 0.9794871794871794490, 0.9820512820512820040, 0.9846153846153846700, 0.9871794871794872250, 0.9897435897435897800, 0.9923076923076923350, 0.9948717948717948900, 0.9974358974358974450, 1.000000000000000000 ),
 .UNSPECIFIED. ) 
 CURVE ( )  GEOMETRIC_REPRESENTATION_ITEM ( )  RATIONAL_B_SPLINE_CURVE ( ( 1.000000000000000000, 0.9510565162951535312, 1.000000000000000000, 0.9510565162951535312, 1.000000000000000000, 0.9510565162951535312, 1.000000000000000000, 0.9510565162951535312, 1.000000000000000000, 0.9510565162951535312, 1.000000000000000000, 0.9510565162951535312, 1.000000000000000000, 0.9510565162951535312, 1.000000000000000000, 0.9510565162951535312, 1.000000000000000000, 0.9510565162951535312, 1.000000000000000000, 0.9510565162951535312, 1.000000000000000000, 0.9510565162951535312, 1.000000000000000000, 0.9510565162951535312, 1.000000000000000000, 0.9510565162951535312, 1.000000000000000000, 0.9510565162951535312, 1.000000000000000000, 0.9510565162951535312, 1.000000000000000000, 0.9510565162951535312, 1.000000000000000000, 0.9510565162951535312, 1.000000000000000000, 0.9510565162951535312, 1.000000000000000000, 0.9510565162951535312, 1.000000000000000000, 0.9510565162951535312, 1.000000000000000000, 0.9510565162951535312, 1.000000000000000000, 0.9510565162951535312, 1.000000000000000000, 0.9510565162951535312, 1.000000000000000000, 0.9510565162951535312, 1.000000000000000000, 0.9510565162951535312, 1.000000000000000000, 0.9510565162951535312, 1.000000000000000000, 0.9510565162951535312, 1.000000000000000000, 0.9510565162951535312, 1.000000000000000000, 0.9510565162951535312, 1.000000000000000000, 0.9510565162951535312, 1.000000000000000000, 0.9510565162951535312, 1.000000000000000000, 0.9510565162951535312, 1.000000000000000000, 0.9510565162951535312, 1.000000000000000000, 0.9510565162951535312, 1.000000000000000000, 0.9510565162951535312, 1.000000000000000000, 0.9510565162951535312, 1.000000000000000000, 0.9510565162951535312, 1.000000000000000000, 0.9510565162951535312, 1.000000000000000000, 0.9510565162951535312, 1.000000000000000000, 0.9510565162951535312, 1.000000000000000000, 0.9510565162951535312, 1.000000000000000000, 0.9510565162951535312, 1.000000000000000000, 0.9510565162951535312, 1.000000000000000000, 0.9510565162951535312, 1.000000000000000000, 0.9510565162951535312, 1.000000000000000000, 0.9510565162951535312, 1.000000000000000000, 0.9510565162951535312, 1.000000000000000000, 0.9510565162951535312, 1.000000000000000000, 0.9510565162951535312, 1.000000000000000000, 0.9510565162951535312, 1.000000000000000000, 0.9510565162951535312, 1.000000000000000000, 0.9510565162951535312, 1.000000000000000000, 0.9510565162951535312, 1.000000000000000000, 0.9510565162951535312, 1.000000000000000000, 0.9510565162951535312, 1.000000000000000000, 0.9510565162951535312, 1.000000000000000000, 0.9510565162951535312, 1.000000000000000000, 0.9510565162951535312, 1.000000000000000000, 0.9510565162951535312, 1.000000000000000000, 0.9510565162951535312, 1.000000000000000000, 0.9510565162951535312, 1.000000000000000000, 0.9510565162951535312, 1.000000000000000000, 0.9510565162951535312, 1.000000000000000000, 0.9510565162951535312, 1.000000000000000000, 0.9510565162951535312, 1.000000000000000000, 0.9510565162951535312, 1.000000000000000000, 0.9510565162951535312, 1.000000000000000000, 0.9510565162951535312, 1.000000000000000000, 0.9510565162951535312, 1.000000000000000000, 0.9510565162951535312, 1.000000000000000000, 0.9510565162951535312, 1.000000000000000000, 0.9510565162951535312, 1.000000000000000000, 0.9510565162951535312, 1.000000000000000000, 0.9510565162951535312, 1.000000000000000000, 0.9510565162951535312, 1.000000000000000000, 0.9510565162951535312, 1.000000000000000000, 0.9510565162951535312, 1.000000000000000000, 0.9510565162951535312, 1.000000000000000000, 0.9510565162951535312, 1.000000000000000000, 0.9510565162951535312, 1.000000000000000000, 0.9510565162951535312, 1.000000000000000000, 0.9510565162951535312, 1.000000000000000000, 0.9510565162951535312, 1.000000000000000000, 0.9510565162951535312, 1.000000000000000000, 0.9510565162951535312, 1.000000000000000000, 0.9510565162951535312, 1.000000000000000000, 0.9510565162951535312, 1.000000000000000000, 0.9510565162951535312, 1.000000000000000000, 0.9510565162951535312, 1.000000000000000000, 0.9510565162951535312, 1.000000000000000000, 0.9510565162951535312, 1.000000000000000000, 0.9510565162951535312, 1.000000000000000000, 0.9510565162951535312, 1.000000000000000000, 0.9510565162951535312, 1.000000000000000000, 0.9510565162951535312, 1.000000000000000000, 0.9510565162951535312, 1.000000000000000000, 0.9510565162951535312, 1.000000000000000000, 0.9510565162951535312, 1.000000000000000000, 0.9510565162951535312, 1.000000000000000000, 0.9510565162951535312, 1.000000000000000000, 0.9510565162951535312, 1.000000000000000000, 0.9510565162951535312, 1.000000000000000000, 0.9510565162951535312, 1.000000000000000000, 0.9510565162951535312, 1.000000000000000000, 0.9510565162951535312, 1.000000000000000000, 0.9510565162951535312, 1.000000000000000000, 0.9510565162951535312, 1.000000000000000000, 0.9510565162951535312, 1.000000000000000000, 0.9510565162951535312, 1.000000000000000000, 0.9510565162951535312, 1.000000000000000000, 0.9510565162951535312, 1.000000000000000000, 0.9510565162951535312, 1.000000000000000000, 0.9510565162951535312, 1.000000000000000000, 0.9510565162951535312, 1.000000000000000000, 0.9510565162951535312, 1.000000000000000000, 0.9510565162951535312, 1.000000000000000000, 0.9510565162951535312, 1.000000000000000000, 0.9510565162951535312, 1.000000000000000000, 0.9510565162951535312, 1.000000000000000000, 0.9510565162951535312, 1.000000000000000000, 0.9510565162951535312, 1.000000000000000000, 0.9510565162951535312, 1.000000000000000000, 0.9510565162951535312, 1.000000000000000000, 0.9510565162951535312, 1.000000000000000000, 0.9510565162951535312, 1.000000000000000000, 0.9510565162951535312, 1.000000000000000000, 0.9510565162951535312, 1.000000000000000000, 0.9510565162951535312, 1.000000000000000000, 0.9510565162951535312, 1.000000000000000000, 0.9510565162951535312, 1.000000000000000000, 0.9510565162951535312, 1.000000000000000000, 0.9510565162951535312, 1.000000000000000000, 0.9510565162951535312, 1.000000000000000000, 0.9510565162951535312, 1.000000000000000000, 0.9510565162951535312, 1.000000000000000000, 0.9510565162951535312, 1.000000000000000000, 0.9510565162951535312, 1.000000000000000000, 0.9510565162951535312, 1.000000000000000000, 0.9510565162951535312, 1.000000000000000000, 0.9510565162951535312, 1.000000000000000000, 0.9510565162951535312, 1.000000000000000000, 0.9510565162951535312, 1.000000000000000000, 0.9510565162951535312, 1.000000000000000000, 0.9510565162951535312, 1.000000000000000000, 0.9510565162951535312, 1.000000000000000000, 0.9510565162951535312, 1.000000000000000000, 0.9510565162951535312, 1.000000000000000000, 0.9510565162951535312, 1.000000000000000000, 0.9510565162951535312, 1.000000000000000000, 0.9510565162951535312, 1.000000000000000000, 0.9510565162951535312, 1.000000000000000000, 0.9510565162951535312, 1.000000000000000000, 0.9510565162951535312, 1.000000000000000000, 0.9510565162951535312, 1.000000000000000000, 0.9510565162951535312, 1.000000000000000000, 0.9510565162951535312, 1.000000000000000000, 0.9510565162951535312, 1.000000000000000000, 0.9510565162951535312, 1.000000000000000000, 0.9510565162951535312, 1.000000000000000000, 0.9510565162951535312, 1.000000000000000000, 0.9510565162951535312, 1.000000000000000000, 0.9510565162951535312, 1.000000000000000000, 0.9510565162951535312, 1.000000000000000000, 0.9510565162951535312, 1.000000000000000000, 0.9510565162951535312, 1.000000000000000000, 0.9510565162951535312, 1.000000000000000000, 0.9510565162951535312, 1.000000000000000000, 0.9510565162951535312, 1.000000000000000000, 0.9510565162951535312, 1.000000000000000000, 0.9510565162951535312, 1.000000000000000000, 0.9510565162951535312, 1.000000000000000000, 0.9510565162951535312, 1.000000000000000000, 0.9510565162951535312, 1.000000000000000000, 0.9510565162951535312, 1.000000000000000000, 0.9510565162951535312, 1.000000000000000000, 0.9510565162951535312, 1.000000000000000000, 0.9510565162951535312, 1.000000000000000000, 0.9510565162951535312, 1.000000000000000000, 0.9510565162951535312, 1.000000000000000000, 0.9510565162951535312, 1.000000000000000000, 0.9510565162951535312, 1.000000000000000000, 0.9510565162951535312, 1.000000000000000000, 0.9510565162951535312, 1.000000000000000000, 0.9510565162951535312, 1.000000000000000000, 0.9510565162951535312, 1.000000000000000000, 0.9510565162951535312, 1.000000000000000000, 0.9510565162951535312, 1.000000000000000000, 0.9510565162951535312, 1.000000000000000000, 0.9510565162951535312, 1.000000000000000000, 0.9510565162951535312, 1.000000000000000000, 0.9510565162951535312, 1.000000000000000000, 0.9510565162951535312, 1.000000000000000000, 0.9510565162951535312, 1.000000000000000000, 0.9510565162951535312, 1.000000000000000000, 0.9510565162951535312, 1.000000000000000000, 0.9510565162951535312, 1.000000000000000000, 0.9510565162951535312, 1.000000000000000000, 0.9510565162951535312, 1.000000000000000000, 0.9510565162951535312, 1.000000000000000000, 0.9510565162951535312, 1.000000000000000000, 0.9510565162951535312, 1.000000000000000000, 0.9510565162951535312, 1.000000000000000000, 0.9510565162951535312, 1.000000000000000000, 0.9510565162951535312, 1.000000000000000000, 0.9510565162951535312, 1.000000000000000000, 0.9510565162951535312, 1.000000000000000000, 0.9510565162951535312, 1.000000000000000000, 0.9510565162951535312, 1.000000000000000000, 0.9510565162951535312, 1.000000000000000000, 0.9510565162951535312, 1.000000000000000000, 0.9510565162951535312, 1.000000000000000000, 0.9510565162951535312, 1.000000000000000000, 0.9510565162951535312, 1.000000000000000000, 0.9510565162951535312, 1.000000000000000000, 0.9510565162951535312, 1.000000000000000000, 0.9510565162951535312, 1.000000000000000000, 0.9510565162951535312, 1.000000000000000000, 0.9510565162951535312, 1.000000000000000000, 0.9510565162951535312, 1.000000000000000000, 0.9510565162951535312, 1.000000000000000000, 0.9510565162951535312, 1.000000000000000000, 0.9510565162951535312, 1.000000000000000000, 0.9510565162951535312, 1.000000000000000000, 0.9510565162951535312, 1.000000000000000000, 0.9510565162951535312, 1.000000000000000000, 0.9510565162951535312, 1.000000000000000000, 0.9510565162951535312, 1.000000000000000000, 0.9510565162951535312, 1.000000000000000000, 0.9510565162951535312, 1.000000000000000000, 0.9510565162951535312, 1.000000000000000000, 0.9510565162951535312, 1.000000000000000000, 0.9510565162951535312, 1.000000000000000000, 0.9510565162951535312, 1.000000000000000000, 0.9510565162951535312, 1.000000000000000000, 0.9510565162951535312, 1.000000000000000000, 0.9510565162951535312, 1.000000000000000000, 0.9510565162951535312, 1.000000000000000000, 0.9510565162951535312, 1.000000000000000000, 0.9510565162951535312, 1.000000000000000000, 0.9510565162951535312, 1.000000000000000000, 0.9510565162951535312, 1.000000000000000000, 0.9510565162951535312, 1.000000000000000000, 0.9510565162951535312, 1.000000000000000000, 0.9510565162951535312, 1.000000000000000000, 0.9510565162951535312, 1.000000000000000000, 0.9510565162951535312, 1.000000000000000000, 0.9510565162951535312, 1.000000000000000000, 0.9510565162951535312, 1.000000000000000000, 0.9510565162951535312, 1.000000000000000000, 0.9510565162951535312, 1.000000000000000000, 0.9510565162951535312, 1.000000000000000000, 0.9510565162951535312, 1.000000000000000000, 0.9510565162951535312, 1.000000000000000000, 0.9510565162951535312, 1.000000000000000000, 0.9510565162951535312, 1.000000000000000000, 0.9510565162951535312, 1.000000000000000000, 0.9510565162951535312, 1.000000000000000000, 0.9510565162951535312, 1.000000000000000000, 0.9510565162951535312, 1.000000000000000000, 0.9510565162951535312, 1.000000000000000000, 0.9510565162951535312, 1.000000000000000000, 0.9510565162951535312, 1.000000000000000000, 0.9510565162951535312, 1.000000000000000000, 0.9510565162951535312, 1.000000000000000000, 0.9510565162951535312, 1.000000000000000000, 0.9510565162951535312, 1.000000000000000000, 0.9510565162951535312, 1.000000000000000000, 0.9510565162951535312, 1.000000000000000000, 0.9510565162951535312, 1.000000000000000000, 0.9510565162951535312, 1.000000000000000000, 0.9510565162951535312, 1.000000000000000000, 0.9510565162951535312, 1.000000000000000000, 0.9510565162951535312, 1.000000000000000000, 0.9510565162951535312, 1.000000000000000000, 0.9510565162951535312, 1.000000000000000000, 0.9510565162951535312, 1.000000000000000000, 0.9510565162951535312, 1.000000000000000000, 0.9510565162951535312, 1.000000000000000000, 0.9510565162951535312, 1.000000000000000000, 0.9510565162951535312, 1.000000000000000000, 0.9510565162951535312, 1.000000000000000000, 0.9510565162951535312, 1.000000000000000000, 0.9510565162951535312, 1.000000000000000000, 0.9510565162951535312, 1.000000000000000000, 0.9510565162951535312, 1.000000000000000000, 0.9510565162951535312, 1.000000000000000000, 0.9510565162951535312, 1.000000000000000000, 0.9510565162951535312, 1.000000000000000000, 0.9510565162951535312, 1.000000000000000000, 0.9510565162951535312, 1.000000000000000000, 0.9510565162951535312, 1.000000000000000000, 0.9510565162951535312, 1.000000000000000000, 0.9510565162951535312, 1.000000000000000000, 0.9510565162951535312, 1.000000000000000000, 0.9510565162951535312, 1.000000000000000000, 0.9510565162951535312, 1.000000000000000000, 0.9510565162951535312, 1.000000000000000000, 0.9510565162951535312, 1.000000000000000000, 0.9510565162951535312, 1.000000000000000000, 0.9510565162951535312, 1.000000000000000000, 0.9510565162951535312, 1.000000000000000000, 0.9510565162951535312, 1.000000000000000000, 0.9510565162951535312, 1.000000000000000000, 0.9510565162951535312, 1.000000000000000000, 0.9510565162951535312, 1.000000000000000000, 0.9510565162951535312, 1.000000000000000000, 0.9510565162951535312, 1.000000000000000000, 0.9510565162951535312, 1.000000000000000000, 0.9510565162951535312, 1.000000000000000000, 0.9510565162951535312, 1.000000000000000000, 0.9510565162951535312, 1.000000000000000000, 0.9510565162951535312, 1.000000000000000000, 0.9510565162951535312, 1.000000000000000000, 0.9510565162951535312, 1.000000000000000000, 0.9510565162951535312, 1.000000000000000000, 0.9510565162951535312, 1.000000000000000000, 0.9510565162951535312, 1.000000000000000000, 0.9510565162951535312, 1.000000000000000000, 0.9510565162951535312, 1.000000000000000000, 0.9510565162951535312, 1.000000000000000000, 0.9510565162951535312, 1.000000000000000000, 0.9510565162951535312, 1.000000000000000000, 0.9510565162951535312, 1.000000000000000000, 0.9510565162951535312, 1.000000000000000000, 0.9510565162951535312, 1.000000000000000000, 0.9510565162951535312, 1.000000000000000000, 0.9510565162951535312, 1.000000000000000000, 0.9510565162951535312, 1.000000000000000000, 0.9510565162951535312, 1.000000000000000000, 0.9510565162951535312, 1.000000000000000000, 0.9510565162951535312, 1.000000000000000000, 0.9510565162951535312, 1.000000000000000000, 0.9510565162951535312, 1.000000000000000000, 0.9510565162951535312, 1.000000000000000000, 0.9510565162951535312, 1.000000000000000000, 0.9510565162951535312, 1.000000000000000000, 0.9510565162951535312, 1.000000000000000000, 0.9510565162951535312, 1.000000000000000000, 0.9510565162951535312, 1.000000000000000000, 0.9510565162951535312, 1.000000000000000000, 0.9510565162951535312, 1.000000000000000000, 0.9510565162951535312, 1.000000000000000000, 0.9510565162951535312, 1.000000000000000000, 0.9510565162951535312, 1.000000000000000000, 0.9510565162951535312, 1.000000000000000000, 0.9510565162951535312, 1.000000000000000000, 0.9510565162951535312, 1.000000000000000000, 0.9510565162951535312, 1.000000000000000000, 0.9510565162951535312, 1.000000000000000000, 0.9510565162951535312, 1.000000000000000000, 0.9510565162951535312, 1.000000000000000000, 0.9510565162951535312, 1.000000000000000000, 0.9510565162951535312, 1.000000000000000000, 0.9510565162951535312, 1.000000000000000000, 0.9510565162951535312, 1.000000000000000000, 0.9510565162951535312, 1.000000000000000000, 0.9510565162951535312, 1.000000000000000000, 0.9510565162951535312, 1.000000000000000000, 0.9510565162951535312, 1.000000000000000000, 0.9510565162951535312, 1.000000000000000000, 0.9510565162951535312, 1.000000000000000000, 0.9510565162951535312, 1.000000000000000000, 0.9510565162951535312, 1.000000000000000000, 0.9510565162951535312, 1.000000000000000000, 0.9510565162951535312, 1.000000000000000000, 0.9510565162951535312, 1.000000000000000000, 0.9510565162951535312, 1.000000000000000000, 0.9510565162951535312, 1.000000000000000000, 0.9510565162951535312, 1.000000000000000000, 0.9510565162951535312, 1.000000000000000000, 0.9510565162951535312, 1.000000000000000000, 0.9510565162951535312, 1.000000000000000000, 0.9510565162951535312, 1.000000000000000000, 0.9510565162951535312, 1.000000000000000000, 0.9510565162951535312, 1.000000000000000000, 0.9510565162951535312, 1.000000000000000000, 0.9510565162951535312, 1.000000000000000000, 0.9510565162951535312, 1.000000000000000000, 0.9510565162951535312, 1.000000000000000000, 0.9510565162951535312, 1.000000000000000000, 0.9510565162951535312, 1.000000000000000000, 0.9510565162951535312, 1.000000000000000000, 0.9510565162951535312, 1.000000000000000000, 0.9510565162951535312, 1.000000000000000000, 0.9510565162951535312, 1.000000000000000000, 0.9510565162951535312, 1.000000000000000000, 0.9510565162951535312, 1.000000000000000000, 0.9510565162951535312, 1.000000000000000000, 0.9510565162951535312, 1.000000000000000000, 0.9510565162951535312, 1.000000000000000000 ) ) 
 REPRESENTATION_ITEM ( '' )  );
#8763=CARTESIAN_POINT ( 'NONE',  ( -20.75514604977248823, 3.075000002731198112, -28.56700777964554305 ) ) ;
#8765=CARTESIAN_POINT ( 'NONE',  ( 10.37757302488624056, 74.77500000273118985, -31.93888565452638417 ) ) ;
#8766=CARTESIAN_POINT ( 'NONE',  ( -7.570916362186215665, 19.14999999453761959, 23.30088464923126423 ) ) ;
#8768=ORIENTED_EDGE ( 'NONE', *, *, #3988, .T. ) ;
#8769=CARTESIAN_POINT ( 'NONE',  ( -24.50000000000001066, 6.849999994537628645, 7.960532557706201828 ) ) ;
#8771=CARTESIAN_POINT ( 'NONE',  ( 15.00000000000000000, 75.09999999999996589, -4.873795443493596835 ) ) ;
#8782=CARTESIAN_POINT ( 'NONE',  ( 7.890940483122900408E-14, 16.49999999999999645, -24.50000000000000000 ) ) ;
#8784=EDGE_CURVE ( 'NONE', #33960, #14496, #6316, .T. ) ;
#8786=DIRECTION ( 'NONE',  ( 0.000000000000000000, 0.000000000000000000, -1.000000000000000000 ) ) ;
#8788=CARTESIAN_POINT ( 'NONE',  ( 33.58253175000000113, 66.47500000273119269, -10.91162601494193751 ) ) ;
#8789=ORIENTED_EDGE ( 'NONE', *, *, #29131, .T. ) ;
#8793=ORIENTED_EDGE ( 'NONE', *, *, #2129, .T. ) ;
#8794=CARTESIAN_POINT ( 'NONE',  ( -33.04126587500000056, 1.687500001365582758, 0.000000000000000000 ) ) ;
#8795=CARTESIAN_POINT ( 'NONE',  ( -10.37757302488624411, 54.72500000273117138, -31.93888565452638417 ) ) ;
#8797=CARTESIAN_POINT ( 'NONE',  ( 20.08610463437157279, 11.80000000546236194, -27.64615127144129758 ) ) ;
#8799=CARTESIAN_POINT ( 'NONE',  ( 7.236395654485760609, 15.52499999726880731, -22.27133577429736633 ) ) ;
#8800=( BOUNDED_CURVE ( )  B_SPLINE_CURVE ( 2, ( #18404, #16490, #19071, #3445, #16166, #32091, #8088, #5516, #29183, #23547, #354, #26283, #10498 ),
 .UNSPECIFIED., .F., .T. ) 
 B_SPLINE_CURVE_WITH_KNOTS ( ( 3, 2, 2, 2, 2, 2, 3 ),
 ( 0.5576923076923077094, 0.5589743589743589869, 0.5615384615384615419, 0.5641025641025640969, 0.5666666666666666519, 0.5692307692307692069, 0.5705128205128204844 ),
 .UNSPECIFIED. ) 
 CURVE ( )  GEOMETRIC_REPRESENTATION_ITEM ( )  RATIONAL_B_SPLINE_CURVE ( ( 0.9755282581475768211, 0.9755282581475768211, 1.000000000000000000, 0.9510565162951535312, 1.000000000000000000, 0.9510565162951535312, 1.000000000000000000, 0.9510565162951535312, 1.000000000000000000, 0.9510565162951535312, 1.000000000000000000, 0.9755282581475768211, 0.9755282581475768211 ) ) 
 REPRESENTATION_ITEM ( '' )  );
#8801=CARTESIAN_POINT ( 'NONE',  ( -10.37757302488624411, 24.97500000273117493, -31.93888565452638417 ) ) ;
#8802=CARTESIAN_POINT ( 'NONE',  ( 4.635254915624212657, 76.59999999999999432, 14.26584774442730286 ) ) ;
#8804=CARTESIAN_POINT ( 'NONE',  ( -5.147494310547640062, 32.44874571845313227, 32.49999999999992895 ) ) ;
#8805=CARTESIAN_POINT ( 'NONE',  ( -10.04305231718578462, 34.39999999999998437, 30.90933677959249337 ) ) ;
#8809=CARTESIAN_POINT ( 'NONE',  ( -4.300734207923755825, 73.27500000273118985, 13.23629886949340673 ) ) ;
#8811=CARTESIAN_POINT ( 'NONE',  ( 33.58253175000000113, 16.12500000273120548, -4.112674001490185761E-15 ) ) ;
#8815=CARTESIAN_POINT ( 'NONE',  ( -20.75514604977248823, 11.07500000273117990, -28.56700777964554305 ) ) ;
#8818=CARTESIAN_POINT ( 'NONE',  ( -15.00000000000000000, 71.12500000273119838, 0.000000000000000000 ) ) ;
#8819=CARTESIAN_POINT ( 'NONE',  ( -11.25946833292375793, 75.17500000273119554, -8.180482586598733619 ) ) ;
#8821=VECTOR ( 'NONE', #28600, 1000.000000000000000 ) ;
#8823=CARTESIAN_POINT ( 'NONE',  ( 33.58253175000000113, 52.12500000273118417, -4.112674001490185761E-15 ) ) ;
#8825=ADVANCED_FACE ( 'NONE', ( #22434 ), #9561, .T. ) ;
#8826=ORIENTED_EDGE ( 'NONE', *, *, #1694, .T. ) ;
#8828=CARTESIAN_POINT ( 'NONE',  ( -10.37757302488623701, 1.525000002731202731, 31.93888565452638417 ) ) ;
#8829=CARTESIAN_POINT ( 'NONE',  ( 14.47279130897151767, 6.924999997268805885, -19.92008829642072598 ) ) ;
#8832=ORIENTED_EDGE ( 'NONE', *, *, #20979, .T. ) ;
#8834=CARTESIAN_POINT ( 'NONE',  ( -26.29305231718578995, 68.70000000546238539, 19.10302069950538595 ) ) ;
#8837=CARTESIAN_POINT ( 'NONE',  ( -20.75514604977248823, 63.07500000273119412, -28.56700777964554305 ) ) ;
#8839=CARTESIAN_POINT ( 'NONE',  ( -27.16883889988624290, 72.92500000273119554, -19.73931689729374028 ) ) ;
#8841=CARTESIAN_POINT ( 'NONE',  ( 19.82091636218621034, 3.799999999999998046, 14.40073868116559730 ) ) ;
#8842=CARTESIAN_POINT ( 'NONE',  ( 0.000000000000000000, 80.00000000000001421, 0.000000000000000000 ) ) ;
#8843=CARTESIAN_POINT ( 'NONE',  ( 27.16883889988624290, 13.92500000273116889, 19.73931689729373673 ) ) ;
#8844=CARTESIAN_POINT ( 'NONE',  ( -11.25946833292375793, 73.07500000273120122, 8.180482586598737171 ) ) ;
#8848=CARTESIAN_POINT ( 'NONE',  ( -9.270509831248421762, 78.29999999999999716, 12.75976212528060039 ) ) ;
#8851=CARTESIAN_POINT ( 'NONE',  ( 32.50000000000000000, 49.50000000546239676, -3.980102097228898626E-15 ) ) ;
#8853=CARTESIAN_POINT ( 'NONE',  ( 20.75514604977249178, 43.82500000273119412, 28.56700777964553950 ) ) ;
#8856=CARTESIAN_POINT ( 'NONE',  ( -27.16883889988623935, 25.57500000273119056, 19.73931689729374739 ) ) ;
#8857=CARTESIAN_POINT ( 'NONE',  ( -14.45873412499999944, 80.56250000409679046, 0.000000000000000000 ) ) ;
#8863=CARTESIAN_POINT ( 'NONE',  ( -23.41746825000000243, 3.724999997268820362, 7.608796670333725309 ) ) ;
#8865=( BOUNDED_CURVE ( )  B_SPLINE_CURVE ( 2, ( #32471, #1065, #32309, #6061, #4166, #25098, #6735, #24428, #12052, #3660, #8802, #6403, #9137 ),
 .UNSPECIFIED., .F., .T. ) 
 B_SPLINE_CURVE_WITH_KNOTS ( ( 3, 2, 2, 2, 2, 2, 3 ),
 ( 0.4500000000000000111, 0.4600000000000000200, 0.4799999999999999822, 0.5000000000000000000, 0.5200000000000000178, 0.5400000000000000355, 0.5500000000000000444 ),
 .UNSPECIFIED. ) 
 CURVE ( )  GEOMETRIC_REPRESENTATION_ITEM ( )  RATIONAL_B_SPLINE_CURVE ( ( 0.9755282581475768211, 0.9755282581475768211, 1.000000000000000000, 0.9510565162951535312, 1.000000000000000000, 0.9510565162951535312, 1.000000000000000000, 0.9510565162951535312, 1.000000000000000000, 0.9510565162951535312, 1.000000000000000000, 0.9755282581475768211, 0.9755282581475768211 ) ) 
 REPRESENTATION_ITEM ( '' )  );
#8866=CARTESIAN_POINT ( 'NONE',  ( 1.555960095263670572E-15, 12.50000000000000355, -24.50000000000000000 ) ) ;
#8869=CARTESIAN_POINT ( 'NONE',  ( 33.58253175000000113, 22.12500000273118062, -4.112674001490185761E-15 ) ) ;
#8870=CARTESIAN_POINT ( 'NONE',  ( 14.47279130897151589, 4.824999997268814234, 19.92008829642072953 ) ) ;
#8872=ORIENTED_EDGE ( 'NONE', *, *, #18822, .F. ) ;
#8878=CARTESIAN_POINT ( 'NONE',  ( -13.91746824999999887, 81.37500000273118417, 0.000000000000000000 ) ) ;
#8879=CARTESIAN_POINT ( 'NONE',  ( 19.82091636218621034, 17.54999999453762882, 14.40073868116559730 ) ) ;
#8880=CARTESIAN_POINT ( 'NONE',  ( 23.41746825000000243, 8.724999997268806595, -7.608796670333727974 ) ) ;
#8881=CARTESIAN_POINT ( 'NONE',  ( 33.58253175000000113, 30.47500000273117493, -10.91162601494193751 ) ) ;
#8882=CARTESIAN_POINT ( 'NONE',  ( 32.50000000000000000, 31.60000000546237686, -10.55989012756945833 ) ) ;
#8883=CARTESIAN_POINT ( 'NONE',  ( -32.50000000000000000, 72.00000000000001421, 0.000000000000000000 ) ) ;
#8885=CARTESIAN_POINT ( 'NONE',  ( 12.13525491562421088, 72.79999999999999716, 8.816778784387095058 ) ) ;
#8887=CARTESIAN_POINT ( 'NONE',  ( 33.58253175000000113, 40.37500000273119838, -4.112674001490185761E-15 ) ) ;
#8888=CARTESIAN_POINT ( 'NONE',  ( -18.94512977948576093, 10.32499999726882400, 13.76444248337722698 ) ) ;
#8889=CARTESIAN_POINT ( 'NONE',  ( 20.08610463437158344, 14.70000000000000107, 27.64615127144129403 ) ) ;
#8893=CARTESIAN_POINT ( 'NONE',  ( 6.486482029760649416E-15, 61.62500000273118417, 35.31076352940723240 ) ) ;
#8894=CARTESIAN_POINT ( 'NONE',  ( -20.75514604977248823, 47.07500000273117280, -28.56700777964554305 ) ) ;
#8897=CARTESIAN_POINT ( 'NONE',  ( 33.58253175000000113, 6.125000002731195714, -4.112674001490185761E-15 ) ) ;
#8903=LINE ( 'NONE', #1167, #25408 ) ;
#8914=CARTESIAN_POINT ( 'NONE',  ( -1.053607264507113999E-13, 64.50000000000000000, 32.50000000000000711 ) ) ;
#8918=EDGE_CURVE ( 'NONE', #33879, #17974, #11963, .T. ) ;
#8920=CARTESIAN_POINT ( 'NONE',  ( -20.08610463437157989, 64.20000000546238539, -27.64615127144129758 ) ) ;
#8921=CARTESIAN_POINT ( 'NONE',  ( 10.37757302488624056, 44.77500000273118275, -31.93888565452638417 ) ) ;
#8922=CARTESIAN_POINT ( 'NONE',  ( -10.04305231718578462, 50.90000000546238113, 30.90933677959249337 ) ) ;
#8924=CARTESIAN_POINT ( 'NONE',  ( -2.162160676586881955E-15, 38.62500000273118417, -35.31076352940723240 ) ) ;
#8926=CARTESIAN_POINT ( 'NONE',  ( -27.16883889988623935, 63.57500000273119412, 19.73931689729374739 ) ) ;
#8928=EDGE_CURVE ( 'NONE', #9120, #10039, #19011, .T. ) ;
#8930=CARTESIAN_POINT ( 'NONE',  ( -26.29305231718579350, 35.79999999999999716, -19.10302069950537884 ) ) ;
#8932=CARTESIAN_POINT ( 'NONE',  ( -20.75514604977248112, 5.675000002731203530, 28.56700777964554661 ) ) ;
#8933=VECTOR ( 'NONE', #12590, 1000.000000000000000 ) ;
#8934=CARTESIAN_POINT ( 'NONE',  ( 1.836970198721029589E-15, 82.00000000000001421, 15.00000000000000000 ) ) ;
#8936=CARTESIAN_POINT ( 'NONE',  ( -33.58253175000000113, 69.47500000273117848, 10.91162601494193929 ) ) ;
#8937=CARTESIAN_POINT ( 'NONE',  ( -7.570916362186215665, 5.399999999999987921, 23.30088464923126423 ) ) ;
#8939=EDGE_CURVE ( 'NONE', #12256, #2384, #9769, .T. ) ;
#8942=CARTESIAN_POINT ( 'NONE',  ( -24.50000000000000355, 6.649999994537636461, -7.960532557706207157 ) ) ;
#8955=CARTESIAN_POINT ( 'NONE',  ( -15.14183272437242778, 5.049999994537627934, 20.84094480462497856 ) ) ;
#8956=VERTEX_POINT ( 'NONE', #24670 ) ;
#8962=ORIENTED_EDGE ( 'NONE', *, *, #5665, .T. ) ;
#8964=CARTESIAN_POINT ( 'NONE',  ( -5.147494310547423346, 74.94874572391552192, 32.50000000000000000 ) ) ;
#8965=CARTESIAN_POINT ( 'NONE',  ( -20.75514604977248823, 54.82500000273118701, -28.56700777964554305 ) ) ;
#8967=CARTESIAN_POINT ( 'NONE',  ( 10.04305231718579705, 11.10000000546237864, 30.90933677959248982 ) ) ;
#8968=LINE ( 'NONE', #26671, #3719 ) ;
#8969=CARTESIAN_POINT ( 'NONE',  ( -23.41746824999999887, 18.12499999726882649, -2.867812753649727150E-15 ) ) ;
#8970=CARTESIAN_POINT ( 'NONE',  ( 20.08610463437158344, 56.69999999999998153, 27.64615127144129403 ) ) ;
#8971=CARTESIAN_POINT ( 'NONE',  ( 20.75514604977249178, 22.07500000273117990, 28.56700777964553950 ) ) ;
#8972=CARTESIAN_POINT ( 'NONE',  ( 26.29305231718579350, 5.300000005462379704, 19.10302069950537529 ) ) ;
#8974=CARTESIAN_POINT ( 'NONE',  ( 13.91746824999999532, 73.97500000273119269, -4.522059556121118540 ) ) ;
#8975=CARTESIAN_POINT ( 'NONE',  ( 7.570916362186207671, 15.60000000000000320, 23.30088464923126779 ) ) ;
#8976=CARTESIAN_POINT ( 'NONE',  ( -5.147494310547430452, 33.55125428154685352, -32.49999999999999289 ) ) ;
#8978=ORIENTED_EDGE ( 'NONE', *, *, #24561, .F. ) ;
#8980=CARTESIAN_POINT ( 'NONE',  ( 2.688165632520823219E-15, 77.37500000273118417, 14.63369212191046387 ) ) ;
#8982=CARTESIAN_POINT ( 'NONE',  ( 20.75514604977249178, 19.82500000273119412, 28.56700777964553950 ) ) ;
#8985=VECTOR ( 'NONE', #12938, 1000.000000000000000 ) ;
#8987=CARTESIAN_POINT ( 'NONE',  ( -33.58253175000000113, 11.47500000273119447, 10.91162601494193929 ) ) ;
#8991=CARTESIAN_POINT ( 'NONE',  ( -11.25946833292375793, 79.17500000273119554, -8.180482586598733619 ) ) ;
#8994=CARTESIAN_POINT ( 'NONE',  ( -20.75514604977248823, 50.82500000273117280, -28.56700777964554305 ) ) ;
#8996=ORIENTED_EDGE ( 'NONE', *, *, #1791, .T. ) ;
#8998=DIRECTION ( 'NONE',  ( 0.000000000000000000, 0.000000000000000000, -1.000000000000000000 ) ) ;
#8999=CARTESIAN_POINT ( 'NONE',  ( -23.41746824999999887, 3.624999997268813168, -2.867812753649727150E-15 ) ) ;
#9001=VERTEX_POINT ( 'NONE', #4412 ) ;
#9003=CARTESIAN_POINT ( 'NONE',  ( 24.50000000000000000, 6.000000000000005329, 0.000000000000000000 ) ) ;
#9007=CARTESIAN_POINT ( 'NONE',  ( -33.58253175000000113, 61.37500000273119127, 0.000000000000000000 ) ) ;
#9009=CARTESIAN_POINT ( 'NONE',  ( 10.37757302488624767, 73.72500000273119269, 31.93888565452638417 ) ) ;
#9011=CARTESIAN_POINT ( 'NONE',  ( 24.50000000000000355, 5.899999999999987921, 7.960532557706212486 ) ) ;
#9012=CARTESIAN_POINT ( 'NONE',  ( -20.75514604977248112, 5.675000002731203530, 28.56700777964554661 ) ) ;
#9013=CARTESIAN_POINT ( 'NONE',  ( -2.162160676586881955E-15, 14.62500000273118239, -35.31076352940723240 ) ) ;
#9015=CARTESIAN_POINT ( 'NONE',  ( -12.13525491562420910, 80.19999999999998863, 8.816778784387098611 ) ) ;
#9017=CARTESIAN_POINT ( 'NONE',  ( -24.50000000000000000, 8.649999994537632020, -7.960532557706207157 ) ) ;
#9021=EDGE_CURVE ( 'NONE', #12035, #969, #1144, .T. ) ;
#9022=CARTESIAN_POINT ( 'NONE',  ( 33.58253175000000113, 40.12500000273119838, -4.112674001490185761E-15 ) ) ;
#9025=CARTESIAN_POINT ( 'NONE',  ( 33.58253175000000113, 30.47500000273117493, -10.91162601494193574 ) ) ;
#9026=CARTESIAN_POINT ( 'NONE',  ( 15.14183272437242067, 17.69999999999999218, 20.84094480462498211 ) ) ;
#9027=EDGE_CURVE ( 'NONE', #16413, #30438, #30773, .T. ) ;
#9029=CARTESIAN_POINT ( 'NONE',  ( -5.147494310547430452, 17.55125428154684641, -32.49999999999999289 ) ) ;
#9030=CARTESIAN_POINT ( 'NONE',  ( 9.270509831248425314, 80.69999999999997442, 12.75976212528059683 ) ) ;
#9033=CARTESIAN_POINT ( 'NONE',  ( -14.47279130897151767, 13.32499999726880624, -19.92008829642072598 ) ) ;
#9035=CARTESIAN_POINT ( 'NONE',  ( 0.000000000000000000, 80.00000000000001421, 0.000000000000000000 ) ) ;
#9037=CARTESIAN_POINT ( 'NONE',  ( 5.779280353836490358E-15, 60.49999999999998579, 32.49999999999999289 ) ) ;
#9038=CARTESIAN_POINT ( 'NONE',  ( -20.75514604977248823, 14.82500000273117813, -28.56700777964554305 ) ) ;
#9039=CARTESIAN_POINT ( 'NONE',  ( 7.236395654485760609, 7.524999997268800200, -22.27133577429736633 ) ) ;
#9044=EDGE_LOOP ( 'NONE', ( #481, #22635, #6478, #9241 ) ) ;
#9048=CARTESIAN_POINT ( 'NONE',  ( 19.82091636218621034, 15.54999999453762705, 14.40073868116559730 ) ) ;
#9049=CARTESIAN_POINT ( 'NONE',  ( -23.41746825000000243, 5.524999997268821517, -7.608796670333730638 ) ) ;
#9050=CARTESIAN_POINT ( 'NONE',  ( -27.16883889988624290, 23.17500000273120619, -19.73931689729374028 ) ) ;
#9051=CARTESIAN_POINT ( 'NONE',  ( 32.50000000000000000, 31.50000000546238255, -3.980102097228898626E-15 ) ) ;
#9052=CARTESIAN_POINT ( 'NONE',  ( -20.08610463437157989, 69.69999999999997442, -27.64615127144129758 ) ) ;
#9053=CARTESIAN_POINT ( 'NONE',  ( -5.147494310547430452, 6.051254287009219190, -32.49999999999999289 ) ) ;
#9054=CARTESIAN_POINT ( 'NONE',  ( -19.82091636218621034, 10.80000000000000426, -14.40073868116559552 ) ) ;
#9056=CARTESIAN_POINT ( 'NONE',  ( 27.16883889988623935, 38.57500000273117280, -19.73931689729374384 ) ) ;
#9059=CARTESIAN_POINT ( 'NONE',  ( 7.236395654485760609, 13.52499999726880553, -22.27133577429736633 ) ) ;
#9060=CARTESIAN_POINT ( 'NONE',  ( -26.29305231718579350, 11.80000000000000426, -19.10302069950537884 ) ) ;
#9063=CARTESIAN_POINT ( 'NONE',  ( -20.75514604977248112, 57.42500000273118843, 28.56700777964554661 ) ) ;
#9064=CARTESIAN_POINT ( 'NONE',  ( -10.37757302488624411, 44.97500000273119269, -31.93888565452638417 ) ) ;
#9066=CARTESIAN_POINT ( 'NONE',  ( -4.405589869732278832E-13, 32.49999999999997868, 32.50000000000000000 ) ) ;
#9067=CARTESIAN_POINT ( 'NONE',  ( -2.162160676586881955E-15, 4.625000002731208149, -35.31076352940723240 ) ) ;
#9073=CARTESIAN_POINT ( 'NONE',  ( 1.093617666956751375E-13, 67.50000000000001421, -32.50000000000000711 ) ) ;
#9075=CARTESIAN_POINT ( 'NONE',  ( -20.08610463437157989, 30.20000000546236407, -27.64615127144129758 ) ) ;
#9078=CARTESIAN_POINT ( 'NONE',  ( 20.75514604977248467, 38.42500000273118133, -28.56700777964554305 ) ) ;
#9083=DIRECTION ( 'NONE',  ( 0.000000000000000000, 0.000000000000000000, -1.000000000000000000 ) ) ;
#9089=CARTESIAN_POINT ( 'NONE',  ( 5.147494310547535257, 57.44874571845315359, -32.49999999999996447 ) ) ;
#9090=CARTESIAN_POINT ( 'NONE',  ( -2.162160676586881955E-15, 42.87500000273119127, -35.31076352940723240 ) ) ;
#9091=CARTESIAN_POINT ( 'NONE',  ( 10.04305231718578817, 49.90000000546238113, -30.90933677959249337 ) ) ;
#9093=CARTESIAN_POINT ( 'NONE',  ( -20.75514604977248823, 30.82500000273119767, -28.56700777964554305 ) ) ;
#9095=CARTESIAN_POINT ( 'NONE',  ( 33.58253175000000113, 56.47500000273116427, -10.91162601494193751 ) ) ;
#9096=SURFACE_STYLE_USAGE ( .BOTH. , #32763 ) ;
#9098=CARTESIAN_POINT ( 'NONE',  ( 26.29305231718578995, 33.20000000000000995, -19.10302069950538240 ) ) ;
#9100=CARTESIAN_POINT ( 'NONE',  ( 33.58253175000000113, 2.475000002731187809, -10.91162601494193751 ) ) ;
#9101=CARTESIAN_POINT ( 'NONE',  ( -26.29305231718578995, 70.70000000546239960, 19.10302069950538595 ) ) ;
#9103=CARTESIAN_POINT ( 'NONE',  ( 33.58253175000000823, 64.27500000273118985, 10.91162601494192685 ) ) ;
#9104=CARTESIAN_POINT ( 'NONE',  ( 19.82091636218621389, 3.949999994537628289, -14.40073868116559197 ) ) ;
#9106=CARTESIAN_POINT ( 'NONE',  ( -4.732186688966233175E-15, 3.249999994537627224, 25.76082449383753925 ) ) ;
#9108=CARTESIAN_POINT ( 'NONE',  ( 12.13525491562420910, 75.19999999999998863, -8.816778784387098611 ) ) ;
#9119=CARTESIAN_POINT ( 'NONE',  ( 5.147494310547643614, 13.94874572391553080, -32.49999999999992895 ) ) ;
#9120=VERTEX_POINT ( 'NONE', #12648 ) ;
#9122=CARTESIAN_POINT ( 'NONE',  ( -32.50000000000000000, 76.10000000000000853, 10.55989012756946366 ) ) ;
#9128=CARTESIAN_POINT ( 'NONE',  ( 4.445600272181915325E-13, 27.50000000000000355, -32.50000000000000000 ) ) ;
#9129=CARTESIAN_POINT ( 'NONE',  ( 33.58253175000000113, 48.12500000273117706, -4.112674001490185761E-15 ) ) ;
#9131=CARTESIAN_POINT ( 'NONE',  ( -20.08610463437156923, 8.800000005462372599, 27.64615127144130113 ) ) ;
#9134=CARTESIAN_POINT ( 'NONE',  ( -18.94512977948575738, 13.92499999726881654, -13.76444248337723231 ) ) ;
#9135=CARTESIAN_POINT ( 'NONE',  ( 32.50000000000000000, 55.09999999999998010, -10.55989012756945833 ) ) ;
#9136=CARTESIAN_POINT ( 'NONE',  ( -33.58253175000000113, 23.47500000273119269, 10.91162601494193929 ) ) ;
#9137=CARTESIAN_POINT ( 'NONE',  ( 2.445080149700053643E-15, 76.49999999999998579, 15.00000000000000000 ) ) ;
#9139=CARTESIAN_POINT ( 'NONE',  ( -4.300734207923759378, 72.47500000273119269, -13.23629886949340495 ) ) ;
#9140=CARTESIAN_POINT ( 'NONE',  ( -20.08610463437156923, 34.29999999999999005, 27.64615127144130113 ) ) ;
#9142=ORIENTED_EDGE ( 'NONE', *, *, #18822, .T. ) ;
#9150=CARTESIAN_POINT ( 'NONE',  ( 33.58253175000000823, 8.275000002731179194, 10.91162601494192685 ) ) ;
#9154=CARTESIAN_POINT ( 'NONE',  ( -13.91746824999999532, 79.27500000273120406, -4.522059556121115875 ) ) ;
#9157=CARTESIAN_POINT ( 'NONE',  ( 10.37757302488624056, 54.52500000273119696, -31.93888565452638417 ) ) ;
#9161=FACE_OUTER_BOUND ( 'NONE', #27698, .T. ) ;
#9162=CARTESIAN_POINT ( 'NONE',  ( -23.41746825000000598, 13.72499999726882258, 7.608796670333726198 ) ) ;
#9169=CARTESIAN_POINT ( 'NONE',  ( 27.16883889988624290, 58.17500000273118133, 19.73931689729373673 ) ) ;
#9170=CARTESIAN_POINT ( 'NONE',  ( 32.50000000000000000, 69.50000000546238255, -3.980102097228898626E-15 ) ) ;
#9171=CARTESIAN_POINT ( 'NONE',  ( -2.162160676586881955E-15, 76.62500000273118417, -35.31076352940723240 ) ) ;
#9173=CARTESIAN_POINT ( 'NONE',  ( 7.570916362186213000, 4.399999999999987033, -23.30088464923126423 ) ) ;
#9174=CARTESIAN_POINT ( 'NONE',  ( -20.75514604977248823, 5.075000002731193227, -28.56700777964554305 ) ) ;
#9175=CARTESIAN_POINT ( 'NONE',  ( 27.16883889988624290, 17.92500000273117422, 19.73931689729373673 ) ) ;
#9176=CARTESIAN_POINT ( 'NONE',  ( 2.688165632520823219E-15, 75.37500000273118417, 14.63369212191046209 ) ) ;
#9178=CARTESIAN_POINT ( 'NONE',  ( -9.657523855033125146E-16, 79.49999999999998579, -15.77193336357400710 ) ) ;
#9180=CARTESIAN_POINT ( 'NONE',  ( -3.880418787951124493, 9.198745712990794132, 24.50000000000000355 ) ) ;
#9182=CARTESIAN_POINT ( 'NONE',  ( 15.00000000000000355, 79.15000000546238823, 4.873795443493592394 ) ) ;
#9184=CARTESIAN_POINT ( 'NONE',  ( 33.58253175000000823, 36.02500000273117564, 10.91162601494192863 ) ) ;
#9187=CARTESIAN_POINT ( 'NONE',  ( -2.162160676586882350E-15, 28.87500000273119838, -35.31076352940722529 ) ) ;
#9192=CARTESIAN_POINT ( 'NONE',  ( 18.94512977948576093, 12.82499999726882578, -13.76444248337722875 ) ) ;
#9197=CARTESIAN_POINT ( 'NONE',  ( -2.162160676586882350E-15, 14.62500000273118239, -35.31076352940722529 ) ) ;
#9198=CARTESIAN_POINT ( 'NONE',  ( -14.47279130897152122, 6.424999997268821872, 19.92008829642072243 ) ) ;
#9200=EDGE_LOOP ( 'NONE', ( #6213, #12162 ) ) ;
#9203=EDGE_CURVE ( 'NONE', #3689, #3815, #8667, .T. ) ;
#9204=ORIENTED_EDGE ( 'NONE', *, *, #1168, .F. ) ;
#9207=CARTESIAN_POINT ( 'NONE',  ( -10.04305231718578462, 72.90000000546237402, 30.90933677959249337 ) ) ;
#9208=CARTESIAN_POINT ( 'NONE',  ( -19.82091636218621389, 16.94999999453761319, 14.40073868116558842 ) ) ;
#9210=CARTESIAN_POINT ( 'NONE',  ( -7.236395654485757944, 5.224999997268803043, -22.27133577429736988 ) ) ;
#9211=CARTESIAN_POINT ( 'NONE',  ( 33.58253175000000823, 22.27500000273116854, 10.91162601494192863 ) ) ;
#9212=CARTESIAN_POINT ( 'NONE',  ( 6.277390505771533514E-15, 27.00000000546237899, 34.17252228774368916 ) ) ;
#9213=CARTESIAN_POINT ( 'NONE',  ( 10.04305231718578817, 75.39999999999999147, -30.90933677959249337 ) ) ;
#9214=CARTESIAN_POINT ( 'NONE',  ( 5.779280353836490358E-15, 7.000000005462371000, 32.49999999999999289 ) ) ;
#9217=CARTESIAN_POINT ( 'NONE',  ( 27.16883889988623935, 36.57500000273117280, -19.73931689729374384 ) ) ;
#9220=CARTESIAN_POINT ( 'NONE',  ( -7.236395654485757944, 11.72499999726880837, -22.27133577429736988 ) ) ;
#9221=CARTESIAN_POINT ( 'NONE',  ( 32.50000000000000000, 15.00000000000001421, -3.980102097228898626E-15 ) ) ;
#9222=CARTESIAN_POINT ( 'NONE',  ( -32.50000000000000000, 51.89999999999998437, -10.55989012756945300 ) ) ;
#9224=CARTESIAN_POINT ( 'NONE',  ( -27.16883889988624290, 56.92500000273120975, -19.73931689729374028 ) ) ;
#9225=CARTESIAN_POINT ( 'NONE',  ( 27.16883889988624290, 50.17500000273117422, 19.73931689729373673 ) ) ;
#9227=CARTESIAN_POINT ( 'NONE',  ( -1.778240108872766143E-15, 37.50000000000000000, -32.49999999999999289 ) ) ;
#9228=CARTESIAN_POINT ( 'NONE',  ( -26.29305231718579350, 5.799999999999999822, -19.10302069950537884 ) ) ;
#9231=CARTESIAN_POINT ( 'NONE',  ( 15.14183272437242422, 4.300000000000009592, -20.84094480462497856 ) ) ;
#9233=FACE_OUTER_BOUND ( 'NONE', #7098, .T. ) ;
#9239=CARTESIAN_POINT ( 'NONE',  ( 6.486482029760648627E-15, 29.62500000273120193, 35.31076352940722529 ) ) ;
#9241=ORIENTED_EDGE ( 'NONE', *, *, #26475, .F. ) ;
#9249=EDGE_CURVE ( 'NONE', #12166, #11992, #14383, .T. ) ;
#9251=CARTESIAN_POINT ( 'NONE',  ( 2.205017735002230837E-13, 57.49999999999999289, -32.50000000000000000 ) ) ;
#9252=CARTESIAN_POINT ( 'NONE',  ( 20.75514604977249178, 40.07500000273118701, 28.56700777964553950 ) ) ;
#9253=CARTESIAN_POINT ( 'NONE',  ( 32.50000000000000711, 47.40000000546237402, 10.55989012756945122 ) ) ;
#9255=CARTESIAN_POINT ( 'NONE',  ( 27.16883889988624290, 27.92500000273118133, 19.73931689729373673 ) ) ;
#9256=CARTESIAN_POINT ( 'NONE',  ( 10.04305231718578817, 31.90000000546239178, -30.90933677959249337 ) ) ;
#9257=CARTESIAN_POINT ( 'NONE',  ( 10.37757302488624056, 56.77500000273119696, -31.93888565452638417 ) ) ;
#9258=( LENGTH_UNIT ( ) NAMED_UNIT ( * ) SI_UNIT ( .MILLI., .METRE. ) );
#9260=CARTESIAN_POINT ( 'NONE',  ( -2.092463501923844636E-15, 35.49999999999998579, -34.17252228774368916 ) ) ;
#9262=CARTESIAN_POINT ( 'NONE',  ( -27.16883889988624290, 72.92500000273119554, -19.73931689729374028 ) ) ;
#9263=CARTESIAN_POINT ( 'NONE',  ( -10.04305231718578462, 70.90000000546237402, 30.90933677959249337 ) ) ;
#9264=CARTESIAN_POINT ( 'NONE',  ( 0.000000000000000000, 0.000000000000000000, 0.000000000000000000 ) ) ;
#9265=CARTESIAN_POINT ( 'NONE',  ( 20.75514604977249178, 64.07500000273120122, 28.56700777964553950 ) ) ;
#9268=CARTESIAN_POINT ( 'NONE',  ( -19.82091636218621389, 4.949999994537629178, 14.40073868116558842 ) ) ;
#9270=CARTESIAN_POINT ( 'NONE',  ( 5.779280353836490358E-15, 26.50000000000000711, 32.49999999999999289 ) ) ;
#9281=CARTESIAN_POINT ( 'NONE',  ( -24.50000000000000000, 4.749999994537623671, -3.000384657911015469E-15 ) ) ;
#9282=EDGE_LOOP ( 'NONE', ( #6475, #1071, #6971, #11527 ) ) ;
#9286=ORIENTED_EDGE ( 'NONE', *, *, #8451, .T. ) ;
#9288=ORIENTED_EDGE ( 'NONE', *, *, #16371, .T. ) ;
#9289=CARTESIAN_POINT ( 'NONE',  ( 32.50000000000000000, 26.99999999999999645, -3.980102097228898626E-15 ) ) ;
#9290=CARTESIAN_POINT ( 'NONE',  ( 33.58253175000000823, 48.02500000273119696, 10.91162601494192863 ) ) ;
#9292=CARTESIAN_POINT ( 'NONE',  ( -32.50000000000000000, 14.60000000546239107, 10.55989012756946366 ) ) ;
#9293=CARTESIAN_POINT ( 'NONE',  ( -12.13525491562420910, 78.19999999999998863, 8.816778784387098611 ) ) ;
#9294=CARTESIAN_POINT ( 'NONE',  ( 7.236395654485755280, 16.72499999726881370, 22.27133577429736988 ) ) ;
#9295=CARTESIAN_POINT ( 'NONE',  ( -26.29305231718579350, 53.80000000000001137, -19.10302069950537884 ) ) ;
#9296=CARTESIAN_POINT ( 'NONE',  ( 3.980102097228898626E-15, 80.00000000000001421, 32.50000000000000000 ) ) ;
#9297=CARTESIAN_POINT ( 'NONE',  ( 27.16883889988624290, 16.17500000273119909, 19.73931689729373673 ) ) ;
#9298=CARTESIAN_POINT ( 'NONE',  ( 32.50000000000000711, 5.400000005462390895, 10.55989012756945122 ) ) ;
#9300=CARTESIAN_POINT ( 'NONE',  ( 8.601468415847520532, 73.57500000273117280, 11.83890561707634781 ) ) ;
#9301=CARTESIAN_POINT ( 'NONE',  ( 0.000000000000000000, 0.000000000000000000, 0.000000000000000000 ) ) ;
#9311=CARTESIAN_POINT ( 'NONE',  ( 10.37757302488624767, 7.975000002731186477, 31.93888565452638417 ) ) ;
#9314=CARTESIAN_POINT ( 'NONE',  ( 26.29305231718579350, 2.799999999999997158, 19.10302069950537529 ) ) ;
#9316=CARTESIAN_POINT ( 'NONE',  ( -19.82091636218621389, 2.949999994537627401, 14.40073868116558842 ) ) ;
#9317=CARTESIAN_POINT ( 'NONE',  ( -27.16883889988623935, 53.32500000273118701, 19.73931689729374739 ) ) ;
#9319=VERTEX_POINT ( 'NONE', #2175 ) ;
#9321=CYLINDRICAL_SURFACE ( 'NONE', #4769, 32.50000000000000000 ) ;
#9322=CARTESIAN_POINT ( 'NONE',  ( -7.236395654485763274, 14.02499999726880553, 22.27133577429736633 ) ) ;
#9325=ORIENTED_EDGE ( 'NONE', *, *, #25677, .F. ) ;
#9327=LINE ( 'NONE', #11744, #14319 ) ;
#9328=VERTEX_POINT ( 'NONE', #15753 ) ;
#9330=CARTESIAN_POINT ( 'NONE',  ( -27.16883889988624290, 63.17500000273118843, -19.73931689729374028 ) ) ;
#9331=CARTESIAN_POINT ( 'NONE',  ( 0.000000000000000000, 82.00000000000001421, -32.50000000000000000 ) ) ;
#9332=CARTESIAN_POINT ( 'NONE',  ( -10.37757302488624411, 70.72500000273119269, -31.93888565452638417 ) ) ;
#9334=EDGE_CURVE ( 'NONE', #20206, #4188, #344, .T. ) ;
#9335=CARTESIAN_POINT ( 'NONE',  ( -19.82091636218621034, 10.80000000000000426, -14.40073868116559552 ) ) ;
#9336=CARTESIAN_POINT ( 'NONE',  ( 20.75514604977248467, 2.675000002731181770, -28.56700777964554305 ) ) ;
#9337=CARTESIAN_POINT ( 'NONE',  ( 27.16883889988623935, 12.32500000273117990, -19.73931689729374384 ) ) ;
#9338=CARTESIAN_POINT ( 'NONE',  ( -32.50000000000000000, 0.5000000054623809920, 0.000000000000000000 ) ) ;
#9340=CARTESIAN_POINT ( 'NONE',  ( 12.13525491562421088, 80.79999999999998295, 8.816778784387095058 ) ) ;
#9342=EDGE_CURVE ( 'NONE', #21143, #12035, #7365, .T. ) ;
#9343=EDGE_CURVE ( 'NONE', #29552, #19947, #19204, .T. ) ;
#9346=CARTESIAN_POINT ( 'NONE',  ( 12.13525491562421088, 79.05000000546236549, 8.816778784387095058 ) ) ;
#9348=CARTESIAN_POINT ( 'NONE',  ( -27.16883889988623935, 35.32500000273120122, 19.73931689729374739 ) ) ;
#9350=VECTOR ( 'NONE', #11885, 1000.000000000000000 ) ;
#9352=CARTESIAN_POINT ( 'NONE',  ( -2.162160676586882350E-15, 30.87500000273119483, -35.31076352940722529 ) ) ;
#9353=CARTESIAN_POINT ( 'NONE',  ( -32.50000000000000000, 68.09999999999996589, 10.55989012756946366 ) ) ;
#9358=CARTESIAN_POINT ( 'NONE',  ( 1.507698388325705758E-15, 13.12499999726881228, -24.62258325217400312 ) ) ;
#9363=CARTESIAN_POINT ( 'NONE',  ( 33.58253175000000113, 10.22500000273117671, -10.91162601494193574 ) ) ;
#9364=CARTESIAN_POINT ( 'NONE',  ( 14.47279130897151589, 14.82499999726881690, 19.92008829642072953 ) ) ;
#9373=VECTOR ( 'NONE', #3362, 1000.000000000000000 ) ;
#9375=CARTESIAN_POINT ( 'NONE',  ( 24.50000000000000355, 13.64999999453761781, 7.960532557706212486 ) ) ;
#9376=CARTESIAN_POINT ( 'NONE',  ( -7.236395654485757944, 15.22499999726881192, -22.27133577429736988 ) ) ;
#9377=CARTESIAN_POINT ( 'NONE',  ( 33.58253175000000113, 20.47500000273120335, -10.91162601494193751 ) ) ;
#9378=CARTESIAN_POINT ( 'NONE',  ( 32.50000000000000000, 25.60000000546239107, -10.55989012756945833 ) ) ;
#9379=CARTESIAN_POINT ( 'NONE',  ( -10.04305231718578462, 70.40000000000001990, 30.90933677959249337 ) ) ;
#9380=CARTESIAN_POINT ( 'NONE',  ( -20.08610463437156923, 6.800000005462376151, 27.64615127144130113 ) ) ;
#9383=CARTESIAN_POINT ( 'NONE',  ( -2.162160676586881955E-15, 36.87500000273116996, -35.31076352940723240 ) ) ;
#9386=CARTESIAN_POINT ( 'NONE',  ( -18.94512977948576093, 12.32499999726882578, 13.76444248337722698 ) ) ;
#9387=CARTESIAN_POINT ( 'NONE',  ( 32.50000000000000000, 15.09999999999998899, -10.55989012756945833 ) ) ;
#9388=CARTESIAN_POINT ( 'NONE',  ( 5.147494310547426899, 9.948745723915520145, -32.50000000000000000 ) ) ;
#9390=CARTESIAN_POINT ( 'NONE',  ( 27.16883889988623935, 58.32500000273119412, -19.73931689729374384 ) ) ;
#9391=CARTESIAN_POINT ( 'NONE',  ( 10.37757302488624056, 48.77500000273118985, -31.93888565452638417 ) ) ;
#9392=CARTESIAN_POINT ( 'NONE',  ( 26.29305231718578995, 45.19999999999998863, -19.10302069950538240 ) ) ;
#9394=CARTESIAN_POINT ( 'NONE',  ( 10.37757302488624767, 1.725000002731180704, 31.93888565452638417 ) ) ;
#9396=EDGE_CURVE ( 'NONE', #30438, #16413, #33522, .T. ) ;
#9398=CARTESIAN_POINT ( 'NONE',  ( 24.50000000000000000, 4.000000000000003553, 0.000000000000000000 ) ) ;
#9403=CARTESIAN_POINT ( 'NONE',  ( 10.04305231718578817, 41.90000000546237402, -30.90933677959249337 ) ) ;
#9406=CARTESIAN_POINT ( 'NONE',  ( 10.04305231718578817, 35.39999999999998437, -30.90933677959249337 ) ) ;
#9407=CARTESIAN_POINT ( 'NONE',  ( 20.75514604977248467, 32.42500000273117422, -28.56700777964554305 ) ) ;
#9408=CARTESIAN_POINT ( 'NONE',  ( -27.16883889988624290, 65.17500000273118133, -19.73931689729374028 ) ) ;
#9410=EDGE_LOOP ( 'NONE', ( #13092, #5537, #8165, #3241 ) ) ;
#9413=CARTESIAN_POINT ( 'NONE',  ( 0.000000000000000000, 82.00000000000001421, 0.000000000000000000 ) ) ;
#9419=CYLINDRICAL_SURFACE ( 'NONE', #27255, 32.50000000000000000 ) ;
#9420=CARTESIAN_POINT ( 'NONE',  ( -27.16883889988623935, 39.57500000273117280, 19.73931689729374739 ) ) ;
#9421=CARTESIAN_POINT ( 'NONE',  ( -20.08610463437156923, 40.80000000546237260, 27.64615127144130113 ) ) ;
#9423=CARTESIAN_POINT ( 'NONE',  ( 20.75514604977248467, 26.42500000273118843, -28.56700777964554305 ) ) ;
#9424=CARTESIAN_POINT ( 'NONE',  ( 19.82091636218621389, 13.94999999453763806, -14.40073868116559197 ) ) ;
#9425=CARTESIAN_POINT ( 'NONE',  ( -20.75514604977248112, 57.67500000273118133, 28.56700777964554661 ) ) ;
#9428=CARTESIAN_POINT ( 'NONE',  ( 6.277390505771533514E-15, 34.49999999999998579, 34.17252228774368916 ) ) ;
#9430=CARTESIAN_POINT ( 'NONE',  ( -33.58253175000000113, 75.12500000273119838, 0.000000000000000000 ) ) ;
#9434=CARTESIAN_POINT ( 'NONE',  ( -33.58253175000000113, 67.37500000273119838, 0.000000000000000000 ) ) ;
#9436=CARTESIAN_POINT ( 'NONE',  ( -20.08610463437156923, 40.80000000546237260, 27.64615127144130113 ) ) ;
#9437=CARTESIAN_POINT ( 'NONE',  ( 15.14183272437242245, 4.049999994537630599, -20.84094480462497856 ) ) ;
#9439=EDGE_CURVE ( 'NONE', #27031, #22725, #18109, .T. ) ;
#9440=CARTESIAN_POINT ( 'NONE',  ( 1.555960095263670572E-15, 8.249999994537619230, -24.50000000000000000 ) ) ;
#9448=CIRCLE ( 'NONE', #16601, 15.00000000000000000 ) ;
#9453=CARTESIAN_POINT ( 'NONE',  ( -26.29305231718579350, 57.80000000000001847, -19.10302069950537884 ) ) ;
#9454=CARTESIAN_POINT ( 'NONE',  ( 10.04305231718578817, 73.90000000546237402, -30.90933677959249337 ) ) ;
#9457=( BOUNDED_CURVE ( )  B_SPLINE_CURVE ( 2, ( #860, #11340, #19909, #15107, #6860, #27972, #25051, #30877, #30358, #6689, #12006, #4455, #14932 ),
 .UNSPECIFIED., .F., .T. ) 
 B_SPLINE_CURVE_WITH_KNOTS ( ( 3, 2, 2, 2, 2, 2, 3 ),
 ( 0.7115384615384615641, 0.7128205128205128416, 0.7153846153846153966, 0.7179487179487179516, 0.7205128205128205066, 0.7230769230769230616, 0.7243589743589743390 ),
 .UNSPECIFIED. ) 
 CURVE ( )  GEOMETRIC_REPRESENTATION_ITEM ( )  RATIONAL_B_SPLINE_CURVE ( ( 0.9755282581475768211, 0.9755282581475768211, 1.000000000000000000, 0.9510565162951535312, 1.000000000000000000, 0.9510565162951535312, 1.000000000000000000, 0.9510565162951535312, 1.000000000000000000, 0.9510565162951535312, 1.000000000000000000, 0.9755282581475768211, 0.9755282581475768211 ) ) 
 REPRESENTATION_ITEM ( '' )  );
#9458=DIRECTION ( 'NONE',  ( -0.000000000000000000, -1.000000000000000000, -0.000000000000000000 ) ) ;
#9459=VERTEX_POINT ( 'NONE', #9693 ) ;
#9463=CARTESIAN_POINT ( 'NONE',  ( -32.50000000000000000, 62.60000000546238397, 10.55989012756946366 ) ) ;
#9465=AXIS2_PLACEMENT_3D ( 'NONE', #7525, #121, #10613 ) ;
#9467=CARTESIAN_POINT ( 'NONE',  ( 10.37757302488624056, 46.52500000273118985, -31.93888565452638417 ) ) ;
#9468=CARTESIAN_POINT ( 'NONE',  ( -7.236395654485763274, 16.02499999726880731, 22.27133577429736633 ) ) ;
#9469=CARTESIAN_POINT ( 'NONE',  ( -5.147494310547430452, 47.55125428154683220, -32.49999999999999289 ) ) ;
#9470=CARTESIAN_POINT ( 'NONE',  ( -2.092463501923844636E-15, 10.00000000546236301, -34.17252228774368916 ) ) ;
#9473=CARTESIAN_POINT ( 'NONE',  ( -14.47279130897151767, 13.82499999726882045, -19.92008829642072598 ) ) ;
#9474=CARTESIAN_POINT ( 'NONE',  ( -32.50000000000000000, 53.90000000000001279, -10.55989012756945478 ) ) ;
#9475=CARTESIAN_POINT ( 'NONE',  ( -5.147494310547430452, 13.55125428154684997, -32.49999999999999289 ) ) ;
#9476=CARTESIAN_POINT ( 'NONE',  ( -33.58253175000000113, 17.27500000273118630, -10.91162601494193218 ) ) ;
#9477=CARTESIAN_POINT ( 'NONE',  ( 3.980102097228898626E-15, 80.00000000000001421, 32.50000000000000000 ) ) ;
#9479=CARTESIAN_POINT ( 'NONE',  ( 13.91746825000000065, 73.77500000273118985, 4.522059556121114987 ) ) ;
#9480=DIRECTION ( 'NONE',  ( -0.000000000000000000, 1.000000000000000000, -0.000000000000000000 ) ) ;
#9485=CARTESIAN_POINT ( 'NONE',  ( 4.300734207923761154, 71.47500000273119269, 13.23629886949340495 ) ) ;
#9490=CARTESIAN_POINT ( 'NONE',  ( 20.75514604977248467, 4.675000002731176885, -28.56700777964554305 ) ) ;
#9492=EDGE_CURVE ( 'NONE', #23750, #26696, #21613, .T. ) ;
#9495=CARTESIAN_POINT ( 'NONE',  ( -1.778240108872766143E-15, 69.49999999999998579, -32.49999999999999289 ) ) ;
#9497=CARTESIAN_POINT ( 'NONE',  ( 10.37757302488624767, 53.72500000273117138, 31.93888565452638417 ) ) ;
#9498=VECTOR ( 'NONE', #10652, 1000.000000000000000 ) ;
#9503=CARTESIAN_POINT ( 'NONE',  ( 26.29305231718579350, 16.79999999999998295, 19.10302069950537529 ) ) ;
#9504=CARTESIAN_POINT ( 'NONE',  ( 14.47279130897151767, 10.92499999726882365, -19.92008829642072598 ) ) ;
#9506=ORIENTED_EDGE ( 'NONE', *, *, #14686, .F. ) ;
#9508=CARTESIAN_POINT ( 'NONE',  ( 3.445340210940985210E-14, 5.499999999999997335, 24.50000000000000000 ) ) ;
#9509=ORIENTED_EDGE ( 'NONE', *, *, #22859, .T. ) ;
#9511=CARTESIAN_POINT ( 'NONE',  ( -2.162160676586881955E-15, 62.87500000273120548, -35.31076352940723240 ) ) ;
#9512=LINE ( 'NONE', #14502, #30263 ) ;
#9513=CARTESIAN_POINT ( 'NONE',  ( 27.16883889988623935, 70.32500000273117280, -19.73931689729374384 ) ) ;
#9515=CARTESIAN_POINT ( 'NONE',  ( 15.14183272437242245, 14.29999999999998472, -20.84094480462497856 ) ) ;
#9517=CARTESIAN_POINT ( 'NONE',  ( 20.75514604977248467, 10.42500000273120087, -28.56700777964554305 ) ) ;
#9518=CARTESIAN_POINT ( 'NONE',  ( 0.000000000000000000, 70.00000000000000000, 0.000000000000000000 ) ) ;
#9520=CARTESIAN_POINT ( 'NONE',  ( 12.13525491562420910, 75.19999999999998863, -8.816778784387098611 ) ) ;
#9521=VECTOR ( 'NONE', #14395, 1000.000000000000000 ) ;
#9524=CARTESIAN_POINT ( 'NONE',  ( 26.29305231718578995, 61.70000000546238539, -19.10302069950538240 ) ) ;
#9526=CARTESIAN_POINT ( 'NONE',  ( -9.657523855033125146E-16, 75.75000000546238255, -15.77193336357400710 ) ) ;
#9528=CARTESIAN_POINT ( 'NONE',  ( 27.16883889988623935, 38.32500000273120122, -19.73931689729374384 ) ) ;
#9531=CARTESIAN_POINT ( 'NONE',  ( -27.16883889988624290, 23.17500000273120619, -19.73931689729374028 ) ) ;
#9532=CARTESIAN_POINT ( 'NONE',  ( 5.147494310547434893, 40.55125428154684641, 32.49999999999999289 ) ) ;
#9534=CARTESIAN_POINT ( 'NONE',  ( -1.778240108872766143E-15, 33.50000000000000000, -32.49999999999999289 ) ) ;
#9536=CARTESIAN_POINT ( 'NONE',  ( -18.94512977948575738, 11.42499999726881477, -13.76444248337723231 ) ) ;
#9541=DIRECTION ( 'NONE',  ( -0.000000000000000000, -1.000000000000000000, -0.000000000000000000 ) ) ;
#9542=CARTESIAN_POINT ( 'NONE',  ( -33.58253175000000113, 15.22500000273119269, 10.91162601494193929 ) ) ;
#9543=CARTESIAN_POINT ( 'NONE',  ( 18.94512977948576093, 15.32499999726882933, -13.76444248337722875 ) ) ;
#9549=ORIENTED_EDGE ( 'NONE', *, *, #26976, .T. ) ;
#9554=CARTESIAN_POINT ( 'NONE',  ( -15.14183272437241889, 18.44999999453760964, -20.84094480462497856 ) ) ;
#9555=EDGE_CURVE ( 'NONE', #2565, #19940, #13472, .T. ) ;
#9556=CARTESIAN_POINT ( 'NONE',  ( -18.94512977948576093, 11.82499999726882578, 13.76444248337722698 ) ) ;
#9557=PRODUCT ( 'primary mounting nut', 'primary mounting nut', '', ( #20743 ) ) ;
#9558=CARTESIAN_POINT ( 'NONE',  ( 20.75514604977249178, 24.07500000273120122, 28.56700777964553950 ) ) ;
#9559=CARTESIAN_POINT ( 'NONE',  ( -10.04305231718579172, 26.10000000546236620, -30.90933677959248982 ) ) ;
#9560=CARTESIAN_POINT ( 'NONE',  ( -20.08610463437156923, 66.30000000000001137, 27.64615127144130113 ) ) ;
#9561=CYLINDRICAL_SURFACE ( 'NONE', #22012, 32.50000000000000000 ) ;
#9564=CARTESIAN_POINT ( 'NONE',  ( 20.75514604977249178, 38.07500000273116569, 28.56700777964553950 ) ) ;
#9567=EDGE_CURVE ( 'NONE', #33751, #12166, #31914, .T. ) ;
#9568=CARTESIAN_POINT ( 'NONE',  ( -4.523095164977116484E-15, 18.62499999726881583, 24.62258325217400312 ) ) ;
#9569=CARTESIAN_POINT ( 'NONE',  ( -26.29305231718578995, 16.19999999999999218, 19.10302069950538595 ) ) ;
#9570=CARTESIAN_POINT ( 'NONE',  ( -10.04305231718579172, 51.60000000000000853, -30.90933677959248982 ) ) ;
#9572=( BOUNDED_CURVE ( )  B_SPLINE_CURVE ( 2, ( #28232, #15024, #1972, #12447, #4718, #15198, #15546, #10896, #15718, #10724, #2491, #26173, #239 ),
 .UNSPECIFIED., .F., .T. ) 
 B_SPLINE_CURVE_WITH_KNOTS ( ( 3, 2, 2, 2, 2, 2, 3 ),
 ( 0.1217948717948718063, 0.1230769230769230838, 0.1256410256410256387, 0.1282051282051281937, 0.1307692307692307765, 0.1333333333333333315, 0.1346153846153846090 ),
 .UNSPECIFIED. ) 
 CURVE ( )  GEOMETRIC_REPRESENTATION_ITEM ( )  RATIONAL_B_SPLINE_CURVE ( ( 0.9755282581475767101, 0.9755282581475768211, 1.000000000000000000, 0.9510565162951535312, 1.000000000000000000, 0.9510565162951535312, 1.000000000000000000, 0.9510565162951535312, 1.000000000000000000, 0.9510565162951535312, 1.000000000000000000, 0.9755282581475768211, 0.9755282581475768211 ) ) 
 REPRESENTATION_ITEM ( '' )  );
#9573=CARTESIAN_POINT ( 'NONE',  ( -33.58253175000000113, 59.22500000273119269, 10.91162601494193929 ) ) ;
#9575=CARTESIAN_POINT ( 'NONE',  ( 33.58253175000000823, 46.27500000273120406, 10.91162601494192685 ) ) ;
#9576=CARTESIAN_POINT ( 'NONE',  ( 5.147494310547434893, 44.55125428154684641, 32.49999999999999289 ) ) ;
#9577=CARTESIAN_POINT ( 'NONE',  ( 5.779280353836490358E-15, 67.00000000546236834, 32.49999999999999289 ) ) ;
#9578=CARTESIAN_POINT ( 'NONE',  ( -32.50000000000000000, 50.09999999999998721, 10.55989012756946366 ) ) ;
#9581=CARTESIAN_POINT ( 'NONE',  ( -26.29305231718579350, 41.80000000000000426, -19.10302069950537884 ) ) ;
#9583=DIRECTION ( 'NONE',  ( 0.000000000000000000, 0.000000000000000000, -1.000000000000000000 ) ) ;
#9588=CARTESIAN_POINT ( 'NONE',  ( 10.37757302488624056, 34.52500000273117564, -31.93888565452638417 ) ) ;
#9595=VERTEX_POINT ( 'NONE', #62 ) ;
#9600=CARTESIAN_POINT ( 'NONE',  ( -5.147494310547531704, 46.44874571845316780, 32.49999999999996447 ) ) ;
#9601=CARTESIAN_POINT ( 'NONE',  ( 33.58253175000000823, 42.27500000273118275, 10.91162601494192863 ) ) ;
#9602=CARTESIAN_POINT ( 'NONE',  ( 20.08610463437158344, 45.20000000546239249, 27.64615127144129403 ) ) ;
#9604=CARTESIAN_POINT ( 'NONE',  ( -10.37757302488623701, 31.52500000273117564, 31.93888565452638417 ) ) ;
#9605=CARTESIAN_POINT ( 'NONE',  ( 15.14183272437242422, 14.04999999453763593, -20.84094480462497856 ) ) ;
#9606=CARTESIAN_POINT ( 'NONE',  ( 27.16883889988623935, 52.57500000273118701, -19.73931689729374384 ) ) ;
#9609=CARTESIAN_POINT ( 'NONE',  ( 10.04305231718579705, 36.59999999999999432, 30.90933677959248982 ) ) ;
#9611=CARTESIAN_POINT ( 'NONE',  ( 33.58253175000000113, 76.12500000273119838, -4.112674001490185761E-15 ) ) ;
#9613=CARTESIAN_POINT ( 'NONE',  ( -27.16883889988624290, 67.17500000273119554, -19.73931689729374028 ) ) ;
#9616=CARTESIAN_POINT ( 'NONE',  ( 20.75514604977248467, 16.42500000273118133, -28.56700777964554305 ) ) ;
#9617=CARTESIAN_POINT ( 'NONE',  ( -19.82091636218621389, 10.94999999453763451, 14.40073868116558842 ) ) ;
#9628=AXIS2_PLACEMENT_3D ( 'NONE', #6535, #27298, #19082 ) ;
#9630=CARTESIAN_POINT ( 'NONE',  ( 3.980102097228898626E-15, 80.00000000000001421, 32.50000000000000000 ) ) ;
#9631=CARTESIAN_POINT ( 'NONE',  ( -32.50000000000000000, 76.60000000546239107, 10.55989012756946366 ) ) ;
#9635=EDGE_LOOP ( 'NONE', ( #29393, #11737, #4444, #12558 ) ) ;
#9636=CARTESIAN_POINT ( 'NONE',  ( -10.37757302488623701, 71.77500000273117564, 31.93888565452638417 ) ) ;
#9638=ORIENTED_EDGE ( 'NONE', *, *, #1940, .F. ) ;
#9640=CARTESIAN_POINT ( 'NONE',  ( 10.04305231718578817, 63.90000000546236691, -30.90933677959249337 ) ) ;
#9642=ORIENTED_EDGE ( 'NONE', *, *, #18618, .T. ) ;
#9644=CARTESIAN_POINT ( 'NONE',  ( -20.75514604977248112, 45.42500000273119554, 28.56700777964554661 ) ) ;
#9645=CARTESIAN_POINT ( 'NONE',  ( -8.891200544363830713E-16, 73.75000000546239676, -15.00000000000000000 ) ) ;
#9648=CARTESIAN_POINT ( 'NONE',  ( -26.29305231718579350, 2.300000005462377040, -19.10302069950537884 ) ) ;
#9650=LINE ( 'NONE', #31096, #13342 ) ;
#9651=CARTESIAN_POINT ( 'NONE',  ( 20.08610463437158344, 50.69999999999999574, 27.64615127144129403 ) ) ;
#9652=CARTESIAN_POINT ( 'NONE',  ( -10.04305231718578462, 14.39999999999999680, 30.90933677959249337 ) ) ;
#9653=CARTESIAN_POINT ( 'NONE',  ( -33.58253175000000113, 17.37500000273117706, 0.000000000000000000 ) ) ;
#9654=CARTESIAN_POINT ( 'NONE',  ( -5.147494310547430452, 24.05125428700921830, -32.49999999999999289 ) ) ;
#9656=CARTESIAN_POINT ( 'NONE',  ( -11.25946833292375793, 77.57500000273121543, 8.180482586598737171 ) ) ;
#9658=CARTESIAN_POINT ( 'NONE',  ( 5.147494310547426899, 53.94874572391552192, -32.50000000000000000 ) ) ;
#9660=ORIENTED_EDGE ( 'NONE', *, *, #20647, .F. ) ;
#9662=CARTESIAN_POINT ( 'NONE',  ( 5.334720326618300005E-14, 72.00000000546238255, -32.50000000000000000 ) ) ;
#9667=CARTESIAN_POINT ( 'NONE',  ( 6.486482029760648627E-15, 1.875000002731177950, 35.31076352940722529 ) ) ;
#9671=( BOUNDED_CURVE ( )  B_SPLINE_CURVE ( 2, ( #18241, #5009, #15, #15492, #2615, #33845, #5185 ),
 .UNSPECIFIED., .F., .T. ) 
 B_SPLINE_CURVE_WITH_KNOTS ( ( 3, 2, 2, 3 ),
 ( 0.9499999999999999556, 0.9599999999999999645, 0.9799999999999999822, 1.000000000000000000 ),
 .UNSPECIFIED. ) 
 CURVE ( )  GEOMETRIC_REPRESENTATION_ITEM ( )  RATIONAL_B_SPLINE_CURVE ( ( 0.9755282581475768211, 0.9755282581475768211, 1.000000000000000000, 0.9510565162951535312, 1.000000000000000000, 0.9510565162951535312, 1.000000000000000000 ) ) 
 REPRESENTATION_ITEM ( '' )  );
#9672=CARTESIAN_POINT ( 'NONE',  ( 2.688165632520823219E-15, 73.87500000273119838, 14.63369212191046209 ) ) ;
#9674=CARTESIAN_POINT ( 'NONE',  ( -33.58253175000000113, 43.12500000273116996, 0.000000000000000000 ) ) ;
#9678=DIRECTION ( 'NONE',  ( 0.000000000000000000, 0.000000000000000000, -1.000000000000000000 ) ) ;
#9679=CARTESIAN_POINT ( 'NONE',  ( 18.94512977948575738, 12.42499999726881477, 13.76444248337723408 ) ) ;
#9684=CARTESIAN_POINT ( 'NONE',  ( -20.08610463437157989, 34.20000000546237828, -27.64615127144129758 ) ) ;
#9687=CARTESIAN_POINT ( 'NONE',  ( -4.934616302121927505E-14, 69.00000000546236834, 32.50000000000000000 ) ) ;
#9688=CARTESIAN_POINT ( 'NONE',  ( 10.37757302488624767, 69.72500000273117848, 31.93888565452638417 ) ) ;
#9690=CARTESIAN_POINT ( 'NONE',  ( 24.50000000000000000, 14.00000000000001243, 0.000000000000000000 ) ) ;
#9692=CARTESIAN_POINT ( 'NONE',  ( 27.16883889988623935, 8.325000002731176352, -19.73931689729374384 ) ) ;
#9693=CARTESIAN_POINT ( 'NONE',  ( 5.779280353836490358E-15, 60.49999999999998579, 32.49999999999999289 ) ) ;
#9695=CARTESIAN_POINT ( 'NONE',  ( -9.270509831248421762, 76.30000000000001137, 12.75976212528060039 ) ) ;
#9697=DIRECTION ( 'NONE',  ( -0.000000000000000000, -1.000000000000000000, -0.000000000000000000 ) ) ;
#9698=CARTESIAN_POINT ( 'NONE',  ( -1.778240108872766143E-15, 62.00000000546238255, -32.49999999999999289 ) ) ;
#9700=CARTESIAN_POINT ( 'NONE',  ( 9.270509831248425314, 76.95000000546239960, 12.75976212528059683 ) ) ;
#9702=CARTESIAN_POINT ( 'NONE',  ( -20.75514604977248112, 35.42500000273119554, 28.56700777964554661 ) ) ;
#9705=CARTESIAN_POINT ( 'NONE',  ( 6.486482029760648627E-15, 23.87500000273118417, 35.31076352940722529 ) ) ;
#9707=CARTESIAN_POINT ( 'NONE',  ( -4.405589869732278832E-13, 9.000000005462366559, 32.50000000000000000 ) ) ;
#9710=CARTESIAN_POINT ( 'NONE',  ( 1.507698388325705758E-15, 9.124999997268822938, -24.62258325217400312 ) ) ;
#9711=CARTESIAN_POINT ( 'NONE',  ( 33.58253175000000113, 62.12500000273119127, -4.112674001490185761E-15 ) ) ;
#9714=CARTESIAN_POINT ( 'NONE',  ( -10.37757302488624411, 14.72500000273119269, -31.93888565452638417 ) ) ;
#9715=CARTESIAN_POINT ( 'NONE',  ( -23.41746824999999887, 12.12499999726882116, -2.867812753649727150E-15 ) ) ;
#9717=ORIENTED_EDGE ( 'NONE', *, *, #16366, .F. ) ;
#9723=CARTESIAN_POINT ( 'NONE',  ( -10.04305231718579172, 79.60000000000000853, -30.90933677959248982 ) ) ;
#9725=CARTESIAN_POINT ( 'NONE',  ( -18.94512977948576093, 6.324999997268820451, 13.76444248337722698 ) ) ;
#9726=CARTESIAN_POINT ( 'NONE',  ( 14.47279130897151589, 10.32499999726881335, 19.92008829642072953 ) ) ;
#9727=CARTESIAN_POINT ( 'NONE',  ( -20.75514604977248823, 19.07500000273118701, -28.56700777964554305 ) ) ;
#9728=CARTESIAN_POINT ( 'NONE',  ( 32.50000000000000000, 27.60000000546238752, -10.55989012756945833 ) ) ;
#9729=CARTESIAN_POINT ( 'NONE',  ( -32.50000000000000000, 64.00000000000000000, 0.000000000000000000 ) ) ;
#9733=CARTESIAN_POINT ( 'NONE',  ( 10.37757302488624767, 33.97500000273117848, 31.93888565452638417 ) ) ;
#9734=CARTESIAN_POINT ( 'NONE',  ( -32.50000000000000000, 32.40000000546238113, -10.55989012756945300 ) ) ;
#9737=CARTESIAN_POINT ( 'NONE',  ( 7.236395654485760609, 17.52499999726880731, -22.27133577429736633 ) ) ;
#9738=CARTESIAN_POINT ( 'NONE',  ( 6.277390505771533514E-15, 10.49999999999998757, 34.17252228774368916 ) ) ;
#9739=CARTESIAN_POINT ( 'NONE',  ( 5.147494310547217289, 9.051254287009214750, 32.50000000000007105 ) ) ;
#9741=CARTESIAN_POINT ( 'NONE',  ( 33.58253175000000823, 56.02500000273117564, 10.91162601494192863 ) ) ;
#9743=CARTESIAN_POINT ( 'NONE',  ( 27.16883889988623935, 42.57500000273117990, -19.73931689729374384 ) ) ;
#9745=CARTESIAN_POINT ( 'NONE',  ( -33.58253175000000113, 79.25000000273118417, 0.000000000000000000 ) ) ;
#9746=CARTESIAN_POINT ( 'NONE',  ( -5.147494310547423346, 6.448745718453161579, 32.50000000000000000 ) ) ;
#9749=CYLINDRICAL_SURFACE ( 'NONE', #18808, 32.50000000000000000 ) ;
#9751=DIRECTION ( 'NONE',  ( -0.000000000000000000, -1.000000000000000000, -0.000000000000000000 ) ) ;
#9753=CARTESIAN_POINT ( 'NONE',  ( 0.000000000000000000, 80.00000000000001421, 0.000000000000000000 ) ) ;
#9757=CARTESIAN_POINT ( 'NONE',  ( -20.75514604977248823, 32.82500000273118701, -28.56700777964554305 ) ) ;
#9758=CARTESIAN_POINT ( 'NONE',  ( 20.75514604977248467, 64.67500000273118133, -28.56700777964554305 ) ) ;
#9760=ORIENTED_EDGE ( 'NONE', *, *, #6694, .T. ) ;
#9765=EDGE_LOOP ( 'NONE', ( #32664, #28126, #33399, #21516 ) ) ;
#9769=( BOUNDED_CURVE ( )  B_SPLINE_CURVE ( 2, ( #32718, #12130, #11626, #25177, #32389, #6985, #14214, #16959, #1655, #33056, #20039, #30484, #17468 ),
 .UNSPECIFIED., .F., .T. ) 
 B_SPLINE_CURVE_WITH_KNOTS ( ( 3, 2, 2, 2, 2, 2, 3 ),
 ( 0.3910256410256410242, 0.3923076923076923017, 0.3948717948717948567, 0.3974358974358974117, 0.4000000000000000222, 0.4025641025641025772, 0.4038461538461538547 ),
 .UNSPECIFIED. ) 
 CURVE ( )  GEOMETRIC_REPRESENTATION_ITEM ( )  RATIONAL_B_SPLINE_CURVE ( ( 0.9755282581475768211, 0.9755282581475768211, 1.000000000000000000, 0.9510565162951535312, 1.000000000000000000, 0.9510565162951535312, 1.000000000000000000, 0.9510565162951535312, 1.000000000000000000, 0.9510565162951535312, 1.000000000000000000, 0.9755282581475768211, 0.9755282581475768211 ) ) 
 REPRESENTATION_ITEM ( '' )  );
#9772=CARTESIAN_POINT ( 'NONE',  ( 27.16883889988624290, 40.17500000273119554, 19.73931689729373673 ) ) ;
#9773=CARTESIAN_POINT ( 'NONE',  ( -20.08610463437157989, 46.20000000546237828, -27.64615127144129758 ) ) ;
#9774=( BOUNDED_CURVE ( )  B_SPLINE_CURVE ( 2, ( #26329, #20854, #10213, #28728, #15706, #33884, #25988, #31300, #2817, #23760, #2131, #30961, #7459 ),
 .UNSPECIFIED., .F., .T. ) 
 B_SPLINE_CURVE_WITH_KNOTS ( ( 3, 2, 2, 2, 2, 2, 3 ),
 ( 0.8141025641025640969, 0.8153846153846153744, 0.8179487179487179294, 0.8205128205128204844, 0.8230769230769230393, 0.8256410256410255943, 0.8269230769230769829 ),
 .UNSPECIFIED. ) 
 CURVE ( )  GEOMETRIC_REPRESENTATION_ITEM ( )  RATIONAL_B_SPLINE_CURVE ( ( 0.9755282581475768211, 0.9755282581475768211, 1.000000000000000000, 0.9510565162951535312, 1.000000000000000000, 0.9510565162951535312, 1.000000000000000000, 0.9510565162951535312, 1.000000000000000000, 0.9510565162951535312, 1.000000000000000000, 0.9755282581475757109, 0.9755282581475768211 ) ) 
 REPRESENTATION_ITEM ( '' )  );
#9776=CARTESIAN_POINT ( 'NONE',  ( 10.37757302488624056, 26.52500000273119696, -31.93888565452638417 ) ) ;
#9778=CARTESIAN_POINT ( 'NONE',  ( 27.16883889988624290, 56.17500000273118133, 19.73931689729373673 ) ) ;
#9780=EDGE_CURVE ( 'NONE', #10039, #15956, #17913, .T. ) ;
#9782=CARTESIAN_POINT ( 'NONE',  ( 6.277390505771533514E-15, 24.50000000000001421, 34.17252228774368916 ) ) ;
#9784=CARTESIAN_POINT ( 'NONE',  ( -20.75514604977248112, 75.42500000273120975, 28.56700777964554661 ) ) ;
#9786=CARTESIAN_POINT ( 'NONE',  ( -1.778240108872766143E-15, 70.00000000546238255, -32.49999999999999289 ) ) ;
#9787=CARTESIAN_POINT ( 'NONE',  ( -5.147494310547430452, 20.05125428700922185, -32.49999999999999289 ) ) ;
#9788=CARTESIAN_POINT ( 'NONE',  ( -27.16883889988623935, 61.57500000273119412, 19.73931689729374739 ) ) ;
#9793=CARTESIAN_POINT ( 'NONE',  ( -33.58253175000000113, 19.02500000273118630, -10.91162601494193218 ) ) ;
#9794=CARTESIAN_POINT ( 'NONE',  ( -24.50000000000001066, 12.84999999453761532, 7.960532557706201828 ) ) ;
#9796=CARTESIAN_POINT ( 'NONE',  ( 10.04305231718579705, 46.60000000000000142, 30.90933677959248982 ) ) ;
#9801=CARTESIAN_POINT ( 'NONE',  ( 10.04305231718579705, 3.100000005462372421, 30.90933677959248982 ) ) ;
#9806=CARTESIAN_POINT ( 'NONE',  ( 0.000000000000000000, 80.00000000000001421, 0.000000000000000000 ) ) ;
#9807=CARTESIAN_POINT ( 'NONE',  ( 32.50000000000000000, 77.50000000546236834, -3.980102097228898626E-15 ) ) ;
#9812=CARTESIAN_POINT ( 'NONE',  ( 20.75514604977248467, 72.67500000273118133, -28.56700777964554305 ) ) ;
#9815=CARTESIAN_POINT ( 'NONE',  ( -32.50000000000000000, 62.50000000546238255, 0.000000000000000000 ) ) ;
#9817=CARTESIAN_POINT ( 'NONE',  ( -26.29305231718578995, 10.70000000546239605, 19.10302069950538595 ) ) ;
#9818=CARTESIAN_POINT ( 'NONE',  ( -33.58253175000000113, 47.22500000273117138, 10.91162601494193929 ) ) ;
#9819=CARTESIAN_POINT ( 'NONE',  ( -7.236395654485757944, 15.22499999726881192, -22.27133577429736988 ) ) ;
#9820=CARTESIAN_POINT ( 'NONE',  ( -32.50000000000000000, 6.600000005462382191, 10.55989012756946366 ) ) ;
#9821=CARTESIAN_POINT ( 'NONE',  ( -5.147494310547430452, 7.551254281546841085, -32.49999999999999289 ) ) ;
#9822=DIRECTION ( 'NONE',  ( 0.000000000000000000, 0.000000000000000000, -1.000000000000000000 ) ) ;
#9823=CARTESIAN_POINT ( 'NONE',  ( -32.50000000000000000, 50.09999999999998721, 10.55989012756946366 ) ) ;
#9824=CARTESIAN_POINT ( 'NONE',  ( -1.778240108872766143E-15, 10.00000000546236834, -32.49999999999999289 ) ) ;
#9825=CARTESIAN_POINT ( 'NONE',  ( 20.75514604977249178, 18.07500000273119056, 28.56700777964553950 ) ) ;
#9826=CARTESIAN_POINT ( 'NONE',  ( 0.000000000000000000, 0.000000000000000000, 0.000000000000000000 ) ) ;
#9828=CARTESIAN_POINT ( 'NONE',  ( 11.25946833292375793, 78.57500000273121543, -8.180482586598735395 ) ) ;
#9832=ORIENTED_EDGE ( 'NONE', *, *, #27334, .F. ) ;
#9840=CARTESIAN_POINT ( 'NONE',  ( 27.16883889988624290, 2.175000002731186655, 19.73931689729373673 ) ) ;
#9845=CARTESIAN_POINT ( 'NONE',  ( -11.25946833292375793, 71.57500000273120122, 8.180482586598737171 ) ) ;
#9847=CARTESIAN_POINT ( 'NONE',  ( -33.58253175000000113, 45.12500000273117706, 0.000000000000000000 ) ) ;
#9850=ORIENTED_EDGE ( 'NONE', *, *, #13566, .F. ) ;
#9852=CARTESIAN_POINT ( 'NONE',  ( -5.147494310547423346, 4.948745723915524586, 32.50000000000000000 ) ) ;
#9854=CARTESIAN_POINT ( 'NONE',  ( 10.37757302488624056, 74.77500000273118985, -31.93888565452638417 ) ) ;
#9858=ORIENTED_EDGE ( 'NONE', *, *, #2571, .F. ) ;
#9859=FACE_OUTER_BOUND ( 'NONE', #22768, .T. ) ;
#9860=CARTESIAN_POINT ( 'NONE',  ( -33.58253175000000113, 65.22500000273117848, 10.91162601494193929 ) ) ;
#9862=CARTESIAN_POINT ( 'NONE',  ( 7.570916362186213000, 14.39999999999999680, -23.30088464923126423 ) ) ;
#9863=CARTESIAN_POINT ( 'NONE',  ( 23.41746824999999887, 1.124999997268810725, 0.000000000000000000 ) ) ;
#9864=CARTESIAN_POINT ( 'NONE',  ( -20.75514604977248823, 12.82500000273118168, -28.56700777964554305 ) ) ;
#9867=CARTESIAN_POINT ( 'NONE',  ( -1.778240108872766143E-15, 37.50000000000000000, -32.49999999999999289 ) ) ;
#9869=CARTESIAN_POINT ( 'NONE',  ( 26.29305231718579350, 22.79999999999998650, 19.10302069950537529 ) ) ;
#9871=CARTESIAN_POINT ( 'NONE',  ( -4.635254915624211769, 77.85000000546237686, -14.26584774442730286 ) ) ;
#9873=( BOUNDED_CURVE ( )  B_SPLINE_CURVE ( 2, ( #21546, #13018, #10442, #5292, #31993, #28117, #25549, #2195, #27523, #14152, #3679, #24609, #14485, #1425, #22212, #24773, #22045, #26854, #1251, #11401, #29578, #9154, #8991, #32659, #8489, #8656, #14317, #29921, #32490, #24446, #3513, #19637, #21878, #922, #19141, #11731, #17062, #6080, #13820, #30080, #16563, #3350, #24288, #1083, #5923, #760, #11241, #6586, #4010, #24941, #19471, #32163, #11903, #22375, #18976, #29421, #29746, #27016, #16400, #21718, #13984, #32328, #8819, #19304, #6252, #6424, #16731, #27187, #11563, #16896, #27358, #3843, #28378, #1591, #23061, #9672, #10024, #17747, #25801, #33168, #20497, #6752, #22890, #2292, #4350, #14656, #19799, #12242, #4867, #7443, #27692, #22539, #2117, #14826, #30249, #33520, #30946, #15347, #9845, #25638, #17405 ),
 .UNSPECIFIED., .F., .T. ) 
 B_SPLINE_CURVE_WITH_KNOTS ( ( 3, 2, 2, 2, 2, 2, 2, 2, 2, 2, 2, 2, 2, 2, 2, 2, 2, 2, 2, 2, 2, 2, 2, 2, 2, 2, 2, 2, 2, 2, 2, 2, 2, 2, 2, 2, 2, 2, 2, 2, 2, 2, 2, 2, 2, 2, 2, 2, 2, 2, 3 ),
 ( 0.000000000000000000, 0.02000000000000000042, 0.04000000000000000083, 0.05999999999999999778, 0.08000000000000000167, 0.1000000000000000056, 0.1199999999999999956, 0.1400000000000000133, 0.1600000000000000033, 0.1799999999999999933, 0.2000000000000000111, 0.2200000000000000011, 0.2399999999999999911, 0.2600000000000000089, 0.2800000000000000266, 0.2999999999999999889, 0.3200000000000000067, 0.3400000000000000244, 0.3599999999999999867, 0.3800000000000000044, 0.4000000000000000222, 0.4199999999999999845, 0.4400000000000000022, 0.4600000000000000200, 0.4799999999999999822, 0.5000000000000000000, 0.5200000000000000178, 0.5400000000000000355, 0.5600000000000000533, 0.5799999999999999600, 0.5999999999999999778, 0.6199999999999999956, 0.6400000000000000133, 0.6600000000000000311, 0.6800000000000000488, 0.6999999999999999556, 0.7199999999999999734, 0.7399999999999999911, 0.7600000000000000089, 0.7800000000000000266, 0.8000000000000000444, 0.8199999999999999512, 0.8399999999999999689, 0.8599999999999999867, 0.8800000000000000044, 0.9000000000000000222, 0.9200000000000000400, 0.9399999999999999467, 0.9599999999999999645, 0.9799999999999999822, 1.000000000000000000 ),
 .UNSPECIFIED. ) 
 CURVE ( )  GEOMETRIC_REPRESENTATION_ITEM ( )  RATIONAL_B_SPLINE_CURVE ( ( 1.000000000000000000, 0.9510565162951535312, 1.000000000000000000, 0.9510565162951535312, 1.000000000000000000, 0.9510565162951535312, 1.000000000000000000, 0.9510565162951535312, 1.000000000000000000, 0.9510565162951535312, 1.000000000000000000, 0.9510565162951535312, 1.000000000000000000, 0.9510565162951535312, 1.000000000000000000, 0.9510565162951535312, 1.000000000000000000, 0.9510565162951535312, 1.000000000000000000, 0.9510565162951535312, 1.000000000000000000, 0.9510565162951535312, 1.000000000000000000, 0.9510565162951535312, 1.000000000000000000, 0.9510565162951535312, 1.000000000000000000, 0.9510565162951535312, 1.000000000000000000, 0.9510565162951535312, 1.000000000000000000, 0.9510565162951535312, 1.000000000000000000, 0.9510565162951535312, 1.000000000000000000, 0.9510565162951535312, 1.000000000000000000, 0.9510565162951535312, 1.000000000000000000, 0.9510565162951535312, 1.000000000000000000, 0.9510565162951535312, 1.000000000000000000, 0.9510565162951535312, 1.000000000000000000, 0.9510565162951535312, 1.000000000000000000, 0.9510565162951535312, 1.000000000000000000, 0.9510565162951535312, 1.000000000000000000, 0.9510565162951535312, 1.000000000000000000, 0.9510565162951535312, 1.000000000000000000, 0.9510565162951535312, 1.000000000000000000, 0.9510565162951535312, 1.000000000000000000, 0.9510565162951535312, 1.000000000000000000, 0.9510565162951535312, 1.000000000000000000, 0.9510565162951535312, 1.000000000000000000, 0.9510565162951535312, 1.000000000000000000, 0.9510565162951535312, 1.000000000000000000, 0.9510565162951535312, 1.000000000000000000, 0.9510565162951535312, 1.000000000000000000, 0.9510565162951535312, 1.000000000000000000, 0.9510565162951535312, 1.000000000000000000, 0.9510565162951535312, 1.000000000000000000, 0.9510565162951535312, 1.000000000000000000, 0.9510565162951535312, 1.000000000000000000, 0.9510565162951535312, 1.000000000000000000, 0.9510565162951535312, 1.000000000000000000, 0.9510565162951535312, 1.000000000000000000, 0.9510565162951535312, 1.000000000000000000, 0.9510565162951535312, 1.000000000000000000, 0.9510565162951535312, 1.000000000000000000, 0.9510565162951535312, 1.000000000000000000, 0.9510565162951535312, 1.000000000000000000, 0.9510565162951535312, 1.000000000000000000 ) ) 
 REPRESENTATION_ITEM ( '' )  );
#9874=CARTESIAN_POINT ( 'NONE',  ( 20.75514604977248467, 28.42500000273118133, -28.56700777964554305 ) ) ;
#9877=CARTESIAN_POINT ( 'NONE',  ( 27.16883889988623935, 22.57500000273118701, -19.73931689729374384 ) ) ;
#9878=CARTESIAN_POINT ( 'NONE',  ( -26.29305231718579350, 12.30000000546238681, -19.10302069950537884 ) ) ;
#9879=CARTESIAN_POINT ( 'NONE',  ( 27.16883889988624290, 73.92500000273119554, 19.73931689729373673 ) ) ;
#9880=EDGE_CURVE ( 'NONE', #25888, #14943, #27167, .T. ) ;
#9881=CARTESIAN_POINT ( 'NONE',  ( -5.147494310547423346, 66.44874571845315359, 32.50000000000000000 ) ) ;
#9884=CARTESIAN_POINT ( 'NONE',  ( 10.37757302488624056, 62.52500000273120406, -31.93888565452638417 ) ) ;
#9890=CARTESIAN_POINT ( 'NONE',  ( 20.75514604977248467, 4.425000002731183990, -28.56700777964554305 ) ) ;
#9891=CARTESIAN_POINT ( 'NONE',  ( -18.94512977948576093, 12.32499999726882578, 13.76444248337722698 ) ) ;
#9899=DIRECTION ( 'NONE',  ( -0.000000000000000000, -1.000000000000000000, -0.000000000000000000 ) ) ;
#9900=CARTESIAN_POINT ( 'NONE',  ( -32.50000000000000000, 72.40000000546238823, -10.55989012756945300 ) ) ;
#9901=CARTESIAN_POINT ( 'NONE',  ( 14.47279130897151589, 4.824999997268814234, 19.92008829642072953 ) ) ;
#9902=CARTESIAN_POINT ( 'NONE',  ( 23.41746825000000243, 12.52499999726880375, 7.608796670333735079 ) ) ;
#9903=CARTESIAN_POINT ( 'NONE',  ( 20.75514604977249178, 18.07500000273119056, 28.56700777964553950 ) ) ;
#9904=CARTESIAN_POINT ( 'NONE',  ( -32.50000000000000000, 24.40000000546237047, -10.55989012756945478 ) ) ;
#9905=CARTESIAN_POINT ( 'NONE',  ( 6.277390505771533514E-15, 66.49999999999998579, 34.17252228774368916 ) ) ;
#9906=CARTESIAN_POINT ( 'NONE',  ( 19.82091636218621034, 11.54999999453762349, 14.40073868116559730 ) ) ;
#9909=CARTESIAN_POINT ( 'NONE',  ( -20.75514604977248112, 29.67500000273119909, 28.56700777964554661 ) ) ;
#9910=CARTESIAN_POINT ( 'NONE',  ( 20.08610463437158344, 43.20000000546236407, 27.64615127144129403 ) ) ;
#9913=CARTESIAN_POINT ( 'NONE',  ( -23.41746824999999887, 14.12499999726882294, -2.867812753649727150E-15 ) ) ;
#9914=( BOUNDED_SURFACE ( )  B_SPLINE_SURFACE ( 1, 2, ( 
 ( #236, #10722, #31644, #18631, #5059, #15544, #5572, #31811, #33892, #31143, #2489, #12958, #26171, #2431, #30563, #28345, #7229, #15141, #33313, #23374, #18059, #20808, #30736, #20119, #4316, #4830, #7060, #20461, #15310, #12899, #25769, #17542, #23199, #33661, #10159, #30912, #17715, #2084, #28002, #25605, #1909, #33487, #25938, #33835, #12386, #5001, #28173, #4489, #23030, #28504, #4661, #20289, #31252, #31084, #7580, #9988, #14965, #12559, #2255, #22681, #15484, #12729, #25431, #10332, #7406, #20641, #22855, #9812, #17892, #17370, #27833, #14791, #25255, #1730, #12210, #33132, #9636, #23383, #9997, #10505, #2616, #20817, #28688, #18581, #17901, #31093, #13079, #7925, #28856, #15669, #31261, #28515, #23553, #10169, #20983, #5186, #26291, #7415, #31432, #20653, #2266, #5524, #23719, #5011, #21153, #5354, #185, #31594, #25947, #16, #15834, #26119, #8094, #18410, #2780, #7590, #13246, #29022, #18067, #15493, #10673, #2441, #20470, #16004, #26459, #2950, #13422, #25778, #33846, #23889, #30922, #28354, #4840, #15321, #12739, #23210, #12909, #33672, #10341, #7755, #18242, #27292, #8593, #10844, #24224, #8758, #31930, #24387, #27124, #19078, #19409, #29857, #19242, #13753, #26628, #11180, #11013, #694, #8926, #31762, #21483, #21817, #8422, #21651, #32266, #3451, #29680, #3122, #32097, #16172, #16837, #861, #6185, #3285, #26793, #6358, #11341, #13594, #526, #21981, #32430, #29517, #6021, #21322, #13922, #16497, #360, #5859, #16337, #16667, #18912, #26952, #1019, #3617, #14091, #14255, #24548, #11502, #3784, #24058, #8254, #18747, #5694, #29189, #29358, #1361, #7200, #14593, #20088, #11840, #24880, #22318, #27803, #12007, #22478, #32926, #1189, #9425, #24712, #30532, #11671, #32762, #17512, #3950, #27973, #30025, #9257, #22153, #4456, #9095, #14933, #32596, #9778, #20260, #30704, #27632, #12179, #1876, #25399, #7029, #4287, #19577, #1533, #4119, #19910, #30359, #6861, #14761, #17340, #6529, #17002, #12354, #25052, #14425, #17681, #22823, #30187, #27459, #28143, #19742, #1701, #25224, #22650, #6690, #4629, #33282, #17174, #33102, #9606, #2053, #26081, #4799, #18203, #2577, #10635, #13042, #15278, #20944, #31393, #7883, #28645, #15452, #33808, #25739, #12869, #33630, #31223, #23680, #145, #10129, #2740, #28479, #23513, #12528, #10302, #4975, #18373, #2219, #12698, #23347, #23168, #30878, #20779, #7716, #5142, #2401, #22996, #33455, #28818, #25907, #20611, #31557, #15796, #31056, #9954, #21113, #28311, #33972, #15630, #10466, #7548, #8054, #26252, #18540, #5314, #17859, #20429, #13203, #18033, #28985, #15108, #25573, #7375, #29147, #11304, #21782, #32230, #19041, #5821, #24182, #5652, #3248, #24017, #21612, #14050, #24511, #489, #27084, #18869, #13885, #26419, #654, #29318, #8719, #16134, #26589, #13716, #13554, #21285, #31889, #983, #5984, #18710, #3085, #3578, #11468, #16297, #11143, #2913, #29480, #26755, #5484, #10971, #21446, #823, #8385, #32057, #6144, #8557, #16461, #19372, #19202, #29641, #26914, #3412, #24351, #16629, #10805, #21942, #32392, #8887, #15963, #13381, #23853, #317, #31726, #8217, #32884, #17131, #27587, #4076, #6319, #14551, #29816, #25180, #16795, #3911, #22605, #9056, #33059, #1147, #16962, #27253, #9564, #14217, #20042, #3745, #14892, #25353, #1832, #32721, #17297, #6988, #30487, #12133, #9383, #24673, #6650, #9217, #25010, #6816, #19701, #1492, #11800, #12310, #17471, #33234, #30146, #32557, #11629, #27758, #19536, #19865, #4246, #22782, #14720, #29984, #1658, #27931, #4415, #30319, #11966, #22437, #6489, #9733, #14380, #22113, #27420, #24839, #1317, #22278, #33585, #29064, #7156, #5402, #10086, #26505, #20386, #7329, #28900, #28271, #2009, #12651, #16219, #21198, #33412, #30837, #8299, #18791, #20565, #15878, #17639, #233, #7507, #20219, #25697, #2178, #16051, #17813, #26335, #21365, #31010, #23121, #571, #405, #10892, #13293, #9909, #2824, #5569, #25532, #31808, #2998, #4757, #3169, #17991, #13471, #15234, #23766, #10719, #31641, #8139, #18628, #23936, #30659, #29235, #28100, #5740, #4588, #26674, #13639, #24103, #15064, #12485, #22954, #21527, #3825, #29403, #14299, #18958, #30063, #6569, #17043, #13964, #32470, #22195, #24756, #27339, #24591, #5905, #21861, #24426, #32308, #16712, #8801, #1064, #19283, #8473, #16382, #1233, #903, #737, #27504, #11711, #16543, #26835, #3994, #24270, #32641, #9136, #19618, #11544, #3331, #29726, #11385, #6232, #27166, #3659, #22026, #14135, #13801, #11223, #14466, #8971, #21697, #24923, #11062, #26996, #32143, #31975, #8637, #19454, #29899, #6402, #3494, #19122, #29559, #6060, #16876, #4164, #22357, #12400, #25097, #4502, #22870, #30928, #33328, #1574, #7241, #17730, #28187, #14977, #1744, #20133, #12051, #33149, #19958, #17558, #10004, #20477, #30406, #23043, #14806, #9825, #32804, #30578, #25271, #4675, #22521, #32972, #9653, #9476, #17216, #27850, #7421, #1923, #14637, #6904, #33501, #17907, #12224, #7074, #9297, #25447, #22697, #1408, #17385, #4333, #30752, #28015, #20302, #2099, #15154, #25619, #15328, #12572, #28360, #4847, #11886, #19781, #30231, #6734, #27675, #192, #2448, #8261, #15677, #21160, #12914, #25955, #23390, #28863, #13085, #23559, #23, #2272, #10512, #25783, #31602, #12745, #33852, #18587, #5017, #29027, #31099, #10347, #23219, #5530, #10177, #16011, #33678, #10852, #21327, #31768, #28695, #13252, #20989, #20824, #7596, #18248, #18753, #26297, #15499, #31268, #13427, #23895, #26125, #31439, #20659, #5360, #7931, #18073, #7762, #5193, #8100, #2622, #18419, #26465, #15840, #2786, #5701, #2958, #366, #23726, #10679, #29195, #28522, #21489, #6363, #24552, #26798, #32600, #6024, #11506, #3292, #16342, #13757, #19245, #3454, #13926, #24390, #26634, #864, #16179, #21986, #3128, #24228, #8932, #29364, #19413, #31936, #698, #13601, #29862, #532, #16841, #24066, #1194, #11675, #22158, #19081, #3622, #27297, #3789, #32434, #29684, #11019, #26955, #29521, #11345, #21822, #32269, #6189, #8763, #8429, #18918, #14260, #16502, #5864, #9100, #24717, #21655, #11185, #19581, #32100, #27128, #16671, #14096, #8598, #30029, #1025 ),
 ( #25578, #1538, #28148, #19916, #14938, #27465, #25231, #30364, #12359, #6695, #27636, #17344, #25056, #33108, #17178, #17516, #1705, #22827, #3955, #7033, #4124, #32768, #2057, #20264, #12013, #17688, #1881, #30710, #4634, #22482, #9611, #25403, #12184, #15113, #22654, #20092, #14599, #9784, #12533, #32931, #9430, #30537, #6865, #6534, #27977, #23002, #33459, #4462, #22323, #27807, #33287, #9958, #24884, #7204, #14429, #20434, #17007, #4291, #1367, #14766, #19746, #11844, #9262, #30192, #7380, #20784, #5320, #28483, #20949, #23685, #5147, #15968, #26424, #15800, #10306, #23173, #7721, #7553, #31229, #5489, #28316, #18038, #18377, #4979, #18208, #28822, #33977, #26256, #33635, #28651, #12702, #13385, #31398, #2744, #33813, #12874, #15634, #2918, #23858, #25743, #13208, #10810, #10471, #25913, #26086, #30884, #2582, #150, #323, #17864, #10639, #15283, #4804, #15457, #20616, #13046, #23518, #7888, #2406, #23351, #21118, #31561, #8059, #18544, #28990, #2225, #10134, #31060, #21786, #13890, #32062, #5988, #29823, #29151, #8389, #24357, #19210, #6149, #26920, #8562, #31730, #29485, #21290, #16634, #8221, #29323, #14056, #493, #24518, #26593, #18874, #18715, #988, #5657, #11473, #16139, #6327, #16804, #27260, #24187, #8726, #32398, #21947, #3584, #827, #3090, #19046, #659, #16465, #3416, #11308, #32234, #29647, #13561, #24024, #8893, #11147, #10976, #3751, #19377, #26760, #21450, #14225, #31893, #27090, #21618, #24681, #3252, #1155, #5825, #16304, #13722, #14391, #32564, #22614, #1327, #14728, #33067, #7165, #9573, #11808, #17478, #27940, #4423, #25189, #11976, #30327, #22286, #9390, #30154, #27768, #20227, #30667, #6658, #33243, #25019, #20049, #9063, #6823, #1499, #14898, #32731, #9224, #19874, #19708, #27427, #4085, #17647, #12141, #24847, #17141, #9741, #28108, #22444, #17305, #19544, #1666, #32891, #11637, #27594, #14559, #6996, #4253, #30495, #12320, #25362, #1840, #25539, #22790, #4595, #15072, #22121, #29992, #6496, #16969, #3918, #10433, #12660, #18509, #25872, #31359, #23129, #2186, #33595, #5110, #23311, #33776, #33942, #4936, #18000, #15418, #8023, #10603, #30846, #20908, #15932, #15594, #31017, #10267, #2018, #2364, #23480, #21081, #31530, #5282, #20395, #28955, #20574, #25705, #20749, #18168, #28610, #7515, #10095, #26048, #31192, #7851, #15765, #28445, #13008, #12837, #12493, #2541, #18339, #7682, #28784, #5451, #9918, #26219, #2711, #13172, #23650, #112, #22962, #33420, #7337, #17822, #28278, #4765, #15243, #23820, #26885, #26556, #18678, #21909, #6112, #10940, #3543, #21750, #16594, #14015, #8350, #19007, #11274, #21580, #24478, #8523, #29451, #3052, #29610, #952, #23986, #13523, #5953, #458, #26388, #3382, #11432, #32359, #24318, #8188, #5786, #13852, #8853, #10774, #27050, #286, #32026, #19334, #18840, #791, #26724, #5621, #29779, #6284, #622, #2880, #16267, #32195, #21415, #16433, #19173, #11110, #13347, #21251, #8689, #3219, #29118, #13687, #31858, #24151, #31695, #16105, #29286, #4214, #14349, #17096, #14688, #19831, #25147, #9022, #27554, #32522, #33199, #6785, #20182, #30113, #19504, #3712, #27726, #6455, #30283, #1623, #12275, #12101, #16929, #22572, #33022, #9528, #17263, #4042, #1458, #27387, #14516, #1284, #32853, #25322, #1796, #11763, #4381, #6617, #20009, #14182, #11936, #24975, #30456, #3876, #24806, #22405, #22245, #29951, #9184, #22748, #6953, #32689, #19668, #14856, #9702, #9348, #17437, #24638, #27899, #30626, #16760, #27219, #1112, #11597, #22077, #12796, #7810, #7477, #10052, #21040, #20870, #31318, #33731, #30801, #15377, #26005, #12452, #18299, #15552, #17779, #23606, #30976, #2497, #28237, #7294, #4723, #10229, #28407, #4897, #25832, #17604, #2322, #7123, #12966, #28066, #15203, #33901, #20352, #10392, #22922, #25667, #4553, #28744, #25497, #5241, #15032, #26179, #2674, #13132, #20533, #28571, #15724, #73, #23440, #20709, #1977, #17958, #23269, #31151, #7642, #18126, #5068, #10561, #33378, #9874, #2146, #12621, #23088, #33552, #32154, #3010, #26346, #16554, #10731, #8482, #21375, #29245, #13482, #3504, #8647, #5915, #11393, #11071, #26516, #5749, #31490, #31820, #18969, #6070, #27007, #747, #15890, #13974, #16061, #21208, #16230, #13649, #24114, #23947, #18639, #21537, #18801, #16392, #11232, #416, #29414, #10903, #7980, #31985, #581, #8310, #26684, #24437, #5411, #29076, #26845, #3341, #13811, #3180, #24279, #21708, #19132, #31653, #29569, #914, #18467, #28910, #2835, #8150, #23779, #13304, #246, #5580, #33465, #17694, #12539, #9965, #4297, #14944, #7211, #17522, #20440, #4470, #25410, #32481, #25583, #30891, #19464, #22037, #1887, #8982, #21870, #33293, #7386, #17870, #20269, #3671, #1712, #9793, #28321, #6242, #2063, #19294, #27983, #4810, #14772, #30716, #22661, #1075, #23010, #15289, #30544, #32320, #12190, #28154, #29913, #12365, #15119, #7040, #25749, #2233, #4640, #33114, #14145, #9616, #6415, #20098, #8811, #29738, #16887, #16723, #27350, #22833, #27178, #24601, #11555, #25237, #13051, #28487, #29157, #2749, #10646, #15639, #28658, #26090, #18721, #21296, #7558, #15465, #33642, #23690, #2413, #15805, #155, #8227, #21123, #12879, #18549, #28994, #5494, #26261, #23523, #31403, #23356, #10476, #31234, #28827, #31736, #5663, #7726, #330, #2587, #31566, #10139, #7897, #33982, #15973, #33817, #10311, #20954, #20789, #4984, #5154, #16146, #13213, #25918, #18214, #10816, #26599, #18381, #5325, #20621, #8064, #26429, #12708, #2922, #13391, #23863, #23179, #31063, #18043, #3420, #5993, #16973, #16808, #27264, #29651, #26766, #11311, #21952, #8394, #3755, #11477, #13727, #19548, #26924, #32401, #24192, #3257, #664, #6154, #24361, #831, #21790, #13567, #32238, #3096, #8897, #24030, #11152, #29827, #16310, #6331, #18880, #21623, #499, #14229, #21456, #24685, #10982, #22125, #32568, #9067, #16469, #24522, #1160, #11641, #19381, #16638, #31899, #13894, #8731, #19215, #27094, #3587, #14060, #992, #29329, #5831, #29996, #6500, #32066, #8566, #19050, #29489, #22290, #12499, #6663, #4428, #17310, #25193, #9394, #33426, #28113, #30851, #6828, #4258, #4089 ) ),
 .UNSPECIFIED., .F., .F., .T. ) 
 B_SPLINE_SURFACE_WITH_KNOTS ( ( 2, 2 ),
 ( 3, 2, 2, 2, 2, 2, 2, 2, 2, 2, 2, 2, 2, 2, 2, 2, 2, 2, 2, 2, 2, 2, 2, 2, 2, 2, 2, 2, 2, 2, 2, 2, 2, 2, 2, 2, 2, 2, 2, 2, 2, 2, 2, 2, 2, 2, 2, 2, 2, 2, 2, 2, 2, 2, 2, 2, 2, 2, 2, 2, 2, 2, 2, 2, 2, 2, 2, 2, 2, 2, 2, 2, 2, 2, 2, 2, 2, 2, 2, 2, 2, 2, 2, 2, 2, 2, 2, 2, 2, 2, 2, 2, 2, 2, 2, 2, 2, 2, 2, 2, 2, 2, 2, 2, 2, 2, 2, 2, 2, 2, 2, 2, 2, 2, 2, 2, 2, 2, 2, 2, 2, 2, 2, 2, 2, 2, 2, 2, 2, 2, 2, 2, 2, 2, 2, 2, 2, 2, 2, 2, 2, 2, 2, 2, 2, 2, 2, 2, 2, 2, 2, 2, 2, 2, 2, 2, 2, 2, 2, 2, 2, 2, 2, 2, 2, 2, 2, 2, 2, 2, 2, 2, 2, 2, 2, 2, 2, 2, 2, 2, 2, 2, 2, 2, 2, 2, 2, 2, 2, 2, 2, 2, 2, 2, 2, 2, 2, 2, 2, 2, 2, 2, 2, 2, 2, 2, 2, 2, 2, 2, 2, 2, 2, 2, 2, 2, 2, 2, 2, 2, 2, 2, 2, 2, 2, 2, 2, 2, 2, 2, 2, 2, 2, 2, 2, 2, 2, 2, 2, 2, 2, 2, 2, 2, 2, 2, 2, 2, 2, 2, 2, 2, 2, 2, 2, 2, 2, 2, 2, 2, 2, 2, 2, 2, 2, 2, 2, 2, 2, 2, 2, 2, 2, 2, 2, 2, 2, 2, 2, 2, 2, 2, 2, 2, 2, 2, 2, 2, 2, 2, 2, 2, 2, 2, 2, 2, 2, 2, 2, 2, 2, 2, 2, 2, 2, 2, 2, 2, 2, 2, 2, 2, 2, 2, 2, 2, 2, 2, 2, 2, 2, 2, 2, 2, 2, 2, 2, 2, 2, 2, 2, 2, 2, 2, 2, 2, 2, 2, 2, 2, 2, 2, 2, 2, 2, 2, 2, 2, 2, 2, 2, 2, 2, 2, 2, 2, 2, 2, 2, 2, 2, 2, 2, 2, 2, 2, 2, 2, 2, 2, 2, 2, 2, 2, 2, 2, 2, 2, 2, 2, 2, 2, 2, 2, 2, 2, 2, 2, 2, 2, 3 ),
 ( 0.000000000000000000, 1.000000000000000000 ),
 ( 0.000000000000000000, 0.002564102564102564100, 0.005128205128205128201, 0.007692307692307692735, 0.01025641025641025640, 0.01282051282051282007, 0.01538461538461538547, 0.01794871794871794740, 0.02051282051282051280, 0.02307692307692307820, 0.02564102564102564014, 0.02820512820512820554, 0.03076923076923077094, 0.03333333333333333287, 0.03589743589743589480, 0.03846153846153846367, 0.04102564102564102561, 0.04358974358974358754, 0.04615384615384615641, 0.04871794871794871834, 0.05128205128205128027, 0.05384615384615384914, 0.05641025641025641107, 0.05897435897435897301, 0.06153846153846154188, 0.06410256410256409687, 0.06666666666666666574, 0.06923076923076923461, 0.07179487179487178961, 0.07435897435897435848, 0.07692307692307692735, 0.07948717948717948234, 0.08205128205128205121, 0.08461538461538462008, 0.08717948717948717507, 0.08974358974358974395, 0.09230769230769231282, 0.09487179487179486781, 0.09743589743589743668, 0.1000000000000000056, 0.1025641025641025605, 0.1051282051282051294, 0.1076923076923076983, 0.1102564102564102533, 0.1128205128205128221, 0.1153846153846153910, 0.1179487179487179460, 0.1205128205128205149, 0.1230769230769230838, 0.1256410256410256387, 0.1282051282051281937, 0.1307692307692307765, 0.1333333333333333315, 0.1358974358974358865, 0.1384615384615384692, 0.1410256410256410242, 0.1435897435897435792, 0.1461538461538461620, 0.1487179487179487170, 0.1512820512820512719, 0.1538461538461538547, 0.1564102564102564097, 0.1589743589743589647, 0.1615384615384615474, 0.1641025641025641024, 0.1666666666666666574, 0.1692307692307692402, 0.1717948717948717952, 0.1743589743589743501, 0.1769230769230769329, 0.1794871794871794879, 0.1820512820512820429, 0.1846153846153846256, 0.1871794871794871806, 0.1897435897435897356, 0.1923076923076923184, 0.1948717948717948734, 0.1974358974358974284, 0.2000000000000000111, 0.2025641025641025661, 0.2051282051282051211, 0.2076923076923077038, 0.2102564102564102588, 0.2128205128205128138, 0.2153846153846153966, 0.2179487179487179516, 0.2205128205128205066, 0.2230769230769230893, 0.2256410256410256443, 0.2282051282051281993, 0.2307692307692307820, 0.2333333333333333370, 0.2358974358974358920, 0.2384615384615384748, 0.2410256410256410298, 0.2435897435897435848, 0.2461538461538461675, 0.2487179487179487225, 0.2512820512820512775, 0.2538461538461538325, 0.2564102564102563875, 0.2589743589743589980, 0.2615384615384615530, 0.2641025641025641080, 0.2666666666666666630, 0.2692307692307692180, 0.2717948717948717730, 0.2743589743589743835, 0.2769230769230769384, 0.2794871794871794934, 0.2820512820512820484, 0.2846153846153846034, 0.2871794871794871584, 0.2897435897435897689, 0.2923076923076923239, 0.2948717948717948789, 0.2974358974358974339, 0.2999999999999999889, 0.3025641025641025439, 0.3051282051282051544, 0.3076923076923077094, 0.3102564102564102644, 0.3128205128205128194, 0.3153846153846153744, 0.3179487179487179294, 0.3205128205128205399, 0.3230769230769230949, 0.3256410256410256499, 0.3282051282051282048, 0.3307692307692307598, 0.3333333333333333148, 0.3358974358974358698, 0.3384615384615384803, 0.3410256410256410353, 0.3435897435897435903, 0.3461538461538461453, 0.3487179487179487003, 0.3512820512820512553, 0.3538461538461538658, 0.3564102564102564208, 0.3589743589743589758, 0.3615384615384615308, 0.3641025641025640858, 0.3666666666666666408, 0.3692307692307692513, 0.3717948717948718063, 0.3743589743589743613, 0.3769230769230769162, 0.3794871794871794712, 0.3820512820512820262, 0.3846153846153846367, 0.3871794871794871917, 0.3897435897435897467, 0.3923076923076923017, 0.3948717948717948567, 0.3974358974358974117, 0.4000000000000000222, 0.4025641025641025772, 0.4051282051282051322, 0.4076923076923076872, 0.4102564102564102422, 0.4128205128205127972, 0.4153846153846154077, 0.4179487179487179627, 0.4205128205128205177, 0.4230769230769230727, 0.4256410256410256276, 0.4282051282051281826, 0.4307692307692307931, 0.4333333333333333481, 0.4358974358974359031, 0.4384615384615384581, 0.4410256410256410131, 0.4435897435897435681, 0.4461538461538461786, 0.4487179487179487336, 0.4512820512820512886, 0.4538461538461538436, 0.4564102564102563986, 0.4589743589743589536, 0.4615384615384615641, 0.4641025641025641191, 0.4666666666666666741, 0.4692307692307692291, 0.4717948717948717841, 0.4743589743589743390, 0.4769230769230769496, 0.4794871794871795045, 0.4820512820512820595, 0.4846153846153846145, 0.4871794871794871695, 0.4897435897435897245, 0.4923076923076923350, 0.4948717948717948900, 0.4974358974358974450, 0.5000000000000000000, 0.5025641025641025550, 0.5051282051282051100, 0.5076923076923076650, 0.5102564102564102200, 0.5128205128205127750, 0.5153846153846153300, 0.5179487179487179960, 0.5205128205128205510, 0.5230769230769231060, 0.5256410256410256610, 0.5282051282051282159, 0.5307692307692307709, 0.5333333333333333259, 0.5358974358974358809, 0.5384615384615384359, 0.5410256410256409909, 0.5435897435897435459, 0.5461538461538461009, 0.5487179487179487669, 0.5512820512820513219, 0.5538461538461538769, 0.5564102564102564319, 0.5589743589743589869, 0.5615384615384615419, 0.5641025641025640969, 0.5666666666666666519, 0.5692307692307692069, 0.5717948717948717618, 0.5743589743589743168, 0.5769230769230768718, 0.5794871794871795379, 0.5820512820512820928, 0.5846153846153846478, 0.5871794871794872028, 0.5897435897435897578, 0.5923076923076923128, 0.5948717948717948678, 0.5974358974358974228, 0.5999999999999999778, 0.6025641025641025328, 0.6051282051282050878, 0.6076923076923076428, 0.6102564102564103088, 0.6128205128205128638, 0.6153846153846154188, 0.6179487179487179738, 0.6205128205128205288, 0.6230769230769230838, 0.6256410256410256387, 0.6282051282051281937, 0.6307692307692307487, 0.6333333333333333037, 0.6358974358974358587, 0.6384615384615384137, 0.6410256410256410797, 0.6435897435897436347, 0.6461538461538461897, 0.6487179487179487447, 0.6512820512820512997, 0.6538461538461538547, 0.6564102564102564097, 0.6589743589743589647, 0.6615384615384615197, 0.6641025641025640747, 0.6666666666666666297, 0.6692307692307691847, 0.6717948717948717396, 0.6743589743589744057, 0.6769230769230769607, 0.6794871794871795156, 0.6820512820512820706, 0.6846153846153846256, 0.6871794871794871806, 0.6897435897435897356, 0.6923076923076922906, 0.6948717948717948456, 0.6974358974358974006, 0.6999999999999999556, 0.7025641025641025106, 0.7051282051282051766, 0.7076923076923077316, 0.7102564102564102866, 0.7128205128205128416, 0.7153846153846153966, 0.7179487179487179516, 0.7205128205128205066, 0.7230769230769230616, 0.7256410256410256165, 0.7282051282051281715, 0.7307692307692307265, 0.7333333333333332815, 0.7358974358974359475, 0.7384615384615385025, 0.7410256410256410575, 0.7435897435897436125, 0.7461538461538461675, 0.7487179487179487225, 0.7512820512820512775, 0.7538461538461538325, 0.7564102564102563875, 0.7589743589743589425, 0.7615384615384614975, 0.7641025641025640525, 0.7666666666666667185, 0.7692307692307692735, 0.7717948717948718285, 0.7743589743589743835, 0.7769230769230769384, 0.7794871794871794934, 0.7820512820512820484, 0.7846153846153846034, 0.7871794871794871584, 0.7897435897435897134, 0.7923076923076922684, 0.7948717948717948234, 0.7974358974358974894, 0.8000000000000000444, 0.8025641025641025994, 0.8051282051282051544, 0.8076923076923077094, 0.8102564102564102644, 0.8128205128205128194, 0.8153846153846153744, 0.8179487179487179294, 0.8205128205128204844, 0.8230769230769230393, 0.8256410256410255943, 0.8282051282051282604, 0.8307692307692308153, 0.8333333333333333703, 0.8358974358974359253, 0.8384615384615384803, 0.8410256410256410353, 0.8435897435897435903, 0.8461538461538461453, 0.8487179487179487003, 0.8512820512820512553, 0.8538461538461538103, 0.8564102564102563653, 0.8589743589743589203, 0.8615384615384615863, 0.8641025641025641413, 0.8666666666666666963, 0.8692307692307692513, 0.8717948717948718063, 0.8743589743589743613, 0.8769230769230769162, 0.8794871794871794712, 0.8820512820512820262, 0.8846153846153845812, 0.8871794871794871362, 0.8897435897435896912, 0.8923076923076923572, 0.8948717948717949122, 0.8974358974358974672, 0.9000000000000000222, 0.9025641025641025772, 0.9051282051282051322, 0.9076923076923076872, 0.9102564102564102422, 0.9128205128205127972, 0.9153846153846153522, 0.9179487179487179072, 0.9205128205128204621, 0.9230769230769231282, 0.9256410256410256832, 0.9282051282051282382, 0.9307692307692307931, 0.9333333333333333481, 0.9358974358974359031, 0.9384615384615384581, 0.9410256410256410131, 0.9435897435897435681, 0.9461538461538461231, 0.9487179487179486781, 0.9512820512820512331, 0.9538461538461538991, 0.9564102564102564541, 0.9589743589743590091, 0.9615384615384615641, 0.9641025641025641191, 0.9666666666666666741, 0.9692307692307692291, 0.9717948717948717841, 0.9743589743589743390, 0.9769230769230768940, 0.9794871794871794490, 0.9820512820512820040, 0.9846153846153846700, 0.9871794871794872250, 0.9897435897435897800, 0.9923076923076923350, 0.9948717948717948900, 0.9974358974358974450, 1.000000000000000000 ),
 .UNSPECIFIED. ) 
 GEOMETRIC_REPRESENTATION_ITEM ( )  RATIONAL_B_SPLINE_SURFACE ( (
 ( 1.000000000000000000, 0.9510565162951535312, 1.000000000000000000, 0.9510565162951535312, 1.000000000000000000, 0.9510565162951535312, 1.000000000000000000, 0.9510565162951535312, 1.000000000000000000, 0.9510565162951535312, 1.000000000000000000, 0.9510565162951535312, 1.000000000000000000, 0.9510565162951535312, 1.000000000000000000, 0.9510565162951535312, 1.000000000000000000, 0.9510565162951535312, 1.000000000000000000, 0.9510565162951535312, 1.000000000000000000, 0.9510565162951535312, 1.000000000000000000, 0.9510565162951535312, 1.000000000000000000, 0.9510565162951535312, 1.000000000000000000, 0.9510565162951535312, 1.000000000000000000, 0.9510565162951535312, 1.000000000000000000, 0.9510565162951535312, 1.000000000000000000, 0.9510565162951535312, 1.000000000000000000, 0.9510565162951535312, 1.000000000000000000, 0.9510565162951535312, 1.000000000000000000, 0.9510565162951535312, 1.000000000000000000, 0.9510565162951535312, 1.000000000000000000, 0.9510565162951535312, 1.000000000000000000, 0.9510565162951535312, 1.000000000000000000, 0.9510565162951535312, 1.000000000000000000, 0.9510565162951535312, 1.000000000000000000, 0.9510565162951535312, 1.000000000000000000, 0.9510565162951535312, 1.000000000000000000, 0.9510565162951535312, 1.000000000000000000, 0.9510565162951535312, 1.000000000000000000, 0.9510565162951535312, 1.000000000000000000, 0.9510565162951535312, 1.000000000000000000, 0.9510565162951535312, 1.000000000000000000, 0.9510565162951535312, 1.000000000000000000, 0.9510565162951535312, 1.000000000000000000, 0.9510565162951535312, 1.000000000000000000, 0.9510565162951535312, 1.000000000000000000, 0.9510565162951535312, 1.000000000000000000, 0.9510565162951535312, 1.000000000000000000, 0.9510565162951535312, 1.000000000000000000, 0.9510565162951535312, 1.000000000000000000, 0.9510565162951535312, 1.000000000000000000, 0.9510565162951535312, 1.000000000000000000, 0.9510565162951535312, 1.000000000000000000, 0.9510565162951535312, 1.000000000000000000, 0.9510565162951535312, 1.000000000000000000, 0.9510565162951535312, 1.000000000000000000, 0.9510565162951535312, 1.000000000000000000, 0.9510565162951535312, 1.000000000000000000, 0.9510565162951535312, 1.000000000000000000, 0.9510565162951535312, 1.000000000000000000, 0.9510565162951535312, 1.000000000000000000, 0.9510565162951535312, 1.000000000000000000, 0.9510565162951535312, 1.000000000000000000, 0.9510565162951535312, 1.000000000000000000, 0.9510565162951535312, 1.000000000000000000, 0.9510565162951535312, 1.000000000000000000, 0.9510565162951535312, 1.000000000000000000, 0.9510565162951535312, 1.000000000000000000, 0.9510565162951535312, 1.000000000000000000, 0.9510565162951535312, 1.000000000000000000, 0.9510565162951535312, 1.000000000000000000, 0.9510565162951535312, 1.000000000000000000, 0.9510565162951535312, 1.000000000000000000, 0.9510565162951535312, 1.000000000000000000, 0.9510565162951535312, 1.000000000000000000, 0.9510565162951535312, 1.000000000000000000, 0.9510565162951535312, 1.000000000000000000, 0.9510565162951535312, 1.000000000000000000, 0.9510565162951535312, 1.000000000000000000, 0.9510565162951535312, 1.000000000000000000, 0.9510565162951535312, 1.000000000000000000, 0.9510565162951535312, 1.000000000000000000, 0.9510565162951535312, 1.000000000000000000, 0.9510565162951535312, 1.000000000000000000, 0.9510565162951535312, 1.000000000000000000, 0.9510565162951535312, 1.000000000000000000, 0.9510565162951535312, 1.000000000000000000, 0.9510565162951535312, 1.000000000000000000, 0.9510565162951535312, 1.000000000000000000, 0.9510565162951535312, 1.000000000000000000, 0.9510565162951535312, 1.000000000000000000, 0.9510565162951535312, 1.000000000000000000, 0.9510565162951535312, 1.000000000000000000, 0.9510565162951535312, 1.000000000000000000, 0.9510565162951535312, 1.000000000000000000, 0.9510565162951535312, 1.000000000000000000, 0.9510565162951535312, 1.000000000000000000, 0.9510565162951535312, 1.000000000000000000, 0.9510565162951535312, 1.000000000000000000, 0.9510565162951535312, 1.000000000000000000, 0.9510565162951535312, 1.000000000000000000, 0.9510565162951535312, 1.000000000000000000, 0.9510565162951535312, 1.000000000000000000, 0.9510565162951535312, 1.000000000000000000, 0.9510565162951535312, 1.000000000000000000, 0.9510565162951535312, 1.000000000000000000, 0.9510565162951535312, 1.000000000000000000, 0.9510565162951535312, 1.000000000000000000, 0.9510565162951535312, 1.000000000000000000, 0.9510565162951535312, 1.000000000000000000, 0.9510565162951535312, 1.000000000000000000, 0.9510565162951535312, 1.000000000000000000, 0.9510565162951535312, 1.000000000000000000, 0.9510565162951535312, 1.000000000000000000, 0.9510565162951535312, 1.000000000000000000, 0.9510565162951535312, 1.000000000000000000, 0.9510565162951535312, 1.000000000000000000, 0.9510565162951535312, 1.000000000000000000, 0.9510565162951535312, 1.000000000000000000, 0.9510565162951535312, 1.000000000000000000, 0.9510565162951535312, 1.000000000000000000, 0.9510565162951535312, 1.000000000000000000, 0.9510565162951535312, 1.000000000000000000, 0.9510565162951535312, 1.000000000000000000, 0.9510565162951535312, 1.000000000000000000, 0.9510565162951535312, 1.000000000000000000, 0.9510565162951535312, 1.000000000000000000, 0.9510565162951535312, 1.000000000000000000, 0.9510565162951535312, 1.000000000000000000, 0.9510565162951535312, 1.000000000000000000, 0.9510565162951535312, 1.000000000000000000, 0.9510565162951535312, 1.000000000000000000, 0.9510565162951535312, 1.000000000000000000, 0.9510565162951535312, 1.000000000000000000, 0.9510565162951535312, 1.000000000000000000, 0.9510565162951535312, 1.000000000000000000, 0.9510565162951535312, 1.000000000000000000, 0.9510565162951535312, 1.000000000000000000, 0.9510565162951535312, 1.000000000000000000, 0.9510565162951535312, 1.000000000000000000, 0.9510565162951535312, 1.000000000000000000, 0.9510565162951535312, 1.000000000000000000, 0.9510565162951535312, 1.000000000000000000, 0.9510565162951535312, 1.000000000000000000, 0.9510565162951535312, 1.000000000000000000, 0.9510565162951535312, 1.000000000000000000, 0.9510565162951535312, 1.000000000000000000, 0.9510565162951535312, 1.000000000000000000, 0.9510565162951535312, 1.000000000000000000, 0.9510565162951535312, 1.000000000000000000, 0.9510565162951535312, 1.000000000000000000, 0.9510565162951535312, 1.000000000000000000, 0.9510565162951535312, 1.000000000000000000, 0.9510565162951535312, 1.000000000000000000, 0.9510565162951535312, 1.000000000000000000, 0.9510565162951535312, 1.000000000000000000, 0.9510565162951535312, 1.000000000000000000, 0.9510565162951535312, 1.000000000000000000, 0.9510565162951535312, 1.000000000000000000, 0.9510565162951535312, 1.000000000000000000, 0.9510565162951535312, 1.000000000000000000, 0.9510565162951535312, 1.000000000000000000, 0.9510565162951535312, 1.000000000000000000, 0.9510565162951535312, 1.000000000000000000, 0.9510565162951535312, 1.000000000000000000, 0.9510565162951535312, 1.000000000000000000, 0.9510565162951535312, 1.000000000000000000, 0.9510565162951535312, 1.000000000000000000, 0.9510565162951535312, 1.000000000000000000, 0.9510565162951535312, 1.000000000000000000, 0.9510565162951535312, 1.000000000000000000, 0.9510565162951535312, 1.000000000000000000, 0.9510565162951535312, 1.000000000000000000, 0.9510565162951535312, 1.000000000000000000, 0.9510565162951535312, 1.000000000000000000, 0.9510565162951535312, 1.000000000000000000, 0.9510565162951535312, 1.000000000000000000, 0.9510565162951535312, 1.000000000000000000, 0.9510565162951535312, 1.000000000000000000, 0.9510565162951535312, 1.000000000000000000, 0.9510565162951535312, 1.000000000000000000, 0.9510565162951535312, 1.000000000000000000, 0.9510565162951535312, 1.000000000000000000, 0.9510565162951535312, 1.000000000000000000, 0.9510565162951535312, 1.000000000000000000, 0.9510565162951535312, 1.000000000000000000, 0.9510565162951535312, 1.000000000000000000, 0.9510565162951535312, 1.000000000000000000, 0.9510565162951535312, 1.000000000000000000, 0.9510565162951535312, 1.000000000000000000, 0.9510565162951535312, 1.000000000000000000, 0.9510565162951535312, 1.000000000000000000, 0.9510565162951535312, 1.000000000000000000, 0.9510565162951535312, 1.000000000000000000, 0.9510565162951535312, 1.000000000000000000, 0.9510565162951535312, 1.000000000000000000, 0.9510565162951535312, 1.000000000000000000, 0.9510565162951535312, 1.000000000000000000, 0.9510565162951535312, 1.000000000000000000, 0.9510565162951535312, 1.000000000000000000, 0.9510565162951535312, 1.000000000000000000, 0.9510565162951535312, 1.000000000000000000, 0.9510565162951535312, 1.000000000000000000, 0.9510565162951535312, 1.000000000000000000, 0.9510565162951535312, 1.000000000000000000, 0.9510565162951535312, 1.000000000000000000, 0.9510565162951535312, 1.000000000000000000, 0.9510565162951535312, 1.000000000000000000, 0.9510565162951535312, 1.000000000000000000, 0.9510565162951535312, 1.000000000000000000, 0.9510565162951535312, 1.000000000000000000, 0.9510565162951535312, 1.000000000000000000, 0.9510565162951535312, 1.000000000000000000, 0.9510565162951535312, 1.000000000000000000, 0.9510565162951535312, 1.000000000000000000, 0.9510565162951535312, 1.000000000000000000, 0.9510565162951535312, 1.000000000000000000, 0.9510565162951535312, 1.000000000000000000, 0.9510565162951535312, 1.000000000000000000, 0.9510565162951535312, 1.000000000000000000, 0.9510565162951535312, 1.000000000000000000, 0.9510565162951535312, 1.000000000000000000, 0.9510565162951535312, 1.000000000000000000, 0.9510565162951535312, 1.000000000000000000, 0.9510565162951535312, 1.000000000000000000, 0.9510565162951535312, 1.000000000000000000, 0.9510565162951535312, 1.000000000000000000, 0.9510565162951535312, 1.000000000000000000, 0.9510565162951535312, 1.000000000000000000, 0.9510565162951535312, 1.000000000000000000, 0.9510565162951535312, 1.000000000000000000, 0.9510565162951535312, 1.000000000000000000, 0.9510565162951535312, 1.000000000000000000, 0.9510565162951535312, 1.000000000000000000, 0.9510565162951535312, 1.000000000000000000, 0.9510565162951535312, 1.000000000000000000, 0.9510565162951535312, 1.000000000000000000, 0.9510565162951535312, 1.000000000000000000, 0.9510565162951535312, 1.000000000000000000, 0.9510565162951535312, 1.000000000000000000, 0.9510565162951535312, 1.000000000000000000, 0.9510565162951535312, 1.000000000000000000, 0.9510565162951535312, 1.000000000000000000, 0.9510565162951535312, 1.000000000000000000, 0.9510565162951535312, 1.000000000000000000, 0.9510565162951535312, 1.000000000000000000, 0.9510565162951535312, 1.000000000000000000, 0.9510565162951535312, 1.000000000000000000, 0.9510565162951535312, 1.000000000000000000, 0.9510565162951535312, 1.000000000000000000, 0.9510565162951535312, 1.000000000000000000, 0.9510565162951535312, 1.000000000000000000, 0.9510565162951535312, 1.000000000000000000, 0.9510565162951535312, 1.000000000000000000, 0.9510565162951535312, 1.000000000000000000, 0.9510565162951535312, 1.000000000000000000, 0.9510565162951535312, 1.000000000000000000, 0.9510565162951535312, 1.000000000000000000, 0.9510565162951535312, 1.000000000000000000, 0.9510565162951535312, 1.000000000000000000, 0.9510565162951535312, 1.000000000000000000, 0.9510565162951535312, 1.000000000000000000, 0.9510565162951535312, 1.000000000000000000, 0.9510565162951535312, 1.000000000000000000, 0.9510565162951535312, 1.000000000000000000, 0.9510565162951535312, 1.000000000000000000, 0.9510565162951535312, 1.000000000000000000, 0.9510565162951535312, 1.000000000000000000, 0.9510565162951535312, 1.000000000000000000, 0.9510565162951535312, 1.000000000000000000, 0.9510565162951535312, 1.000000000000000000, 0.9510565162951535312, 1.000000000000000000, 0.9510565162951535312, 1.000000000000000000, 0.9510565162951535312, 1.000000000000000000, 0.9510565162951535312, 1.000000000000000000, 0.9510565162951535312, 1.000000000000000000, 0.9510565162951535312, 1.000000000000000000, 0.9510565162951535312, 1.000000000000000000, 0.9510565162951535312, 1.000000000000000000, 0.9510565162951535312, 1.000000000000000000, 0.9510565162951535312, 1.000000000000000000, 0.9510565162951535312, 1.000000000000000000, 0.9510565162951535312, 1.000000000000000000, 0.9510565162951535312, 1.000000000000000000, 0.9510565162951535312, 1.000000000000000000, 0.9510565162951535312, 1.000000000000000000, 0.9510565162951535312, 1.000000000000000000, 0.9510565162951535312, 1.000000000000000000, 0.9510565162951535312, 1.000000000000000000, 0.9510565162951535312, 1.000000000000000000, 0.9510565162951535312, 1.000000000000000000, 0.9510565162951535312, 1.000000000000000000, 0.9510565162951535312, 1.000000000000000000, 0.9510565162951535312, 1.000000000000000000, 0.9510565162951535312, 1.000000000000000000, 0.9510565162951535312, 1.000000000000000000, 0.9510565162951535312, 1.000000000000000000, 0.9510565162951535312, 1.000000000000000000, 0.9510565162951535312, 1.000000000000000000, 0.9510565162951535312, 1.000000000000000000, 0.9510565162951535312, 1.000000000000000000, 0.9510565162951535312, 1.000000000000000000, 0.9510565162951535312, 1.000000000000000000, 0.9510565162951535312, 1.000000000000000000, 0.9510565162951535312, 1.000000000000000000, 0.9510565162951535312, 1.000000000000000000, 0.9510565162951535312, 1.000000000000000000, 0.9510565162951535312, 1.000000000000000000, 0.9510565162951535312, 1.000000000000000000, 0.9510565162951535312, 1.000000000000000000, 0.9510565162951535312, 1.000000000000000000, 0.9510565162951535312, 1.000000000000000000, 0.9510565162951535312, 1.000000000000000000, 0.9510565162951535312, 1.000000000000000000, 0.9510565162951535312, 1.000000000000000000, 0.9510565162951535312, 1.000000000000000000, 0.9510565162951535312, 1.000000000000000000, 0.9510565162951535312, 1.000000000000000000, 0.9510565162951535312, 1.000000000000000000, 0.9510565162951535312, 1.000000000000000000, 0.9510565162951535312, 1.000000000000000000, 0.9510565162951535312, 1.000000000000000000, 0.9510565162951535312, 1.000000000000000000, 0.9510565162951535312, 1.000000000000000000, 0.9510565162951535312, 1.000000000000000000, 0.9510565162951535312, 1.000000000000000000, 0.9510565162951535312, 1.000000000000000000, 0.9510565162951535312, 1.000000000000000000, 0.9510565162951535312, 1.000000000000000000, 0.9510565162951535312, 1.000000000000000000, 0.9510565162951535312, 1.000000000000000000, 0.9510565162951535312, 1.000000000000000000, 0.9510565162951535312, 1.000000000000000000, 0.9510565162951535312, 1.000000000000000000, 0.9510565162951535312, 1.000000000000000000, 0.9510565162951535312, 1.000000000000000000, 0.9510565162951535312, 1.000000000000000000, 0.9510565162951535312, 1.000000000000000000, 0.9510565162951535312, 1.000000000000000000, 0.9510565162951535312, 1.000000000000000000, 0.9510565162951535312, 1.000000000000000000, 0.9510565162951535312, 1.000000000000000000, 0.9510565162951535312, 1.000000000000000000, 0.9510565162951535312, 1.000000000000000000, 0.9510565162951535312, 1.000000000000000000, 0.9510565162951535312, 1.000000000000000000, 0.9510565162951535312, 1.000000000000000000, 0.9510565162951535312, 1.000000000000000000, 0.9510565162951535312, 1.000000000000000000, 0.9510565162951535312, 1.000000000000000000, 0.9510565162951535312, 1.000000000000000000, 0.9510565162951535312, 1.000000000000000000, 0.9510565162951535312, 1.000000000000000000, 0.9510565162951535312, 1.000000000000000000, 0.9510565162951535312, 1.000000000000000000, 0.9510565162951535312, 1.000000000000000000, 0.9510565162951535312, 1.000000000000000000, 0.9510565162951535312, 1.000000000000000000, 0.9510565162951535312, 1.000000000000000000, 0.9510565162951535312, 1.000000000000000000, 0.9510565162951535312, 1.000000000000000000, 0.9510565162951535312, 1.000000000000000000, 0.9510565162951535312, 1.000000000000000000, 0.9510565162951535312, 1.000000000000000000, 0.9510565162951535312, 1.000000000000000000, 0.9510565162951535312, 1.000000000000000000, 0.9510565162951535312, 1.000000000000000000, 0.9510565162951535312, 1.000000000000000000, 0.9510565162951535312, 1.000000000000000000, 0.9510565162951535312, 1.000000000000000000, 0.9510565162951535312, 1.000000000000000000, 0.9510565162951535312, 1.000000000000000000, 0.9510565162951535312, 1.000000000000000000, 0.9510565162951535312, 1.000000000000000000, 0.9510565162951535312, 1.000000000000000000, 0.9510565162951535312, 1.000000000000000000, 0.9510565162951535312, 1.000000000000000000, 0.9510565162951535312, 1.000000000000000000, 0.9510565162951535312, 1.000000000000000000, 0.9510565162951535312, 1.000000000000000000, 0.9510565162951535312, 1.000000000000000000, 0.9510565162951535312, 1.000000000000000000, 0.9510565162951535312, 1.000000000000000000, 0.9510565162951535312, 1.000000000000000000, 0.9510565162951535312, 1.000000000000000000, 0.9510565162951535312, 1.000000000000000000, 0.9510565162951535312, 1.000000000000000000, 0.9510565162951535312, 1.000000000000000000, 0.9510565162951535312, 1.000000000000000000, 0.9510565162951535312, 1.000000000000000000, 0.9510565162951535312, 1.000000000000000000, 0.9510565162951535312, 1.000000000000000000, 0.9510565162951535312, 1.000000000000000000, 0.9510565162951535312, 1.000000000000000000, 0.9510565162951535312, 1.000000000000000000, 0.9510565162951535312, 1.000000000000000000, 0.9510565162951535312, 1.000000000000000000, 0.9510565162951535312, 1.000000000000000000, 0.9510565162951535312, 1.000000000000000000, 0.9510565162951535312, 1.000000000000000000),
 ( 1.000000000000000000, 0.9510565162951535312, 1.000000000000000000, 0.9510565162951535312, 1.000000000000000000, 0.9510565162951535312, 1.000000000000000000, 0.9510565162951535312, 1.000000000000000000, 0.9510565162951535312, 1.000000000000000000, 0.9510565162951535312, 1.000000000000000000, 0.9510565162951535312, 1.000000000000000000, 0.9510565162951535312, 1.000000000000000000, 0.9510565162951535312, 1.000000000000000000, 0.9510565162951535312, 1.000000000000000000, 0.9510565162951535312, 1.000000000000000000, 0.9510565162951535312, 1.000000000000000000, 0.9510565162951535312, 1.000000000000000000, 0.9510565162951535312, 1.000000000000000000, 0.9510565162951535312, 1.000000000000000000, 0.9510565162951535312, 1.000000000000000000, 0.9510565162951535312, 1.000000000000000000, 0.9510565162951535312, 1.000000000000000000, 0.9510565162951535312, 1.000000000000000000, 0.9510565162951535312, 1.000000000000000000, 0.9510565162951535312, 1.000000000000000000, 0.9510565162951535312, 1.000000000000000000, 0.9510565162951535312, 1.000000000000000000, 0.9510565162951535312, 1.000000000000000000, 0.9510565162951535312, 1.000000000000000000, 0.9510565162951535312, 1.000000000000000000, 0.9510565162951535312, 1.000000000000000000, 0.9510565162951535312, 1.000000000000000000, 0.9510565162951535312, 1.000000000000000000, 0.9510565162951535312, 1.000000000000000000, 0.9510565162951535312, 1.000000000000000000, 0.9510565162951535312, 1.000000000000000000, 0.9510565162951535312, 1.000000000000000000, 0.9510565162951535312, 1.000000000000000000, 0.9510565162951535312, 1.000000000000000000, 0.9510565162951535312, 1.000000000000000000, 0.9510565162951535312, 1.000000000000000000, 0.9510565162951535312, 1.000000000000000000, 0.9510565162951535312, 1.000000000000000000, 0.9510565162951535312, 1.000000000000000000, 0.9510565162951535312, 1.000000000000000000, 0.9510565162951535312, 1.000000000000000000, 0.9510565162951535312, 1.000000000000000000, 0.9510565162951535312, 1.000000000000000000, 0.9510565162951535312, 1.000000000000000000, 0.9510565162951535312, 1.000000000000000000, 0.9510565162951535312, 1.000000000000000000, 0.9510565162951535312, 1.000000000000000000, 0.9510565162951535312, 1.000000000000000000, 0.9510565162951535312, 1.000000000000000000, 0.9510565162951535312, 1.000000000000000000, 0.9510565162951535312, 1.000000000000000000, 0.9510565162951535312, 1.000000000000000000, 0.9510565162951535312, 1.000000000000000000, 0.9510565162951535312, 1.000000000000000000, 0.9510565162951535312, 1.000000000000000000, 0.9510565162951535312, 1.000000000000000000, 0.9510565162951535312, 1.000000000000000000, 0.9510565162951535312, 1.000000000000000000, 0.9510565162951535312, 1.000000000000000000, 0.9510565162951535312, 1.000000000000000000, 0.9510565162951535312, 1.000000000000000000, 0.9510565162951535312, 1.000000000000000000, 0.9510565162951535312, 1.000000000000000000, 0.9510565162951535312, 1.000000000000000000, 0.9510565162951535312, 1.000000000000000000, 0.9510565162951535312, 1.000000000000000000, 0.9510565162951535312, 1.000000000000000000, 0.9510565162951535312, 1.000000000000000000, 0.9510565162951535312, 1.000000000000000000, 0.9510565162951535312, 1.000000000000000000, 0.9510565162951535312, 1.000000000000000000, 0.9510565162951535312, 1.000000000000000000, 0.9510565162951535312, 1.000000000000000000, 0.9510565162951535312, 1.000000000000000000, 0.9510565162951535312, 1.000000000000000000, 0.9510565162951535312, 1.000000000000000000, 0.9510565162951535312, 1.000000000000000000, 0.9510565162951535312, 1.000000000000000000, 0.9510565162951535312, 1.000000000000000000, 0.9510565162951535312, 1.000000000000000000, 0.9510565162951535312, 1.000000000000000000, 0.9510565162951535312, 1.000000000000000000, 0.9510565162951535312, 1.000000000000000000, 0.9510565162951535312, 1.000000000000000000, 0.9510565162951535312, 1.000000000000000000, 0.9510565162951535312, 1.000000000000000000, 0.9510565162951535312, 1.000000000000000000, 0.9510565162951535312, 1.000000000000000000, 0.9510565162951535312, 1.000000000000000000, 0.9510565162951535312, 1.000000000000000000, 0.9510565162951535312, 1.000000000000000000, 0.9510565162951535312, 1.000000000000000000, 0.9510565162951535312, 1.000000000000000000, 0.9510565162951535312, 1.000000000000000000, 0.9510565162951535312, 1.000000000000000000, 0.9510565162951535312, 1.000000000000000000, 0.9510565162951535312, 1.000000000000000000, 0.9510565162951535312, 1.000000000000000000, 0.9510565162951535312, 1.000000000000000000, 0.9510565162951535312, 1.000000000000000000, 0.9510565162951535312, 1.000000000000000000, 0.9510565162951535312, 1.000000000000000000, 0.9510565162951535312, 1.000000000000000000, 0.9510565162951535312, 1.000000000000000000, 0.9510565162951535312, 1.000000000000000000, 0.9510565162951535312, 1.000000000000000000, 0.9510565162951535312, 1.000000000000000000, 0.9510565162951535312, 1.000000000000000000, 0.9510565162951535312, 1.000000000000000000, 0.9510565162951535312, 1.000000000000000000, 0.9510565162951535312, 1.000000000000000000, 0.9510565162951535312, 1.000000000000000000, 0.9510565162951535312, 1.000000000000000000, 0.9510565162951535312, 1.000000000000000000, 0.9510565162951535312, 1.000000000000000000, 0.9510565162951535312, 1.000000000000000000, 0.9510565162951535312, 1.000000000000000000, 0.9510565162951535312, 1.000000000000000000, 0.9510565162951535312, 1.000000000000000000, 0.9510565162951535312, 1.000000000000000000, 0.9510565162951535312, 1.000000000000000000, 0.9510565162951535312, 1.000000000000000000, 0.9510565162951535312, 1.000000000000000000, 0.9510565162951535312, 1.000000000000000000, 0.9510565162951535312, 1.000000000000000000, 0.9510565162951535312, 1.000000000000000000, 0.9510565162951535312, 1.000000000000000000, 0.9510565162951535312, 1.000000000000000000, 0.9510565162951535312, 1.000000000000000000, 0.9510565162951535312, 1.000000000000000000, 0.9510565162951535312, 1.000000000000000000, 0.9510565162951535312, 1.000000000000000000, 0.9510565162951535312, 1.000000000000000000, 0.9510565162951535312, 1.000000000000000000, 0.9510565162951535312, 1.000000000000000000, 0.9510565162951535312, 1.000000000000000000, 0.9510565162951535312, 1.000000000000000000, 0.9510565162951535312, 1.000000000000000000, 0.9510565162951535312, 1.000000000000000000, 0.9510565162951535312, 1.000000000000000000, 0.9510565162951535312, 1.000000000000000000, 0.9510565162951535312, 1.000000000000000000, 0.9510565162951535312, 1.000000000000000000, 0.9510565162951535312, 1.000000000000000000, 0.9510565162951535312, 1.000000000000000000, 0.9510565162951535312, 1.000000000000000000, 0.9510565162951535312, 1.000000000000000000, 0.9510565162951535312, 1.000000000000000000, 0.9510565162951535312, 1.000000000000000000, 0.9510565162951535312, 1.000000000000000000, 0.9510565162951535312, 1.000000000000000000, 0.9510565162951535312, 1.000000000000000000, 0.9510565162951535312, 1.000000000000000000, 0.9510565162951535312, 1.000000000000000000, 0.9510565162951535312, 1.000000000000000000, 0.9510565162951535312, 1.000000000000000000, 0.9510565162951535312, 1.000000000000000000, 0.9510565162951535312, 1.000000000000000000, 0.9510565162951535312, 1.000000000000000000, 0.9510565162951535312, 1.000000000000000000, 0.9510565162951535312, 1.000000000000000000, 0.9510565162951535312, 1.000000000000000000, 0.9510565162951535312, 1.000000000000000000, 0.9510565162951535312, 1.000000000000000000, 0.9510565162951535312, 1.000000000000000000, 0.9510565162951535312, 1.000000000000000000, 0.9510565162951535312, 1.000000000000000000, 0.9510565162951535312, 1.000000000000000000, 0.9510565162951535312, 1.000000000000000000, 0.9510565162951535312, 1.000000000000000000, 0.9510565162951535312, 1.000000000000000000, 0.9510565162951535312, 1.000000000000000000, 0.9510565162951535312, 1.000000000000000000, 0.9510565162951535312, 1.000000000000000000, 0.9510565162951535312, 1.000000000000000000, 0.9510565162951535312, 1.000000000000000000, 0.9510565162951535312, 1.000000000000000000, 0.9510565162951535312, 1.000000000000000000, 0.9510565162951535312, 1.000000000000000000, 0.9510565162951535312, 1.000000000000000000, 0.9510565162951535312, 1.000000000000000000, 0.9510565162951535312, 1.000000000000000000, 0.9510565162951535312, 1.000000000000000000, 0.9510565162951535312, 1.000000000000000000, 0.9510565162951535312, 1.000000000000000000, 0.9510565162951535312, 1.000000000000000000, 0.9510565162951535312, 1.000000000000000000, 0.9510565162951535312, 1.000000000000000000, 0.9510565162951535312, 1.000000000000000000, 0.9510565162951535312, 1.000000000000000000, 0.9510565162951535312, 1.000000000000000000, 0.9510565162951535312, 1.000000000000000000, 0.9510565162951535312, 1.000000000000000000, 0.9510565162951535312, 1.000000000000000000, 0.9510565162951535312, 1.000000000000000000, 0.9510565162951535312, 1.000000000000000000, 0.9510565162951535312, 1.000000000000000000, 0.9510565162951535312, 1.000000000000000000, 0.9510565162951535312, 1.000000000000000000, 0.9510565162951535312, 1.000000000000000000, 0.9510565162951535312, 1.000000000000000000, 0.9510565162951535312, 1.000000000000000000, 0.9510565162951535312, 1.000000000000000000, 0.9510565162951535312, 1.000000000000000000, 0.9510565162951535312, 1.000000000000000000, 0.9510565162951535312, 1.000000000000000000, 0.9510565162951535312, 1.000000000000000000, 0.9510565162951535312, 1.000000000000000000, 0.9510565162951535312, 1.000000000000000000, 0.9510565162951535312, 1.000000000000000000, 0.9510565162951535312, 1.000000000000000000, 0.9510565162951535312, 1.000000000000000000, 0.9510565162951535312, 1.000000000000000000, 0.9510565162951535312, 1.000000000000000000, 0.9510565162951535312, 1.000000000000000000, 0.9510565162951535312, 1.000000000000000000, 0.9510565162951535312, 1.000000000000000000, 0.9510565162951535312, 1.000000000000000000, 0.9510565162951535312, 1.000000000000000000, 0.9510565162951535312, 1.000000000000000000, 0.9510565162951535312, 1.000000000000000000, 0.9510565162951535312, 1.000000000000000000, 0.9510565162951535312, 1.000000000000000000, 0.9510565162951535312, 1.000000000000000000, 0.9510565162951535312, 1.000000000000000000, 0.9510565162951535312, 1.000000000000000000, 0.9510565162951535312, 1.000000000000000000, 0.9510565162951535312, 1.000000000000000000, 0.9510565162951535312, 1.000000000000000000, 0.9510565162951535312, 1.000000000000000000, 0.9510565162951535312, 1.000000000000000000, 0.9510565162951535312, 1.000000000000000000, 0.9510565162951535312, 1.000000000000000000, 0.9510565162951535312, 1.000000000000000000, 0.9510565162951535312, 1.000000000000000000, 0.9510565162951535312, 1.000000000000000000, 0.9510565162951535312, 1.000000000000000000, 0.9510565162951535312, 1.000000000000000000, 0.9510565162951535312, 1.000000000000000000, 0.9510565162951535312, 1.000000000000000000, 0.9510565162951535312, 1.000000000000000000, 0.9510565162951535312, 1.000000000000000000, 0.9510565162951535312, 1.000000000000000000, 0.9510565162951535312, 1.000000000000000000, 0.9510565162951535312, 1.000000000000000000, 0.9510565162951535312, 1.000000000000000000, 0.9510565162951535312, 1.000000000000000000, 0.9510565162951535312, 1.000000000000000000, 0.9510565162951535312, 1.000000000000000000, 0.9510565162951535312, 1.000000000000000000, 0.9510565162951535312, 1.000000000000000000, 0.9510565162951535312, 1.000000000000000000, 0.9510565162951535312, 1.000000000000000000, 0.9510565162951535312, 1.000000000000000000, 0.9510565162951535312, 1.000000000000000000, 0.9510565162951535312, 1.000000000000000000, 0.9510565162951535312, 1.000000000000000000, 0.9510565162951535312, 1.000000000000000000, 0.9510565162951535312, 1.000000000000000000, 0.9510565162951535312, 1.000000000000000000, 0.9510565162951535312, 1.000000000000000000, 0.9510565162951535312, 1.000000000000000000, 0.9510565162951535312, 1.000000000000000000, 0.9510565162951535312, 1.000000000000000000, 0.9510565162951535312, 1.000000000000000000, 0.9510565162951535312, 1.000000000000000000, 0.9510565162951535312, 1.000000000000000000, 0.9510565162951535312, 1.000000000000000000, 0.9510565162951535312, 1.000000000000000000, 0.9510565162951535312, 1.000000000000000000, 0.9510565162951535312, 1.000000000000000000, 0.9510565162951535312, 1.000000000000000000, 0.9510565162951535312, 1.000000000000000000, 0.9510565162951535312, 1.000000000000000000, 0.9510565162951535312, 1.000000000000000000, 0.9510565162951535312, 1.000000000000000000, 0.9510565162951535312, 1.000000000000000000, 0.9510565162951535312, 1.000000000000000000, 0.9510565162951535312, 1.000000000000000000, 0.9510565162951535312, 1.000000000000000000, 0.9510565162951535312, 1.000000000000000000, 0.9510565162951535312, 1.000000000000000000, 0.9510565162951535312, 1.000000000000000000, 0.9510565162951535312, 1.000000000000000000, 0.9510565162951535312, 1.000000000000000000, 0.9510565162951535312, 1.000000000000000000, 0.9510565162951535312, 1.000000000000000000, 0.9510565162951535312, 1.000000000000000000, 0.9510565162951535312, 1.000000000000000000, 0.9510565162951535312, 1.000000000000000000, 0.9510565162951535312, 1.000000000000000000, 0.9510565162951535312, 1.000000000000000000, 0.9510565162951535312, 1.000000000000000000, 0.9510565162951535312, 1.000000000000000000, 0.9510565162951535312, 1.000000000000000000, 0.9510565162951535312, 1.000000000000000000, 0.9510565162951535312, 1.000000000000000000, 0.9510565162951535312, 1.000000000000000000, 0.9510565162951535312, 1.000000000000000000, 0.9510565162951535312, 1.000000000000000000, 0.9510565162951535312, 1.000000000000000000, 0.9510565162951535312, 1.000000000000000000, 0.9510565162951535312, 1.000000000000000000, 0.9510565162951535312, 1.000000000000000000, 0.9510565162951535312, 1.000000000000000000, 0.9510565162951535312, 1.000000000000000000, 0.9510565162951535312, 1.000000000000000000, 0.9510565162951535312, 1.000000000000000000, 0.9510565162951535312, 1.000000000000000000, 0.9510565162951535312, 1.000000000000000000, 0.9510565162951535312, 1.000000000000000000, 0.9510565162951535312, 1.000000000000000000, 0.9510565162951535312, 1.000000000000000000, 0.9510565162951535312, 1.000000000000000000, 0.9510565162951535312, 1.000000000000000000, 0.9510565162951535312, 1.000000000000000000, 0.9510565162951535312, 1.000000000000000000, 0.9510565162951535312, 1.000000000000000000, 0.9510565162951535312, 1.000000000000000000, 0.9510565162951535312, 1.000000000000000000, 0.9510565162951535312, 1.000000000000000000, 0.9510565162951535312, 1.000000000000000000, 0.9510565162951535312, 1.000000000000000000, 0.9510565162951535312, 1.000000000000000000, 0.9510565162951535312, 1.000000000000000000, 0.9510565162951535312, 1.000000000000000000, 0.9510565162951535312, 1.000000000000000000, 0.9510565162951535312, 1.000000000000000000, 0.9510565162951535312, 1.000000000000000000, 0.9510565162951535312, 1.000000000000000000, 0.9510565162951535312, 1.000000000000000000, 0.9510565162951535312, 1.000000000000000000, 0.9510565162951535312, 1.000000000000000000, 0.9510565162951535312, 1.000000000000000000, 0.9510565162951535312, 1.000000000000000000, 0.9510565162951535312, 1.000000000000000000, 0.9510565162951535312, 1.000000000000000000, 0.9510565162951535312, 1.000000000000000000, 0.9510565162951535312, 1.000000000000000000, 0.9510565162951535312, 1.000000000000000000, 0.9510565162951535312, 1.000000000000000000, 0.9510565162951535312, 1.000000000000000000, 0.9510565162951535312, 1.000000000000000000, 0.9510565162951535312, 1.000000000000000000, 0.9510565162951535312, 1.000000000000000000, 0.9510565162951535312, 1.000000000000000000, 0.9510565162951535312, 1.000000000000000000, 0.9510565162951535312, 1.000000000000000000, 0.9510565162951535312, 1.000000000000000000, 0.9510565162951535312, 1.000000000000000000, 0.9510565162951535312, 1.000000000000000000, 0.9510565162951535312, 1.000000000000000000, 0.9510565162951535312, 1.000000000000000000, 0.9510565162951535312, 1.000000000000000000, 0.9510565162951535312, 1.000000000000000000, 0.9510565162951535312, 1.000000000000000000, 0.9510565162951535312, 1.000000000000000000, 0.9510565162951535312, 1.000000000000000000, 0.9510565162951535312, 1.000000000000000000, 0.9510565162951535312, 1.000000000000000000, 0.9510565162951535312, 1.000000000000000000, 0.9510565162951535312, 1.000000000000000000, 0.9510565162951535312, 1.000000000000000000, 0.9510565162951535312, 1.000000000000000000, 0.9510565162951535312, 1.000000000000000000, 0.9510565162951535312, 1.000000000000000000, 0.9510565162951535312, 1.000000000000000000, 0.9510565162951535312, 1.000000000000000000, 0.9510565162951535312, 1.000000000000000000, 0.9510565162951535312, 1.000000000000000000, 0.9510565162951535312, 1.000000000000000000, 0.9510565162951535312, 1.000000000000000000, 0.9510565162951535312, 1.000000000000000000, 0.9510565162951535312, 1.000000000000000000, 0.9510565162951535312, 1.000000000000000000, 0.9510565162951535312, 1.000000000000000000, 0.9510565162951535312, 1.000000000000000000, 0.9510565162951535312, 1.000000000000000000, 0.9510565162951535312, 1.000000000000000000, 0.9510565162951535312, 1.000000000000000000, 0.9510565162951535312, 1.000000000000000000, 0.9510565162951535312, 1.000000000000000000, 0.9510565162951535312, 1.000000000000000000, 0.9510565162951535312, 1.000000000000000000, 0.9510565162951535312, 1.000000000000000000, 0.9510565162951535312, 1.000000000000000000, 0.9510565162951535312, 1.000000000000000000, 0.9510565162951535312, 1.000000000000000000, 0.9510565162951535312, 1.000000000000000000) ) ) 
 REPRESENTATION_ITEM ( '' )  SURFACE ( )  );
#9915=CARTESIAN_POINT ( 'NONE',  ( 26.29305231718578995, 9.199999999999985079, -19.10302069950538240 ) ) ;
#9916=CARTESIAN_POINT ( 'NONE',  ( -10.04305231718578462, 52.40000000000000568, 30.90933677959249337 ) ) ;
#9918=CARTESIAN_POINT ( 'NONE',  ( 20.75514604977248467, 48.42500000273119554, -28.56700777964554305 ) ) ;
#9920=CARTESIAN_POINT ( 'NONE',  ( -10.37757302488623701, 39.77500000273118275, 31.93888565452638417 ) ) ;
#9923=CARTESIAN_POINT ( 'NONE',  ( 3.980102097228898626E-15, 80.00000000000001421, 32.50000000000000000 ) ) ;
#9927=CARTESIAN_POINT ( 'NONE',  ( 0.000000000000000000, 0.000000000000000000, 0.000000000000000000 ) ) ;
#9932=CARTESIAN_POINT ( 'NONE',  ( 2.375766604868046361, 70.80125428700921475, 14.99999999999999822 ) ) ;
#9933=CARTESIAN_POINT ( 'NONE',  ( -10.37757302488624411, 24.72500000273119980, -31.93888565452638417 ) ) ;
#9934=VECTOR ( 'NONE', #23299, 1000.000000000000114 ) ;
#9935=CIRCLE ( 'NONE', #615, 15.00000000000000000 ) ;
#9941=ORIENTED_EDGE ( 'NONE', *, *, #31376, .F. ) ;
#9944=EDGE_LOOP ( 'NONE', ( #26661, #20370, #11655, #31715 ) ) ;
#9947=CARTESIAN_POINT ( 'NONE',  ( -5.147494310547430452, 46.05125428700922896, -32.49999999999999289 ) ) ;
#9948=CARTESIAN_POINT ( 'NONE',  ( -10.37757302488623701, 31.77500000273120051, 31.93888565452638417 ) ) ;
#9949=CARTESIAN_POINT ( 'NONE',  ( -32.50000000000000000, 46.40000000546238113, -10.55989012756945478 ) ) ;
#9950=EDGE_CURVE ( 'NONE', #33526, #16018, #8865, .T. ) ;
#9952=CARTESIAN_POINT ( 'NONE',  ( 33.58253175000000113, 24.22500000273119625, -10.91162601494193751 ) ) ;
#9953=CARTESIAN_POINT ( 'NONE',  ( 20.08610463437157279, 31.80000000546236905, -27.64615127144129758 ) ) ;
#9954=CARTESIAN_POINT ( 'NONE',  ( 10.37757302488624767, 47.97500000273119269, 31.93888565452638417 ) ) ;
#9956=CARTESIAN_POINT ( 'NONE',  ( -2.092463501923844636E-15, 27.50000000000000355, -34.17252228774368916 ) ) ;
#9958=CARTESIAN_POINT ( 'NONE',  ( 33.58253175000000823, 74.02500000273120406, 10.91162601494192863 ) ) ;
#9962=CARTESIAN_POINT ( 'NONE',  ( 10.37757302488624056, 58.77500000273119696, -31.93888565452638417 ) ) ;
#9965=CARTESIAN_POINT ( 'NONE',  ( -33.58253175000000113, 21.22500000273117848, 10.91162601494193929 ) ) ;
#9966=CARTESIAN_POINT ( 'NONE',  ( 7.570916362186207671, 9.349999994537617098, 23.30088464923126779 ) ) ;
#9968=CARTESIAN_POINT ( 'NONE',  ( -32.50000000000000000, 25.99999999999999645, 0.000000000000000000 ) ) ;
#9970=DIRECTION ( 'NONE',  ( -0.000000000000000000, -1.000000000000000000, -0.000000000000000000 ) ) ;
#9980=CARTESIAN_POINT ( 'NONE',  ( 32.50000000000000711, 63.40000000546236691, 10.55989012756945122 ) ) ;
#9981=EDGE_CURVE ( 'NONE', #8583, #27363, #26420, .T. ) ;
#9982=CARTESIAN_POINT ( 'NONE',  ( 26.29305231718578995, 77.70000000546239960, -19.10302069950538240 ) ) ;
#9985=( BOUNDED_CURVE ( )  B_SPLINE_CURVE ( 2, ( #17690, #23175, #2059, #28653, #12361, #20094, #28150, #30539, #12535, #25915, #7035, #9787, #12876 ),
 .UNSPECIFIED., .F., .T. ) 
 B_SPLINE_CURVE_WITH_KNOTS ( ( 3, 2, 2, 2, 2, 2, 3 ),
 ( 0.7371794871794872250, 0.7384615384615385025, 0.7410256410256410575, 0.7435897435897436125, 0.7461538461538461675, 0.7487179487179487225, 0.7500000000000000000 ),
 .UNSPECIFIED. ) 
 CURVE ( )  GEOMETRIC_REPRESENTATION_ITEM ( )  RATIONAL_B_SPLINE_CURVE ( ( 0.9755282581475768211, 0.9755282581475768211, 1.000000000000000000, 0.9510565162951535312, 1.000000000000000000, 0.9510565162951535312, 1.000000000000000000, 0.9510565162951535312, 1.000000000000000000, 0.9510565162951535312, 1.000000000000000000, 0.9755282581475768211, 0.9755282581475768211 ) ) 
 REPRESENTATION_ITEM ( '' )  );
#9987=ORIENTED_EDGE ( 'NONE', *, *, #8784, .T. ) ;
#9988=CARTESIAN_POINT ( 'NONE',  ( 6.486482029760649416E-15, 73.87500000273119838, 35.31076352940723240 ) ) ;
#9990=EDGE_CURVE ( 'NONE', #1219, #684, #4504, .T. ) ;
#9992=CARTESIAN_POINT ( 'NONE',  ( 10.04305231718579705, 61.10000000546239818, 30.90933677959248982 ) ) ;
#9995=CARTESIAN_POINT ( 'NONE',  ( -33.58253175000000113, 39.12500000273119838, 0.000000000000000000 ) ) ;
#9996=CARTESIAN_POINT ( 'NONE',  ( 7.236395654485760609, 15.02499999726880731, -22.27133577429736633 ) ) ;
#9997=CARTESIAN_POINT ( 'NONE',  ( -27.16883889988623935, 71.57500000273120122, 19.73931689729374739 ) ) ;
#9998=CARTESIAN_POINT ( 'NONE',  ( -10.04305231718579172, 4.100000005462373309, -30.90933677959248982 ) ) ;
#9999=EDGE_CURVE ( 'NONE', #23029, #5175, #2762, .T. ) ;
#10002=CARTESIAN_POINT ( 'NONE',  ( 10.04305231718579705, 48.60000000000000142, 30.90933677959248982 ) ) ;
#10003=CARTESIAN_POINT ( 'NONE',  ( -26.29305231718579350, 13.79999999999997939, -19.10302069950537884 ) ) ;
#10004=CARTESIAN_POINT ( 'NONE',  ( 27.16883889988623935, 18.57500000273118346, -19.73931689729374384 ) ) ;
#10005=AXIS2_PLACEMENT_3D ( 'NONE', #22133, #33081, #12672 ) ;
#10006=CARTESIAN_POINT ( 'NONE',  ( 3.445340210940985210E-14, 7.499999999999994671, 24.50000000000000000 ) ) ;
#10008=CARTESIAN_POINT ( 'NONE',  ( -11.25946833292375793, 81.17500000273119554, -8.180482586598733619 ) ) ;
#10009=CARTESIAN_POINT ( 'NONE',  ( -1.778240108872766143E-15, 42.00000000546236834, -32.49999999999999289 ) ) ;
#10010=CARTESIAN_POINT ( 'NONE',  ( -1.778240108872766143E-15, 43.50000000000000000, -32.49999999999999289 ) ) ;
#10024=CARTESIAN_POINT ( 'NONE',  ( -4.300734207923755825, 73.77500000273118985, 13.23629886949340673 ) ) ;
#10026=CARTESIAN_POINT ( 'NONE',  ( -20.75514604977248112, 47.42500000273119554, 28.56700777964554661 ) ) ;
#10031=DIRECTION ( 'NONE',  ( -0.000000000000000000, 1.000000000000000000, -0.000000000000000000 ) ) ;
#10034=CARTESIAN_POINT ( 'NONE',  ( -33.58253175000000113, 73.47500000273117848, 10.91162601494193929 ) ) ;
#10039=VERTEX_POINT ( 'NONE', #20660 ) ;
#10040=CARTESIAN_POINT ( 'NONE',  ( -33.58253175000000113, 65.12500000273119838, 0.000000000000000000 ) ) ;
#10042=CARTESIAN_POINT ( 'NONE',  ( 15.14183272437241889, 11.70000000000000995, 20.84094480462498211 ) ) ;
#10043=CARTESIAN_POINT ( 'NONE',  ( 23.41746824999999887, 1.224999997268811480, -7.608796670333727974 ) ) ;
#10044=CARTESIAN_POINT ( 'NONE',  ( 27.16883889988624290, 9.925000002731193760, 19.73931689729373673 ) ) ;
#10046=CARTESIAN_POINT ( 'NONE',  ( -15.00000000000000000, 75.90000000000000568, -4.873795443493594171 ) ) ;
#10047=CARTESIAN_POINT ( 'NONE',  ( 5.147494310547426899, 19.94874572391552547, -32.50000000000000000 ) ) ;
#10048=CARTESIAN_POINT ( 'NONE',  ( -2.375766604868041476, 74.69874572391552192, 14.99999999999999822 ) ) ;
#10050=CARTESIAN_POINT ( 'NONE',  ( 2.897257156509938333E-15, 72.75000000546236834, 15.77193336357400710 ) ) ;
#10052=CARTESIAN_POINT ( 'NONE',  ( 33.58253175000000823, 34.02500000273118275, 10.91162601494192863 ) ) ;
#10055=CARTESIAN_POINT ( 'NONE',  ( 33.58253175000000113, 24.47500000273118914, -10.91162601494193574 ) ) ;
#10056=CARTESIAN_POINT ( 'NONE',  ( -32.50000000000000000, 12.40000000546237402, -10.55989012756945300 ) ) ;
#10057=AXIS2_PLACEMENT_3D ( 'NONE', #2445, #30925, #25781 ) ;
#10058=CARTESIAN_POINT ( 'NONE',  ( 33.58253175000000113, 78.12500000273119838, -4.112674001490185761E-15 ) ) ;
#10059=CARTESIAN_POINT ( 'NONE',  ( 10.04305231718578817, 59.90000000546235981, -30.90933677959249337 ) ) ;
#10061=CARTESIAN_POINT ( 'NONE',  ( -23.41746825000000243, 17.72499999726881370, 7.608796670333725309 ) ) ;
#10062=CARTESIAN_POINT ( 'NONE',  ( 33.58253175000000113, 64.22500000273117848, -10.91162601494193574 ) ) ;
#10065=CARTESIAN_POINT ( 'NONE',  ( -33.58253175000000113, 7.225000002731182924, 10.91162601494193929 ) ) ;
#10066=CARTESIAN_POINT ( 'NONE',  ( -23.41746824999999887, 14.12499999726882294, -2.867812753649727150E-15 ) ) ;
#10070=ORIENTED_EDGE ( 'NONE', *, *, #6408, .T. ) ;
#10074=CARTESIAN_POINT ( 'NONE',  ( -4.223320258572819786E-15, 9.499999999999992895, 24.50000000000000000 ) ) ;
#10075=CARTESIAN_POINT ( 'NONE',  ( 23.41746824999999887, 1.124999997268810725, 0.000000000000000000 ) ) ;
#10076=VECTOR ( 'NONE', #12847, 1000.000000000000000 ) ;
#10077=CARTESIAN_POINT ( 'NONE',  ( -4.523095164977116484E-15, 14.12499999726881050, 24.62258325217400312 ) ) ;
#10078=CARTESIAN_POINT ( 'NONE',  ( -20.75514604977248823, 13.07500000273120300, -28.56700777964554305 ) ) ;
#10079=CARTESIAN_POINT ( 'NONE',  ( 10.04305231718579705, 19.10000000546238752, 30.90933677959248982 ) ) ;
#10080=EDGE_CURVE ( 'NONE', #564, #25987, #25784, .T. ) ;
#10081=( BOUNDED_CURVE ( )  B_SPLINE_CURVE ( 2, ( #33195, #10048, #20178, #6613, #30622, #7118, #22918, #4549, #17091, #17600, #12448, #27550, #4038 ),
 .UNSPECIFIED., .F., .T. ) 
 B_SPLINE_CURVE_WITH_KNOTS ( ( 3, 2, 2, 2, 2, 2, 3 ),
 ( 0.5500000000000000444, 0.5600000000000000533, 0.5799999999999999600, 0.5999999999999999778, 0.6199999999999999956, 0.6400000000000000133, 0.6500000000000000222 ),
 .UNSPECIFIED. ) 
 CURVE ( )  GEOMETRIC_REPRESENTATION_ITEM ( )  RATIONAL_B_SPLINE_CURVE ( ( 0.9755282581475768211, 0.9755282581475768211, 1.000000000000000000, 0.9510565162951535312, 1.000000000000000000, 0.9510565162951535312, 1.000000000000000000, 0.9510565162951535312, 1.000000000000000000, 0.9510565162951535312, 1.000000000000000000, 0.9755282581475768211, 0.9755282581475768211 ) ) 
 REPRESENTATION_ITEM ( '' )  );
#10082=CARTESIAN_POINT ( 'NONE',  ( 20.08610463437157279, 65.29999999999999716, -27.64615127144129758 ) ) ;
#10083=CARTESIAN_POINT ( 'NONE',  ( 24.50000000000000000, 11.74999999453762989, 0.000000000000000000 ) ) ;
#10084=CARTESIAN_POINT ( 'NONE',  ( -10.04305231718579172, 29.60000000000001563, -30.90933677959248982 ) ) ;
#10086=CARTESIAN_POINT ( 'NONE',  ( -2.162160676586881955E-15, 32.87500000273118417, -35.31076352940723240 ) ) ;
#10087=FACE_OUTER_BOUND ( 'NONE', #25979, .T. ) ;
#10091=CARTESIAN_POINT ( 'NONE',  ( -18.94512977948576093, 16.32499999726880091, 13.76444248337722698 ) ) ;
#10092=CARTESIAN_POINT ( 'NONE',  ( 20.08610463437157279, 9.299999999999998934, -27.64615127144129758 ) ) ;
#10095=CARTESIAN_POINT ( 'NONE',  ( 20.75514604977249178, 49.82500000273117990, 28.56700777964553950 ) ) ;
#10097=CARTESIAN_POINT ( 'NONE',  ( -20.75514604977248823, 43.07500000273118701, -28.56700777964554305 ) ) ;
#10099=FACE_OUTER_BOUND ( 'NONE', #30173, .T. ) ;
#10100=DIRECTION ( 'NONE',  ( -0.000000000000000000, -1.000000000000000000, -0.000000000000000000 ) ) ;
#10103=CARTESIAN_POINT ( 'NONE',  ( 26.29305231718579350, 6.800000000000000711, 19.10302069950537529 ) ) ;
#10104=FACE_OUTER_BOUND ( 'NONE', #17117, .T. ) ;
#10106=CARTESIAN_POINT ( 'NONE',  ( 24.50000000000000000, 9.649999994537628467, 7.960532557706212486 ) ) ;
#10109=CARTESIAN_POINT ( 'NONE',  ( -15.14183272437242067, 10.44999999453763095, -20.84094480462497856 ) ) ;
#10110=CARTESIAN_POINT ( 'NONE',  ( -2.162160676586882350E-15, 24.62500000273118772, -35.31076352940722529 ) ) ;
#10111=CARTESIAN_POINT ( 'NONE',  ( 10.37757302488624767, 65.97500000273120691, 31.93888565452638417 ) ) ;
#10113=ORIENTED_EDGE ( 'NONE', *, *, #21593, .F. ) ;
#10123=CARTESIAN_POINT ( 'NONE',  ( -33.58253175000000113, 35.27500000273120406, -10.91162601494193218 ) ) ;
#10124=CARTESIAN_POINT ( 'NONE',  ( 10.04305231718579705, 35.10000000546236976, 30.90933677959248982 ) ) ;
#10127=CARTESIAN_POINT ( 'NONE',  ( 10.37757302488624767, 25.72500000273120335, 31.93888565452638417 ) ) ;
#10128=CARTESIAN_POINT ( 'NONE',  ( -15.00000000000000000, 81.90000000000000568, -4.873795443493594171 ) ) ;
#10129=CARTESIAN_POINT ( 'NONE',  ( 33.58253175000000113, 50.47500000273117848, -10.91162601494193751 ) ) ;
#10132=CARTESIAN_POINT ( 'NONE',  ( 10.04305231718579705, 24.60000000000001208, 30.90933677959248982 ) ) ;
#10134=CARTESIAN_POINT ( 'NONE',  ( 10.37757302488624056, 66.52500000273120406, -31.93888565452638417 ) ) ;
#10136=CARTESIAN_POINT ( 'NONE',  ( -3.880418787951136483, 14.55125428154684997, -24.50000000000000000 ) ) ;
#10137=CARTESIAN_POINT ( 'NONE',  ( -33.58253175000000113, 59.37500000273118417, 0.000000000000000000 ) ) ;
#10138=CARTESIAN_POINT ( 'NONE',  ( 10.04305231718579705, 72.59999999999999432, 30.90933677959248982 ) ) ;
#10139=CARTESIAN_POINT ( 'NONE',  ( -10.37757302488623701, 11.52500000273118452, 31.93888565452638417 ) ) ;
#10140=CARTESIAN_POINT ( 'NONE',  ( -19.82091636218621389, 8.949999994537632730, 14.40073868116558842 ) ) ;
#10145=CARTESIAN_POINT ( 'NONE',  ( 32.50000000000000711, 18.90000000000001279, 10.55989012756945122 ) ) ;
#10149=AXIS2_PLACEMENT_3D ( 'NONE', #8702, #21766, #32209 ) ;
#10151=CARTESIAN_POINT ( 'NONE',  ( 20.08610463437157279, 63.30000000000001137, -27.64615127144129758 ) ) ;
#10153=CARTESIAN_POINT ( 'NONE',  ( 5.147494310547426899, 63.94874572391551482, -32.50000000000000000 ) ) ;
#10154=CARTESIAN_POINT ( 'NONE',  ( 32.50000000000000000, 73.50000000546236834, -3.980102097228898626E-15 ) ) ;
#10158=EDGE_LOOP ( 'NONE', ( #20245, #7059, #24658, #22589 ) ) ;
#10159=CARTESIAN_POINT ( 'NONE',  ( 10.37757302488624767, 75.97500000273119269, 31.93888565452638417 ) ) ;
#10163=CARTESIAN_POINT ( 'NONE',  ( -20.75514604977248823, 55.07500000273117990, -28.56700777964554305 ) ) ;
#10164=CARTESIAN_POINT ( 'NONE',  ( 20.08610463437158344, 63.20000000546237118, 27.64615127144129403 ) ) ;
#10165=ORIENTED_EDGE ( 'NONE', *, *, #32350, .T. ) ;
#10166=CARTESIAN_POINT ( 'NONE',  ( -1.778240108872766143E-15, 10.00000000546236834, -32.49999999999999289 ) ) ;
#10167=CARTESIAN_POINT ( 'NONE',  ( -33.58253175000000113, 43.12500000273116996, 0.000000000000000000 ) ) ;
#10168=CARTESIAN_POINT ( 'NONE',  ( -23.41746824999999887, 17.62499999726882649, -2.867812753649727150E-15 ) ) ;
#10169=CARTESIAN_POINT ( 'NONE',  ( 20.75514604977249178, 70.07500000273120122, 28.56700777964553950 ) ) ;
#10171=CARTESIAN_POINT ( 'NONE',  ( -2.092463501923844636E-15, 4.000000005462377217, -34.17252228774368916 ) ) ;
#10175=CARTESIAN_POINT ( 'NONE',  ( 26.29305231718579350, 48.80000000000001137, 19.10302069950537529 ) ) ;
#10176=CARTESIAN_POINT ( 'NONE',  ( 3.000384657911015469E-15, 0.000000000000000000, -24.50000000000000000 ) ) ;
#10177=CARTESIAN_POINT ( 'NONE',  ( -27.16883889988623935, 11.57500000273120655, 19.73931689729374739 ) ) ;
#10178=CARTESIAN_POINT ( 'NONE',  ( -26.29305231718579350, 73.80000000000001137, -19.10302069950537884 ) ) ;
#10180=CARTESIAN_POINT ( 'NONE',  ( -13.91746824999999532, 79.27500000273118985, -4.522059556121115875 ) ) ;
#10181=CARTESIAN_POINT ( 'NONE',  ( 4.635254915624212657, 74.85000000546237686, 14.26584774442730286 ) ) ;
#10182=DIRECTION ( 'NONE',  ( -0.000000000000000000, 1.000000000000000000, -0.000000000000000000 ) ) ;
#10184=ORIENTED_EDGE ( 'NONE', *, *, #23725, .F. ) ;
#10188=VECTOR ( 'NONE', #22027, 1000.000000000000000 ) ;
#10194=VECTOR ( 'NONE', #24325, 1000.000000000000000 ) ;
#10195=( BOUNDED_CURVE ( )  B_SPLINE_CURVE ( 2, ( #26977, #1392, #32788, #17027, #21844, #11206, #9281, #11865, #19765, #8955, #24410, #32623, #24250 ),
 .UNSPECIFIED., .F., .T. ) 
 B_SPLINE_CURVE_WITH_KNOTS ( ( 3, 2, 2, 2, 2, 2, 3 ),
 ( 0.1388888888888888673, 0.1444444444444444309, 0.1555555555555555580, 0.1666666666666666574, 0.1777777777777777846, 0.1888888888888888840, 0.1944444444444444475 ),
 .UNSPECIFIED. ) 
 CURVE ( )  GEOMETRIC_REPRESENTATION_ITEM ( )  RATIONAL_B_SPLINE_CURVE ( ( 0.9755282581475768211, 0.9755282581475768211, 1.000000000000000000, 0.9510565162951535312, 1.000000000000000000, 0.9510565162951535312, 1.000000000000000000, 0.9510565162951535312, 1.000000000000000000, 0.9510565162951535312, 1.000000000000000000, 0.9755282581475768211, 0.9755282581475768211 ) ) 
 REPRESENTATION_ITEM ( '' )  );
#10201=CARTESIAN_POINT ( 'NONE',  ( -33.58253175000000113, 45.02500000273117564, -10.91162601494193041 ) ) ;
#10203=CARTESIAN_POINT ( 'NONE',  ( 15.00000000000000000, 79.00000000000001421, -1.836970198721029589E-15 ) ) ;
#10204=ORIENTED_EDGE ( 'NONE', *, *, #28242, .F. ) ;
#10207=CARTESIAN_POINT ( 'NONE',  ( -2.162160676586881955E-15, 72.87500000273115575, -35.31076352940723240 ) ) ;
#10208=ORIENTED_EDGE ( 'NONE', *, *, #31652, .T. ) ;
#10211=ORIENTED_EDGE ( 'NONE', *, *, #30533, .F. ) ;
#10213=CARTESIAN_POINT ( 'NONE',  ( -10.04305231718578462, 14.90000000546237757, 30.90933677959249337 ) ) ;
#10214=CARTESIAN_POINT ( 'NONE',  ( 27.16883889988624290, 59.92500000273118133, 19.73931689729373673 ) ) ;
#10216=CARTESIAN_POINT ( 'NONE',  ( -24.50000000000000000, 17.00000000000001421, -3.000384657911015469E-15 ) ) ;
#10217=CARTESIAN_POINT ( 'NONE',  ( 18.94512977948575738, 4.924999997268808549, 13.76444248337723408 ) ) ;
#10218=EDGE_CURVE ( 'NONE', #1559, #28004, #13288, .T. ) ;
#10219=CARTESIAN_POINT ( 'NONE',  ( 6.486482029760649416E-15, 3.625000002731181059, 35.31076352940723240 ) ) ;
#10222=CARTESIAN_POINT ( 'NONE',  ( -15.00000000000000000, 72.09999999999999432, 4.873795443493597723 ) ) ;
#10227=CARTESIAN_POINT ( 'NONE',  ( 4.635254915624212657, 72.85000000546237686, 14.26584774442730286 ) ) ;
#10229=CARTESIAN_POINT ( 'NONE',  ( 33.58253175000000113, 32.22500000273117848, -10.91162601494193751 ) ) ;
#10232=CARTESIAN_POINT ( 'NONE',  ( -27.16883889988623935, 23.57500000273119056, 19.73931689729374739 ) ) ;
#10233=CARTESIAN_POINT ( 'NONE',  ( 1.093617666956751375E-13, 67.50000000000001421, -32.50000000000000711 ) ) ;
#10234=CARTESIAN_POINT ( 'NONE',  ( 10.37757302488624767, 77.72500000273119269, 31.93888565452638417 ) ) ;
#10235=CARTESIAN_POINT ( 'NONE',  ( -32.50000000000000000, 66.10000000000000853, 10.55989012756946366 ) ) ;
#10237=CARTESIAN_POINT ( 'NONE',  ( 14.47279130897151767, 18.32499999726882578, 19.92008829642072953 ) ) ;
#10238=CARTESIAN_POINT ( 'NONE',  ( -10.37757302488624411, 64.72500000273117848, -31.93888565452638417 ) ) ;
#10242=CARTESIAN_POINT ( 'NONE',  ( 33.58253175000000823, 10.02500000273118275, 10.91162601494192685 ) ) ;
#10243=CARTESIAN_POINT ( 'NONE',  ( 1.507698388325705758E-15, 15.62499999726882116, -24.62258325217400312 ) ) ;
#10245=ORIENTED_EDGE ( 'NONE', *, *, #18742, .T. ) ;
#10247=ORIENTED_EDGE ( 'NONE', *, *, #5383, .F. ) ;
#10249=LINE ( 'NONE', #12816, #4558 ) ;
#10251=CARTESIAN_POINT ( 'NONE',  ( 20.75514604977248467, 78.42500000273116711, -28.56700777964554305 ) ) ;
#10252=CARTESIAN_POINT ( 'NONE',  ( 23.41746825000000243, 3.024999997268812635, 7.608796670333735079 ) ) ;
#10253=CARTESIAN_POINT ( 'NONE',  ( 23.41746825000000243, 16.52499999726882152, 7.608796670333735079 ) ) ;
#10254=CARTESIAN_POINT ( 'NONE',  ( 10.37757302488624767, 17.97500000273119625, 31.93888565452638417 ) ) ;
#10255=CARTESIAN_POINT ( 'NONE',  ( -10.04305231718579172, 18.10000000546238397, -30.90933677959248982 ) ) ;
#10256=CARTESIAN_POINT ( 'NONE',  ( 32.50000000000000711, 66.90000000000001990, 10.55989012756945122 ) ) ;
#10257=CARTESIAN_POINT ( 'NONE',  ( -10.04305231718578462, 30.39999999999998437, 30.90933677959249337 ) ) ;
#10262=DIRECTION ( 'NONE',  ( -0.000000000000000000, -1.000000000000000000, -0.000000000000000000 ) ) ;
#10263=CARTESIAN_POINT ( 'NONE',  ( -7.236395654485757944, 17.72499999726881370, -22.27133577429736988 ) ) ;
#10264=CARTESIAN_POINT ( 'NONE',  ( -10.04305231718578462, 6.400000000000016342, 30.90933677959249337 ) ) ;
#10265=CYLINDRICAL_SURFACE ( 'NONE', #2837, 32.50000000000000000 ) ;
#10267=CARTESIAN_POINT ( 'NONE',  ( -27.16883889988623935, 51.32500000273118701, 19.73931689729374739 ) ) ;
#10269=CARTESIAN_POINT ( 'NONE',  ( 10.37757302488624767, 37.97500000273118559, 31.93888565452638417 ) ) ;
#10270=DIRECTION ( 'NONE',  ( -0.000000000000000000, 1.000000000000000000, -0.000000000000000000 ) ) ;
#10274=CARTESIAN_POINT ( 'NONE',  ( 10.04305231718579705, 51.10000000546238397, 30.90933677959248982 ) ) ;
#10277=CARTESIAN_POINT ( 'NONE',  ( -20.08610463437156923, 62.80000000546237260, 27.64615127144130113 ) ) ;
#10278=CARTESIAN_POINT ( 'NONE',  ( 1.836970198721029589E-15, 82.00000000000001421, 15.00000000000000000 ) ) ;
#10279=CARTESIAN_POINT ( 'NONE',  ( -20.08610463437156923, 40.30000000000001137, 27.64615127144130113 ) ) ;
#10282=ADVANCED_FACE ( 'NONE', ( #27851 ), #25620, .F. ) ;
#10283=CARTESIAN_POINT ( 'NONE',  ( 7.570916362186207671, 17.34999999453762243, 23.30088464923126779 ) ) ;
#10284=CARTESIAN_POINT ( 'NONE',  ( -27.16883889988623935, 27.32500000273119412, 19.73931689729374739 ) ) ;
#10295=CARTESIAN_POINT ( 'NONE',  ( -1.778240108872766143E-15, 46.00000000546238255, -32.49999999999999289 ) ) ;
#10296=CARTESIAN_POINT ( 'NONE',  ( 33.58253175000000823, 32.27500000273117564, 10.91162601494192863 ) ) ;
#10297=CARTESIAN_POINT ( 'NONE',  ( -32.50000000000000000, 40.50000000546238965, 0.000000000000000000 ) ) ;
#10299=CARTESIAN_POINT ( 'NONE',  ( -5.147494310547423346, 48.44874571845315359, 32.50000000000000000 ) ) ;
#10300=CARTESIAN_POINT ( 'NONE',  ( -27.16883889988623935, 25.32500000273119056, 19.73931689729374739 ) ) ;
#10302=CARTESIAN_POINT ( 'NONE',  ( 10.37757302488624767, 49.97500000273119269, 31.93888565452638417 ) ) ;
#10304=CARTESIAN_POINT ( 'NONE',  ( -2.092463501923844636E-15, 25.50000000000001066, -34.17252228774368916 ) ) ;
#10306=CARTESIAN_POINT ( 'NONE',  ( 10.37757302488624767, 71.72500000273119269, 31.93888565452638417 ) ) ;
#10307=CARTESIAN_POINT ( 'NONE',  ( -10.04305231718579172, 77.60000000000000853, -30.90933677959248982 ) ) ;
#10308=CARTESIAN_POINT ( 'NONE',  ( -7.570916362186210335, 14.60000000000000142, -23.30088464923126779 ) ) ;
#10309=CARTESIAN_POINT ( 'NONE',  ( 20.75514604977249178, 58.07500000273117990, 28.56700777964553950 ) ) ;
#10310=CARTESIAN_POINT ( 'NONE',  ( -1.778240108872766143E-15, 40.00000000546237544, -32.49999999999999289 ) ) ;
#10311=CARTESIAN_POINT ( 'NONE',  ( -33.58253175000000113, 11.02500000273117919, -10.91162601494193218 ) ) ;
#10321=EDGE_CURVE ( 'NONE', #32300, #30131, #29906, .T. ) ;
#10325=CARTESIAN_POINT ( 'NONE',  ( -10.04305231718578462, 54.40000000000000568, 30.90933677959249337 ) ) ;
#10327=CARTESIAN_POINT ( 'NONE',  ( -32.50000000000000000, 66.50000000546238255, 0.000000000000000000 ) ) ;
#10332=CARTESIAN_POINT ( 'NONE',  ( -20.75514604977248823, 73.07500000273115859, -28.56700777964554305 ) ) ;
#10336=CARTESIAN_POINT ( 'NONE',  ( 20.75514604977249178, 52.07500000273119412, 28.56700777964553950 ) ) ;
#10337=CARTESIAN_POINT ( 'NONE',  ( 20.08610463437158344, 57.20000000546237828, 27.64615127144129403 ) ) ;
#10338=CARTESIAN_POINT ( 'NONE',  ( -5.147494310547430452, 10.05125428700921653, -32.49999999999999289 ) ) ;
#10339=CARTESIAN_POINT ( 'NONE',  ( -27.16883889988624290, 44.92500000273119554, -19.73931689729374028 ) ) ;
#10341=CARTESIAN_POINT ( 'NONE',  ( -27.16883889988623935, 65.57500000273120122, 19.73931689729374739 ) ) ;
#10342=CARTESIAN_POINT ( 'NONE',  ( 20.08610463437158344, 7.200000005462393382, 27.64615127144129403 ) ) ;
#10345=CARTESIAN_POINT ( 'NONE',  ( 32.50000000000000000, 45.10000000000000853, -10.55989012756945833 ) ) ;
#10347=CARTESIAN_POINT ( 'NONE',  ( 6.486482029760649416E-15, 11.87500000273118062, 35.31076352940723240 ) ) ;
#10349=CARTESIAN_POINT ( 'NONE',  ( -8.601468415847518756, 77.07500000273117280, -11.83890561707634781 ) ) ;
#10350=CARTESIAN_POINT ( 'NONE',  ( 0.000000000000000000, 0.000000000000000000, 0.000000000000000000 ) ) ;
#10353=ORIENTED_EDGE ( 'NONE', *, *, #20920, .T. ) ;
#10364=CARTESIAN_POINT ( 'NONE',  ( 33.58253175000000823, 44.02500000273118275, 10.91162601494192685 ) ) ;
#10371=CARTESIAN_POINT ( 'NONE',  ( -10.37757302488624411, 78.97500000273119269, -31.93888565452638417 ) ) ;
#10375=VERTEX_POINT ( 'NONE', #7075 ) ;
#10376=CARTESIAN_POINT ( 'NONE',  ( 5.147494310547426899, 29.94874572391553258, -32.50000000000000000 ) ) ;
#10377=CARTESIAN_POINT ( 'NONE',  ( -20.75514604977248823, 62.82500000273119412, -28.56700777964554305 ) ) ;
#10381=CARTESIAN_POINT ( 'NONE',  ( 20.75514604977248467, 6.425000002731179549, -28.56700777964554305 ) ) ;
#10382=CARTESIAN_POINT ( 'NONE',  ( -24.50000000000000711, 6.849999994537629533, 7.960532557706201828 ) ) ;
#10386=CARTESIAN_POINT ( 'NONE',  ( 20.08610463437157279, 9.299999999999995381, -27.64615127144129758 ) ) ;
#10390=CARTESIAN_POINT ( 'NONE',  ( 8.601468415847516980, 80.17500000273116711, -11.83890561707634781 ) ) ;
#10392=CARTESIAN_POINT ( 'NONE',  ( -33.58253175000000113, 31.02500000273118630, -10.91162601494193218 ) ) ;
#10395=CARTESIAN_POINT ( 'NONE',  ( 27.16883889988624290, 18.17500000273120264, 19.73931689729373673 ) ) ;
#10396=CARTESIAN_POINT ( 'NONE',  ( -5.147494310547377161, 67.55125428154684641, -32.50000000000002132 ) ) ;
#10398=CARTESIAN_POINT ( 'NONE',  ( -27.16883889988624290, 76.92500000273119554, -19.73931689729374028 ) ) ;
#10401=CARTESIAN_POINT ( 'NONE',  ( -23.41746824999999887, 17.52499999726881796, -7.608796670333730638 ) ) ;
#10402=CARTESIAN_POINT ( 'NONE',  ( -33.58253175000000113, 65.12500000273119838, 0.000000000000000000 ) ) ;
#10405=CARTESIAN_POINT ( 'NONE',  ( -10.37757302488624411, 4.725000002731183812, -31.93888565452638417 ) ) ;
#10406=CARTESIAN_POINT ( 'NONE',  ( -23.41746825000000598, 18.22499999726879949, 7.608796670333726198 ) ) ;
#10413=CARTESIAN_POINT ( 'NONE',  ( -20.08610463437157989, 79.70000000000000284, -27.64615127144129758 ) ) ;
#10415=CARTESIAN_POINT ( 'NONE',  ( 6.486482029760649416E-15, 77.62500000273121259, 35.31076352940723240 ) ) ;
#10416=CARTESIAN_POINT ( 'NONE',  ( -4.523095164977116484E-15, 6.624999997268815832, 24.62258325217400312 ) ) ;
#10417=EDGE_CURVE ( 'NONE', #390, #23284, #33423, .T. ) ;
#10418=CARTESIAN_POINT ( 'NONE',  ( -18.94512977948575738, 15.42499999726881832, -13.76444248337723231 ) ) ;
#10419=CARTESIAN_POINT ( 'NONE',  ( 27.16883889988624290, 18.17500000273120264, 19.73931689729373673 ) ) ;
#10420=CARTESIAN_POINT ( 'NONE',  ( -10.04305231718579172, 57.59999999999998721, -30.90933677959248982 ) ) ;
#10421=CARTESIAN_POINT ( 'NONE',  ( -1.089172066684569321E-14, 76.75000000546238255, 15.00000000000000000 ) ) ;
#10422=DIRECTION ( 'NONE',  ( 0.000000000000000000, 0.000000000000000000, -1.000000000000000000 ) ) ;
#10424=CARTESIAN_POINT ( 'NONE',  ( -4.300734207923759378, 76.97500000273119269, -13.23629886949340495 ) ) ;
#10427=ADVANCED_FACE ( 'NONE', ( #26635 ), #7763, .T. ) ;
#10428=DIRECTION ( 'NONE',  ( 0.000000000000000000, 1.000000000000000000, 0.000000000000000000 ) ) ;
#10429=CARTESIAN_POINT ( 'NONE',  ( 5.779280353836490358E-15, 68.50000000000000000, 32.49999999999999289 ) ) ;
#10430=CARTESIAN_POINT ( 'NONE',  ( 32.50000000000000711, 6.900000000000014566, 10.55989012756945122 ) ) ;
#10433=CARTESIAN_POINT ( 'NONE',  ( -10.37757302488623701, 53.52500000273118985, 31.93888565452638417 ) ) ;
#10435=CARTESIAN_POINT ( 'NONE',  ( 20.75514604977248467, 40.67500000273117422, -28.56700777964554305 ) ) ;
#10436=CARTESIAN_POINT ( 'NONE',  ( 10.04305231718579705, 24.60000000000001208, 30.90933677959248982 ) ) ;
#10438=CARTESIAN_POINT ( 'NONE',  ( 5.779280353836490358E-15, 15.00000000546237899, 32.49999999999999289 ) ) ;
#10440=CARTESIAN_POINT ( 'NONE',  ( -26.29305231718579350, 27.79999999999999005, -19.10302069950537884 ) ) ;
#10442=CARTESIAN_POINT ( 'NONE',  ( -11.25946833292375793, 81.17500000273119554, -8.180482586598733619 ) ) ;
#10444=CARTESIAN_POINT ( 'NONE',  ( 0.000000000000000000, 80.00000000000001421, 0.000000000000000000 ) ) ;
#10447=CARTESIAN_POINT ( 'NONE',  ( -3.880418787951142701, 11.19874571299079058, 24.49999999999999645 ) ) ;
#10449=CARTESIAN_POINT ( 'NONE',  ( 33.58253175000000113, 24.22500000273119625, -10.91162601494193574 ) ) ;
#10451=ORIENTED_EDGE ( 'NONE', *, *, #20393, .T. ) ;
#10454=ORIENTED_EDGE ( 'NONE', *, *, #9880, .F. ) ;
#10459=CARTESIAN_POINT ( 'NONE',  ( 5.779280353836490358E-15, 15.00000000546237899, 32.49999999999999289 ) ) ;
#10460=CARTESIAN_POINT ( 'NONE',  ( 10.37757302488624056, 34.77500000273120406, -31.93888565452638417 ) ) ;
#10461=CARTESIAN_POINT ( 'NONE',  ( 32.50000000000000000, 37.60000000546235555, -10.55989012756945833 ) ) ;
#10464=CARTESIAN_POINT ( 'NONE',  ( 10.37757302488624056, 20.52500000273119340, -31.93888565452638417 ) ) ;
#10465=CARTESIAN_POINT ( 'NONE',  ( 24.50000000000000000, 5.749999994537624559, 0.000000000000000000 ) ) ;
#10466=CARTESIAN_POINT ( 'NONE',  ( -33.58253175000000113, 47.47500000273119269, 10.91162601494193929 ) ) ;
#10468=CARTESIAN_POINT ( 'NONE',  ( 6.277390505771533514E-15, 26.50000000000000711, 34.17252228774368916 ) ) ;
#10470=ADVANCED_FACE ( 'NONE', ( #33853 ), #31937, .T. ) ;
#10471=CARTESIAN_POINT ( 'NONE',  ( -27.16883889988624290, 68.92500000273119554, -19.73931689729374028 ) ) ;
#10472=CARTESIAN_POINT ( 'NONE',  ( -4.934616302121927505E-14, 71.00000000546238255, 32.50000000000000000 ) ) ;
#10473=CARTESIAN_POINT ( 'NONE',  ( -26.29305231718578995, 76.70000000546239960, 19.10302069950538595 ) ) ;
#10474=CARTESIAN_POINT ( 'NONE',  ( -27.16883889988624290, 59.17500000273118133, -19.73931689729374028 ) ) ;
#10475=CARTESIAN_POINT ( 'NONE',  ( -10.04305231718579172, 40.10000000546237686, -30.90933677959248982 ) ) ;
#10476=CARTESIAN_POINT ( 'NONE',  ( 20.75514604977248467, 12.42500000273119554, -28.56700777964554305 ) ) ;
#10479=CARTESIAN_POINT ( 'NONE',  ( 27.16883889988624290, 4.175000002731188431, 19.73931689729373673 ) ) ;
#10481=CARTESIAN_POINT ( 'NONE',  ( 20.08610463437157279, 45.80000000546239391, -27.64615127144129758 ) ) ;
#10482=CARTESIAN_POINT ( 'NONE',  ( 5.779280353836490358E-15, 18.50000000000000000, 32.49999999999999289 ) ) ;
#10489=CARTESIAN_POINT ( 'NONE',  ( 20.08610463437157279, 63.80000000546237970, -27.64615127144129758 ) ) ;
#10490=CARTESIAN_POINT ( 'NONE',  ( 26.29305231718579350, 67.30000000546237970, 19.10302069950537529 ) ) ;
#10494=VERTEX_POINT ( 'NONE', #8262 ) ;
#10498=CARTESIAN_POINT ( 'NONE',  ( -1.778240108872766143E-15, 35.49999999999998579, -32.49999999999999289 ) ) ;
#10499=CARTESIAN_POINT ( 'NONE',  ( -10.37757302488623701, 53.77500000273119696, 31.93888565452638417 ) ) ;
#10500=CARTESIAN_POINT ( 'NONE',  ( -2.092463501923844636E-15, 54.00000000546236834, -34.17252228774368916 ) ) ;
#10502=CARTESIAN_POINT ( 'NONE',  ( 33.58253175000000113, 40.22500000273119269, -10.91162601494193751 ) ) ;
#10504=VECTOR ( 'NONE', #1829, 1000.000000000000000 ) ;
#10505=CARTESIAN_POINT ( 'NONE',  ( -33.58253175000000113, 71.47500000273119269, 10.91162601494193929 ) ) ;
#10509=CARTESIAN_POINT ( 'NONE',  ( -26.29305231718578995, 44.20000000000001705, 19.10302069950538595 ) ) ;
#10511=EDGE_CURVE ( 'NONE', #26665, #29691, #2973, .T. ) ;
#10512=CARTESIAN_POINT ( 'NONE',  ( 10.37757302488624056, 12.77500000273118452, -31.93888565452638417 ) ) ;
#10516=CARTESIAN_POINT ( 'NONE',  ( 2.489536152421872915E-14, 77.50000000000000000, -32.49999999999999289 ) ) ;
#10517=CARTESIAN_POINT ( 'NONE',  ( 0.000000000000000000, 80.00000000000001421, 0.000000000000000000 ) ) ;
#10520=ORIENTED_EDGE ( 'NONE', *, *, #30533, .T. ) ;
#10531=CARTESIAN_POINT ( 'NONE',  ( -10.37757302488624411, 38.72500000273118559, -31.93888565452638417 ) ) ;
#10534=CARTESIAN_POINT ( 'NONE',  ( 2.445080149700053643E-15, 74.75000000546236834, 15.00000000000000000 ) ) ;
#10537=CARTESIAN_POINT ( 'NONE',  ( 23.41746824999999887, 0.8749999972688105032, 0.000000000000000000 ) ) ;
#10539=CARTESIAN_POINT ( 'NONE',  ( -33.58253175000000113, 77.47500000273120691, 10.91162601494193929 ) ) ;
#10540=VERTEX_POINT ( 'NONE', #2787 ) ;
#10544=CARTESIAN_POINT ( 'NONE',  ( 10.04305231718578817, 29.90000000546239178, -30.90933677959249337 ) ) ;
#10545=CARTESIAN_POINT ( 'NONE',  ( -20.75514604977248823, 58.82500000273117990, -28.56700777964554305 ) ) ;
#10547=CARTESIAN_POINT ( 'NONE',  ( -18.94512977948576093, 10.32499999726882400, 13.76444248337722698 ) ) ;
#10548=CARTESIAN_POINT ( 'NONE',  ( 20.75514604977248467, 4.425000002731183990, -28.56700777964554305 ) ) ;
#10551=CARTESIAN_POINT ( 'NONE',  ( -15.00000000000000000, 80.15000000546234560, -4.873795443493594171 ) ) ;
#10553=CARTESIAN_POINT ( 'NONE',  ( 20.08610463437158344, 8.699999999999986855, 27.64615127144129403 ) ) ;
#10557=EDGE_CURVE ( 'NONE', #11416, #11025, #7932, .T. ) ;
#10559=CARTESIAN_POINT ( 'NONE',  ( -4.635254915624211769, 73.85000000546237686, -14.26584774442730286 ) ) ;
#10561=CARTESIAN_POINT ( 'NONE',  ( -2.162160676586881955E-15, 28.62500000273118062, -35.31076352940723240 ) ) ;
#10564=CARTESIAN_POINT ( 'NONE',  ( 33.58253175000000113, 16.47500000273118204, -10.91162601494193574 ) ) ;
#10565=CARTESIAN_POINT ( 'NONE',  ( -1.053607264507113999E-13, 64.50000000000000000, 32.50000000000000711 ) ) ;
#10568=CARTESIAN_POINT ( 'NONE',  ( -10.37757302488624411, 74.72500000273119269, -31.93888565452638417 ) ) ;
#10569=CARTESIAN_POINT ( 'NONE',  ( 24.50000000000000000, 8.100000000000006750, -7.960532557706203605 ) ) ;
#10571=CARTESIAN_POINT ( 'NONE',  ( -18.94512977948575738, 17.42499999726882010, -13.76444248337723231 ) ) ;
#10572=CARTESIAN_POINT ( 'NONE',  ( 10.37757302488624056, 56.52500000273119696, -31.93888565452638417 ) ) ;
#10577=CARTESIAN_POINT ( 'NONE',  ( 33.58253175000000113, 8.125000002731198379, -4.112674001490185761E-15 ) ) ;
#10578=CARTESIAN_POINT ( 'NONE',  ( 7.236395654485760609, 15.52499999726880731, -22.27133577429736633 ) ) ;
#10582=( BOUNDED_CURVE ( )  B_SPLINE_CURVE ( 2, ( #26378, #13162, #10257, #5441, #10763, #28943, #2530, #26208, #33931, #26036, #10084, #28269, #12998 ),
 .UNSPECIFIED., .F., .T. ) 
 B_SPLINE_CURVE_WITH_KNOTS ( ( 3, 2, 2, 2, 2, 2, 3 ),
 ( 0.6346153846153845812, 0.6358974358974358587, 0.6384615384615384137, 0.6410256410256410797, 0.6435897435897436347, 0.6461538461538461897, 0.6474358974358974672 ),
 .UNSPECIFIED. ) 
 CURVE ( )  GEOMETRIC_REPRESENTATION_ITEM ( )  RATIONAL_B_SPLINE_CURVE ( ( 0.9755282581475768211, 0.9755282581475768211, 1.000000000000000000, 0.9510565162951535312, 1.000000000000000000, 0.9510565162951535312, 1.000000000000000000, 0.9510565162951535312, 1.000000000000000000, 0.9510565162951535312, 1.000000000000000000, 0.9755282581475768211, 0.9755282581475768211 ) ) 
 REPRESENTATION_ITEM ( '' )  );
#10585=CARTESIAN_POINT ( 'NONE',  ( 5.147494310547434893, 4.551254281546843750, 32.49999999999999289 ) ) ;
#10587=CARTESIAN_POINT ( 'NONE',  ( 26.29305231718578995, 27.70000000546238184, -19.10302069950538240 ) ) ;
#10589=CARTESIAN_POINT ( 'NONE',  ( 24.50000000000000000, 0.000000000000000000, 0.000000000000000000 ) ) ;
#10590=CARTESIAN_POINT ( 'NONE',  ( 6.486482029760649416E-15, 17.87500000273119838, 35.31076352940723240 ) ) ;
#10592=CARTESIAN_POINT ( 'NONE',  ( 20.08610463437157279, 61.30000000000001847, -27.64615127144129758 ) ) ;
#10593=CARTESIAN_POINT ( 'NONE',  ( 20.08610463437158344, 57.20000000546237828, 27.64615127144129403 ) ) ;
#10594=CARTESIAN_POINT ( 'NONE',  ( 32.50000000000000000, 73.60000000546239107, -10.55989012756945833 ) ) ;
#10596=CARTESIAN_POINT ( 'NONE',  ( 11.25946833292375793, 76.57500000273120122, -8.180482586598735395 ) ) ;
#10598=CYLINDRICAL_SURFACE ( 'NONE', #7510, 15.00000000000000000 ) ;
#10599=CARTESIAN_POINT ( 'NONE',  ( -24.50000000000000000, 13.00000000000001066, -3.000384657911015469E-15 ) ) ;
#10600=CARTESIAN_POINT ( 'NONE',  ( 10.04305231718579705, 4.599999999999992539, 30.90933677959248982 ) ) ;
#10603=CARTESIAN_POINT ( 'NONE',  ( 27.16883889988624290, 51.92500000273120264, 19.73931689729373673 ) ) ;
#10606=CARTESIAN_POINT ( 'NONE',  ( 20.75514604977248467, 32.67500000273119554, -28.56700777964554305 ) ) ;
#10608=LINE ( 'NONE', #22966, #8447 ) ;
#10610=CARTESIAN_POINT ( 'NONE',  ( -20.08610463437156923, 22.80000000546236549, 27.64615127144130113 ) ) ;
#10613=DIRECTION ( 'NONE',  ( 0.000000000000000000, 0.000000000000000000, 1.000000000000000000 ) ) ;
#10615=CARTESIAN_POINT ( 'NONE',  ( 19.82091636218621389, 9.949999994537634507, -14.40073868116559197 ) ) ;
#10618=CARTESIAN_POINT ( 'NONE',  ( 32.50000000000000711, 10.90000000000000568, 10.55989012756945122 ) ) ;
#10619=CARTESIAN_POINT ( 'NONE',  ( -33.58253175000000113, 23.22500000273117493, 10.91162601494193929 ) ) ;
#10622=ADVANCED_FACE ( 'NONE', ( #13253 ), #193, .T. ) ;
#10623=ORIENTED_EDGE ( 'NONE', *, *, #14259, .T. ) ;
#10629=CARTESIAN_POINT ( 'NONE',  ( -23.41746824999999887, 1.624999997268811169, -2.867812753649727150E-15 ) ) ;
#10630=CARTESIAN_POINT ( 'NONE',  ( -27.16883889988623935, 37.57500000273117280, 19.73931689729374739 ) ) ;
#10631=CARTESIAN_POINT ( 'NONE',  ( 26.29305231718578995, 35.70000000546236407, -19.10302069950538240 ) ) ;
#10632=CARTESIAN_POINT ( 'NONE',  ( 20.08610463437157279, 79.30000000000001137, -27.64615127144129758 ) ) ;
#10634=CARTESIAN_POINT ( 'NONE',  ( 0.000000000000000000, 0.000000000000000000, 24.50000000000000000 ) ) ;
#10635=CARTESIAN_POINT ( 'NONE',  ( 10.37757302488624767, 51.97500000273119980, 31.93888565452638417 ) ) ;
#10637=CARTESIAN_POINT ( 'NONE',  ( -32.50000000000000000, 24.09999999999999787, 10.55989012756946366 ) ) ;
#10639=CARTESIAN_POINT ( 'NONE',  ( 33.58253175000000113, 68.12500000273119838, -4.112674001490185761E-15 ) ) ;
#10643=CARTESIAN_POINT ( 'NONE',  ( 20.75514604977248467, 56.67500000273119554, -28.56700777964554305 ) ) ;
#10645=CARTESIAN_POINT ( 'NONE',  ( 20.08610463437157279, 7.800000005462373487, -27.64615127144129758 ) ) ;
#10646=CARTESIAN_POINT ( 'NONE',  ( -10.37757302488624411, 14.72500000273119269, -31.93888565452638417 ) ) ;
#10649=CARTESIAN_POINT ( 'NONE',  ( 10.37757302488624056, 2.775000002731176085, -31.93888565452638417 ) ) ;
#10652=DIRECTION ( 'NONE',  ( -0.000000000000000000, -1.000000000000000000, -0.000000000000000000 ) ) ;
#10659=CARTESIAN_POINT ( 'NONE',  ( 23.41746825000000243, 3.224999997268806151, -7.608796670333727974 ) ) ;
#10660=CARTESIAN_POINT ( 'NONE',  ( -20.08610463437157989, 68.20000000546239960, -27.64615127144129758 ) ) ;
#10668=CARTESIAN_POINT ( 'NONE',  ( 2.489536152421872915E-14, 75.50000000000001421, -32.49999999999999289 ) ) ;
#10669=CARTESIAN_POINT ( 'NONE',  ( -27.16883889988624290, 53.17500000273117422, -19.73931689729374028 ) ) ;
#10670=CARTESIAN_POINT ( 'NONE',  ( 26.29305231718578995, 59.70000000546238539, -19.10302069950538240 ) ) ;
#10672=CARTESIAN_POINT ( 'NONE',  ( -27.16883889988624290, 40.92500000273119554, -19.73931689729374028 ) ) ;
#10673=CARTESIAN_POINT ( 'NONE',  ( -33.58253175000000113, 67.37500000273119838, 0.000000000000000000 ) ) ;
#10677=CARTESIAN_POINT ( 'NONE',  ( 26.29305231718579350, 44.80000000000000426, 19.10302069950537529 ) ) ;
#10679=CARTESIAN_POINT ( 'NONE',  ( 10.37757302488624767, 7.975000002731186477, 31.93888565452638417 ) ) ;
#10680=CARTESIAN_POINT ( 'NONE',  ( 0.000000000000000000, 80.00000000000001421, 0.000000000000000000 ) ) ;
#10682=CARTESIAN_POINT ( 'NONE',  ( 4.300734207923761154, 73.97500000273119269, 13.23629886949340495 ) ) ;
#10685=ORIENTED_EDGE ( 'NONE', *, *, #23142, .T. ) ;
#10686=CYLINDRICAL_SURFACE ( 'NONE', #14582, 32.50000000000000000 ) ;
#10687=AXIS2_PLACEMENT_3D ( 'NONE', #25885, #15779, #301 ) ;
#10698=CARTESIAN_POINT ( 'NONE',  ( -20.75514604977248112, 39.42500000273118843, 28.56700777964554661 ) ) ;
#10701=CARTESIAN_POINT ( 'NONE',  ( 3.000384657911015469E-15, 0.000000000000000000, -24.50000000000000000 ) ) ;
#10706=CARTESIAN_POINT ( 'NONE',  ( -2.162160676586881955E-15, 70.87500000273118417, -35.31076352940723240 ) ) ;
#10708=ORIENTED_EDGE ( 'NONE', *, *, #15565, .F. ) ;
#10713=CARTESIAN_POINT ( 'NONE',  ( 32.50000000000000711, 29.40000000546238823, 10.55989012756945122 ) ) ;
#10714=CARTESIAN_POINT ( 'NONE',  ( -10.37757302488623701, 61.52500000273120406, 31.93888565452638417 ) ) ;
#10716=CARTESIAN_POINT ( 'NONE',  ( 5.779280353836490358E-15, 67.00000000546236834, 32.49999999999999289 ) ) ;
#10717=CARTESIAN_POINT ( 'NONE',  ( -23.41746824999999887, 8.124999997268817609, -2.867812753649727150E-15 ) ) ;
#10718=CARTESIAN_POINT ( 'NONE',  ( 27.16883889988624290, 3.925000002731188431, 19.73931689729373673 ) ) ;
#10719=CARTESIAN_POINT ( 'NONE',  ( 33.58253175000000113, 28.47500000273118204, -10.91162601494193751 ) ) ;
#10722=CARTESIAN_POINT ( 'NONE',  ( -33.58253175000000113, 79.27500000273118985, -10.91162601494193218 ) ) ;
#10724=CARTESIAN_POINT ( 'NONE',  ( -20.08610463437157989, 69.69999999999997442, -27.64615127144129758 ) ) ;
#10729=CARTESIAN_POINT ( 'NONE',  ( -11.25946833292375793, 79.07500000273121543, 8.180482586598737171 ) ) ;
#10731=CARTESIAN_POINT ( 'NONE',  ( -10.37757302488623701, 27.52500000273119696, 31.93888565452638417 ) ) ;
#10734=CARTESIAN_POINT ( 'NONE',  ( 33.58253175000000113, 12.47500000273119447, -10.91162601494193574 ) ) ;
#10737=CARTESIAN_POINT ( 'NONE',  ( -20.75514604977248823, 68.82500000273118701, -28.56700777964554305 ) ) ;
#10738=CARTESIAN_POINT ( 'NONE',  ( 26.29305231718579350, 59.30000000546237260, 19.10302069950537529 ) ) ;
#10740=DIRECTION ( 'NONE',  ( -0.000000000000000000, -1.000000000000000000, -0.000000000000000000 ) ) ;
#10741=CARTESIAN_POINT ( 'NONE',  ( -33.58253175000000113, 61.02500000273118985, -10.91162601494193041 ) ) ;
#10743=ADVANCED_FACE ( 'NONE', ( #21656 ), #6364, .T. ) ;
#10744=ORIENTED_EDGE ( 'NONE', *, *, #15171, .F. ) ;
#10748=CARTESIAN_POINT ( 'NONE',  ( -7.236395654485757944, 1.224999997268799712, -22.27133577429736988 ) ) ;
#10757=CARTESIAN_POINT ( 'NONE',  ( 20.08610463437157279, 27.80000000546238326, -27.64615127144129758 ) ) ;
#10759=CARTESIAN_POINT ( 'NONE',  ( 15.14183272437241889, 1.700000000000004396, 20.84094480462498211 ) ) ;
#10760=CARTESIAN_POINT ( 'NONE',  ( 27.16883889988623935, 8.575000002731202997, -19.73931689729374384 ) ) ;
#10761=CARTESIAN_POINT ( 'NONE',  ( -20.08610463437157989, 57.70000000000000284, -27.64615127144129758 ) ) ;
#10762=CARTESIAN_POINT ( 'NONE',  ( 32.50000000000000000, 57.50000000546237544, -3.980102097228898626E-15 ) ) ;
#10763=CARTESIAN_POINT ( 'NONE',  ( -26.29305231718578995, 30.20000000000000284, 19.10302069950538595 ) ) ;
#10766=CARTESIAN_POINT ( 'NONE',  ( -13.91746824999999887, 75.37500000273116996, 0.000000000000000000 ) ) ;
#10769=CARTESIAN_POINT ( 'NONE',  ( 3.980102097228898626E-15, 80.00000000000001421, 32.50000000000000000 ) ) ;
#10770=CARTESIAN_POINT ( 'NONE',  ( -1.053607264507113999E-13, 64.50000000000000000, 32.50000000000000711 ) ) ;
#10771=CARTESIAN_POINT ( 'NONE',  ( -32.50000000000000000, 4.099999999999986322, 10.55989012756946366 ) ) ;
#10774=CARTESIAN_POINT ( 'NONE',  ( 10.37757302488624767, 43.72500000273119269, 31.93888565452638417 ) ) ;
#10777=CARTESIAN_POINT ( 'NONE',  ( -10.37757302488624411, 34.97500000273118559, -31.93888565452638417 ) ) ;
#10778=CARTESIAN_POINT ( 'NONE',  ( 26.29305231718579350, 24.79999999999999005, 19.10302069950537529 ) ) ;
#10780=CARTESIAN_POINT ( 'NONE',  ( -5.147494310547377161, 61.55125428154684641, -32.50000000000002132 ) ) ;
#10781=CARTESIAN_POINT ( 'NONE',  ( 5.779280353836490358E-15, 23.00000000546237899, 32.49999999999999289 ) ) ;
#10785=CARTESIAN_POINT ( 'NONE',  ( 5.779280353836490358E-15, 40.49999999999999289, 32.49999999999999289 ) ) ;
#10788=( BOUNDED_SURFACE ( )  B_SPLINE_SURFACE ( 1, 2, ( 
 ( #7738, #7910, #20966, #31417, #1903, #12380, #22848, #33307, #15304, #30729, #7223, #4655, #20455, #30906, #7400, #17886, #21924, #11613, #30129, #19187, #19354, #10659, #15820, #808, #26274, #32374, #24494, #22261, #14200, #6128, #29966, #1299, #2763, #16945, #21138, #967, #24655, #8870, #19518, #14032, #3559, #19683, #16776, #13868, #18564, #11781, #31579, #11448, #3729, #24333, #32703, #27236, #16612, #9198, #29796, #6300, #27403, #6473, #1128, #13228, #27065, #22095, #23703, #32539, #9039, #14364, #29625, #3892, #24821, #169, #8078, #29007, #5970, #16447, #26899, #11289, #3398, #21768, #32211, #8704, #6969, #28253, #1475, #27914, #30641, #27739, #6632, #25511, #6799, #12290, #7309, #17454, #4397, #22763, #22936, #15047, #17278, #14531, #30298, #4736, #33216, #14871, #33392, #25335, #20198, #25680, #32867, #1813, #4229, #14703, #9715, #7138, #9891, #25161, #28080, #1991, #24992, #1639, #23104, #17619, #20368, #20024, #33568, #4569, #12466, #30817, #17794, #12634, #15217, #2160, #10066, #20546, #17111, #27570, #4058, #11949, #22418, #9364, #19846, #12115, #22587, #33039, #9543, #30470, #10578, #10243, #2851, #23963, #13148, #28422, #12981, #5084, #23622, #13322, #90, #31164, #33748, #4911, #7999, #15569, #26193, #5426, #12810, #28927, #7656, #20723, #26532, #23282, #23455, #29091, #25847, #10406, #10917, #2688, #21056, #31506, #18143, #5595, #15391, #261, #28586 ),
 ( #18483, #31334, #13497, #15738, #15906, #31669, #10748, #18315, #30992, #20885, #26362, #3026, #23795, #21225, #16077, #7826, #28761, #8163, #18653, #7491, #33917, #433, #2337, #17971, #26023, #2514, #5257, #29587, #14326, #21727, #8999, #16244, #8665, #11410, #8497, #21389, #6260, #21557, #27026, #22054, #32172, #19149, #3521, #3687, #29755, #32001, #29260, #11086, #19480, #13994, #6089, #14161, #16571, #930, #6432, #13665, #24455, #18985, #29429, #21886, #32336, #24617, #5932, #8829, #16739, #5764, #16410, #3851, #19313, #1091, #769, #24782, #27197, #11574, #32499, #29929, #27366, #16904, #1260, #31834, #8328, #18817, #26699, #3196, #24129, #595, #26863, #3358, #13828, #24297, #11250, #7101, #17414, #30432, #4019, #1771, #14663, #19646, #6931, #19809, #25123, #22546, #1601, #9504, #11911, #19985, #32997, #27531, #22383, #30088, #27876, #17241, #4360, #14835, #4532, #6594, #25301, #14493, #9679, #4191, #30605, #12251, #22728, #24951, #33177, #1954, #27701, #20161, #17584, #30259, #28045, #9162, #15006, #12428, #9322, #17071, #22220, #6762, #25475, #11740, #1432, #32832, #32667, #12078, #9996, #14799, #9819, #1567, #22863, #28010, #20469, #14972, #30744, #2264, #9468, #25440, #17378, #4325, #20296, #4496, #30921, #25264, #4668, #12566, #12043, #6897, #33671, #12393, #7414, #30571, #10168, #1916, #33321, #17900, #15148, #23209, #7235, #28181, #12738, #17723, #25612 ) ),
 .UNSPECIFIED., .F., .F., .T. ) 
 B_SPLINE_SURFACE_WITH_KNOTS ( ( 2, 2 ),
 ( 3, 2, 2, 2, 2, 2, 2, 2, 2, 2, 2, 2, 2, 2, 2, 2, 2, 2, 2, 2, 2, 2, 2, 2, 2, 2, 2, 2, 2, 2, 2, 2, 2, 2, 2, 2, 2, 2, 2, 2, 2, 2, 2, 2, 2, 2, 2, 2, 2, 2, 2, 2, 2, 2, 2, 2, 2, 2, 2, 2, 2, 2, 2, 2, 2, 2, 2, 2, 2, 2, 2, 2, 2, 2, 2, 2, 2, 2, 2, 2, 2, 2, 2, 2, 2, 2, 2, 2, 2, 2, 3 ),
 ( 0.000000000000000000, 1.000000000000000000 ),
 ( 0.000000000000000000, 0.01111111111111111154, 0.02222222222222222307, 0.03333333333333333287, 0.04444444444444444614, 0.05555555555555555247, 0.06666666666666666574, 0.07777777777777777901, 0.08888888888888889228, 0.1000000000000000056, 0.1111111111111111049, 0.1222222222222222182, 0.1333333333333333315, 0.1444444444444444309, 0.1555555555555555580, 0.1666666666666666574, 0.1777777777777777846, 0.1888888888888888840, 0.2000000000000000111, 0.2111111111111111105, 0.2222222222222222099, 0.2333333333333333370, 0.2444444444444444364, 0.2555555555555555358, 0.2666666666666666630, 0.2777777777777777901, 0.2888888888888888618, 0.2999999999999999889, 0.3111111111111111160, 0.3222222222222222432, 0.3333333333333333148, 0.3444444444444444420, 0.3555555555555555691, 0.3666666666666666408, 0.3777777777777777679, 0.3888888888888888951, 0.4000000000000000222, 0.4111111111111110938, 0.4222222222222222210, 0.4333333333333333481, 0.4444444444444444198, 0.4555555555555555469, 0.4666666666666666741, 0.4777777777777778012, 0.4888888888888888729, 0.5000000000000000000, 0.5111111111111110716, 0.5222222222222222543, 0.5333333333333333259, 0.5444444444444443976, 0.5555555555555555802, 0.5666666666666666519, 0.5777777777777777235, 0.5888888888888889062, 0.5999999999999999778, 0.6111111111111111605, 0.6222222222222222321, 0.6333333333333333037, 0.6444444444444444864, 0.6555555555555555580, 0.6666666666666666297, 0.6777777777777778123, 0.6888888888888888840, 0.6999999999999999556, 0.7111111111111111382, 0.7222222222222222099, 0.7333333333333332815, 0.7444444444444444642, 0.7555555555555555358, 0.7666666666666667185, 0.7777777777777777901, 0.7888888888888888618, 0.8000000000000000444, 0.8111111111111111160, 0.8222222222222221877, 0.8333333333333333703, 0.8444444444444444420, 0.8555555555555555136, 0.8666666666666666963, 0.8777777777777777679, 0.8888888888888888395, 0.9000000000000000222, 0.9111111111111110938, 0.9222222222222222765, 0.9333333333333333481, 0.9444444444444444198, 0.9555555555555556024, 0.9666666666666666741, 0.9777777777777777457, 0.9888888888888889284, 1.000000000000000000 ),
 .UNSPECIFIED. ) 
 GEOMETRIC_REPRESENTATION_ITEM ( )  RATIONAL_B_SPLINE_SURFACE ( (
 ( 1.000000000000000000, 0.9510565162951535312, 1.000000000000000000, 0.9510565162951535312, 1.000000000000000000, 0.9510565162951535312, 1.000000000000000000, 0.9510565162951535312, 1.000000000000000000, 0.9510565162951535312, 1.000000000000000000, 0.9510565162951535312, 1.000000000000000000, 0.9510565162951535312, 1.000000000000000000, 0.9510565162951535312, 1.000000000000000000, 0.9510565162951535312, 1.000000000000000000, 0.9510565162951535312, 1.000000000000000000, 0.9510565162951535312, 1.000000000000000000, 0.9510565162951535312, 1.000000000000000000, 0.9510565162951535312, 1.000000000000000000, 0.9510565162951535312, 1.000000000000000000, 0.9510565162951535312, 1.000000000000000000, 0.9510565162951535312, 1.000000000000000000, 0.9510565162951535312, 1.000000000000000000, 0.9510565162951535312, 1.000000000000000000, 0.9510565162951535312, 1.000000000000000000, 0.9510565162951535312, 1.000000000000000000, 0.9510565162951535312, 1.000000000000000000, 0.9510565162951535312, 1.000000000000000000, 0.9510565162951535312, 1.000000000000000000, 0.9510565162951535312, 1.000000000000000000, 0.9510565162951535312, 1.000000000000000000, 0.9510565162951535312, 1.000000000000000000, 0.9510565162951535312, 1.000000000000000000, 0.9510565162951535312, 1.000000000000000000, 0.9510565162951535312, 1.000000000000000000, 0.9510565162951535312, 1.000000000000000000, 0.9510565162951535312, 1.000000000000000000, 0.9510565162951535312, 1.000000000000000000, 0.9510565162951535312, 1.000000000000000000, 0.9510565162951535312, 1.000000000000000000, 0.9510565162951535312, 1.000000000000000000, 0.9510565162951535312, 1.000000000000000000, 0.9510565162951535312, 1.000000000000000000, 0.9510565162951535312, 1.000000000000000000, 0.9510565162951535312, 1.000000000000000000, 0.9510565162951535312, 1.000000000000000000, 0.9510565162951535312, 1.000000000000000000, 0.9510565162951535312, 1.000000000000000000, 0.9510565162951535312, 1.000000000000000000, 0.9510565162951535312, 1.000000000000000000, 0.9510565162951535312, 1.000000000000000000, 0.9510565162951535312, 1.000000000000000000, 0.9510565162951535312, 1.000000000000000000, 0.9510565162951535312, 1.000000000000000000, 0.9510565162951535312, 1.000000000000000000, 0.9510565162951535312, 1.000000000000000000, 0.9510565162951535312, 1.000000000000000000, 0.9510565162951535312, 1.000000000000000000, 0.9510565162951535312, 1.000000000000000000, 0.9510565162951535312, 1.000000000000000000, 0.9510565162951535312, 1.000000000000000000, 0.9510565162951535312, 1.000000000000000000, 0.9510565162951535312, 1.000000000000000000, 0.9510565162951535312, 1.000000000000000000, 0.9510565162951535312, 1.000000000000000000, 0.9510565162951535312, 1.000000000000000000, 0.9510565162951535312, 1.000000000000000000, 0.9510565162951535312, 1.000000000000000000, 0.9510565162951535312, 1.000000000000000000, 0.9510565162951535312, 1.000000000000000000, 0.9510565162951535312, 1.000000000000000000, 0.9510565162951535312, 1.000000000000000000, 0.9510565162951535312, 1.000000000000000000, 0.9510565162951535312, 1.000000000000000000, 0.9510565162951535312, 1.000000000000000000, 0.9510565162951535312, 1.000000000000000000, 0.9510565162951535312, 1.000000000000000000, 0.9510565162951535312, 1.000000000000000000, 0.9510565162951535312, 1.000000000000000000, 0.9510565162951535312, 1.000000000000000000, 0.9510565162951535312, 1.000000000000000000, 0.9510565162951535312, 1.000000000000000000, 0.9510565162951535312, 1.000000000000000000, 0.9510565162951535312, 1.000000000000000000, 0.9510565162951535312, 1.000000000000000000, 0.9510565162951535312, 1.000000000000000000, 0.9510565162951535312, 1.000000000000000000, 0.9510565162951535312, 1.000000000000000000, 0.9510565162951535312, 1.000000000000000000, 0.9510565162951535312, 1.000000000000000000, 0.9510565162951535312, 1.000000000000000000, 0.9510565162951535312, 1.000000000000000000, 0.9510565162951535312, 1.000000000000000000, 0.9510565162951535312, 1.000000000000000000, 0.9510565162951535312, 1.000000000000000000, 0.9510565162951535312, 1.000000000000000000),
 ( 1.000000000000000000, 0.9510565162951535312, 1.000000000000000000, 0.9510565162951535312, 1.000000000000000000, 0.9510565162951535312, 1.000000000000000000, 0.9510565162951535312, 1.000000000000000000, 0.9510565162951535312, 1.000000000000000000, 0.9510565162951535312, 1.000000000000000000, 0.9510565162951535312, 1.000000000000000000, 0.9510565162951535312, 1.000000000000000000, 0.9510565162951535312, 1.000000000000000000, 0.9510565162951535312, 1.000000000000000000, 0.9510565162951535312, 1.000000000000000000, 0.9510565162951535312, 1.000000000000000000, 0.9510565162951535312, 1.000000000000000000, 0.9510565162951535312, 1.000000000000000000, 0.9510565162951535312, 1.000000000000000000, 0.9510565162951535312, 1.000000000000000000, 0.9510565162951535312, 1.000000000000000000, 0.9510565162951535312, 1.000000000000000000, 0.9510565162951535312, 1.000000000000000000, 0.9510565162951535312, 1.000000000000000000, 0.9510565162951535312, 1.000000000000000000, 0.9510565162951535312, 1.000000000000000000, 0.9510565162951535312, 1.000000000000000000, 0.9510565162951535312, 1.000000000000000000, 0.9510565162951535312, 1.000000000000000000, 0.9510565162951535312, 1.000000000000000000, 0.9510565162951535312, 1.000000000000000000, 0.9510565162951535312, 1.000000000000000000, 0.9510565162951535312, 1.000000000000000000, 0.9510565162951535312, 1.000000000000000000, 0.9510565162951535312, 1.000000000000000000, 0.9510565162951535312, 1.000000000000000000, 0.9510565162951535312, 1.000000000000000000, 0.9510565162951535312, 1.000000000000000000, 0.9510565162951535312, 1.000000000000000000, 0.9510565162951535312, 1.000000000000000000, 0.9510565162951535312, 1.000000000000000000, 0.9510565162951535312, 1.000000000000000000, 0.9510565162951535312, 1.000000000000000000, 0.9510565162951535312, 1.000000000000000000, 0.9510565162951535312, 1.000000000000000000, 0.9510565162951535312, 1.000000000000000000, 0.9510565162951535312, 1.000000000000000000, 0.9510565162951535312, 1.000000000000000000, 0.9510565162951535312, 1.000000000000000000, 0.9510565162951535312, 1.000000000000000000, 0.9510565162951535312, 1.000000000000000000, 0.9510565162951535312, 1.000000000000000000, 0.9510565162951535312, 1.000000000000000000, 0.9510565162951535312, 1.000000000000000000, 0.9510565162951535312, 1.000000000000000000, 0.9510565162951535312, 1.000000000000000000, 0.9510565162951535312, 1.000000000000000000, 0.9510565162951535312, 1.000000000000000000, 0.9510565162951535312, 1.000000000000000000, 0.9510565162951535312, 1.000000000000000000, 0.9510565162951535312, 1.000000000000000000, 0.9510565162951535312, 1.000000000000000000, 0.9510565162951535312, 1.000000000000000000, 0.9510565162951535312, 1.000000000000000000, 0.9510565162951535312, 1.000000000000000000, 0.9510565162951535312, 1.000000000000000000, 0.9510565162951535312, 1.000000000000000000, 0.9510565162951535312, 1.000000000000000000, 0.9510565162951535312, 1.000000000000000000, 0.9510565162951535312, 1.000000000000000000, 0.9510565162951535312, 1.000000000000000000, 0.9510565162951535312, 1.000000000000000000, 0.9510565162951535312, 1.000000000000000000, 0.9510565162951535312, 1.000000000000000000, 0.9510565162951535312, 1.000000000000000000, 0.9510565162951535312, 1.000000000000000000, 0.9510565162951535312, 1.000000000000000000, 0.9510565162951535312, 1.000000000000000000, 0.9510565162951535312, 1.000000000000000000, 0.9510565162951535312, 1.000000000000000000, 0.9510565162951535312, 1.000000000000000000, 0.9510565162951535312, 1.000000000000000000, 0.9510565162951535312, 1.000000000000000000, 0.9510565162951535312, 1.000000000000000000, 0.9510565162951535312, 1.000000000000000000, 0.9510565162951535312, 1.000000000000000000, 0.9510565162951535312, 1.000000000000000000, 0.9510565162951535312, 1.000000000000000000, 0.9510565162951535312, 1.000000000000000000, 0.9510565162951535312, 1.000000000000000000, 0.9510565162951535312, 1.000000000000000000, 0.9510565162951535312, 1.000000000000000000, 0.9510565162951535312, 1.000000000000000000, 0.9510565162951535312, 1.000000000000000000) ) ) 
 REPRESENTATION_ITEM ( '' )  SURFACE ( )  );
#10789=CARTESIAN_POINT ( 'NONE',  ( 32.50000000000000000, 11.00000000000001066, -3.980102097228898626E-15 ) ) ;
#10790=CARTESIAN_POINT ( 'NONE',  ( 20.75514604977249178, 19.82500000273119412, 28.56700777964553950 ) ) ;
#10792=ORIENTED_EDGE ( 'NONE', *, *, #2764, .F. ) ;
#10794=ORIENTED_EDGE ( 'NONE', *, *, #4749, .T. ) ;
#10799=CARTESIAN_POINT ( 'NONE',  ( 5.779280353836490358E-15, 44.49999999999999289, 32.49999999999999289 ) ) ;
#10800=CARTESIAN_POINT ( 'NONE',  ( 33.58253175000000113, 26.47500000273118559, -10.91162601494193751 ) ) ;
#10801=CARTESIAN_POINT ( 'NONE',  ( -20.08610463437156923, 34.80000000546240102, 27.64615127144130113 ) ) ;
#10805=CARTESIAN_POINT ( 'NONE',  ( 20.75514604977248467, 40.67500000273116711, -28.56700777964554305 ) ) ;
#10808=CARTESIAN_POINT ( 'NONE',  ( 26.29305231718578995, 21.19999999999999574, -19.10302069950538240 ) ) ;
#10810=CARTESIAN_POINT ( 'NONE',  ( -33.58253175000000113, 69.02500000273118985, -10.91162601494193218 ) ) ;
#10813=CARTESIAN_POINT ( 'NONE',  ( -10.37757302488624411, 52.97500000273119980, -31.93888565452638417 ) ) ;
#10815=CARTESIAN_POINT ( 'NONE',  ( 26.29305231718579350, 7.300000005462381480, 19.10302069950537529 ) ) ;
#10816=CARTESIAN_POINT ( 'NONE',  ( 33.58253175000000113, 10.12500000273119838, -4.112674001490185761E-15 ) ) ;
#10821=CARTESIAN_POINT ( 'NONE',  ( -32.50000000000000000, 18.60000000546238397, 10.55989012756946366 ) ) ;
#10829=CARTESIAN_POINT ( 'NONE',  ( 26.29305231718578995, 67.70000000546238539, -19.10302069950538240 ) ) ;
#10833=ORIENTED_EDGE ( 'NONE', *, *, #9249, .T. ) ;
#10836=ADVANCED_FACE ( 'NONE', ( #1369 ), #27466, .T. ) ;
#10839=CARTESIAN_POINT ( 'NONE',  ( -20.75514604977248112, 51.67500000273117422, 28.56700777964554661 ) ) ;
#10840=CARTESIAN_POINT ( 'NONE',  ( 32.50000000000000000, 57.50000000546237544, -3.980102097228898626E-15 ) ) ;
#10842=CARTESIAN_POINT ( 'NONE',  ( -20.75514604977248112, 37.42500000273118843, 28.56700777964554661 ) ) ;
#10843=CARTESIAN_POINT ( 'NONE',  ( 32.50000000000000000, 55.09999999999997300, -10.55989012756945833 ) ) ;
#10844=CARTESIAN_POINT ( 'NONE',  ( -20.75514604977248823, 65.07500000273118701, -28.56700777964554305 ) ) ;
#10846=ADVANCED_FACE ( 'NONE', ( #11186 ), #3456, .T. ) ;
#10848=EDGE_CURVE ( 'NONE', #23926, #32333, #6467, .T. ) ;
#10850=CARTESIAN_POINT ( 'NONE',  ( 26.29305231718579350, 38.80000000000000426, 19.10302069950537529 ) ) ;
#10852=CARTESIAN_POINT ( 'NONE',  ( -33.58253175000000113, 11.27500000273117031, -10.91162601494193218 ) ) ;
#10853=DIRECTION ( 'NONE',  ( 0.000000000000000000, 0.000000000000000000, 1.000000000000000000 ) ) ;
#10855=CYLINDRICAL_SURFACE ( 'NONE', #26495, 15.00000000000000000 ) ;
#10856=CARTESIAN_POINT ( 'NONE',  ( 27.16883889988624290, 70.17500000273119554, 19.73931689729373673 ) ) ;
#10857=DIRECTION ( 'NONE',  ( 0.000000000000000000, 0.000000000000000000, -1.000000000000000000 ) ) ;
#10870=CARTESIAN_POINT ( 'NONE',  ( -32.50000000000000000, 56.60000000546236976, 10.55989012756946366 ) ) ;
#10871=CARTESIAN_POINT ( 'NONE',  ( 33.58253175000000823, 38.02500000273117564, 10.91162601494192685 ) ) ;
#10875=ORIENTED_EDGE ( 'NONE', *, *, #19034, .F. ) ;
#10879=CARTESIAN_POINT ( 'NONE',  ( 20.75514604977249178, 68.07500000273118701, 28.56700777964553950 ) ) ;
#10885=CARTESIAN_POINT ( 'NONE',  ( 33.58253175000000113, 52.22500000273117848, -10.91162601494193751 ) ) ;
#10887=( BOUNDED_CURVE ( )  B_SPLINE_CURVE ( 2, ( #27365, #24950, #12077, #27196, #30256, #29928, #22053, #25300, #9503, #14325, #6930, #25122, #19984 ),
 .UNSPECIFIED., .F., .F. ) 
 B_SPLINE_CURVE_WITH_KNOTS ( ( 3, 2, 2, 2, 2, 2, 3 ),
 ( 0.8012820512820513219, 0.8025641025641025994, 0.8051282051282051544, 0.8076923076923077094, 0.8102564102564102644, 0.8128205128205128194, 0.8141025641025640969 ),
 .UNSPECIFIED. ) 
 CURVE ( )  GEOMETRIC_REPRESENTATION_ITEM ( )  RATIONAL_B_SPLINE_CURVE ( ( 0.9755282581475768211, 0.9755282581475768211, 1.000000000000000000, 0.9510565162951535312, 1.000000000000000000, 0.9510565162951535312, 1.000000000000000000, 0.9510565162951535312, 1.000000000000000000, 0.9510565162951535312, 1.000000000000000000, 0.9755282581475768211, 0.9755282581475768211 ) ) 
 REPRESENTATION_ITEM ( '' )  );
#10888=CARTESIAN_POINT ( 'NONE',  ( 32.50000000000000000, 17.60000000546238397, -10.55989012756945833 ) ) ;
#10890=CARTESIAN_POINT ( 'NONE',  ( 23.41746824999999887, 9.024999997268826846, 7.608796670333735079 ) ) ;
#10892=CARTESIAN_POINT ( 'NONE',  ( 6.486482029760649416E-15, 29.87500000273119838, 35.31076352940723240 ) ) ;
#10895=CARTESIAN_POINT ( 'NONE',  ( 13.91746824999999532, 77.97500000273119269, -4.522059556121118540 ) ) ;
#10896=CARTESIAN_POINT ( 'NONE',  ( -32.50000000000000000, 69.90000000000000568, -10.55989012756945300 ) ) ;
#10900=CARTESIAN_POINT ( 'NONE',  ( 11.25946833292375793, 74.07500000273120122, -8.180482586598735395 ) ) ;
#10902=EDGE_CURVE ( 'NONE', #8956, #12338, #24391, .T. ) ;
#10903=CARTESIAN_POINT ( 'NONE',  ( 33.58253175000000113, 24.22500000273119625, -10.91162601494193751 ) ) ;
#10906=CARTESIAN_POINT ( 'NONE',  ( -10.37757302488624411, 16.97500000273119269, -31.93888565452638417 ) ) ;
#10908=CARTESIAN_POINT ( 'NONE',  ( -10.37757302488624411, 70.72500000273119269, -31.93888565452638417 ) ) ;
#10909=CARTESIAN_POINT ( 'NONE',  ( 32.50000000000000000, 3.500000005462383434, -3.980102097228898626E-15 ) ) ;
#10912=CARTESIAN_POINT ( 'NONE',  ( -10.37757302488623701, 59.52500000273119696, 31.93888565452638417 ) ) ;
#10914=ORIENTED_EDGE ( 'NONE', *, *, #19531, .F. ) ;
#10916=CARTESIAN_POINT ( 'NONE',  ( 10.37757302488624056, 2.525000002731203619, -31.93888565452638417 ) ) ;
#10917=CARTESIAN_POINT ( 'NONE',  ( -18.94512977948576093, 18.32499999726880446, 13.76444248337722698 ) ) ;
#10919=EDGE_LOOP ( 'NONE', ( #30691, #23566, #32455, #26359 ) ) ;
#10921=CARTESIAN_POINT ( 'NONE',  ( -32.50000000000000000, 42.50000000546238965, 0.000000000000000000 ) ) ;
#10922=ORIENTED_EDGE ( 'NONE', *, *, #19623, .T. ) ;
#10924=CARTESIAN_POINT ( 'NONE',  ( -4.223320258572821363E-15, 78.75000000546238255, 15.00000000000000355 ) ) ;
#10926=CARTESIAN_POINT ( 'NONE',  ( 23.41746824999999887, 18.62499999726882649, 0.000000000000000000 ) ) ;
#10927=CARTESIAN_POINT ( 'NONE',  ( -10.37757302488624411, 10.97500000273118914, -31.93888565452638417 ) ) ;
#10928=CARTESIAN_POINT ( 'NONE',  ( 32.50000000000000711, 58.90000000000000568, 10.55989012756945122 ) ) ;
#10929=CARTESIAN_POINT ( 'NONE',  ( 13.91746824999999887, 77.87500000273116996, -1.704398294459741270E-15 ) ) ;
#10932=CARTESIAN_POINT ( 'NONE',  ( -8.960552108402742093E-16, 76.87500000273115575, -14.63369212191046387 ) ) ;
#10935=FACE_OUTER_BOUND ( 'NONE', #14921, .T. ) ;
#10936=CARTESIAN_POINT ( 'NONE',  ( -27.16883889988624290, 79.17500000273119554, -19.73931689729374028 ) ) ;
#10940=CARTESIAN_POINT ( 'NONE',  ( 10.37757302488624056, 46.52500000273118985, -31.93888565452638417 ) ) ;
#10943=CARTESIAN_POINT ( 'NONE',  ( -27.16883889988623935, 37.57500000273117280, 19.73931689729374739 ) ) ;
#10944=CARTESIAN_POINT ( 'NONE',  ( 32.50000000000000000, 23.50000000546237544, -3.980102097228898626E-15 ) ) ;
#10945=EDGE_CURVE ( 'NONE', #33751, #6723, #14430, .T. ) ;
#10947=CARTESIAN_POINT ( 'NONE',  ( -5.147494310547423346, 18.44874571845315003, 32.50000000000000000 ) ) ;
#10948=CARTESIAN_POINT ( 'NONE',  ( -9.270509831248419985, 76.30000000000001137, 12.75976212528060039 ) ) ;
#10951=CARTESIAN_POINT ( 'NONE',  ( -4.523095164977117273E-15, 6.124999997268802510, 24.62258325217400312 ) ) ;
#10954=CARTESIAN_POINT ( 'NONE',  ( -2.375766604868048137, 76.69874572391553613, 14.99999999999999822 ) ) ;
#10955=CARTESIAN_POINT ( 'NONE',  ( -27.16883889988624290, 20.92500000273117422, -19.73931689729374028 ) ) ;
#10957=VERTEX_POINT ( 'NONE', #24885 ) ;
#10959=ORIENTED_EDGE ( 'NONE', *, *, #32068, .T. ) ;
#10964=VERTEX_POINT ( 'NONE', #11346 ) ;
#10966=CARTESIAN_POINT ( 'NONE',  ( -27.16883889988623935, 25.57500000273119056, 19.73931689729374739 ) ) ;
#10967=CARTESIAN_POINT ( 'NONE',  ( 32.50000000000000711, 29.40000000546239178, 10.55989012756945122 ) ) ;
#10968=CARTESIAN_POINT ( 'NONE',  ( -10.04305231718579172, 79.60000000000000853, -30.90933677959248982 ) ) ;
#10969=CARTESIAN_POINT ( 'NONE',  ( 3.980102097228898626E-15, 80.00000000000001421, 32.50000000000000000 ) ) ;
#10970=CARTESIAN_POINT ( 'NONE',  ( 5.147494310547426899, 37.94874572391552192, -32.50000000000000000 ) ) ;
#10971=CARTESIAN_POINT ( 'NONE',  ( 27.16883889988624290, 42.17500000273119554, 19.73931689729373673 ) ) ;
#10974=CARTESIAN_POINT ( 'NONE',  ( 6.277390505771533514E-15, 20.49999999999999289, 34.17252228774368916 ) ) ;
#10976=CARTESIAN_POINT ( 'NONE',  ( -20.75514604977248112, 61.42500000273118133, 28.56700777964554661 ) ) ;
#10978=CARTESIAN_POINT ( 'NONE',  ( -32.50000000000000000, 76.60000000546236265, 10.55989012756946366 ) ) ;
#10979=CARTESIAN_POINT ( 'NONE',  ( 27.16883889988623935, 54.57500000273118701, -19.73931689729374384 ) ) ;
#10981=CARTESIAN_POINT ( 'NONE',  ( 0.000000000000000000, 80.00000000000001421, -32.50000000000000000 ) ) ;
#10982=CARTESIAN_POINT ( 'NONE',  ( -27.16883889988624290, 4.925000002731189319, -19.73931689729374028 ) ) ;
#10985=( BOUNDED_CURVE ( )  B_SPLINE_CURVE ( 2, ( #25875, #21085, #23653, #18844, #23483, #23990, #290, #31534, #10778, #20911, #10436, #8027, #26392 ),
 .UNSPECIFIED., .F., .F. ) 
 B_SPLINE_CURVE_WITH_KNOTS ( ( 3, 2, 2, 2, 2, 2, 3 ),
 ( 0.6987179487179486781, 0.6999999999999999556, 0.7025641025641025106, 0.7051282051282051766, 0.7076923076923077316, 0.7102564102564102866, 0.7115384615384615641 ),
 .UNSPECIFIED. ) 
 CURVE ( )  GEOMETRIC_REPRESENTATION_ITEM ( )  RATIONAL_B_SPLINE_CURVE ( ( 0.9755282581475768211, 0.9755282581475768211, 1.000000000000000000, 0.9510565162951535312, 1.000000000000000000, 0.9510565162951535312, 1.000000000000000000, 0.9510565162951535312, 1.000000000000000000, 0.9510565162951535312, 1.000000000000000000, 0.9755282581475768211, 0.9755282581475768211 ) ) 
 REPRESENTATION_ITEM ( '' )  );
#10986=CARTESIAN_POINT ( 'NONE',  ( 5.147494310547643614, 25.94874572391553258, -32.49999999999992895 ) ) ;
#10995=CARTESIAN_POINT ( 'NONE',  ( 10.04305231718578817, 49.39999999999999858, -30.90933677959249337 ) ) ;
#10996=CARTESIAN_POINT ( 'NONE',  ( 10.04305231718578817, 61.40000000000001279, -30.90933677959249337 ) ) ;
#10999=CARTESIAN_POINT ( 'NONE',  ( -32.50000000000000000, 72.60000000546236265, 10.55989012756946366 ) ) ;
#11007=FACE_OUTER_BOUND ( 'NONE', #11871, .T. ) ;
#11008=CARTESIAN_POINT ( 'NONE',  ( 10.37757302488624056, 46.77500000273118985, -31.93888565452638417 ) ) ;
#11009=CARTESIAN_POINT ( 'NONE',  ( 32.50000000000000000, 59.50000000546237544, -3.980102097228898626E-15 ) ) ;
#11011=CARTESIAN_POINT ( 'NONE',  ( 10.37757302488624056, 36.52500000273117564, -31.93888565452638417 ) ) ;
#11012=DIRECTION ( 'NONE',  ( -0.000000000000000000, -1.000000000000000000, -0.000000000000000000 ) ) ;
#11013=CARTESIAN_POINT ( 'NONE',  ( -10.37757302488623701, 63.77500000273117564, 31.93888565452638417 ) ) ;
#11017=CARTESIAN_POINT ( 'NONE',  ( 32.50000000000000711, 42.90000000000001279, 10.55989012756945122 ) ) ;
#11019=CARTESIAN_POINT ( 'NONE',  ( -10.37757302488623701, 3.775000002731176973, 31.93888565452638417 ) ) ;
#11020=CARTESIAN_POINT ( 'NONE',  ( 5.779280353836490358E-15, 35.00000000546238255, 32.49999999999999289 ) ) ;
#11021=CARTESIAN_POINT ( 'NONE',  ( -33.04126587500000056, 78.81250000409679046, 0.000000000000000000 ) ) ;
#11022=CARTESIAN_POINT ( 'NONE',  ( -20.75514604977248112, 73.67500000273120975, 28.56700777964554661 ) ) ;
#11023=CARTESIAN_POINT ( 'NONE',  ( 24.50000000000000000, 3.749999994537622783, 0.000000000000000000 ) ) ;
#11025=VERTEX_POINT ( 'NONE', #22159 ) ;
#11026=( BOUNDED_CURVE ( )  B_SPLINE_CURVE ( 2, ( #20566, #12311, #25354, #22783, #28272, #12486, #22955, #33413, #1659, #9910, #1833, #7508, #33060 ),
 .UNSPECIFIED., .F., .T. ) 
 B_SPLINE_CURVE_WITH_KNOTS ( ( 3, 2, 2, 2, 2, 2, 3 ),
 ( 0.4423076923076922906, 0.4435897435897435681, 0.4461538461538461786, 0.4487179487179487336, 0.4512820512820512886, 0.4538461538461538436, 0.4551282051282051211 ),
 .UNSPECIFIED. ) 
 CURVE ( )  GEOMETRIC_REPRESENTATION_ITEM ( )  RATIONAL_B_SPLINE_CURVE ( ( 0.9755282581475768211, 0.9755282581475768211, 1.000000000000000000, 0.9510565162951535312, 1.000000000000000000, 0.9510565162951535312, 1.000000000000000000, 0.9510565162951535312, 1.000000000000000000, 0.9510565162951535312, 1.000000000000000000, 0.9755282581475768211, 0.9755282581475768211 ) ) 
 REPRESENTATION_ITEM ( '' )  );
#11027=FACE_OUTER_BOUND ( 'NONE', #13738, .T. ) ;
#11036=VECTOR ( 'NONE', #4434, 1000.000000000000000 ) ;
#11038=CARTESIAN_POINT ( 'NONE',  ( 27.16883889988624290, 35.92500000273118843, 19.73931689729373673 ) ) ;
#11041=EDGE_CURVE ( 'NONE', #11374, #7955, #24897, .T. ) ;
#11046=CARTESIAN_POINT ( 'NONE',  ( 10.04305231718578817, 51.39999999999999858, -30.90933677959249337 ) ) ;
#11050=CARTESIAN_POINT ( 'NONE',  ( -20.75514604977248112, 71.67500000273116711, 28.56700777964554661 ) ) ;
#11051=ORIENTED_EDGE ( 'NONE', *, *, #4371, .T. ) ;
#11053=EDGE_CURVE ( 'NONE', #25478, #15526, #27808, .T. ) ;
#11055=ORIENTED_EDGE ( 'NONE', *, *, #31228, .F. ) ;
#11056=CARTESIAN_POINT ( 'NONE',  ( 1.093617666956751375E-13, 66.00000000546238255, -32.50000000000000711 ) ) ;
#11057=CARTESIAN_POINT ( 'NONE',  ( 33.58253175000000823, 56.02500000273117564, 10.91162601494192863 ) ) ;
#11059=CARTESIAN_POINT ( 'NONE',  ( 10.04305231718578817, 19.90000000546238113, -30.90933677959249337 ) ) ;
#11061=CARTESIAN_POINT ( 'NONE',  ( 18.94512977948575738, 6.924999997268810326, 13.76444248337723408 ) ) ;
#11062=CARTESIAN_POINT ( 'NONE',  ( -10.37757302488623701, 21.77500000273119340, 31.93888565452638417 ) ) ;
#11065=CARTESIAN_POINT ( 'NONE',  ( 10.04305231718578817, 75.90000000546237402, -30.90933677959249337 ) ) ;
#11069=CARTESIAN_POINT ( 'NONE',  ( -8.601468415847518756, 78.57500000273120122, -11.83890561707634781 ) ) ;
#11071=CARTESIAN_POINT ( 'NONE',  ( -2.162160676586881955E-15, 26.62500000273118417, -35.31076352940723240 ) ) ;
#11075=CARTESIAN_POINT ( 'NONE',  ( -33.58253175000000113, 15.47500000273118381, 10.91162601494193929 ) ) ;
#11077=CARTESIAN_POINT ( 'NONE',  ( -10.37757302488623701, 71.52500000273120406, 31.93888565452638417 ) ) ;
#11081=CARTESIAN_POINT ( 'NONE',  ( 27.16883889988624290, 57.92500000273120975, 19.73931689729373673 ) ) ;
#11085=CARTESIAN_POINT ( 'NONE',  ( -20.75514604977248823, 2.825000002731177240, -28.56700777964554305 ) ) ;
#11086=CARTESIAN_POINT ( 'NONE',  ( -14.47279130897151589, 5.324999997268799135, -19.92008829642072598 ) ) ;
#11088=( BOUNDED_CURVE ( )  B_SPLINE_CURVE ( 2, ( #9508, #12082, #1438, #22550, #4537, #33002, #9003, #22059, #19484, #19650, #17419, #32503, #27536 ),
 .UNSPECIFIED., .F., .T. ) 
 B_SPLINE_CURVE_WITH_KNOTS ( ( 3, 2, 2, 2, 2, 2, 3 ),
 ( 0.3055555555555555802, 0.3111111111111111160, 0.3222222222222222432, 0.3333333333333333148, 0.3444444444444444420, 0.3555555555555555691, 0.3611111111111111049 ),
 .UNSPECIFIED. ) 
 CURVE ( )  GEOMETRIC_REPRESENTATION_ITEM ( )  RATIONAL_B_SPLINE_CURVE ( ( 0.9755282581475767101, 0.9755282581475768211, 1.000000000000000000, 0.9510565162951535312, 1.000000000000000000, 0.9510565162951535312, 1.000000000000000000, 0.9510565162951535312, 1.000000000000000000, 0.9510565162951535312, 1.000000000000000000, 0.9755282581475768211, 0.9755282581475768211 ) ) 
 REPRESENTATION_ITEM ( '' )  );
#11092=ORIENTED_EDGE ( 'NONE', *, *, #22664, .F. ) ;
#11093=( BOUNDED_CURVE ( )  B_SPLINE_CURVE ( 2, ( #27496, #3985, #32463, #17376, #14797, #25261, #14458, #1400, #11876, #13076, #30742, #23207, #26288 ),
 .UNSPECIFIED., .F., .T. ) 
 B_SPLINE_CURVE_WITH_KNOTS ( ( 3, 2, 2, 2, 2, 2, 3 ),
 ( 0.5833333333333332593, 0.5888888888888889062, 0.5999999999999999778, 0.6111111111111111605, 0.6222222222222222321, 0.6333333333333333037, 0.6388888888888889506 ),
 .UNSPECIFIED. ) 
 CURVE ( )  GEOMETRIC_REPRESENTATION_ITEM ( )  RATIONAL_B_SPLINE_CURVE ( ( 0.9755282581475768211, 0.9755282581475765991, 1.000000000000000000, 0.9510565162951535312, 1.000000000000000000, 0.9510565162951535312, 1.000000000000000000, 0.9510565162951535312, 1.000000000000000000, 0.9510565162951535312, 1.000000000000000000, 0.9755282581475765991, 0.9755282581475768211 ) ) 
 REPRESENTATION_ITEM ( '' )  );
#11095=CARTESIAN_POINT ( 'NONE',  ( -1.778240108872766143E-15, 12.00000000546238077, -32.49999999999999289 ) ) ;
#11097=CARTESIAN_POINT ( 'NONE',  ( -10.37757302488624411, 74.72500000273119269, -31.93888565452638417 ) ) ;
#11099=CARTESIAN_POINT ( 'NONE',  ( 24.50000000000000355, 7.900000000000012790, 7.960532557706212486 ) ) ;
#11100=CARTESIAN_POINT ( 'NONE',  ( 6.486482029760649416E-15, 7.875000002731193049, 35.31076352940723240 ) ) ;
#11101=CARTESIAN_POINT ( 'NONE',  ( -20.75514604977248823, 24.82500000273117635, -28.56700777964554305 ) ) ;
#11102=CARTESIAN_POINT ( 'NONE',  ( -13.91746824999999532, 76.97500000273119269, 4.522059556121122093 ) ) ;
#11105=CARTESIAN_POINT ( 'NONE',  ( 8.601468415847520532, 76.07500000273118701, 11.83890561707634781 ) ) ;
#11108=CARTESIAN_POINT ( 'NONE',  ( 5.779280353836490358E-15, 39.00000000546237544, 32.49999999999999289 ) ) ;
#11110=CARTESIAN_POINT ( 'NONE',  ( 27.16883889988624290, 41.92500000273119554, 19.73931689729373673 ) ) ;
#11114=CARTESIAN_POINT ( 'NONE',  ( 27.16883889988623935, 36.57500000273117280, -19.73931689729374384 ) ) ;
#11116=VECTOR ( 'NONE', #15845, 1000.000000000000000 ) ;
#11119=CARTESIAN_POINT ( 'NONE',  ( -5.147494310547531704, 44.94874572391552192, 32.49999999999996447 ) ) ;
#11122=CARTESIAN_POINT ( 'NONE',  ( 1.507698388325705758E-15, 3.124999997268809615, -24.62258325217400312 ) ) ;
#11125=CARTESIAN_POINT ( 'NONE',  ( -1.778240108872766143E-15, 59.50000000000000711, -32.49999999999999289 ) ) ;
#11126=CARTESIAN_POINT ( 'NONE',  ( 33.58253175000000113, 18.22500000273118559, -10.91162601494193574 ) ) ;
#11131=ORIENTED_EDGE ( 'NONE', *, *, #33267, .F. ) ;
#11136=ORIENTED_EDGE ( 'NONE', *, *, #22154, .F. ) ;
#11137=CARTESIAN_POINT ( 'NONE',  ( 23.41746824999999887, 0.6249999972688102812, 0.000000000000000000 ) ) ;
#11138=CARTESIAN_POINT ( 'NONE',  ( -20.75514604977248823, 31.07500000273118701, -28.56700777964554305 ) ) ;
#11139=CARTESIAN_POINT ( 'NONE',  ( 20.08610463437158344, 29.20000000546237118, 27.64615127144129403 ) ) ;
#11141=CARTESIAN_POINT ( 'NONE',  ( -32.50000000000000000, 54.40000000546238823, -10.55989012756945300 ) ) ;
#11143=CARTESIAN_POINT ( 'NONE',  ( 20.75514604977248467, 42.67500000273119554, -28.56700777964554305 ) ) ;
#11145=CARTESIAN_POINT ( 'NONE',  ( 26.29305231718579350, 18.79999999999998295, 19.10302069950537529 ) ) ;
#11147=CARTESIAN_POINT ( 'NONE',  ( -10.37757302488623701, 61.52500000273120406, 31.93888565452638417 ) ) ;
#11149=CARTESIAN_POINT ( 'NONE',  ( -33.58253175000000113, 53.37500000273118417, 0.000000000000000000 ) ) ;
#11152=CARTESIAN_POINT ( 'NONE',  ( 27.16883889988624290, 5.925000002731190207, 19.73931689729373673 ) ) ;
#11155=CARTESIAN_POINT ( 'NONE',  ( -10.04305231718579172, 19.60000000000000497, -30.90933677959248982 ) ) ;
#11160=CARTESIAN_POINT ( 'NONE',  ( -26.29305231718579350, 30.30000000546237260, -19.10302069950537884 ) ) ;
#11175=CARTESIAN_POINT ( 'NONE',  ( 20.75514604977248467, 44.67500000273118843, -28.56700777964554305 ) ) ;
#11176=CARTESIAN_POINT ( 'NONE',  ( 10.04305231718579705, 53.10000000546239107, 30.90933677959248982 ) ) ;
#11178=CARTESIAN_POINT ( 'NONE',  ( 27.16883889988624290, 35.92500000273118843, 19.73931689729373673 ) ) ;
#11179=LINE ( 'NONE', #21650, #7195 ) ;
#11180=CARTESIAN_POINT ( 'NONE',  ( 6.486482029760649416E-15, 63.87500000273119127, 35.31076352940723240 ) ) ;
#11181=AXIS2_PLACEMENT_3D ( 'NONE', #5705, #29200, #10857 ) ;
#11182=CARTESIAN_POINT ( 'NONE',  ( -2.092463501923844636E-15, 43.49999999999999289, -34.17252228774368916 ) ) ;
#11184=( BOUNDED_CURVE ( )  B_SPLINE_CURVE ( 2, ( #1676, #12151, #28455, #10277, #4945, #12503, #2029, #33785, #15081, #22971, #33430, #20918, #13182 ),
 .UNSPECIFIED., .F., .F. ) 
 B_SPLINE_CURVE_WITH_KNOTS ( ( 3, 2, 2, 2, 2, 2, 3 ),
 ( 0.1987179487179487336, 0.2000000000000000111, 0.2025641025641025661, 0.2051282051282051211, 0.2076923076923077038, 0.2102564102564102588, 0.2115384615384615363 ),
 .UNSPECIFIED. ) 
 CURVE ( )  GEOMETRIC_REPRESENTATION_ITEM ( )  RATIONAL_B_SPLINE_CURVE ( ( 0.9755282581475768211, 0.9755282581475770431, 1.000000000000000000, 0.9510565162951535312, 1.000000000000000000, 0.9510565162951535312, 1.000000000000000000, 0.9510565162951535312, 1.000000000000000000, 0.9510565162951535312, 1.000000000000000000, 0.9755282581475768211, 0.9755282581475768211 ) ) 
 REPRESENTATION_ITEM ( '' )  );
#11185=CARTESIAN_POINT ( 'NONE',  ( 27.16883889988624290, 2.175000002731186655, 19.73931689729373673 ) ) ;
#11186=FACE_OUTER_BOUND ( 'NONE', #28125, .T. ) ;
#11187=CARTESIAN_POINT ( 'NONE',  ( -13.91746824999999532, 75.47500000273116427, 4.522059556121122093 ) ) ;
#11188=CARTESIAN_POINT ( 'NONE',  ( 33.58253175000000113, 72.47500000273119269, -10.91162601494193574 ) ) ;
#11189=DIRECTION ( 'NONE',  ( -0.000000000000000000, -1.000000000000000000, -0.000000000000000000 ) ) ;
#11191=ORIENTED_EDGE ( 'NONE', *, *, #9439, .T. ) ;
#11202=LINE ( 'NONE', #19100, #32491 ) ;
#11203=CARTESIAN_POINT ( 'NONE',  ( 27.16883889988623935, 40.32500000273120122, -19.73931689729374384 ) ) ;
#11206=CARTESIAN_POINT ( 'NONE',  ( -24.50000000000000000, 4.649999994537640902, -7.960532557706207157 ) ) ;
#11207=ORIENTED_EDGE ( 'NONE', *, *, #5341, .F. ) ;
#11209=DIRECTION ( 'NONE',  ( 0.000000000000000000, 0.000000000000000000, 1.000000000000000000 ) ) ;
#11211=CARTESIAN_POINT ( 'NONE',  ( 27.16883889988623935, 70.57500000273120122, -19.73931689729374384 ) ) ;
#11215=ORIENTED_EDGE ( 'NONE', *, *, #8603, .T. ) ;
#11216=CARTESIAN_POINT ( 'NONE',  ( 5.147494310547434893, 65.05125428700922896, 32.49999999999999289 ) ) ;
#11217=CARTESIAN_POINT ( 'NONE',  ( -33.58253175000000113, 55.02500000273118985, -10.91162601494193218 ) ) ;
#11219=CARTESIAN_POINT ( 'NONE',  ( -32.50000000000000000, 16.40000000546239178, -10.55989012756945478 ) ) ;
#11220=CARTESIAN_POINT ( 'NONE',  ( 0.000000000000000000, 0.000000000000000000, 0.000000000000000000 ) ) ;
#11221=CARTESIAN_POINT ( 'NONE',  ( 18.94512977948576093, 11.32499999726882578, -13.76444248337722875 ) ) ;
#11223=CARTESIAN_POINT ( 'NONE',  ( 33.58253175000000823, 22.27500000273116854, 10.91162601494192863 ) ) ;
#11225=CARTESIAN_POINT ( 'NONE',  ( -4.300734207923755825, 79.27500000273118985, 13.23629886949340673 ) ) ;
#11230=CARTESIAN_POINT ( 'NONE',  ( 8.601468415847516980, 76.17500000273116711, -11.83890561707634781 ) ) ;
#11232=CARTESIAN_POINT ( 'NONE',  ( 10.37757302488624056, 24.52500000273119696, -31.93888565452638417 ) ) ;
#11236=CARTESIAN_POINT ( 'NONE',  ( -33.58253175000000113, 7.375000002731169069, 0.000000000000000000 ) ) ;
#11238=CARTESIAN_POINT ( 'NONE',  ( -2.162160676586882350E-15, 72.62500000273118417, -35.31076352940722529 ) ) ;
#11240=CARTESIAN_POINT ( 'NONE',  ( -1.778240108872766143E-15, 12.00000000546238077, -32.49999999999999289 ) ) ;
#11241=CARTESIAN_POINT ( 'NONE',  ( 4.300734207923757602, 76.77500000273118985, -13.23629886949340673 ) ) ;
#11243=CARTESIAN_POINT ( 'NONE',  ( 0.000000000000000000, 80.00000000000001421, 0.000000000000000000 ) ) ;
#11244=CARTESIAN_POINT ( 'NONE',  ( 33.58253175000000113, 60.12500000273119127, -4.112674001490185761E-15 ) ) ;
#11249=CARTESIAN_POINT ( 'NONE',  ( -26.29305231718578995, 16.19999999999999218, 19.10302069950538595 ) ) ;
#11250=CARTESIAN_POINT ( 'NONE',  ( -23.41746824999999887, 9.624999997268817609, -2.867812753649727150E-15 ) ) ;
#11254=CARTESIAN_POINT ( 'NONE',  ( -20.08610463437156923, 68.80000000546236549, 27.64615127144130113 ) ) ;
#11260=CARTESIAN_POINT ( 'NONE',  ( -33.58253175000000113, 75.12500000273119838, 0.000000000000000000 ) ) ;
#11262=CARTESIAN_POINT ( 'NONE',  ( 15.14183272437242245, 6.300000000000004263, -20.84094480462497856 ) ) ;
#11263=CARTESIAN_POINT ( 'NONE',  ( -27.16883889988624290, 7.175000002731191096, -19.73931689729374028 ) ) ;
#11264=CARTESIAN_POINT ( 'NONE',  ( 10.37757302488624056, 18.52500000273118985, -31.93888565452638417 ) ) ;
#11265=CARTESIAN_POINT ( 'NONE',  ( 8.601468415847516980, 76.17500000273118133, -11.83890561707634603 ) ) ;
#11268=CARTESIAN_POINT ( 'NONE',  ( -9.270509831248425314, 77.70000000000003126, -12.75976212528059861 ) ) ;
#11270=EDGE_CURVE ( 'NONE', #3811, #8544, #7433, .T. ) ;
#11271=AXIS2_PLACEMENT_3D ( 'NONE', #6979, #20377, #7319 ) ;
#11272=CARTESIAN_POINT ( 'NONE',  ( 10.04305231718578817, 71.40000000000001990, -30.90933677959249337 ) ) ;
#11274=CARTESIAN_POINT ( 'NONE',  ( 20.75514604977249178, 45.82500000273118701, 28.56700777964553950 ) ) ;
#11277=CARTESIAN_POINT ( 'NONE',  ( 20.75514604977249178, 32.07500000273117990, 28.56700777964553950 ) ) ;
#11281=CARTESIAN_POINT ( 'NONE',  ( 32.50000000000000711, 30.89999999999998437, 10.55989012756945122 ) ) ;
#11284=CARTESIAN_POINT ( 'NONE',  ( 23.41746824999999887, 4.524999997268823293, 7.608796670333735079 ) ) ;
#11287=FACE_OUTER_BOUND ( 'NONE', #17665, .T. ) ;
#11288=CARTESIAN_POINT ( 'NONE',  ( 10.37757302488624767, 17.72500000273119625, 31.93888565452638417 ) ) ;
#11289=CARTESIAN_POINT ( 'NONE',  ( -4.523095164977116484E-15, 8.624999997268810503, 24.62258325217400312 ) ) ;
#11297=CARTESIAN_POINT ( 'NONE',  ( 23.41746824999999887, 4.624999997268814056, 0.000000000000000000 ) ) ;
#11298=CARTESIAN_POINT ( 'NONE',  ( 10.37757302488624056, 30.77500000273120051, -31.93888565452638417 ) ) ;
#11299=CARTESIAN_POINT ( 'NONE',  ( -20.08610463437156923, 30.80000000546237615, 27.64615127144130113 ) ) ;
#11300=VECTOR ( 'NONE', #5709, 1000.000000000000000 ) ;
#11301=CARTESIAN_POINT ( 'NONE',  ( -32.50000000000000000, 76.10000000000002274, 10.55989012756946366 ) ) ;
#11302=CARTESIAN_POINT ( 'NONE',  ( -2.165007332552593587E-13, 52.50000000000000711, 32.50000000000000000 ) ) ;
#11304=CARTESIAN_POINT ( 'NONE',  ( 10.37757302488624767, 45.97500000273119269, 31.93888565452638417 ) ) ;
#11306=CARTESIAN_POINT ( 'NONE',  ( -2.092463501923844636E-15, 19.49999999999998934, -34.17252228774368916 ) ) ;
#11308=CARTESIAN_POINT ( 'NONE',  ( 33.58253175000000113, 62.12500000273119127, -4.112674001490185761E-15 ) ) ;
#11309=CARTESIAN_POINT ( 'NONE',  ( -20.75514604977248823, 53.07500000273118701, -28.56700777964554305 ) ) ;
#11311=CARTESIAN_POINT ( 'NONE',  ( 33.58253175000000823, 8.025000002731188076, 10.91162601494192863 ) ) ;
#11314=CARTESIAN_POINT ( 'NONE',  ( 20.08610463437157279, 25.80000000546238681, -27.64615127144129758 ) ) ;
#11317=CARTESIAN_POINT ( 'NONE',  ( 3.000384657911015469E-15, 0.000000000000000000, -24.50000000000000000 ) ) ;
#11318=CARTESIAN_POINT ( 'NONE',  ( -26.29305231718578995, 58.70000000546238539, 19.10302069950538595 ) ) ;
#11320=CARTESIAN_POINT ( 'NONE',  ( 19.82091636218621389, 14.19999999999999041, -14.40073868116559197 ) ) ;
#11329=LINE ( 'NONE', #14579, #5880 ) ;
#11335=CARTESIAN_POINT ( 'NONE',  ( -1.778240108872766143E-15, 64.00000000546238255, -32.49999999999999289 ) ) ;
#11336=CARTESIAN_POINT ( 'NONE',  ( -27.16883889988624290, 45.17500000273119554, -19.73931689729374028 ) ) ;
#11337=CARTESIAN_POINT ( 'NONE',  ( -2.092463501923844636E-15, 52.00000000546236834, -34.17252228774368916 ) ) ;
#11339=CARTESIAN_POINT ( 'NONE',  ( -2.162160676586881955E-15, 34.62500000273119127, -35.31076352940723240 ) ) ;
#11340=CARTESIAN_POINT ( 'NONE',  ( -5.147494310547423346, 24.44874571845316069, 32.50000000000000000 ) ) ;
#11341=CARTESIAN_POINT ( 'NONE',  ( -10.37757302488623701, 61.77500000273117564, 31.93888565452638417 ) ) ;
#11342=PRESENTATION_STYLE_ASSIGNMENT (( #9096 ) ) ;
#11343=CARTESIAN_POINT ( 'NONE',  ( 20.08610463437157279, 39.30000000000001137, -27.64615127144129758 ) ) ;
#11345=CARTESIAN_POINT ( 'NONE',  ( -33.58253175000000113, 3.475000002731185589, 10.91162601494193929 ) ) ;
#11346=CARTESIAN_POINT ( 'NONE',  ( 24.50000000000000000, 1.749999994537621006, 0.000000000000000000 ) ) ;
#11348=CARTESIAN_POINT ( 'NONE',  ( 33.58253175000000113, 74.37500000273116996, -4.112674001490185761E-15 ) ) ;
#11349=CARTESIAN_POINT ( 'NONE',  ( 0.000000000000000000, 80.00000000000001421, -32.50000000000000000 ) ) ;
#11352=CARTESIAN_POINT ( 'NONE',  ( 24.50000000000000355, 3.849999994537637082, -7.960532557706203605 ) ) ;
#11361=EDGE_CURVE ( 'NONE', #14943, #12209, #13499, .T. ) ;
#11368=CARTESIAN_POINT ( 'NONE',  ( 20.08610463437157279, 13.80000000546235839, -27.64615127144129758 ) ) ;
#11371=CARTESIAN_POINT ( 'NONE',  ( -20.08610463437156923, 76.30000000000001137, 27.64615127144130113 ) ) ;
#11373=CARTESIAN_POINT ( 'NONE',  ( 10.37757302488624056, 66.77500000273117564, -31.93888565452638417 ) ) ;
#11374=VERTEX_POINT ( 'NONE', #10472 ) ;
#11378=( BOUNDED_CURVE ( )  B_SPLINE_CURVE ( 2, ( #16312, #10986, #24032, #11314, #16810, #14231, #24525, #32570, #24687, #3589, #29331, #8733, #19052 ),
 .UNSPECIFIED., .F., .T. ) 
 B_SPLINE_CURVE_WITH_KNOTS ( ( 3, 2, 2, 2, 2, 2, 3 ),
 ( 0.6730769230769231282, 0.6743589743589744057, 0.6769230769230769607, 0.6794871794871795156, 0.6820512820512820706, 0.6846153846153846256, 0.6858974358974359031 ),
 .UNSPECIFIED. ) 
 CURVE ( )  GEOMETRIC_REPRESENTATION_ITEM ( )  RATIONAL_B_SPLINE_CURVE ( ( 0.9755282581475768211, 0.9755282581475778203, 1.000000000000000000, 0.9510565162951535312, 1.000000000000000000, 0.9510565162951535312, 1.000000000000000000, 0.9510565162951535312, 1.000000000000000000, 0.9510565162951535312, 1.000000000000000000, 0.9755282581475768211, 0.9755282581475768211 ) ) 
 REPRESENTATION_ITEM ( '' )  );
#11379=CARTESIAN_POINT ( 'NONE',  ( 26.29305231718578995, 65.70000000546238539, -19.10302069950538240 ) ) ;
#11380=CARTESIAN_POINT ( 'NONE',  ( -2.162160676586881955E-15, 56.62500000273116996, -35.31076352940723240 ) ) ;
#11382=CARTESIAN_POINT ( 'NONE',  ( -32.50000000000000000, 12.40000000546237224, -10.55989012756945478 ) ) ;
#11383=CARTESIAN_POINT ( 'NONE',  ( 7.570916362186213000, 16.14999999453761603, -23.30088464923126423 ) ) ;
#11384=CARTESIAN_POINT ( 'NONE',  ( -7.236395654485763274, 16.52499999726880731, 22.27133577429736633 ) ) ;
#11385=CARTESIAN_POINT ( 'NONE',  ( -10.37757302488624411, 22.97500000273117138, -31.93888565452638417 ) ) ;
#11387=CARTESIAN_POINT ( 'NONE',  ( 13.91746825000000065, 79.77500000273118985, 4.522059556121114987 ) ) ;
#11391=CARTESIAN_POINT ( 'NONE',  ( 8.601468415847520532, 73.57500000273117280, 11.83890561707634781 ) ) ;
#11393=CARTESIAN_POINT ( 'NONE',  ( -10.37757302488624411, 26.72500000273120335, -31.93888565452638417 ) ) ;
#11397=CARTESIAN_POINT ( 'NONE',  ( 10.37757302488624056, 6.775000002731179194, -31.93888565452638417 ) ) ;
#11400=CARTESIAN_POINT ( 'NONE',  ( -1.778240108872766143E-15, 21.50000000000000000, -32.49999999999999289 ) ) ;
#11401=CARTESIAN_POINT ( 'NONE',  ( -13.91746824999999532, 79.47500000273119269, 4.522059556121122093 ) ) ;
#11404=CARTESIAN_POINT ( 'NONE',  ( 33.58253175000000113, 54.12500000273118417, -4.112674001490185761E-15 ) ) ;
#11407=ORIENTED_EDGE ( 'NONE', *, *, #27617, .F. ) ;
#11410=CARTESIAN_POINT ( 'NONE',  ( -14.47279130897152122, 3.924999997268813434, 19.92008829642072243 ) ) ;
#11416=VERTEX_POINT ( 'NONE', #21335 ) ;
#11418=CARTESIAN_POINT ( 'NONE',  ( -20.75514604977248112, 61.67500000273117422, 28.56700777964554661 ) ) ;
#11420=CARTESIAN_POINT ( 'NONE',  ( 20.75514604977249178, 75.82500000273118701, 28.56700777964553950 ) ) ;
#11422=CARTESIAN_POINT ( 'NONE',  ( -24.50000000000001066, 7.100000000000007638, 7.960532557706201828 ) ) ;
#11423=CARTESIAN_POINT ( 'NONE',  ( 20.75514604977248467, 10.67500000273119021, -28.56700777964554305 ) ) ;
#11424=CARTESIAN_POINT ( 'NONE',  ( -33.58253175000000113, 15.22500000273119447, 10.91162601494193929 ) ) ;
#11425=CARTESIAN_POINT ( 'NONE',  ( 11.25946833292375793, 72.07500000273120122, -8.180482586598735395 ) ) ;
#11427=CARTESIAN_POINT ( 'NONE',  ( -12.13525491562421088, 81.79999999999998295, -8.816778784387096835 ) ) ;
#11432=CARTESIAN_POINT ( 'NONE',  ( 20.75514604977248467, 44.42500000273120264, -28.56700777964554305 ) ) ;
#11435=CARTESIAN_POINT ( 'NONE',  ( 33.58253175000000113, 26.37500000273118417, -4.112674001490185761E-15 ) ) ;
#11442=CARTESIAN_POINT ( 'NONE',  ( -7.236395654485763274, 6.024999997268825958, 22.27133577429736633 ) ) ;
#11443=EDGE_CURVE ( 'NONE', #771, #1133, #20606, .T. ) ;
#11446=CARTESIAN_POINT ( 'NONE',  ( -10.04305231718579172, 59.59999999999998721, -30.90933677959248982 ) ) ;
#11447=CARTESIAN_POINT ( 'NONE',  ( -20.75514604977248823, 16.82500000273120122, -28.56700777964554305 ) ) ;
#11448=CARTESIAN_POINT ( 'NONE',  ( -14.47279130897151589, 5.824999997268811569, -19.92008829642072598 ) ) ;
#11450=EDGE_CURVE ( 'NONE', #10494, #21929, #23736, .T. ) ;
#11453=ADVANCED_FACE ( 'NONE', ( #200 ), #10686, .T. ) ;
#11459=CARTESIAN_POINT ( 'NONE',  ( 15.14183272437242245, 14.04999999453763593, -20.84094480462497856 ) ) ;
#11460=ADVANCED_FACE ( 'NONE', ( #16349 ), #31611, .T. ) ;
#11461=CARTESIAN_POINT ( 'NONE',  ( 7.236395654485755280, 8.224999997268806595, 22.27133577429736988 ) ) ;
#11462=CARTESIAN_POINT ( 'NONE',  ( 27.16883889988624290, 30.17500000273118488, 19.73931689729373673 ) ) ;
#11463=CARTESIAN_POINT ( 'NONE',  ( -10.04305231718579172, 28.10000000546236620, -30.90933677959248982 ) ) ;
#11464=CARTESIAN_POINT ( 'NONE',  ( 20.08610463437158344, 72.70000000000001705, 27.64615127144129403 ) ) ;
#11465=CARTESIAN_POINT ( 'NONE',  ( 20.08610463437157279, 33.80000000546236549, -27.64615127144129758 ) ) ;
#11466=CARTESIAN_POINT ( 'NONE',  ( 0.000000000000000000, 80.00000000000001421, 0.000000000000000000 ) ) ;
#11468=CARTESIAN_POINT ( 'NONE',  ( -2.162160676586881955E-15, 42.87500000273119127, -35.31076352940723240 ) ) ;
#11469=CARTESIAN_POINT ( 'NONE',  ( -14.47279130897151589, 9.824999997268802687, -19.92008829642072598 ) ) ;
#11470=CARTESIAN_POINT ( 'NONE',  ( -26.29305231718578995, 12.19999999999998863, 19.10302069950538595 ) ) ;
#11473=CARTESIAN_POINT ( 'NONE',  ( 10.37757302488624767, 63.72500000273117848, 31.93888565452638417 ) ) ;
#11474=CARTESIAN_POINT ( 'NONE',  ( 10.37757302488624056, 46.77500000273118985, -31.93888565452638417 ) ) ;
#11477=CARTESIAN_POINT ( 'NONE',  ( 6.486482029760649416E-15, 7.625000002731170845, 35.31076352940723240 ) ) ;
#11483=CARTESIAN_POINT ( 'NONE',  ( -20.08610463437157989, 58.20000000546238539, -27.64615127144129758 ) ) ;
#11496=CARTESIAN_POINT ( 'NONE',  ( -32.50000000000000000, 46.50000000546239676, 0.000000000000000000 ) ) ;
#11497=CARTESIAN_POINT ( 'NONE',  ( 6.486482029760649416E-15, 47.87500000273117706, 35.31076352940723240 ) ) ;
#11498=CARTESIAN_POINT ( 'NONE',  ( -32.50000000000000000, 52.60000000546235555, 10.55989012756946366 ) ) ;
#11500=CARTESIAN_POINT ( 'NONE',  ( 33.58253175000000823, 34.02500000273118275, 10.91162601494192863 ) ) ;
#11501=CARTESIAN_POINT ( 'NONE',  ( 26.29305231718578995, 77.70000000546239960, -19.10302069950538240 ) ) ;
#11502=CARTESIAN_POINT ( 'NONE',  ( -20.75514604977248112, 59.67500000273118133, 28.56700777964554661 ) ) ;
#11504=CARTESIAN_POINT ( 'NONE',  ( 20.08610463437157279, 43.30000000000000426, -27.64615127144129758 ) ) ;
#11506=CARTESIAN_POINT ( 'NONE',  ( -20.75514604977248823, 7.075000002731188786, -28.56700777964554305 ) ) ;
#11509=CARTESIAN_POINT ( 'NONE',  ( 20.75514604977249178, 72.07500000273120122, 28.56700777964553950 ) ) ;
#11510=CARTESIAN_POINT ( 'NONE',  ( -4.223320258572819786E-15, 19.24999999453763166, 24.50000000000000000 ) ) ;
#11512=ORIENTED_EDGE ( 'NONE', *, *, #841, .F. ) ;
#11513=CARTESIAN_POINT ( 'NONE',  ( -7.570916362186215665, 7.149999994537637349, 23.30088464923126423 ) ) ;
#11515=CARTESIAN_POINT ( 'NONE',  ( 5.779280353836490358E-15, 75.00000000546236834, 32.49999999999999289 ) ) ;
#11525=CYLINDRICAL_SURFACE ( 'NONE', #25281, 32.50000000000000000 ) ;
#11526=CARTESIAN_POINT ( 'NONE',  ( -3.880418787951142701, 17.44874571845315359, 24.49999999999999645 ) ) ;
#11527=ORIENTED_EDGE ( 'NONE', *, *, #20920, .F. ) ;
#11534=EDGE_CURVE ( 'NONE', #9120, #9319, #31776, .T. ) ;
#11537=CARTESIAN_POINT ( 'NONE',  ( -27.16883889988623935, 57.32500000273119412, 19.73931689729374739 ) ) ;
#11539=ADVANCED_FACE ( 'NONE', ( #11027 ), #8108, .F. ) ;
#11540=CARTESIAN_POINT ( 'NONE',  ( -32.50000000000000000, 12.60000000546236620, 10.55989012756946366 ) ) ;
#11541=CARTESIAN_POINT ( 'NONE',  ( 19.82091636218621034, 15.54999999453762705, 14.40073868116559730 ) ) ;
#11542=CARTESIAN_POINT ( 'NONE',  ( -4.523095164977117273E-15, 16.62499999726881583, 24.62258325217400312 ) ) ;
#11543=CARTESIAN_POINT ( 'NONE',  ( 32.50000000000000000, 59.09999999999999432, -10.55989012756945833 ) ) ;
#11544=CARTESIAN_POINT ( 'NONE',  ( -33.58253175000000113, 23.27500000273116854, -10.91162601494193218 ) ) ;
#11545=CARTESIAN_POINT ( 'NONE',  ( 20.08610463437158344, 5.200000005462368513, 27.64615127144129403 ) ) ;
#11547=CARTESIAN_POINT ( 'NONE',  ( 11.25946833292375793, 77.67500000273119554, 8.180482586598731842 ) ) ;
#11548=CYLINDRICAL_SURFACE ( 'NONE', #875, 24.50000000000000000 ) ;
#11549=CARTESIAN_POINT ( 'NONE',  ( 32.50000000000000711, 14.89999999999999503, 10.55989012756945122 ) ) ;
#11553=CARTESIAN_POINT ( 'NONE',  ( -8.601468415847515203, 73.17500000273119554, 11.83890561707634959 ) ) ;
#11555=CARTESIAN_POINT ( 'NONE',  ( -27.16883889988623935, 15.32500000273118168, 19.73931689729374739 ) ) ;
#11559=CARTESIAN_POINT ( 'NONE',  ( 20.75514604977249178, 6.075000002731190563, 28.56700777964553950 ) ) ;
#11563=CARTESIAN_POINT ( 'NONE',  ( 11.25946833292375793, 74.57500000273120122, -8.180482586598735395 ) ) ;
#11568=CARTESIAN_POINT ( 'NONE',  ( 20.75514604977248467, 54.42500000273117422, -28.56700777964554305 ) ) ;
#11570=EDGE_LOOP ( 'NONE', ( #10744, #5088, #21350, #21312 ) ) ;
#11572=( BOUNDED_CURVE ( )  B_SPLINE_CURVE ( 2, ( #9037, #5801, #8367, #32039, #24165, #29623, #24653, #6126, #16445, #11611, #11446, #8538, #11125 ),
 .UNSPECIFIED., .F., .T. ) 
 B_SPLINE_CURVE_WITH_KNOTS ( ( 3, 2, 2, 2, 2, 2, 3 ),
 ( 0.2500000000000000000, 0.2512820512820512775, 0.2538461538461538325, 0.2564102564102563875, 0.2589743589743589980, 0.2615384615384615530, 0.2628205128205128305 ),
 .UNSPECIFIED. ) 
 CURVE ( )  GEOMETRIC_REPRESENTATION_ITEM ( )  RATIONAL_B_SPLINE_CURVE ( ( 0.9755282581475768211, 0.9755282581475768211, 1.000000000000000000, 0.9510565162951535312, 1.000000000000000000, 0.9510565162951535312, 1.000000000000000000, 0.9510565162951535312, 1.000000000000000000, 0.9510565162951535312, 1.000000000000000000, 0.9755282581475768211, 0.9755282581475768211 ) ) 
 REPRESENTATION_ITEM ( '' )  );
#11573=CYLINDRICAL_SURFACE ( 'NONE', #25044, 32.50000000000000000 ) ;
#11574=CARTESIAN_POINT ( 'NONE',  ( -14.47279130897152122, 7.924999997268803220, 19.92008829642072243 ) ) ;
#11576=EDGE_LOOP ( 'NONE', ( #22905, #32811, #19966, #31299 ) ) ;
#11578=LINE ( 'NONE', #20166, #4465 ) ;
#11581=CARTESIAN_POINT ( 'NONE',  ( 10.37757302488624056, 60.77500000273117564, -31.93888565452638417 ) ) ;
#11582=CARTESIAN_POINT ( 'NONE',  ( -3.880418787951127602, 2.551254281546845082, -24.50000000000000000 ) ) ;
#11583=CARTESIAN_POINT ( 'NONE',  ( -27.16883889988624290, 74.92500000273119554, -19.73931689729374028 ) ) ;
#11585=CARTESIAN_POINT ( 'NONE',  ( -19.82091636218621389, 7.200000000000011724, 14.40073868116558842 ) ) ;
#11587=CARTESIAN_POINT ( 'NONE',  ( 33.58253175000000823, 4.275000002731189852, 10.91162601494192863 ) ) ;
#11589=CARTESIAN_POINT ( 'NONE',  ( 10.37757302488624767, 15.72500000273119269, 31.93888565452638417 ) ) ;
#11592=CARTESIAN_POINT ( 'NONE',  ( -15.00000000000000000, 78.00000000000001421, 0.000000000000000000 ) ) ;
#11595=CARTESIAN_POINT ( 'NONE',  ( -32.50000000000000000, 38.60000000546239107, 10.55989012756946366 ) ) ;
#11597=CARTESIAN_POINT ( 'NONE',  ( 10.37757302488624056, 34.52500000273117564, -31.93888565452638417 ) ) ;
#11600=CARTESIAN_POINT ( 'NONE',  ( -33.58253175000000113, 25.37500000273118417, 0.000000000000000000 ) ) ;
#11604=CARTESIAN_POINT ( 'NONE',  ( 0.000000000000000000, 80.00000000000001421, -32.50000000000000000 ) ) ;
#11607=CARTESIAN_POINT ( 'NONE',  ( -18.94512977948575738, 13.42499999726881654, -13.76444248337723231 ) ) ;
#11611=CARTESIAN_POINT ( 'NONE',  ( -20.08610463437157989, 59.70000000000000284, -27.64615127144129758 ) ) ;
#11612=CARTESIAN_POINT ( 'NONE',  ( 10.37757302488624767, 11.72500000273118914, 31.93888565452638417 ) ) ;
#11613=CARTESIAN_POINT ( 'NONE',  ( 14.47279130897151589, 2.824999997268819119, 19.92008829642072953 ) ) ;
#11618=ORIENTED_EDGE ( 'NONE', *, *, #23499, .F. ) ;
#11621=CARTESIAN_POINT ( 'NONE',  ( -24.50000000000001066, 18.84999999453762953, 7.960532557706201828 ) ) ;
#11622=CARTESIAN_POINT ( 'NONE',  ( 23.41746824999999887, 2.624999997268812280, 0.000000000000000000 ) ) ;
#11623=CARTESIAN_POINT ( 'NONE',  ( -33.58253175000000113, 21.27500000273117209, -10.91162601494193218 ) ) ;
#11624=CARTESIAN_POINT ( 'NONE',  ( 10.04305231718578817, 31.90000000546239178, -30.90933677959249337 ) ) ;
#11625=CARTESIAN_POINT ( 'NONE',  ( -32.50000000000000000, 74.10000000000002274, 10.55989012756946366 ) ) ;
#11626=CARTESIAN_POINT ( 'NONE',  ( 10.04305231718578817, 47.90000000546238113, -30.90933677959249337 ) ) ;
#11627=CARTESIAN_POINT ( 'NONE',  ( 20.08610463437158344, 37.20000000546237828, 27.64615127144129403 ) ) ;
#11629=CARTESIAN_POINT ( 'NONE',  ( -33.58253175000000113, 35.47500000273118559, 10.91162601494193929 ) ) ;
#11633=CARTESIAN_POINT ( 'NONE',  ( 1.507698388325705758E-15, 9.624999997268808727, -24.62258325217400312 ) ) ;
#11634=CARTESIAN_POINT ( 'NONE',  ( 26.29305231718579350, 12.79999999999997762, 19.10302069950537529 ) ) ;
#11637=CARTESIAN_POINT ( 'NONE',  ( -27.16883889988623935, 55.32500000273118701, 19.73931689729374739 ) ) ;
#11638=CARTESIAN_POINT ( 'NONE',  ( 20.75514604977248467, 50.67500000273117422, -28.56700777964554305 ) ) ;
#11641=CARTESIAN_POINT ( 'NONE',  ( 33.58253175000000113, 4.225000002731190030, -10.91162601494193751 ) ) ;
#11644=CARTESIAN_POINT ( 'NONE',  ( 24.50000000000000000, 4.099999999999986322, -7.960532557706203605 ) ) ;
#11649=CARTESIAN_POINT ( 'NONE',  ( 2.489536152421872915E-14, 74.00000000546238255, -32.49999999999999289 ) ) ;
#11652=SURFACE_STYLE_FILL_AREA ( #16984 ) ;
#11655=ORIENTED_EDGE ( 'NONE', *, *, #11053, .T. ) ;
#11656=AXIS2_PLACEMENT_3D ( 'NONE', #20336, #12950, #5052 ) ;
#11659=CARTESIAN_POINT ( 'NONE',  ( 0.000000000000000000, 70.00000000000000000, 0.000000000000000000 ) ) ;
#11665=CARTESIAN_POINT ( 'NONE',  ( -2.162160676586881955E-15, 48.87500000273117706, -35.31076352940723240 ) ) ;
#11666=CARTESIAN_POINT ( 'NONE',  ( 10.04305231718578817, 51.90000000546238113, -30.90933677959249337 ) ) ;
#11669=CARTESIAN_POINT ( 'NONE',  ( -27.16883889988623935, 31.32500000273119412, 19.73931689729374739 ) ) ;
#11671=CARTESIAN_POINT ( 'NONE',  ( -33.58253175000000113, 57.37500000273118417, 0.000000000000000000 ) ) ;
#11673=CARTESIAN_POINT ( 'NONE',  ( 26.29305231718579350, 34.79999999999999716, 19.10302069950537529 ) ) ;
#11675=CARTESIAN_POINT ( 'NONE',  ( 27.16883889988623935, 4.575000002731199444, -19.73931689729374384 ) ) ;
#11676=CARTESIAN_POINT ( 'NONE',  ( 32.50000000000000000, 13.00000000000001066, -3.980102097228898626E-15 ) ) ;
#11678=CARTESIAN_POINT ( 'NONE',  ( 33.58253175000000113, 64.37500000273119838, -4.112674001490185761E-15 ) ) ;
#11679=AXIS2_PLACEMENT_3D ( 'NONE', #9264, #4126, #27129 ) ;
#11681=CARTESIAN_POINT ( 'NONE',  ( 15.14183272437242245, 2.049999994537635484, -20.84094480462497856 ) ) ;
#11691=CARTESIAN_POINT ( 'NONE',  ( 1.093617666956751375E-13, 67.50000000000000000, -32.50000000000000711 ) ) ;
#11693=DIRECTION ( 'NONE',  ( -0.000000000000000000, 1.000000000000000000, -0.000000000000000000 ) ) ;
#11694=CARTESIAN_POINT ( 'NONE',  ( -15.14183272437242778, 17.30000000000000782, 20.84094480462497856 ) ) ;
#11702=EDGE_LOOP ( 'NONE', ( #17933, #32295, #4024, #12425 ) ) ;
#11703=VERTEX_POINT ( 'NONE', #31447 ) ;
#11704=CARTESIAN_POINT ( 'NONE',  ( -10.04305231718578462, 56.40000000000000568, 30.90933677959249337 ) ) ;
#11705=CARTESIAN_POINT ( 'NONE',  ( 10.37757302488624056, 48.52500000273118985, -31.93888565452638417 ) ) ;
#11707=CARTESIAN_POINT ( 'NONE',  ( -32.50000000000000000, 10.60000000546237331, 10.55989012756946366 ) ) ;
#11708=CARTESIAN_POINT ( 'NONE',  ( -4.223320258572819786E-15, 15.24999999453762278, 24.50000000000000000 ) ) ;
#11709=CARTESIAN_POINT ( 'NONE',  ( 23.41746824999999887, 13.22499999726881192, -7.608796670333727974 ) ) ;
#11710=CARTESIAN_POINT ( 'NONE',  ( -20.08610463437156923, 54.30000000000000426, 27.64615127144130113 ) ) ;
#11711=CARTESIAN_POINT ( 'NONE',  ( 20.75514604977249178, 24.07500000273120122, 28.56700777964553950 ) ) ;
#11714=CARTESIAN_POINT ( 'NONE',  ( -13.91746824999999887, 72.87500000273119838, 0.000000000000000000 ) ) ;
#11716=CARTESIAN_POINT ( 'NONE',  ( -1.778240108872766143E-15, 28.00000000546237544, -32.49999999999999289 ) ) ;
#11718=ORIENTED_EDGE ( 'NONE', *, *, #27471, .F. ) ;
#11720=CARTESIAN_POINT ( 'NONE',  ( 32.50000000000000000, 71.50000000546235412, -3.980102097228898626E-15 ) ) ;
#11726=CARTESIAN_POINT ( 'NONE',  ( 27.16883889988623935, 10.57500000273120477, -19.73931689729374384 ) ) ;
#11729=CARTESIAN_POINT ( 'NONE',  ( 5.147494310547434893, 3.051254287009221411, 32.49999999999999289 ) ) ;
#11730=EDGE_CURVE ( 'NONE', #33131, #25303, #7939, .T. ) ;
#11731=CARTESIAN_POINT ( 'NONE',  ( 2.688165632520823219E-15, 77.87500000273118417, 14.63369212191046209 ) ) ;
#11733=CARTESIAN_POINT ( 'NONE',  ( -19.82091636218621034, 2.549999994537616388, -14.40073868116559552 ) ) ;
#11734=CARTESIAN_POINT ( 'NONE',  ( -33.58253175000000113, 51.22500000273119269, 10.91162601494193929 ) ) ;
#11735=ADVANCED_FACE ( 'NONE', ( #24890 ), #28613, .F. ) ;
#11737=ORIENTED_EDGE ( 'NONE', *, *, #6084, .T. ) ;
#11739=CARTESIAN_POINT ( 'NONE',  ( 0.000000000000000000, 80.00000000000001421, 0.000000000000000000 ) ) ;
#11740=CARTESIAN_POINT ( 'NONE',  ( 23.41746825000000243, 14.52499999726880020, 7.608796670333735079 ) ) ;
#11744=CARTESIAN_POINT ( 'NONE',  ( 0.000000000000000000, 0.000000000000000000, 24.50000000000000000 ) ) ;
#11748=CARTESIAN_POINT ( 'NONE',  ( -33.58253175000000113, 61.27500000273118985, -10.91162601494193218 ) ) ;
#11750=CARTESIAN_POINT ( 'NONE',  ( -33.58253175000000113, 73.02500000273120406, -10.91162601494193218 ) ) ;
#11752=CARTESIAN_POINT ( 'NONE',  ( -7.570916362186210335, 4.599999999999992539, -23.30088464923126779 ) ) ;
#11754=CARTESIAN_POINT ( 'NONE',  ( -10.37757302488624411, 16.72500000273119269, -31.93888565452638417 ) ) ;
#11755=CARTESIAN_POINT ( 'NONE',  ( -13.91746824999999532, 74.97500000273116427, 4.522059556121122093 ) ) ;
#11757=CARTESIAN_POINT ( 'NONE',  ( -9.270509831248425314, 79.70000000000000284, -12.75976212528059861 ) ) ;
#11759=CARTESIAN_POINT ( 'NONE',  ( -7.570916362186215665, 9.149999994537639125, 23.30088464923126423 ) ) ;
#11761=CARTESIAN_POINT ( 'NONE',  ( 9.270509831248425314, 78.95000000546239960, 12.75976212528059683 ) ) ;
#11763=CARTESIAN_POINT ( 'NONE',  ( -27.16883889988623935, 37.32500000273120122, 19.73931689729374739 ) ) ;
#11766=CARTESIAN_POINT ( 'NONE',  ( -27.16883889988624290, 29.17500000273118133, -19.73931689729374028 ) ) ;
#11767=CARTESIAN_POINT ( 'NONE',  ( 0.000000000000000000, 80.00000000000001421, -32.50000000000000000 ) ) ;
#11769=CARTESIAN_POINT ( 'NONE',  ( -32.50000000000000000, 17.89999999999998437, -10.55989012756945300 ) ) ;
#11771=EDGE_CURVE ( 'NONE', #30131, #5051, #25203, .T. ) ;
#11772=CARTESIAN_POINT ( 'NONE',  ( 4.635254915624212657, 80.60000000000000853, 14.26584774442730286 ) ) ;
#11775=CARTESIAN_POINT ( 'NONE',  ( -14.47279130897151767, 11.32499999726881157, -19.92008829642072598 ) ) ;
#11780=CARTESIAN_POINT ( 'NONE',  ( 33.58253175000000823, 14.02500000273117209, 10.91162601494192685 ) ) ;
#11781=CARTESIAN_POINT ( 'NONE',  ( 1.507698388325705758E-15, 5.624999997268818497, -24.62258325217400312 ) ) ;
#11783=ORIENTED_EDGE ( 'NONE', *, *, #14919, .T. ) ;
#11789=VECTOR ( 'NONE', #24932, 1000.000000000000000 ) ;
#11791=CARTESIAN_POINT ( 'NONE',  ( 24.50000000000000355, 17.64999999453763380, 7.960532557706212486 ) ) ;
#11792=CARTESIAN_POINT ( 'NONE',  ( -7.236395654485763274, 6.024999997268825958, 22.27133577429736633 ) ) ;
#11793=CARTESIAN_POINT ( 'NONE',  ( 10.37757302488624056, 20.77500000273119340, -31.93888565452638417 ) ) ;
#11795=CARTESIAN_POINT ( 'NONE',  ( 32.50000000000000000, 25.50000000546237544, -3.980102097228898626E-15 ) ) ;
#11796=CARTESIAN_POINT ( 'NONE',  ( 26.29305231718578995, 75.19999999999998863, -19.10302069950538240 ) ) ;
#11800=CARTESIAN_POINT ( 'NONE',  ( 20.75514604977249178, 36.07500000273117990, 28.56700777964553950 ) ) ;
#11804=CARTESIAN_POINT ( 'NONE',  ( -7.236395654485763274, 10.52499999726880198, 22.27133577429736633 ) ) ;
#11805=CARTESIAN_POINT ( 'NONE',  ( -10.04305231718579172, 11.59999999999999964, -30.90933677959248982 ) ) ;
#11808=CARTESIAN_POINT ( 'NONE',  ( -33.58253175000000113, 59.12500000273118417, 0.000000000000000000 ) ) ;
#11811=CARTESIAN_POINT ( 'NONE',  ( 33.58253175000000113, 44.37500000273119838, -4.112674001490185761E-15 ) ) ;
#11813=CARTESIAN_POINT ( 'NONE',  ( 0.000000000000000000, 0.000000000000000000, 24.50000000000000000 ) ) ;
#11814=CARTESIAN_POINT ( 'NONE',  ( -1.778240108872766143E-15, 46.00000000546238255, -32.49999999999999289 ) ) ;
#11817=DIRECTION ( 'NONE',  ( -0.000000000000000000, -1.000000000000000000, -0.000000000000000000 ) ) ;
#11819=CARTESIAN_POINT ( 'NONE',  ( 0.000000000000000000, 80.00000000000001421, 0.000000000000000000 ) ) ;
#11823=DIRECTION ( 'NONE',  ( -0.000000000000000000, -1.000000000000000000, -0.000000000000000000 ) ) ;
#11824=CARTESIAN_POINT ( 'NONE',  ( -33.58253175000000113, 31.02500000273118630, -10.91162601494193041 ) ) ;
#11829=CARTESIAN_POINT ( 'NONE',  ( 4.445600272181915325E-13, 26.00000000546237189, -32.50000000000000000 ) ) ;
#11834=CARTESIAN_POINT ( 'NONE',  ( 5.147494310547434893, 20.55125428154684286, 32.49999999999999289 ) ) ;
#11835=CARTESIAN_POINT ( 'NONE',  ( 10.37757302488624767, 43.97500000273119269, 31.93888565452638417 ) ) ;
#11836=CARTESIAN_POINT ( 'NONE',  ( 26.29305231718578995, 47.70000000546237118, -19.10302069950538240 ) ) ;
#11838=CARTESIAN_POINT ( 'NONE',  ( -10.37757302488624411, 28.72500000273120335, -31.93888565452638417 ) ) ;
#11839=CARTESIAN_POINT ( 'NONE',  ( 0.000000000000000000, 80.00000000000001421, -32.50000000000000000 ) ) ;
#11840=CARTESIAN_POINT ( 'NONE',  ( 33.58253175000000113, 58.47500000273118559, -10.91162601494193751 ) ) ;
#11842=CARTESIAN_POINT ( 'NONE',  ( -32.50000000000000000, 36.00000000000000711, 0.000000000000000000 ) ) ;
#11844=CARTESIAN_POINT ( 'NONE',  ( -33.58253175000000113, 73.02500000273120406, -10.91162601494193218 ) ) ;
#11845=DIRECTION ( 'NONE',  ( -0.000000000000000000, -1.000000000000000000, -0.000000000000000000 ) ) ;
#11847=CARTESIAN_POINT ( 'NONE',  ( 6.486482029760648627E-15, 63.87500000273119127, 35.31076352940722529 ) ) ;
#11850=CARTESIAN_POINT ( 'NONE',  ( -15.14183272437242600, 3.049999994537633263, 20.84094480462497856 ) ) ;
#11858=VECTOR ( 'NONE', #25240, 1000.000000000000000 ) ;
#11863=CARTESIAN_POINT ( 'NONE',  ( -5.147494310547423346, 58.44874571845314648, 32.50000000000000000 ) ) ;
#11864=ADVANCED_FACE ( 'NONE', ( #23983 ), #6406, .T. ) ;
#11865=CARTESIAN_POINT ( 'NONE',  ( -24.50000000000000711, 4.849999994537633974, 7.960532557706201828 ) ) ;
#11866=ORIENTED_EDGE ( 'NONE', *, *, #14197, .T. ) ;
#11868=( BOUNDED_CURVE ( )  B_SPLINE_CURVE ( 2, ( #33141, #31092, #22514, #17551, #17208, #33495, #27667, #14630, #27841, #25088, #32965, #19950, #1738 ),
 .UNSPECIFIED., .F., .T. ) 
 B_SPLINE_CURVE_WITH_KNOTS ( ( 3, 2, 2, 2, 2, 2, 3 ),
 ( 0.2884615384615384914, 0.2897435897435897689, 0.2923076923076923239, 0.2948717948717948789, 0.2974358974358974339, 0.2999999999999999889, 0.3012820512820512664 ),
 .UNSPECIFIED. ) 
 CURVE ( )  GEOMETRIC_REPRESENTATION_ITEM ( )  RATIONAL_B_SPLINE_CURVE ( ( 0.9755282581475768211, 0.9755282581475772652, 1.000000000000000000, 0.9510565162951535312, 1.000000000000000000, 0.9510565162951535312, 1.000000000000000000, 0.9510565162951535312, 1.000000000000000000, 0.9510565162951535312, 1.000000000000000000, 0.9755282581475768211, 0.9755282581475768211 ) ) 
 REPRESENTATION_ITEM ( '' )  );
#11871=EDGE_LOOP ( 'NONE', ( #26472, #2089, #32504, #29306 ) ) ;
#11872=ADVANCED_FACE ( 'NONE', ( #10935 ), #11548, .F. ) ;
#11875=VERTEX_POINT ( 'NONE', #10429 ) ;
#11876=CARTESIAN_POINT ( 'NONE',  ( -19.82091636218621389, 12.94999999453763628, 14.40073868116558842 ) ) ;
#11877=CARTESIAN_POINT ( 'NONE',  ( -20.75514604977248823, 48.82500000273117280, -28.56700777964554305 ) ) ;
#11879=CARTESIAN_POINT ( 'NONE',  ( -26.29305231718579350, 14.30000000546238681, -19.10302069950537884 ) ) ;
#11880=EDGE_CURVE ( 'NONE', #31338, #7013, #21908, .T. ) ;
#11881=CARTESIAN_POINT ( 'NONE',  ( -32.50000000000000000, 8.100000000000006750, 10.55989012756946366 ) ) ;
#11883=CARTESIAN_POINT ( 'NONE',  ( 7.236395654485760609, 13.52499999726880553, -22.27133577429736633 ) ) ;
#11884=CARTESIAN_POINT ( 'NONE',  ( -26.29305231718578995, 56.20000000000000284, 19.10302069950538595 ) ) ;
#11885=DIRECTION ( 'NONE',  ( -0.000000000000000000, 1.000000000000000000, -0.000000000000000000 ) ) ;
#11886=CARTESIAN_POINT ( 'NONE',  ( 27.16883889988623935, 14.57500000273120833, -19.73931689729374384 ) ) ;
#11888=CARTESIAN_POINT ( 'NONE',  ( -11.25946833292375793, 72.67500000273119554, -8.180482586598733619 ) ) ;
#11890=CARTESIAN_POINT ( 'NONE',  ( 5.147494310547434893, 14.55125428154684997, 32.49999999999999289 ) ) ;
#11891=VECTOR ( 'NONE', #6387, 1000.000000000000000 ) ;
#11893=VERTEX_POINT ( 'NONE', #282 ) ;
#11900=CARTESIAN_POINT ( 'NONE',  ( 27.16883889988624290, 10.17500000273119376, 19.73931689729373673 ) ) ;
#11903=CARTESIAN_POINT ( 'NONE',  ( 11.25946833292375793, 76.17500000273119554, 8.180482586598731842 ) ) ;
#11905=CARTESIAN_POINT ( 'NONE',  ( -3.880418787951136039, 2.301254276084479411, -24.50000000000000000 ) ) ;
#11906=CARTESIAN_POINT ( 'NONE',  ( 20.75514604977248467, 50.42500000273118843, -28.56700777964554305 ) ) ;
#11908=EDGE_LOOP ( 'NONE', ( #3628, #17938, #17206, #33834 ) ) ;
#11911=CARTESIAN_POINT ( 'NONE',  ( 7.236395654485760609, 11.02499999726880375, -22.27133577429736633 ) ) ;
#11913=ORIENTED_EDGE ( 'NONE', *, *, #8508, .F. ) ;
#11916=CARTESIAN_POINT ( 'NONE',  ( 5.779280353836490358E-15, 76.49999999999998579, 32.49999999999999289 ) ) ;
#11919=CARTESIAN_POINT ( 'NONE',  ( -33.58253175000000113, 59.27500000273119696, -10.91162601494193218 ) ) ;
#11920=CARTESIAN_POINT ( 'NONE',  ( -1.778240108872766143E-15, 29.50000000000000711, -32.49999999999999289 ) ) ;
#11921=CARTESIAN_POINT ( 'NONE',  ( -20.75514604977248112, 67.42500000273118133, 28.56700777964554661 ) ) ;
#11923=ADVANCED_BREP_SHAPE_REPRESENTATION ( '', ( #32241, #1376 ), #16210 ) ;
#11924=CARTESIAN_POINT ( 'NONE',  ( -15.14183272437241889, 10.70000000000001172, -20.84094480462497856 ) ) ;
#11925=CARTESIAN_POINT ( 'NONE',  ( 6.486482029760649416E-15, 5.875000002731167292, 35.31076352940723240 ) ) ;
#11926=EDGE_CURVE ( 'NONE', #29752, #6637, #33318, .T. ) ;
#11927=CARTESIAN_POINT ( 'NONE',  ( 20.75514604977249178, 7.825000002731194115, 28.56700777964553950 ) ) ;
#11928=CARTESIAN_POINT ( 'NONE',  ( -8.601468415847515203, 71.17500000273116711, 11.83890561707634959 ) ) ;
#11930=CARTESIAN_POINT ( 'NONE',  ( 15.00000000000000000, 81.00000000000001421, -1.836970198721029589E-15 ) ) ;
#11932=CARTESIAN_POINT ( 'NONE',  ( 10.04305231718579705, 61.10000000546239818, 30.90933677959248982 ) ) ;
#11934=CARTESIAN_POINT ( 'NONE',  ( -12.13525491562420910, 78.45000000546237118, 8.816778784387098611 ) ) ;
#11936=CARTESIAN_POINT ( 'NONE',  ( -20.75514604977248823, 36.82500000273117990, -28.56700777964554305 ) ) ;
#11939=CARTESIAN_POINT ( 'NONE',  ( 20.75514604977248467, 26.67500000273118133, -28.56700777964554305 ) ) ;
#11940=CARTESIAN_POINT ( 'NONE',  ( 10.04305231718579705, 40.59999999999999432, 30.90933677959248982 ) ) ;
#11941=CARTESIAN_POINT ( 'NONE',  ( -33.58253175000000113, 79.37500000273118417, 0.000000000000000000 ) ) ;
#11942=CARTESIAN_POINT ( 'NONE',  ( 2.375766604868044141, 81.44874571845316780, -14.99999999999999822 ) ) ;
#11944=CARTESIAN_POINT ( 'NONE',  ( 23.41746824999999887, 8.724999997268806595, -7.608796670333727974 ) ) ;
#11948=CARTESIAN_POINT ( 'NONE',  ( 20.75514604977249178, 13.82500000273117813, 28.56700777964553950 ) ) ;
#11949=CARTESIAN_POINT ( 'NONE',  ( -4.523095164977116484E-15, 14.62499999726882649, 24.62258325217400312 ) ) ;
#11951=ORIENTED_EDGE ( 'NONE', *, *, #8784, .F. ) ;
#11958=CARTESIAN_POINT ( 'NONE',  ( -15.14183272437242600, 15.04999999453763238, 20.84094480462497856 ) ) ;
#11959=CARTESIAN_POINT ( 'NONE',  ( 14.47279130897151767, 6.924999997268805885, -19.92008829642072598 ) ) ;
#11960=CARTESIAN_POINT ( 'NONE',  ( -27.16883889988623935, 21.57500000273118701, 19.73931689729374739 ) ) ;
#11961=CARTESIAN_POINT ( 'NONE',  ( -32.50000000000000000, 22.60000000546236976, 10.55989012756946366 ) ) ;
#11962=CARTESIAN_POINT ( 'NONE',  ( 20.08610463437158344, 70.70000000000000284, 27.64615127144129403 ) ) ;
#11963=LINE ( 'NONE', #4073, #7206 ) ;
#11966=CARTESIAN_POINT ( 'NONE',  ( 33.58253175000000823, 34.27500000273116854, 10.91162601494192863 ) ) ;
#11969=( BOUNDED_CURVE ( )  B_SPLINE_CURVE ( 2, ( #18776, #392, #11046, #8624, #21513, #28887, #29545, #26322, #29051, #31961, #16368, #26822, #26658 ),
 .UNSPECIFIED., .F., .T. ) 
 B_SPLINE_CURVE_WITH_KNOTS ( ( 3, 2, 2, 2, 2, 2, 3 ),
 ( 0.3653846153846153633, 0.3666666666666666408, 0.3692307692307692513, 0.3717948717948718063, 0.3743589743589743613, 0.3769230769230769162, 0.3782051282051281937 ),
 .UNSPECIFIED. ) 
 CURVE ( )  GEOMETRIC_REPRESENTATION_ITEM ( )  RATIONAL_B_SPLINE_CURVE ( ( 0.9755282581475768211, 0.9755282581475768211, 1.000000000000000000, 0.9510565162951535312, 1.000000000000000000, 0.9510565162951535312, 1.000000000000000000, 0.9510565162951535312, 1.000000000000000000, 0.9510565162951535312, 1.000000000000000000, 0.9755282581475768211, 0.9755282581475768211 ) ) 
 REPRESENTATION_ITEM ( '' )  );
#11970=EDGE_CURVE ( 'NONE', #22014, #12120, #28720, .T. ) ;
#11971=CARTESIAN_POINT ( 'NONE',  ( 23.41746825000000243, 9.224999997268820806, -7.608796670333727974 ) ) ;
#11972=CARTESIAN_POINT ( 'NONE',  ( 10.04305231718579705, 16.60000000000000497, 30.90933677959248982 ) ) ;
#11975=( BOUNDED_CURVE ( )  B_SPLINE_CURVE ( 2, ( #2277, #30410, #17912, #30757, #28020, #7247, #25276, #19963, #14982, #20306, #6910, #15159, #10010 ),
 .UNSPECIFIED., .F., .T. ) 
 B_SPLINE_CURVE_WITH_KNOTS ( ( 3, 2, 2, 2, 2, 2, 3 ),
 ( 0.4551282051282051211, 0.4564102564102563986, 0.4589743589743589536, 0.4615384615384615641, 0.4641025641025641191, 0.4666666666666666741, 0.4679487179487179516 ),
 .UNSPECIFIED. ) 
 CURVE ( )  GEOMETRIC_REPRESENTATION_ITEM ( )  RATIONAL_B_SPLINE_CURVE ( ( 0.9755282581475768211, 0.9755282581475768211, 1.000000000000000000, 0.9510565162951535312, 1.000000000000000000, 0.9510565162951535312, 1.000000000000000000, 0.9510565162951535312, 1.000000000000000000, 0.9510565162951535312, 1.000000000000000000, 0.9755282581475768211, 0.9755282581475768211 ) ) 
 REPRESENTATION_ITEM ( '' )  );
#11976=CARTESIAN_POINT ( 'NONE',  ( -2.162160676586881955E-15, 58.62500000273118417, -35.31076352940723240 ) ) ;
#11977=CARTESIAN_POINT ( 'NONE',  ( -2.162160676586882350E-15, 46.87500000273118417, -35.31076352940722529 ) ) ;
#11980=CARTESIAN_POINT ( 'NONE',  ( -26.29305231718578995, 50.19999999999999574, 19.10302069950538595 ) ) ;
#11982=CARTESIAN_POINT ( 'NONE',  ( 19.82091636218621389, 4.200000000000009059, -14.40073868116559197 ) ) ;
#11985=CARTESIAN_POINT ( 'NONE',  ( 26.29305231718579350, 41.30000000546238681, 19.10302069950537529 ) ) ;
#11988=CARTESIAN_POINT ( 'NONE',  ( -26.29305231718579350, 60.30000000546237260, -19.10302069950537884 ) ) ;
#11989=CARTESIAN_POINT ( 'NONE',  ( 6.486482029760648627E-15, 35.62500000273118417, 35.31076352940722529 ) ) ;
#11990=CARTESIAN_POINT ( 'NONE',  ( -27.16883889988623935, 65.57500000273120122, 19.73931689729374739 ) ) ;
#11992=VERTEX_POINT ( 'NONE', #7246 ) ;
#11995=LINE ( 'NONE', #1178, #15741 ) ;
#11996=ORIENTED_EDGE ( 'NONE', *, *, #6694, .F. ) ;
#12001=CARTESIAN_POINT ( 'NONE',  ( -10.04305231718578462, 64.90000000546235981, 30.90933677959249337 ) ) ;
#12002=CARTESIAN_POINT ( 'NONE',  ( -10.37757302488624411, 38.97500000273118559, -31.93888565452638417 ) ) ;
#12003=CARTESIAN_POINT ( 'NONE',  ( 10.04305231718578817, 43.90000000546237402, -30.90933677959249337 ) ) ;
#12005=CARTESIAN_POINT ( 'NONE',  ( -10.37757302488624411, 26.72500000273120335, -31.93888565452638417 ) ) ;
#12006=CARTESIAN_POINT ( 'NONE',  ( -10.04305231718579172, 23.60000000000000853, -30.90933677959248982 ) ) ;
#12007=CARTESIAN_POINT ( 'NONE',  ( 20.75514604977249178, 58.07500000273117990, 28.56700777964553950 ) ) ;
#12008=EDGE_CURVE ( 'NONE', #6801, #29733, #14470, .T. ) ;
#12010=ADVANCED_FACE ( 'NONE', ( #12055 ), #19962, .F. ) ;
#12011=CARTESIAN_POINT ( 'NONE',  ( -32.50000000000000000, 32.10000000000000142, 10.55989012756946366 ) ) ;
#12013=CARTESIAN_POINT ( 'NONE',  ( -10.37757302488624411, 76.72500000273119269, -31.93888565452638417 ) ) ;
#12014=CARTESIAN_POINT ( 'NONE',  ( -32.50000000000000000, 70.40000000546237402, -10.55989012756945300 ) ) ;
#12016=CARTESIAN_POINT ( 'NONE',  ( -10.37757302488623701, 67.77500000273117564, 31.93888565452638417 ) ) ;
#12019=CARTESIAN_POINT ( 'NONE',  ( -24.50000000000001066, 4.849999994537633974, 7.960532557706201828 ) ) ;
#12021=CARTESIAN_POINT ( 'NONE',  ( 20.08610463437158344, 46.70000000000000284, 27.64615127144129403 ) ) ;
#12035=VERTEX_POINT ( 'NONE', #12228 ) ;
#12039=CARTESIAN_POINT ( 'NONE',  ( -20.08610463437157989, 60.20000000546237828, -27.64615127144129758 ) ) ;
#12040=ORIENTED_EDGE ( 'NONE', *, *, #11053, .F. ) ;
#12041=CARTESIAN_POINT ( 'NONE',  ( -20.08610463437156923, 56.29999999999999716, 27.64615127144130113 ) ) ;
#12042=CARTESIAN_POINT ( 'NONE',  ( 27.16883889988623935, 48.32500000273117990, -19.73931689729374384 ) ) ;
#12043=CARTESIAN_POINT ( 'NONE',  ( 7.236395654485760609, 17.02499999726880731, -22.27133577429736633 ) ) ;
#12044=FACE_OUTER_BOUND ( 'NONE', #1266, .T. ) ;
#12046=CARTESIAN_POINT ( 'NONE',  ( -32.50000000000000000, 10.50000000546236123, 0.000000000000000000 ) ) ;
#12048=CARTESIAN_POINT ( 'NONE',  ( -23.41746824999999887, 14.12499999726882294, -2.867812753649727150E-15 ) ) ;
#12049=CARTESIAN_POINT ( 'NONE',  ( 10.04305231718578817, 53.40000000000000568, -30.90933677959249337 ) ) ;
#12051=CARTESIAN_POINT ( 'NONE',  ( -10.37757302488624411, 18.97500000273119625, -31.93888565452638417 ) ) ;
#12052=CARTESIAN_POINT ( 'NONE',  ( 12.13525491562421088, 76.80000000000001137, 8.816778784387095058 ) ) ;
#12054=CARTESIAN_POINT ( 'NONE',  ( 13.91746825000000065, 77.77500000273117564, 4.522059556121114987 ) ) ;
#12055=FACE_OUTER_BOUND ( 'NONE', #6066, .T. ) ;
#12056=CARTESIAN_POINT ( 'NONE',  ( -32.50000000000000000, 21.99999999999999289, 0.000000000000000000 ) ) ;
#12058=VERTEX_POINT ( 'NONE', #24927 ) ;
#12065=CARTESIAN_POINT ( 'NONE',  ( -10.37757302488624411, 2.975000002731182036, -31.93888565452638417 ) ) ;
#12069=( BOUNDED_CURVE ( )  B_SPLINE_CURVE ( 2, ( #27054, #26728, #21755, #9026, #24482, #3716, #29614 ),
 .UNSPECIFIED., .F., .F. ) 
 B_SPLINE_CURVE_WITH_KNOTS ( ( 3, 2, 2, 3 ),
 ( 0.9722222222222222099, 0.9777777777777777457, 0.9888888888888889284, 1.000000000000000000 ),
 .UNSPECIFIED. ) 
 CURVE ( )  GEOMETRIC_REPRESENTATION_ITEM ( )  RATIONAL_B_SPLINE_CURVE ( ( 0.9755282581475768211, 0.9755282581475768211, 1.000000000000000000, 0.9510565162951535312, 1.000000000000000000, 0.9510565162951535312, 1.000000000000000000 ) ) 
 REPRESENTATION_ITEM ( '' )  );
#12071=CARTESIAN_POINT ( 'NONE',  ( 10.37757302488624056, 52.52500000273118985, -31.93888565452638417 ) ) ;
#12074=CARTESIAN_POINT ( 'NONE',  ( 10.04305231718578817, 21.90000000546238468, -30.90933677959249337 ) ) ;
#12075=ORIENTED_EDGE ( 'NONE', *, *, #28655, .F. ) ;
#12077=CARTESIAN_POINT ( 'NONE',  ( 10.04305231718578817, 17.39999999999999858, -30.90933677959249337 ) ) ;
#12078=CARTESIAN_POINT ( 'NONE',  ( 14.47279130897151767, 14.92499999726881299, -19.92008829642072598 ) ) ;
#12080=ORIENTED_EDGE ( 'NONE', *, *, #26284, .F. ) ;
#12082=CARTESIAN_POINT ( 'NONE',  ( 3.880418787951153803, 5.551254281546845526, 24.49999999999999645 ) ) ;
#12083=ORIENTED_EDGE ( 'NONE', *, *, #4225, .F. ) ;
#12085=CARTESIAN_POINT ( 'NONE',  ( -33.58253175000000113, 61.47500000273117848, 10.91162601494193929 ) ) ;
#12087=CARTESIAN_POINT ( 'NONE',  ( 27.16883889988624290, 67.92500000273119554, 19.73931689729373673 ) ) ;
#12089=CARTESIAN_POINT ( 'NONE',  ( -4.732186688966233175E-15, 15.50000000000000533, 25.76082449383753925 ) ) ;
#12090=CARTESIAN_POINT ( 'NONE',  ( -33.58253175000000113, 5.375000002731167292, 0.000000000000000000 ) ) ;
#12091=CARTESIAN_POINT ( 'NONE',  ( -20.75514604977248823, 8.825000002731190563, -28.56700777964554305 ) ) ;
#12092=CARTESIAN_POINT ( 'NONE',  ( -26.29305231718578995, 0.7000000054623867207, 19.10302069950538595 ) ) ;
#12094=CARTESIAN_POINT ( 'NONE',  ( -4.635254915624208216, 76.40000000000001990, 14.26584774442730463 ) ) ;
#12097=CARTESIAN_POINT ( 'NONE',  ( 5.147494310547426899, 61.94874572391551482, -32.50000000000000000 ) ) ;
#12101=CARTESIAN_POINT ( 'NONE',  ( -10.37757302488624411, 38.72500000273118559, -31.93888565452638417 ) ) ;
#12104=CARTESIAN_POINT ( 'NONE',  ( -33.58253175000000113, 31.27500000273117919, -10.91162601494193041 ) ) ;
#12105=CARTESIAN_POINT ( 'NONE',  ( 26.29305231718578995, 41.20000000000001705, -19.10302069950538240 ) ) ;
#12106=CARTESIAN_POINT ( 'NONE',  ( -26.29305231718579350, 8.300000005462383257, -19.10302069950537884 ) ) ;
#12107=CARTESIAN_POINT ( 'NONE',  ( 26.29305231718579350, 32.79999999999999716, 19.10302069950537529 ) ) ;
#12109=CARTESIAN_POINT ( 'NONE',  ( -4.523095164977117273E-15, 10.12499999726882116, 24.62258325217400312 ) ) ;
#12114=CARTESIAN_POINT ( 'NONE',  ( 27.16883889988624290, 11.92500000273116711, 19.73931689729373673 ) ) ;
#12115=CARTESIAN_POINT ( 'NONE',  ( 23.41746825000000243, 15.02499999726881086, 7.608796670333735079 ) ) ;
#12117=ORIENTED_EDGE ( 'NONE', *, *, #11270, .F. ) ;
#12120=VERTEX_POINT ( 'NONE', #27679 ) ;
#12125=CARTESIAN_POINT ( 'NONE',  ( 1.577395562988744260E-15, 14.24999999453762989, -25.76082449383753925 ) ) ;
#12126=CARTESIAN_POINT ( 'NONE',  ( -23.41746825000000598, 13.72499999726882258, 7.608796670333726198 ) ) ;
#12127=CARTESIAN_POINT ( 'NONE',  ( 27.16883889988623935, 24.57500000273119056, -19.73931689729374384 ) ) ;
#12128=CARTESIAN_POINT ( 'NONE',  ( -26.29305231718579350, 24.30000000546236905, -19.10302069950537884 ) ) ;
#12129=CARTESIAN_POINT ( 'NONE',  ( 20.08610463437157279, 69.29999999999996874, -27.64615127144129758 ) ) ;
#12130=CARTESIAN_POINT ( 'NONE',  ( 5.147494310547426899, 47.94874572391553613, -32.50000000000000000 ) ) ;
#12133=CARTESIAN_POINT ( 'NONE',  ( -10.37757302488624411, 36.97500000273118559, -31.93888565452638417 ) ) ;
#12134=CYLINDRICAL_SURFACE ( 'NONE', #18535, 32.50000000000000000 ) ;
#12137=CARTESIAN_POINT ( 'NONE',  ( 23.41746825000000243, 13.02499999726881619, 7.608796670333735079 ) ) ;
#12138=CARTESIAN_POINT ( 'NONE',  ( -20.08610463437157989, 17.69999999999999218, -27.64615127144129758 ) ) ;
#12141=CARTESIAN_POINT ( 'NONE',  ( 27.16883889988623935, 56.32500000273118701, -19.73931689729374384 ) ) ;
#12143=CARTESIAN_POINT ( 'NONE',  ( 27.16883889988624290, 46.17500000273119554, 19.73931689729373673 ) ) ;
#12144=CARTESIAN_POINT ( 'NONE',  ( 32.50000000000000000, 44.99999999999998579, -3.980102097228898626E-15 ) ) ;
#12149=CARTESIAN_POINT ( 'NONE',  ( -32.50000000000000000, 42.09999999999997300, 10.55989012756946366 ) ) ;
#12151=CARTESIAN_POINT ( 'NONE',  ( -5.147494310547478413, 62.94874572391552192, 32.49999999999998579 ) ) ;
#12153=DIRECTION ( 'NONE',  ( 0.000000000000000000, 0.000000000000000000, -1.000000000000000000 ) ) ;
#12157=CARTESIAN_POINT ( 'NONE',  ( 5.779280353836490358E-15, 12.49999999999999112, 32.49999999999999289 ) ) ;
#12158=CARTESIAN_POINT ( 'NONE',  ( -20.75514604977248823, 30.82500000273119412, -28.56700777964554305 ) ) ;
#12159=CARTESIAN_POINT ( 'NONE',  ( -20.75514604977248823, 65.07500000273118701, -28.56700777964554305 ) ) ;
#12162=ORIENTED_EDGE ( 'NONE', *, *, #22557, .T. ) ;
#12166=VERTEX_POINT ( 'NONE', #32645 ) ;
#12170=( BOUNDED_CURVE ( )  B_SPLINE_CURVE ( 2, ( #30631, #14355, #4219, #6461, #25502, #1290, #1982, #27905, #12457, #4387, #14861, #28578, #28916 ),
 .UNSPECIFIED., .F., .T. ) 
 B_SPLINE_CURVE_WITH_KNOTS ( ( 3, 2, 2, 2, 2, 2, 3 ),
 ( 0.6944444444444444198, 0.6999999999999999556, 0.7111111111111111382, 0.7222222222222222099, 0.7333333333333332815, 0.7444444444444444642, 0.7500000000000000000 ),
 .UNSPECIFIED. ) 
 CURVE ( )  GEOMETRIC_REPRESENTATION_ITEM ( )  RATIONAL_B_SPLINE_CURVE ( ( 0.9755282581475768211, 0.9755282581475768211, 1.000000000000000000, 0.9510565162951535312, 1.000000000000000000, 0.9510565162951535312, 1.000000000000000000, 0.9510565162951535312, 1.000000000000000000, 0.9510565162951535312, 1.000000000000000000, 0.9755282581475768211, 0.9755282581475768211 ) ) 
 REPRESENTATION_ITEM ( '' )  );
#12172=CARTESIAN_POINT ( 'NONE',  ( -32.50000000000000000, 46.09999999999999432, 10.55989012756946366 ) ) ;
#12173=CARTESIAN_POINT ( 'NONE',  ( -20.75514604977248112, 39.67500000273118133, 28.56700777964554661 ) ) ;
#12174=CARTESIAN_POINT ( 'NONE',  ( -2.092463501923844636E-15, 42.00000000546236834, -34.17252228774368916 ) ) ;
#12175=( BOUNDED_CURVE ( )  B_SPLINE_CURVE ( 2, ( #4046, #12625, #2150, #17783, #22409, #28070, #32857, #10056, #9878, #30460, #24979, #1801, #4726 ),
 .UNSPECIFIED., .F., .F. ) 
 B_SPLINE_CURVE_WITH_KNOTS ( ( 3, 2, 2, 2, 2, 2, 3 ),
 ( 0.8397435897435897578, 0.8410256410256410353, 0.8435897435897435903, 0.8461538461538461453, 0.8487179487179487003, 0.8512820512820512553, 0.8525641025641025328 ),
 .UNSPECIFIED. ) 
 CURVE ( )  GEOMETRIC_REPRESENTATION_ITEM ( )  RATIONAL_B_SPLINE_CURVE ( ( 0.9755282581475768211, 0.9755282581475768211, 1.000000000000000000, 0.9510565162951535312, 1.000000000000000000, 0.9510565162951535312, 1.000000000000000000, 0.9510565162951535312, 1.000000000000000000, 0.9510565162951535312, 1.000000000000000000, 0.9755282581475768211, 0.9755282581475768211 ) ) 
 REPRESENTATION_ITEM ( '' )  );
#12177=CARTESIAN_POINT ( 'NONE',  ( -27.16883889988623935, 29.32500000273119412, 19.73931689729374739 ) ) ;
#12179=CARTESIAN_POINT ( 'NONE',  ( -10.37757302488623701, 55.77500000273119696, 31.93888565452638417 ) ) ;
#12182=CARTESIAN_POINT ( 'NONE',  ( -20.08610463437156923, 36.29999999999997584, 27.64615127144130113 ) ) ;
#12184=CARTESIAN_POINT ( 'NONE',  ( 27.16883889988624290, 75.92500000273119554, 19.73931689729373673 ) ) ;
#12186=CARTESIAN_POINT ( 'NONE',  ( -26.29305231718579350, 37.79999999999999716, -19.10302069950537884 ) ) ;
#12187=CARTESIAN_POINT ( 'NONE',  ( 33.58253175000000113, 66.47500000273119269, -10.91162601494193574 ) ) ;
#12190=CARTESIAN_POINT ( 'NONE',  ( -10.37757302488623701, 17.52500000273118985, 31.93888565452638417 ) ) ;
#12191=CARTESIAN_POINT ( 'NONE',  ( -19.82091636218621389, 12.94999999453763628, 14.40073868116558842 ) ) ;
#12193=CARTESIAN_POINT ( 'NONE',  ( 7.570916362186213000, 8.149999994537637349, -23.30088464923126423 ) ) ;
#12201=EDGE_CURVE ( 'NONE', #564, #1581, #24121, .T. ) ;
#12205=CARTESIAN_POINT ( 'NONE',  ( 10.04305231718578817, 77.90000000546237402, -30.90933677959249337 ) ) ;
#12209=VERTEX_POINT ( 'NONE', #10516 ) ;
#12210=CARTESIAN_POINT ( 'NONE',  ( 10.37757302488624767, 71.97500000273119269, 31.93888565452638417 ) ) ;
#12214=CARTESIAN_POINT ( 'NONE',  ( -10.04305231718579172, 66.10000000546237686, -30.90933677959248982 ) ) ;
#12217=CARTESIAN_POINT ( 'NONE',  ( -10.37757302488623701, 45.52500000273118985, 31.93888565452638417 ) ) ;
#12218=CARTESIAN_POINT ( 'NONE',  ( -32.50000000000000000, 2.400000005462369135, -10.55989012756945478 ) ) ;
#12222=CARTESIAN_POINT ( 'NONE',  ( 32.50000000000000000, 50.99999999999999289, -3.980102097228898626E-15 ) ) ;
#12224=CARTESIAN_POINT ( 'NONE',  ( 33.58253175000000113, 16.37500000273117706, -4.112674001490185761E-15 ) ) ;
#12227=CARTESIAN_POINT ( 'NONE',  ( 4.300734207923761154, 77.47500000273119269, 13.23629886949340495 ) ) ;
#12228=CARTESIAN_POINT ( 'NONE',  ( -13.91746824999999887, 70.87500000273119838, 0.000000000000000000 ) ) ;
#12238=CARTESIAN_POINT ( 'NONE',  ( 33.58253175000000823, 2.275000002731194293, 10.91162601494192685 ) ) ;
#12242=CARTESIAN_POINT ( 'NONE',  ( 8.601468415847516980, 72.67500000273118133, -11.83890561707634603 ) ) ;
#12244=CARTESIAN_POINT ( 'NONE',  ( 27.16883889988624290, 47.92500000273120264, 19.73931689729373673 ) ) ;
#12250=CARTESIAN_POINT ( 'NONE',  ( -33.58253175000000113, 79.25000000273118417, 0.000000000000000000 ) ) ;
#12251=CARTESIAN_POINT ( 'NONE',  ( 23.41746825000000243, 12.72499999726882436, -7.608796670333727974 ) ) ;
#12255=CARTESIAN_POINT ( 'NONE',  ( -10.04305231718578462, 34.90000000546239534, 30.90933677959249337 ) ) ;
#12256=VERTEX_POINT ( 'NONE', #28526 ) ;
#12257=CARTESIAN_POINT ( 'NONE',  ( -32.50000000000000000, 36.60000000546239818, 10.55989012756946366 ) ) ;
#12258=CARTESIAN_POINT ( 'NONE',  ( 20.75514604977248467, 70.42500000273119554, -28.56700777964554305 ) ) ;
#12260=CARTESIAN_POINT ( 'NONE',  ( 7.570916362186213000, 10.39999999999999325, -23.30088464923126423 ) ) ;
#12261=DIRECTION ( 'NONE',  ( -0.000000000000000000, 1.000000000000000000, -0.000000000000000000 ) ) ;
#12262=CARTESIAN_POINT ( 'NONE',  ( 33.58253175000000823, 10.02500000273118275, 10.91162601494192863 ) ) ;
#12263=CARTESIAN_POINT ( 'NONE',  ( -1.778240108872766143E-15, 29.50000000000000711, -32.49999999999999289 ) ) ;
#12265=CARTESIAN_POINT ( 'NONE',  ( 32.50000000000000711, 36.89999999999999858, 10.55989012756945122 ) ) ;
#12272=CARTESIAN_POINT ( 'NONE',  ( 15.00000000000000000, 75.35000000546239107, -4.873795443493596835 ) ) ;
#12274=( BOUNDED_CURVE ( )  B_SPLINE_CURVE ( 2, ( #29775, #16430, #22073, #32685, #1280, #9017, #8519, #24475, #27383, #21747, #11759, #9180, #19664 ),
 .UNSPECIFIED., .F., .T. ) 
 B_SPLINE_CURVE_WITH_KNOTS ( ( 3, 2, 2, 2, 2, 2, 3 ),
 ( 0.3611111111111111049, 0.3666666666666666408, 0.3777777777777777679, 0.3888888888888888951, 0.4000000000000000222, 0.4111111111111110938, 0.4166666666666666852 ),
 .UNSPECIFIED. ) 
 CURVE ( )  GEOMETRIC_REPRESENTATION_ITEM ( )  RATIONAL_B_SPLINE_CURVE ( ( 0.9755282581475768211, 0.9755282581475768211, 1.000000000000000000, 0.9510565162951535312, 1.000000000000000000, 0.9510565162951535312, 1.000000000000000000, 0.9510565162951535312, 1.000000000000000000, 0.9510565162951535312, 1.000000000000000000, 0.9755282581475765991, 0.9755282581475767101 ) ) 
 REPRESENTATION_ITEM ( '' )  );
#12275=CARTESIAN_POINT ( 'NONE',  ( -20.75514604977248823, 38.82500000273120122, -28.56700777964554305 ) ) ;
#12278=CARTESIAN_POINT ( 'NONE',  ( -20.75514604977248112, 23.67500000273118843, 28.56700777964554661 ) ) ;
#12279=CARTESIAN_POINT ( 'NONE',  ( -24.50000000000000000, 16.64999999453763735, -7.960532557706207157 ) ) ;
#12280=CARTESIAN_POINT ( 'NONE',  ( -1.778240108872766143E-15, 17.50000000000000000, -32.49999999999999289 ) ) ;
#12283=CARTESIAN_POINT ( 'NONE',  ( 7.236395654485755280, 12.22499999726881015, 22.27133577429736988 ) ) ;
#12289=CARTESIAN_POINT ( 'NONE',  ( 20.75514604977248467, 12.42500000273119376, -28.56700777964554305 ) ) ;
#12290=CARTESIAN_POINT ( 'NONE',  ( -23.41746825000000243, 10.02499999726882507, -7.608796670333730638 ) ) ;
#12293=VERTEX_POINT ( 'NONE', #10009 ) ;
#12300=CARTESIAN_POINT ( 'NONE',  ( -1.778240108872766143E-15, 18.00000000546237544, -32.49999999999999289 ) ) ;
#12301=CARTESIAN_POINT ( 'NONE',  ( 23.41746825000000243, 5.024999997268808194, 7.608796670333735079 ) ) ;
#12302=EDGE_CURVE ( 'NONE', #28216, #21432, #4165, .T. ) ;
#12303=CARTESIAN_POINT ( 'NONE',  ( -14.47279130897152122, 13.92499999726881654, 19.92008829642072243 ) ) ;
#12304=CARTESIAN_POINT ( 'NONE',  ( -33.58253175000000113, 19.47500000273117493, 10.91162601494193929 ) ) ;
#12305=CARTESIAN_POINT ( 'NONE',  ( -10.04305231718578462, 24.90000000546238468, 30.90933677959249337 ) ) ;
#12306=CARTESIAN_POINT ( 'NONE',  ( 26.29305231718579350, 64.79999999999999716, 19.10302069950537529 ) ) ;
#12310=CARTESIAN_POINT ( 'NONE',  ( 10.37757302488624767, 35.97500000273118559, 31.93888565452638417 ) ) ;
#12311=CARTESIAN_POINT ( 'NONE',  ( 5.147494310547426899, 43.94874572391553613, -32.50000000000000000 ) ) ;
#12314=CARTESIAN_POINT ( 'NONE',  ( -14.47279130897152122, 16.42499999726882365, 19.92008829642072243 ) ) ;
#12315=( BOUNDED_CURVE ( )  B_SPLINE_CURVE ( 2, ( #9867, #30969, #7468, #25140, #1616, #1788, #28400, #12265, #33192, #7972, #23599, #7802, #28903 ),
 .UNSPECIFIED., .F., .F. ) 
 B_SPLINE_CURVE_WITH_KNOTS ( ( 3, 2, 2, 2, 2, 2, 3 ),
 ( 0.5448717948717948234, 0.5461538461538461009, 0.5487179487179487669, 0.5512820512820513219, 0.5538461538461538769, 0.5564102564102564319, 0.5576923076923077094 ),
 .UNSPECIFIED. ) 
 CURVE ( )  GEOMETRIC_REPRESENTATION_ITEM ( )  RATIONAL_B_SPLINE_CURVE ( ( 0.9755282581475768211, 0.9755282581475768211, 1.000000000000000000, 0.9510565162951535312, 1.000000000000000000, 0.9510565162951535312, 1.000000000000000000, 0.9510565162951535312, 1.000000000000000000, 0.9510565162951535312, 1.000000000000000000, 0.9755282581475768211, 0.9755282581475768211 ) ) 
 REPRESENTATION_ITEM ( '' )  );
#12316=CARTESIAN_POINT ( 'NONE',  ( -20.08610463437157989, 9.700000000000013500, -27.64615127144129758 ) ) ;
#12317=STYLED_ITEM ( 'NONE', ( #6341 ), #32241 ) ;
#12318=CARTESIAN_POINT ( 'NONE',  ( 20.08610463437158344, 9.200000005462387165, 27.64615127144129403 ) ) ;
#12320=CARTESIAN_POINT ( 'NONE',  ( -10.37757302488624411, 54.72500000273117138, -31.93888565452638417 ) ) ;
#12322=CARTESIAN_POINT ( 'NONE',  ( 10.37757302488624056, 38.77500000273118275, -31.93888565452638417 ) ) ;
#12324=DIRECTION ( 'NONE',  ( -0.000000000000000000, -1.000000000000000000, -0.000000000000000000 ) ) ;
#12330=LINE ( 'NONE', #14401, #17155 ) ;
#12332=CARTESIAN_POINT ( 'NONE',  ( -32.50000000000000000, 78.40000000546234560, -10.55989012756945300 ) ) ;
#12335=CARTESIAN_POINT ( 'NONE',  ( 4.635254915624212657, 70.85000000546237686, 14.26584774442730286 ) ) ;
#12336=CARTESIAN_POINT ( 'NONE',  ( -10.37757302488624411, 34.72500000273118559, -31.93888565452638417 ) ) ;
#12338=VERTEX_POINT ( 'NONE', #25623 ) ;
#12341=MECHANICAL_DESIGN_GEOMETRIC_PRESENTATION_REPRESENTATION('',(#29870),#15674);
#12343=ORIENTED_EDGE ( 'NONE', *, *, #25091, .F. ) ;
#12349=CARTESIAN_POINT ( 'NONE',  ( 6.486482029760649416E-15, 39.87500000273119127, 35.31076352940723240 ) ) ;
#12350=CARTESIAN_POINT ( 'NONE',  ( 32.50000000000000711, 45.40000000546237402, 10.55989012756945122 ) ) ;
#12352=CARTESIAN_POINT ( 'NONE',  ( -27.16883889988623935, 27.32500000273119412, 19.73931689729374739 ) ) ;
#12354=CARTESIAN_POINT ( 'NONE',  ( 33.58253175000000823, 54.27500000273118275, 10.91162601494192863 ) ) ;
#12356=CARTESIAN_POINT ( 'NONE',  ( 10.04305231718578817, 31.39999999999998437, -30.90933677959249337 ) ) ;
#12359=CARTESIAN_POINT ( 'NONE',  ( 27.16883889988623935, 78.32500000273118701, -19.73931689729374384 ) ) ;
#12361=CARTESIAN_POINT ( 'NONE',  ( -26.29305231718578995, 20.70000000546237828, 19.10302069950538595 ) ) ;
#12362=CARTESIAN_POINT ( 'NONE',  ( -33.58253175000000113, 65.47500000273117848, 10.91162601494193929 ) ) ;
#12364=CARTESIAN_POINT ( 'NONE',  ( 0.000000000000000000, 80.00000000000001421, -32.50000000000000000 ) ) ;
#12365=CARTESIAN_POINT ( 'NONE',  ( -33.58253175000000113, 17.22500000273118559, 10.91162601494193929 ) ) ;
#12366=CARTESIAN_POINT ( 'NONE',  ( 24.50000000000000355, 11.64999999453762314, 7.960532557706212486 ) ) ;
#12368=CARTESIAN_POINT ( 'NONE',  ( 26.29305231718578995, 47.19999999999998863, -19.10302069950538240 ) ) ;
#12379=( BOUNDED_CURVE ( )  B_SPLINE_CURVE ( 2, ( #7986, #18473, #31325, #12802, #15208, #33737, #33558, #23274, #31496, #20359, #10058, #23094, #5074, #23612, #10234, #25839, #2842, #2680, #13139, #15559, #12626, #20715, #10398, #5417, #15896, #26184, #7300, #26352, #7483, #20538, #31156, #26012, #2504, #17963, #30982, #12972, #7648, #7816, #81, #28412, #33908, #4902, #15730, #2151, #10568, #28243, #15383, #33383, #21047, #17784, #22926, #30805, #9879, #4727, #18134, #23446, #25672, #20877, #18306, #5248, #28750, #18974, #26522, #18644, #16560, #11238, #421, #8653, #3348, #21714, #23952, #19138, #27013, #23785, #24119, #29575, #11077, #21543, #3015, #756, #6076, #32160, #21380, #31825, #10908, #13981, #18806, #29082, #252, #29419, #16066, #31991, #5921, #3510, #16398, #13487, #13818, #24285, #24443, #8487, #5754, #5586, #13311, #10737, #26851, #31659, #3185, #21214, #29251, #8155, #8317, #16235, #26689, #13654, #586, #17613, #20363, #7487, #7304, #15042, #25675, #30810, #20719, #17788, #33563, #31160, #2331, #7652, #2156, #26016, #7133, #23278, #2684, #4731, #25507, #28248, #20881, #28755, #20193, #28416, #10402, #28075, #18310, #12461, #10238, #23099, #12976, #15212, #12630, #10062, #13143, #20542, #1986, #30636, #18138, #22931, #12806, #28582, #5252, #5078, #33387, #4906, #15734, #30987, #15564, #17967, #9884, #2509, #26188, #15387, #9711, #25843, #23451, #33743, #33912, #31330, #7821, #33208, #4564, #13823, #24292, #10741, #31829, #31663, #5421, #16071, #19143, #24124, #2846, #23789, #11244, #21721, #13491, #23956, #32166, #18477, #10912, #13659, #21219, #23616, #8492, #3019, #29581, #8659, #28921, #31996, #3516, #3189, #18648, #21384, #85, #426, #11081, #6083, #16566, #26857, #7992, #27020, #8158, #13316, #8322, #29086, #26693, #18811, #29255, #5758, #10572, #16238, #21051, #18979, #31500, #5590, #16403, #256, #3353, #15901, #26527, #26356, #763, #590, #21550, #29424, #5926, #24776, #27525, #29749, #9157, #11568, #19640, #30252, #11404, #14488, #14155, #6255, #9497, #27695, #32494, #25118, #9317, #4185, #22541, #19979, #24945, #27190, #24612, #1593, #12071, #3846, #14321, #32990, #8823, #1254, #4013, #1086, #13987, #32826, #22048, #30083, #14658, #11734, #16899, #27870, #1428, #8994, #22215, #24449, #32662, #11906, #30425, #6924, #17235, #32331, #17407, #19474, #3682, #6589, #17066, #22378, #29924, #6426, #19804, #6755, #925, #27361, #21881, #19307, #16734, #4869, #30948, #15175, #23063, #12934, #12244, #25469, #7445, #2295, #23240, #10026, #25640, #17929, #20154, #31287, #18094, #20681, #28380, #22722, #2119, #17749, #12592, #20499, #33523, #15349, #25803, #1764, #33871, #12767, #28209, #33700, #20842, #5038, #9847, #10201, #14999, #7614, #23410, #1946, #12422, #22892, #31121, #28541, #15523, #10364, #25975, #2468, #30599, #4695, #7781, #18267, #33170, #4352, #9674, #14828, #25294, #7094, #17578, #28038, #4524, #33349, #20324, #30774, #7264, #13778, #23746, #16361, #8119, #3147, #15694, #28715, #31458, #26145, #13104, #5548, #5380, #29045, #24246, #13619, #18606, #386, #11203, #29384, #211, #23577, #717, #7951, #5720, #16029, #8448, #10698, #21179, #2804, #32579, #21674, #26816, #26652, #10531, #26484, #16198, #9078, #43, #18939, #2641, #10871, #5211, #31621, #24084, #2979, #18438, #31955, #21008, #13447, #28882, #15859, #23914, #3312, #21346, #552, #26315, #13271, #31787, #8278, #18770, #29214, #11038, #21506, #5884, #11989, #15087, #20068, #32746, #19724, #7181, #22632, #17494, #22458, #12336, #27442, #9588, #22977, #25034, #1343, #6513, #32908, #25555, #28123, #14408, #27956, #33436, #33085, #14574, #17320, #19560, #4438, #24862, #9757, #14914, #30170, #2035, #9407, #25380, #6674, #17156, #27614, #30512, #6841, #27783, #4269, #30008, #14743, #16985, #1859, #3934, #11824, #7011, #12158, #30342, #25205, #4611, #22301, #4100, #22806, #33263, #20242, #1682, #30683, #17662, #9239, #12510, #1514, #19890, #26236, #7353, #20763, #23327, #31207, #15612, #7698, #23497, #18184, #17838, #28970, #23145, #20925, #33791, #23665, #25886, #2381, #18015, #13363, #10284, #12676, #30860, #25721, #28627, #31374, #5466, #28293, #128, #4781, #26064, #15948, #12852, #7865, #5125, #33610, #13189, #2896, #2557, #20410, #13024, #18356, #7531, #33955, #28801, #15259, #9933, #10110, #2201, #20589, #31035, #10449, #28461, #4953, #5298, #26403, #15780, #15433, #2725, #31542, #8038, #10619, #21098, #18524, #23837, #24332, #3728, #5802, #16118, #21268, #13701, #6299, #8869, #29133, #8703, #14199, #13867, #29302, #32040, #302, #636, #21767, #19353, #19186, #10955, #16775, #24166, #29624, #21430, #472, #31871, #3397, #21595, #8540, #19024, #10790, #29465, #31711, #6127, #8203, #8368, #27064, #13538, #18693, #29795, #5635, #18854, #26898, #32210, #16611, #5969, #11126, #807, #26571, #16446, #16282, #11288, #3558, #3068, #14031, #26740, #24001, #27235, #24493, #966, #11447, #3233, #21923, #32373, #14530, #30297, #7137, #25334, #30128, #19517, #4568, #4396, #14870, #17277, #14363, #32866, #9542, #29965, #20197, #27913, #9038, #9714, #9197, #24820, #22417, #6798, #27738, #19682, #11780, #14702, #11948, #33038, #1812, #6631, #1638, #4057, #24654, #25160, #22260, #19845, #32702, #1127, #17453, #6472, #12289, #32538, #30640, #17618, #4228, #12114, #28079, #11612, #22762, #6968, #22586, #16944, #1474, #24991, #22094, #33215, #17110, #27402, #20023, #3891, #27569, #1298, #9363, #30469, #10242, #26192, #31163, #7655, #25679, #18314, #23621, #12633, #23103, #2159, #33567, #18482, #28421, #17793, #1990, #26022, #4735, #18142, #2512, #10577, #12980, #15216, #20884, #31333, #7825, #28585, #15390, #33746, #10065, #12809, #23281, #25510, #4910, #23454, #20545, #5082, #28760, #20722, #89, #15568, #5255, #15737, #15046, #25846, #30990, #2336, #21055, #12465, #7490, #33916, #17970, #2687, #13147, #10405, #31505, #7997, #9890, #28926, #22935, #33391, #20367, #30816, #7308, #28252, #6088, #5763, #8327, #16570, #768, #29586, #13827, #29259, #11085, #21885, #27025, #10916, #260, #24453, #18652, #16409, #16242, #19148, #21388, #31833, #13495, #8828, #18816, #8162, #26361, #26862 ),
 .UNSPECIFIED., .F., .F. ) 
 B_SPLINE_CURVE_WITH_KNOTS ( ( 3, 2, 2, 2, 2, 2, 2, 2, 2, 2, 2, 2, 2, 2, 2, 2, 2, 2, 2, 2, 2, 2, 2, 2, 2, 2, 2, 2, 2, 2, 2, 2, 2, 2, 2, 2, 2, 2, 2, 2, 2, 2, 2, 2, 2, 2, 2, 2, 2, 2, 2, 2, 2, 2, 2, 2, 2, 2, 2, 2, 2, 2, 2, 2, 2, 2, 2, 2, 2, 2, 2, 2, 2, 2, 2, 2, 2, 2, 2, 2, 2, 2, 2, 2, 2, 2, 2, 2, 2, 2, 2, 2, 2, 2, 2, 2, 2, 2, 2, 2, 2, 2, 2, 2, 2, 2, 2, 2, 2, 2, 2, 2, 2, 2, 2, 2, 2, 2, 2, 2, 2, 2, 2, 2, 2, 2, 2, 2, 2, 2, 2, 2, 2, 2, 2, 2, 2, 2, 2, 2, 2, 2, 2, 2, 2, 2, 2, 2, 2, 2, 2, 2, 2, 2, 2, 2, 2, 2, 2, 2, 2, 2, 2, 2, 2, 2, 2, 2, 2, 2, 2, 2, 2, 2, 2, 2, 2, 2, 2, 2, 2, 2, 2, 2, 2, 2, 2, 2, 2, 2, 2, 2, 2, 2, 2, 2, 2, 2, 2, 2, 2, 2, 2, 2, 2, 2, 2, 2, 2, 2, 2, 2, 2, 2, 2, 2, 2, 2, 2, 2, 2, 2, 2, 2, 2, 2, 2, 2, 2, 2, 2, 2, 2, 2, 2, 2, 2, 2, 2, 2, 2, 2, 2, 2, 2, 2, 2, 2, 2, 2, 2, 2, 2, 2, 2, 2, 2, 2, 2, 2, 2, 2, 2, 2, 2, 2, 2, 2, 2, 2, 2, 2, 2, 2, 2, 2, 2, 2, 2, 2, 2, 2, 2, 2, 2, 2, 2, 2, 2, 2, 2, 2, 2, 2, 2, 2, 2, 2, 2, 2, 2, 2, 2, 2, 2, 2, 2, 2, 2, 2, 2, 2, 2, 2, 2, 2, 2, 2, 2, 2, 2, 2, 2, 2, 2, 2, 2, 2, 2, 2, 2, 2, 2, 2, 2, 2, 2, 2, 2, 2, 2, 2, 2, 2, 2, 2, 2, 2, 2, 2, 2, 2, 2, 2, 2, 2, 2, 2, 2, 2, 2, 2, 2, 2, 2, 2, 2, 2, 2, 2, 2, 2, 2, 2, 2, 2, 2, 2, 2, 2, 2, 2, 2, 2, 2, 2, 2, 2, 2, 2, 3 ),
 ( 0.000000000000000000, 0.002564102564102564100, 0.005128205128205128201, 0.007692307692307692735, 0.01025641025641025640, 0.01282051282051282007, 0.01538461538461538547, 0.01794871794871794740, 0.02051282051282051280, 0.02307692307692307820, 0.02564102564102564014, 0.02820512820512820554, 0.03076923076923077094, 0.03333333333333333287, 0.03589743589743589480, 0.03846153846153846367, 0.04102564102564102561, 0.04358974358974358754, 0.04615384615384615641, 0.04871794871794871834, 0.05128205128205128027, 0.05384615384615384914, 0.05641025641025641107, 0.05897435897435897301, 0.06153846153846154188, 0.06410256410256409687, 0.06666666666666666574, 0.06923076923076923461, 0.07179487179487178961, 0.07435897435897435848, 0.07692307692307692735, 0.07948717948717948234, 0.08205128205128205121, 0.08461538461538462008, 0.08717948717948717507, 0.08974358974358974395, 0.09230769230769231282, 0.09487179487179486781, 0.09743589743589743668, 0.1000000000000000056, 0.1025641025641025605, 0.1051282051282051294, 0.1076923076923076983, 0.1102564102564102533, 0.1128205128205128221, 0.1153846153846153910, 0.1179487179487179460, 0.1205128205128205149, 0.1230769230769230838, 0.1256410256410256387, 0.1282051282051281937, 0.1307692307692307765, 0.1333333333333333315, 0.1358974358974358865, 0.1384615384615384692, 0.1410256410256410242, 0.1435897435897435792, 0.1461538461538461620, 0.1487179487179487170, 0.1512820512820512719, 0.1538461538461538547, 0.1564102564102564097, 0.1589743589743589647, 0.1615384615384615474, 0.1641025641025641024, 0.1666666666666666574, 0.1692307692307692402, 0.1717948717948717952, 0.1743589743589743501, 0.1769230769230769329, 0.1794871794871794879, 0.1820512820512820429, 0.1846153846153846256, 0.1871794871794871806, 0.1897435897435897356, 0.1923076923076923184, 0.1948717948717948734, 0.1974358974358974284, 0.2000000000000000111, 0.2025641025641025661, 0.2051282051282051211, 0.2076923076923077038, 0.2102564102564102588, 0.2128205128205128138, 0.2153846153846153966, 0.2179487179487179516, 0.2205128205128205066, 0.2230769230769230893, 0.2256410256410256443, 0.2282051282051281993, 0.2307692307692307820, 0.2333333333333333370, 0.2358974358974358920, 0.2384615384615384748, 0.2410256410256410298, 0.2435897435897435848, 0.2461538461538461675, 0.2487179487179487225, 0.2512820512820512775, 0.2538461538461538325, 0.2564102564102563875, 0.2589743589743589980, 0.2615384615384615530, 0.2641025641025641080, 0.2666666666666666630, 0.2692307692307692180, 0.2717948717948717730, 0.2743589743589743835, 0.2769230769230769384, 0.2794871794871794934, 0.2820512820512820484, 0.2846153846153846034, 0.2871794871794871584, 0.2897435897435897689, 0.2923076923076923239, 0.2948717948717948789, 0.2974358974358974339, 0.2999999999999999889, 0.3025641025641025439, 0.3051282051282051544, 0.3076923076923077094, 0.3102564102564102644, 0.3128205128205128194, 0.3153846153846153744, 0.3179487179487179294, 0.3205128205128205399, 0.3230769230769230949, 0.3256410256410256499, 0.3282051282051282048, 0.3307692307692307598, 0.3333333333333333148, 0.3358974358974358698, 0.3384615384615384803, 0.3410256410256410353, 0.3435897435897435903, 0.3461538461538461453, 0.3487179487179487003, 0.3512820512820512553, 0.3538461538461538658, 0.3564102564102564208, 0.3589743589743589758, 0.3615384615384615308, 0.3641025641025640858, 0.3666666666666666408, 0.3692307692307692513, 0.3717948717948718063, 0.3743589743589743613, 0.3769230769230769162, 0.3794871794871794712, 0.3820512820512820262, 0.3846153846153846367, 0.3871794871794871917, 0.3897435897435897467, 0.3923076923076923017, 0.3948717948717948567, 0.3974358974358974117, 0.4000000000000000222, 0.4025641025641025772, 0.4051282051282051322, 0.4076923076923076872, 0.4102564102564102422, 0.4128205128205127972, 0.4153846153846154077, 0.4179487179487179627, 0.4205128205128205177, 0.4230769230769230727, 0.4256410256410256276, 0.4282051282051281826, 0.4307692307692307931, 0.4333333333333333481, 0.4358974358974359031, 0.4384615384615384581, 0.4410256410256410131, 0.4435897435897435681, 0.4461538461538461786, 0.4487179487179487336, 0.4512820512820512886, 0.4538461538461538436, 0.4564102564102563986, 0.4589743589743589536, 0.4615384615384615641, 0.4641025641025641191, 0.4666666666666666741, 0.4692307692307692291, 0.4717948717948717841, 0.4743589743589743390, 0.4769230769230769496, 0.4794871794871795045, 0.4820512820512820595, 0.4846153846153846145, 0.4871794871794871695, 0.4897435897435897245, 0.4923076923076923350, 0.4948717948717948900, 0.4974358974358974450, 0.5000000000000000000, 0.5025641025641025550, 0.5051282051282051100, 0.5076923076923076650, 0.5102564102564102200, 0.5128205128205127750, 0.5153846153846153300, 0.5179487179487179960, 0.5205128205128205510, 0.5230769230769231060, 0.5256410256410256610, 0.5282051282051282159, 0.5307692307692307709, 0.5333333333333333259, 0.5358974358974358809, 0.5384615384615384359, 0.5410256410256409909, 0.5435897435897435459, 0.5461538461538461009, 0.5487179487179487669, 0.5512820512820513219, 0.5538461538461538769, 0.5564102564102564319, 0.5589743589743589869, 0.5615384615384615419, 0.5641025641025640969, 0.5666666666666666519, 0.5692307692307692069, 0.5717948717948717618, 0.5743589743589743168, 0.5769230769230768718, 0.5794871794871795379, 0.5820512820512820928, 0.5846153846153846478, 0.5871794871794872028, 0.5897435897435897578, 0.5923076923076923128, 0.5948717948717948678, 0.5974358974358974228, 0.5999999999999999778, 0.6025641025641025328, 0.6051282051282050878, 0.6076923076923076428, 0.6102564102564103088, 0.6128205128205128638, 0.6153846153846154188, 0.6179487179487179738, 0.6205128205128205288, 0.6230769230769230838, 0.6256410256410256387, 0.6282051282051281937, 0.6307692307692307487, 0.6333333333333333037, 0.6358974358974358587, 0.6384615384615384137, 0.6410256410256410797, 0.6435897435897436347, 0.6461538461538461897, 0.6487179487179487447, 0.6512820512820512997, 0.6538461538461538547, 0.6564102564102564097, 0.6589743589743589647, 0.6615384615384615197, 0.6641025641025640747, 0.6666666666666666297, 0.6692307692307691847, 0.6717948717948717396, 0.6743589743589744057, 0.6769230769230769607, 0.6794871794871795156, 0.6820512820512820706, 0.6846153846153846256, 0.6871794871794871806, 0.6897435897435897356, 0.6923076923076922906, 0.6948717948717948456, 0.6974358974358974006, 0.6999999999999999556, 0.7025641025641025106, 0.7051282051282051766, 0.7076923076923077316, 0.7102564102564102866, 0.7128205128205128416, 0.7153846153846153966, 0.7179487179487179516, 0.7205128205128205066, 0.7230769230769230616, 0.7256410256410256165, 0.7282051282051281715, 0.7307692307692307265, 0.7333333333333332815, 0.7358974358974359475, 0.7384615384615385025, 0.7410256410256410575, 0.7435897435897436125, 0.7461538461538461675, 0.7487179487179487225, 0.7512820512820512775, 0.7538461538461538325, 0.7564102564102563875, 0.7589743589743589425, 0.7615384615384614975, 0.7641025641025640525, 0.7666666666666667185, 0.7692307692307692735, 0.7717948717948718285, 0.7743589743589743835, 0.7769230769230769384, 0.7794871794871794934, 0.7820512820512820484, 0.7846153846153846034, 0.7871794871794871584, 0.7897435897435897134, 0.7923076923076922684, 0.7948717948717948234, 0.7974358974358974894, 0.8000000000000000444, 0.8025641025641025994, 0.8051282051282051544, 0.8076923076923077094, 0.8102564102564102644, 0.8128205128205128194, 0.8153846153846153744, 0.8179487179487179294, 0.8205128205128204844, 0.8230769230769230393, 0.8256410256410255943, 0.8282051282051282604, 0.8307692307692308153, 0.8333333333333333703, 0.8358974358974359253, 0.8384615384615384803, 0.8410256410256410353, 0.8435897435897435903, 0.8461538461538461453, 0.8487179487179487003, 0.8512820512820512553, 0.8538461538461538103, 0.8564102564102563653, 0.8589743589743589203, 0.8615384615384615863, 0.8641025641025641413, 0.8666666666666666963, 0.8692307692307692513, 0.8717948717948718063, 0.8743589743589743613, 0.8769230769230769162, 0.8794871794871794712, 0.8820512820512820262, 0.8846153846153845812, 0.8871794871794871362, 0.8897435897435896912, 0.8923076923076923572, 0.8948717948717949122, 0.8974358974358974672, 0.9000000000000000222, 0.9025641025641025772, 0.9051282051282051322, 0.9076923076923076872, 0.9102564102564102422, 0.9128205128205127972, 0.9153846153846153522, 0.9179487179487179072, 0.9205128205128204621, 0.9230769230769231282, 0.9256410256410256832, 0.9282051282051282382, 0.9307692307692307931, 0.9333333333333333481, 0.9358974358974359031, 0.9384615384615384581, 0.9410256410256410131, 0.9435897435897435681, 0.9461538461538461231, 0.9487179487179486781, 0.9512820512820512331, 0.9538461538461538991, 0.9564102564102564541, 0.9589743589743590091, 0.9615384615384615641, 0.9641025641025641191, 0.9666666666666666741, 0.9692307692307692291, 0.9717948717948717841, 0.9743589743589743390, 0.9769230769230768940, 0.9794871794871794490, 0.9820512820512820040, 0.9846153846153846700, 0.9871794871794872250, 0.9897435897435897800, 0.9923076923076923350, 0.9948717948717948900, 0.9974358974358974450, 1.000000000000000000 ),
 .UNSPECIFIED. ) 
 CURVE ( )  GEOMETRIC_REPRESENTATION_ITEM ( )  RATIONAL_B_SPLINE_CURVE ( ( 1.000000000000000000, 0.9510565162951535312, 1.000000000000000000, 0.9510565162951535312, 1.000000000000000000, 0.9510565162951535312, 1.000000000000000000, 0.9510565162951535312, 1.000000000000000000, 0.9510565162951535312, 1.000000000000000000, 0.9510565162951535312, 1.000000000000000000, 0.9510565162951535312, 1.000000000000000000, 0.9510565162951535312, 1.000000000000000000, 0.9510565162951535312, 1.000000000000000000, 0.9510565162951535312, 1.000000000000000000, 0.9510565162951535312, 1.000000000000000000, 0.9510565162951535312, 1.000000000000000000, 0.9510565162951535312, 1.000000000000000000, 0.9510565162951535312, 1.000000000000000000, 0.9510565162951535312, 1.000000000000000000, 0.9510565162951535312, 1.000000000000000000, 0.9510565162951535312, 1.000000000000000000, 0.9510565162951535312, 1.000000000000000000, 0.9510565162951535312, 1.000000000000000000, 0.9510565162951535312, 1.000000000000000000, 0.9510565162951535312, 1.000000000000000000, 0.9510565162951535312, 1.000000000000000000, 0.9510565162951535312, 1.000000000000000000, 0.9510565162951535312, 1.000000000000000000, 0.9510565162951535312, 1.000000000000000000, 0.9510565162951535312, 1.000000000000000000, 0.9510565162951535312, 1.000000000000000000, 0.9510565162951535312, 1.000000000000000000, 0.9510565162951535312, 1.000000000000000000, 0.9510565162951535312, 1.000000000000000000, 0.9510565162951535312, 1.000000000000000000, 0.9510565162951535312, 1.000000000000000000, 0.9510565162951535312, 1.000000000000000000, 0.9510565162951535312, 1.000000000000000000, 0.9510565162951535312, 1.000000000000000000, 0.9510565162951535312, 1.000000000000000000, 0.9510565162951535312, 1.000000000000000000, 0.9510565162951535312, 1.000000000000000000, 0.9510565162951535312, 1.000000000000000000, 0.9510565162951535312, 1.000000000000000000, 0.9510565162951535312, 1.000000000000000000, 0.9510565162951535312, 1.000000000000000000, 0.9510565162951535312, 1.000000000000000000, 0.9510565162951535312, 1.000000000000000000, 0.9510565162951535312, 1.000000000000000000, 0.9510565162951535312, 1.000000000000000000, 0.9510565162951535312, 1.000000000000000000, 0.9510565162951535312, 1.000000000000000000, 0.9510565162951535312, 1.000000000000000000, 0.9510565162951535312, 1.000000000000000000, 0.9510565162951535312, 1.000000000000000000, 0.9510565162951535312, 1.000000000000000000, 0.9510565162951535312, 1.000000000000000000, 0.9510565162951535312, 1.000000000000000000, 0.9510565162951535312, 1.000000000000000000, 0.9510565162951535312, 1.000000000000000000, 0.9510565162951535312, 1.000000000000000000, 0.9510565162951535312, 1.000000000000000000, 0.9510565162951535312, 1.000000000000000000, 0.9510565162951535312, 1.000000000000000000, 0.9510565162951535312, 1.000000000000000000, 0.9510565162951535312, 1.000000000000000000, 0.9510565162951535312, 1.000000000000000000, 0.9510565162951535312, 1.000000000000000000, 0.9510565162951535312, 1.000000000000000000, 0.9510565162951535312, 1.000000000000000000, 0.9510565162951535312, 1.000000000000000000, 0.9510565162951535312, 1.000000000000000000, 0.9510565162951535312, 1.000000000000000000, 0.9510565162951535312, 1.000000000000000000, 0.9510565162951535312, 1.000000000000000000, 0.9510565162951535312, 1.000000000000000000, 0.9510565162951535312, 1.000000000000000000, 0.9510565162951535312, 1.000000000000000000, 0.9510565162951535312, 1.000000000000000000, 0.9510565162951535312, 1.000000000000000000, 0.9510565162951535312, 1.000000000000000000, 0.9510565162951535312, 1.000000000000000000, 0.9510565162951535312, 1.000000000000000000, 0.9510565162951535312, 1.000000000000000000, 0.9510565162951535312, 1.000000000000000000, 0.9510565162951535312, 1.000000000000000000, 0.9510565162951535312, 1.000000000000000000, 0.9510565162951535312, 1.000000000000000000, 0.9510565162951535312, 1.000000000000000000, 0.9510565162951535312, 1.000000000000000000, 0.9510565162951535312, 1.000000000000000000, 0.9510565162951535312, 1.000000000000000000, 0.9510565162951535312, 1.000000000000000000, 0.9510565162951535312, 1.000000000000000000, 0.9510565162951535312, 1.000000000000000000, 0.9510565162951535312, 1.000000000000000000, 0.9510565162951535312, 1.000000000000000000, 0.9510565162951535312, 1.000000000000000000, 0.9510565162951535312, 1.000000000000000000, 0.9510565162951535312, 1.000000000000000000, 0.9510565162951535312, 1.000000000000000000, 0.9510565162951535312, 1.000000000000000000, 0.9510565162951535312, 1.000000000000000000, 0.9510565162951535312, 1.000000000000000000, 0.9510565162951535312, 1.000000000000000000, 0.9510565162951535312, 1.000000000000000000, 0.9510565162951535312, 1.000000000000000000, 0.9510565162951535312, 1.000000000000000000, 0.9510565162951535312, 1.000000000000000000, 0.9510565162951535312, 1.000000000000000000, 0.9510565162951535312, 1.000000000000000000, 0.9510565162951535312, 1.000000000000000000, 0.9510565162951535312, 1.000000000000000000, 0.9510565162951535312, 1.000000000000000000, 0.9510565162951535312, 1.000000000000000000, 0.9510565162951535312, 1.000000000000000000, 0.9510565162951535312, 1.000000000000000000, 0.9510565162951535312, 1.000000000000000000, 0.9510565162951535312, 1.000000000000000000, 0.9510565162951535312, 1.000000000000000000, 0.9510565162951535312, 1.000000000000000000, 0.9510565162951535312, 1.000000000000000000, 0.9510565162951535312, 1.000000000000000000, 0.9510565162951535312, 1.000000000000000000, 0.9510565162951535312, 1.000000000000000000, 0.9510565162951535312, 1.000000000000000000, 0.9510565162951535312, 1.000000000000000000, 0.9510565162951535312, 1.000000000000000000, 0.9510565162951535312, 1.000000000000000000, 0.9510565162951535312, 1.000000000000000000, 0.9510565162951535312, 1.000000000000000000, 0.9510565162951535312, 1.000000000000000000, 0.9510565162951535312, 1.000000000000000000, 0.9510565162951535312, 1.000000000000000000, 0.9510565162951535312, 1.000000000000000000, 0.9510565162951535312, 1.000000000000000000, 0.9510565162951535312, 1.000000000000000000, 0.9510565162951535312, 1.000000000000000000, 0.9510565162951535312, 1.000000000000000000, 0.9510565162951535312, 1.000000000000000000, 0.9510565162951535312, 1.000000000000000000, 0.9510565162951535312, 1.000000000000000000, 0.9510565162951535312, 1.000000000000000000, 0.9510565162951535312, 1.000000000000000000, 0.9510565162951535312, 1.000000000000000000, 0.9510565162951535312, 1.000000000000000000, 0.9510565162951535312, 1.000000000000000000, 0.9510565162951535312, 1.000000000000000000, 0.9510565162951535312, 1.000000000000000000, 0.9510565162951535312, 1.000000000000000000, 0.9510565162951535312, 1.000000000000000000, 0.9510565162951535312, 1.000000000000000000, 0.9510565162951535312, 1.000000000000000000, 0.9510565162951535312, 1.000000000000000000, 0.9510565162951535312, 1.000000000000000000, 0.9510565162951535312, 1.000000000000000000, 0.9510565162951535312, 1.000000000000000000, 0.9510565162951535312, 1.000000000000000000, 0.9510565162951535312, 1.000000000000000000, 0.9510565162951535312, 1.000000000000000000, 0.9510565162951535312, 1.000000000000000000, 0.9510565162951535312, 1.000000000000000000, 0.9510565162951535312, 1.000000000000000000, 0.9510565162951535312, 1.000000000000000000, 0.9510565162951535312, 1.000000000000000000, 0.9510565162951535312, 1.000000000000000000, 0.9510565162951535312, 1.000000000000000000, 0.9510565162951535312, 1.000000000000000000, 0.9510565162951535312, 1.000000000000000000, 0.9510565162951535312, 1.000000000000000000, 0.9510565162951535312, 1.000000000000000000, 0.9510565162951535312, 1.000000000000000000, 0.9510565162951535312, 1.000000000000000000, 0.9510565162951535312, 1.000000000000000000, 0.9510565162951535312, 1.000000000000000000, 0.9510565162951535312, 1.000000000000000000, 0.9510565162951535312, 1.000000000000000000, 0.9510565162951535312, 1.000000000000000000, 0.9510565162951535312, 1.000000000000000000, 0.9510565162951535312, 1.000000000000000000, 0.9510565162951535312, 1.000000000000000000, 0.9510565162951535312, 1.000000000000000000, 0.9510565162951535312, 1.000000000000000000, 0.9510565162951535312, 1.000000000000000000, 0.9510565162951535312, 1.000000000000000000, 0.9510565162951535312, 1.000000000000000000, 0.9510565162951535312, 1.000000000000000000, 0.9510565162951535312, 1.000000000000000000, 0.9510565162951535312, 1.000000000000000000, 0.9510565162951535312, 1.000000000000000000, 0.9510565162951535312, 1.000000000000000000, 0.9510565162951535312, 1.000000000000000000, 0.9510565162951535312, 1.000000000000000000, 0.9510565162951535312, 1.000000000000000000, 0.9510565162951535312, 1.000000000000000000, 0.9510565162951535312, 1.000000000000000000, 0.9510565162951535312, 1.000000000000000000, 0.9510565162951535312, 1.000000000000000000, 0.9510565162951535312, 1.000000000000000000, 0.9510565162951535312, 1.000000000000000000, 0.9510565162951535312, 1.000000000000000000, 0.9510565162951535312, 1.000000000000000000, 0.9510565162951535312, 1.000000000000000000, 0.9510565162951535312, 1.000000000000000000, 0.9510565162951535312, 1.000000000000000000, 0.9510565162951535312, 1.000000000000000000, 0.9510565162951535312, 1.000000000000000000, 0.9510565162951535312, 1.000000000000000000, 0.9510565162951535312, 1.000000000000000000, 0.9510565162951535312, 1.000000000000000000, 0.9510565162951535312, 1.000000000000000000, 0.9510565162951535312, 1.000000000000000000, 0.9510565162951535312, 1.000000000000000000, 0.9510565162951535312, 1.000000000000000000, 0.9510565162951535312, 1.000000000000000000, 0.9510565162951535312, 1.000000000000000000, 0.9510565162951535312, 1.000000000000000000, 0.9510565162951535312, 1.000000000000000000, 0.9510565162951535312, 1.000000000000000000, 0.9510565162951535312, 1.000000000000000000, 0.9510565162951535312, 1.000000000000000000, 0.9510565162951535312, 1.000000000000000000, 0.9510565162951535312, 1.000000000000000000, 0.9510565162951535312, 1.000000000000000000, 0.9510565162951535312, 1.000000000000000000, 0.9510565162951535312, 1.000000000000000000, 0.9510565162951535312, 1.000000000000000000, 0.9510565162951535312, 1.000000000000000000, 0.9510565162951535312, 1.000000000000000000, 0.9510565162951535312, 1.000000000000000000, 0.9510565162951535312, 1.000000000000000000, 0.9510565162951535312, 1.000000000000000000, 0.9510565162951535312, 1.000000000000000000, 0.9510565162951535312, 1.000000000000000000, 0.9510565162951535312, 1.000000000000000000, 0.9510565162951535312, 1.000000000000000000, 0.9510565162951535312, 1.000000000000000000, 0.9510565162951535312, 1.000000000000000000, 0.9510565162951535312, 1.000000000000000000, 0.9510565162951535312, 1.000000000000000000, 0.9510565162951535312, 1.000000000000000000, 0.9510565162951535312, 1.000000000000000000, 0.9510565162951535312, 1.000000000000000000, 0.9510565162951535312, 1.000000000000000000, 0.9510565162951535312, 1.000000000000000000, 0.9510565162951535312, 1.000000000000000000, 0.9510565162951535312, 1.000000000000000000, 0.9510565162951535312, 1.000000000000000000, 0.9510565162951535312, 1.000000000000000000, 0.9510565162951535312, 1.000000000000000000, 0.9510565162951535312, 1.000000000000000000, 0.9510565162951535312, 1.000000000000000000, 0.9510565162951535312, 1.000000000000000000, 0.9510565162951535312, 1.000000000000000000, 0.9510565162951535312, 1.000000000000000000, 0.9510565162951535312, 1.000000000000000000, 0.9510565162951535312, 1.000000000000000000, 0.9510565162951535312, 1.000000000000000000, 0.9510565162951535312, 1.000000000000000000, 0.9510565162951535312, 1.000000000000000000, 0.9510565162951535312, 1.000000000000000000, 0.9510565162951535312, 1.000000000000000000, 0.9510565162951535312, 1.000000000000000000, 0.9510565162951535312, 1.000000000000000000, 0.9510565162951535312, 1.000000000000000000, 0.9510565162951535312, 1.000000000000000000, 0.9510565162951535312, 1.000000000000000000, 0.9510565162951535312, 1.000000000000000000, 0.9510565162951535312, 1.000000000000000000, 0.9510565162951535312, 1.000000000000000000, 0.9510565162951535312, 1.000000000000000000, 0.9510565162951535312, 1.000000000000000000, 0.9510565162951535312, 1.000000000000000000, 0.9510565162951535312, 1.000000000000000000, 0.9510565162951535312, 1.000000000000000000, 0.9510565162951535312, 1.000000000000000000, 0.9510565162951535312, 1.000000000000000000, 0.9510565162951535312, 1.000000000000000000, 0.9510565162951535312, 1.000000000000000000, 0.9510565162951535312, 1.000000000000000000, 0.9510565162951535312, 1.000000000000000000, 0.9510565162951535312, 1.000000000000000000, 0.9510565162951535312, 1.000000000000000000, 0.9510565162951535312, 1.000000000000000000, 0.9510565162951535312, 1.000000000000000000, 0.9510565162951535312, 1.000000000000000000, 0.9510565162951535312, 1.000000000000000000, 0.9510565162951535312, 1.000000000000000000, 0.9510565162951535312, 1.000000000000000000, 0.9510565162951535312, 1.000000000000000000, 0.9510565162951535312, 1.000000000000000000, 0.9510565162951535312, 1.000000000000000000, 0.9510565162951535312, 1.000000000000000000, 0.9510565162951535312, 1.000000000000000000, 0.9510565162951535312, 1.000000000000000000, 0.9510565162951535312, 1.000000000000000000, 0.9510565162951535312, 1.000000000000000000, 0.9510565162951535312, 1.000000000000000000, 0.9510565162951535312, 1.000000000000000000, 0.9510565162951535312, 1.000000000000000000, 0.9510565162951535312, 1.000000000000000000, 0.9510565162951535312, 1.000000000000000000, 0.9510565162951535312, 1.000000000000000000, 0.9510565162951535312, 1.000000000000000000, 0.9510565162951535312, 1.000000000000000000, 0.9510565162951535312, 1.000000000000000000, 0.9510565162951535312, 1.000000000000000000, 0.9510565162951535312, 1.000000000000000000, 0.9510565162951535312, 1.000000000000000000, 0.9510565162951535312, 1.000000000000000000, 0.9510565162951535312, 1.000000000000000000, 0.9510565162951535312, 1.000000000000000000, 0.9510565162951535312, 1.000000000000000000, 0.9510565162951535312, 1.000000000000000000, 0.9510565162951535312, 1.000000000000000000, 0.9510565162951535312, 1.000000000000000000, 0.9510565162951535312, 1.000000000000000000, 0.9510565162951535312, 1.000000000000000000, 0.9510565162951535312, 1.000000000000000000, 0.9510565162951535312, 1.000000000000000000, 0.9510565162951535312, 1.000000000000000000, 0.9510565162951535312, 1.000000000000000000, 0.9510565162951535312, 1.000000000000000000, 0.9510565162951535312, 1.000000000000000000, 0.9510565162951535312, 1.000000000000000000, 0.9510565162951535312, 1.000000000000000000, 0.9510565162951535312, 1.000000000000000000, 0.9510565162951535312, 1.000000000000000000, 0.9510565162951535312, 1.000000000000000000, 0.9510565162951535312, 1.000000000000000000, 0.9510565162951535312, 1.000000000000000000, 0.9510565162951535312, 1.000000000000000000, 0.9510565162951535312, 1.000000000000000000, 0.9510565162951535312, 1.000000000000000000, 0.9510565162951535312, 1.000000000000000000, 0.9510565162951535312, 1.000000000000000000, 0.9510565162951535312, 1.000000000000000000, 0.9510565162951535312, 1.000000000000000000, 0.9510565162951535312, 1.000000000000000000, 0.9510565162951535312, 1.000000000000000000, 0.9510565162951535312, 1.000000000000000000, 0.9510565162951535312, 1.000000000000000000, 0.9510565162951535312, 1.000000000000000000, 0.9510565162951535312, 1.000000000000000000, 0.9510565162951535312, 1.000000000000000000, 0.9510565162951535312, 1.000000000000000000, 0.9510565162951535312, 1.000000000000000000, 0.9510565162951535312, 1.000000000000000000, 0.9510565162951535312, 1.000000000000000000, 0.9510565162951535312, 1.000000000000000000, 0.9510565162951535312, 1.000000000000000000, 0.9510565162951535312, 1.000000000000000000, 0.9510565162951535312, 1.000000000000000000, 0.9510565162951535312, 1.000000000000000000, 0.9510565162951535312, 1.000000000000000000, 0.9510565162951535312, 1.000000000000000000, 0.9510565162951535312, 1.000000000000000000, 0.9510565162951535312, 1.000000000000000000, 0.9510565162951535312, 1.000000000000000000, 0.9510565162951535312, 1.000000000000000000, 0.9510565162951535312, 1.000000000000000000, 0.9510565162951535312, 1.000000000000000000, 0.9510565162951535312, 1.000000000000000000, 0.9510565162951535312, 1.000000000000000000, 0.9510565162951535312, 1.000000000000000000, 0.9510565162951535312, 1.000000000000000000, 0.9510565162951535312, 1.000000000000000000, 0.9510565162951535312, 1.000000000000000000, 0.9510565162951535312, 1.000000000000000000, 0.9510565162951535312, 1.000000000000000000, 0.9510565162951535312, 1.000000000000000000, 0.9510565162951535312, 1.000000000000000000, 0.9510565162951535312, 1.000000000000000000, 0.9510565162951535312, 1.000000000000000000, 0.9510565162951535312, 1.000000000000000000, 0.9510565162951535312, 1.000000000000000000, 0.9510565162951535312, 1.000000000000000000, 0.9510565162951535312, 1.000000000000000000, 0.9510565162951535312, 1.000000000000000000, 0.9510565162951535312, 1.000000000000000000, 0.9510565162951535312, 1.000000000000000000, 0.9510565162951535312, 1.000000000000000000, 0.9510565162951535312, 1.000000000000000000, 0.9510565162951535312, 1.000000000000000000, 0.9510565162951535312, 1.000000000000000000, 0.9510565162951535312, 1.000000000000000000, 0.9510565162951535312, 1.000000000000000000, 0.9510565162951535312, 1.000000000000000000, 0.9510565162951535312, 1.000000000000000000, 0.9510565162951535312, 1.000000000000000000, 0.9510565162951535312, 1.000000000000000000, 0.9510565162951535312, 1.000000000000000000, 0.9510565162951535312, 1.000000000000000000, 0.9510565162951535312, 1.000000000000000000 ) ) 
 REPRESENTATION_ITEM ( '' )  );
#12380=CARTESIAN_POINT ( 'NONE',  ( 1.507698388325705758E-15, 1.624999997268798735, -24.62258325217400312 ) ) ;
#12381=CARTESIAN_POINT ( 'NONE',  ( 32.50000000000000000, 75.50000000546236834, -3.980102097228898626E-15 ) ) ;
#12385=ORIENTED_EDGE ( 'NONE', *, *, #30248, .F. ) ;
#12386=CARTESIAN_POINT ( 'NONE',  ( -10.37757302488624411, 74.97500000273119269, -31.93888565452638417 ) ) ;
#12389=CARTESIAN_POINT ( 'NONE',  ( -32.50000000000000000, 64.40000000546238823, -10.55989012756945478 ) ) ;
#12390=ORIENTED_EDGE ( 'NONE', *, *, #15026, .F. ) ;
#12391=CARTESIAN_POINT ( 'NONE',  ( -20.08610463437156923, 10.80000000546236372, 27.64615127144130113 ) ) ;
#12392=CARTESIAN_POINT ( 'NONE',  ( -27.16883889988623935, 49.32500000273118701, 19.73931689729374739 ) ) ;
#12393=CARTESIAN_POINT ( 'NONE',  ( -14.47279130897151589, 17.32499999726882933, -19.92008829642072598 ) ) ;
#12394=CARTESIAN_POINT ( 'NONE',  ( -32.50000000000000000, 6.500000005462358565, 0.000000000000000000 ) ) ;
#12395=CARTESIAN_POINT ( 'NONE',  ( -8.891200544363830713E-16, 77.50000000000001421, -15.00000000000000000 ) ) ;
#12397=CARTESIAN_POINT ( 'NONE',  ( 20.08610463437157279, 53.29999999999999716, -27.64615127144129758 ) ) ;
#12400=CARTESIAN_POINT ( 'NONE',  ( 33.58253175000000823, 20.27500000273117564, 10.91162601494192863 ) ) ;
#12401=CARTESIAN_POINT ( 'NONE',  ( -24.50000000000000000, 6.899999999999985256, -7.960532557706207157 ) ) ;
#12403=CARTESIAN_POINT ( 'NONE',  ( -4.300734207923759378, 78.97500000273119269, -13.23629886949340495 ) ) ;
#12404=DIRECTION ( 'NONE',  ( -0.000000000000000000, -1.000000000000000000, -0.000000000000000000 ) ) ;
#12405=CARTESIAN_POINT ( 'NONE',  ( 26.29305231718579350, 53.30000000546236549, 19.10302069950537529 ) ) ;
#12406=ADVANCED_FACE ( 'NONE', ( #15158 ), #2790, .T. ) ;
#12410=CARTESIAN_POINT ( 'NONE',  ( 13.91746824999999532, 71.97500000273120691, -4.522059556121118540 ) ) ;
#12416=CARTESIAN_POINT ( 'NONE',  ( -10.37757302488623701, 3.775000002731176973, 31.93888565452638417 ) ) ;
#12420=LINE ( 'NONE', #27868, #8933 ) ;
#12422=CARTESIAN_POINT ( 'NONE',  ( 10.37757302488624056, 44.52500000273118275, -31.93888565452638417 ) ) ;
#12424=CARTESIAN_POINT ( 'NONE',  ( -1.089172066684569321E-14, 78.49999999999998579, 15.00000000000000000 ) ) ;
#12425=ORIENTED_EDGE ( 'NONE', *, *, #19964, .F. ) ;
#12427=LINE ( 'NONE', #28721, #12984 ) ;
#12428=CARTESIAN_POINT ( 'NONE',  ( -14.47279130897152122, 13.92499999726881654, 19.92008829642072243 ) ) ;
#12430=CARTESIAN_POINT ( 'NONE',  ( -10.37757302488623701, 77.77500000273118985, 31.93888565452638417 ) ) ;
#12435=VERTEX_POINT ( 'NONE', #28364 ) ;
#12436=DIRECTION ( 'NONE',  ( -0.000000000000000000, -1.000000000000000000, -0.000000000000000000 ) ) ;
#12437=CARTESIAN_POINT ( 'NONE',  ( 6.486482029760649416E-15, 65.62500000273116996, 35.31076352940723240 ) ) ;
#12439=AXIS2_PLACEMENT_3D ( 'NONE', #21472, #24211, #32418 ) ;
#12440=CARTESIAN_POINT ( 'NONE',  ( -24.50000000000001066, 13.09999999999999432, 7.960532557706201828 ) ) ;
#12441=CARTESIAN_POINT ( 'NONE',  ( 23.41746824999999887, 5.224999997268801266, -7.608796670333727974 ) ) ;
#12442=CARTESIAN_POINT ( 'NONE',  ( -10.37757302488623701, 9.525000002731182747, 31.93888565452638417 ) ) ;
#12443=CARTESIAN_POINT ( 'NONE',  ( 3.445340210940985210E-14, 7.249999994537621895, 24.50000000000000000 ) ) ;
#12445=CARTESIAN_POINT ( 'NONE',  ( -9.270509831248421762, 72.30000000000002558, 12.75976212528060039 ) ) ;
#12447=CARTESIAN_POINT ( 'NONE',  ( -20.08610463437156923, 70.30000000000001137, 27.64615127144130113 ) ) ;
#12448=CARTESIAN_POINT ( 'NONE',  ( -4.635254915624211769, 73.85000000546237686, -14.26584774442730286 ) ) ;
#12450=CARTESIAN_POINT ( 'NONE',  ( -15.00000000000000000, 76.35000000546234844, 4.873795443493597723 ) ) ;
#12452=CARTESIAN_POINT ( 'NONE',  ( -33.58253175000000113, 33.22500000273117138, 10.91162601494193929 ) ) ;
#12455=CARTESIAN_POINT ( 'NONE',  ( -2.162160676586882350E-15, 18.87500000273119483, -35.31076352940722529 ) ) ;
#12456=LINE ( 'NONE', #17441, #18469 ) ;
#12457=CARTESIAN_POINT ( 'NONE',  ( -19.82091636218621389, 14.94999999453763806, 14.40073868116558842 ) ) ;
#12460=CARTESIAN_POINT ( 'NONE',  ( 23.41746824999999887, 14.72499999726882081, -7.608796670333727974 ) ) ;
#12461=CARTESIAN_POINT ( 'NONE',  ( -20.75514604977248823, 64.82500000273120122, -28.56700777964554305 ) ) ;
#12464=EDGE_CURVE ( 'NONE', #5395, #25303, #8762, .T. ) ;
#12465=CARTESIAN_POINT ( 'NONE',  ( -27.16883889988623935, 5.325000002731172799, 19.73931689729374739 ) ) ;
#12466=CARTESIAN_POINT ( 'NONE',  ( 7.236395654485760609, 13.52499999726880553, -22.27133577429736633 ) ) ;
#12468=ORIENTED_EDGE ( 'NONE', *, *, #4225, .T. ) ;
#12475=LINE ( 'NONE', #4746, #8520 ) ;
#12476=CARTESIAN_POINT ( 'NONE',  ( 14.47279130897151767, 3.424999997268800112, -19.92008829642072598 ) ) ;
#12477=CARTESIAN_POINT ( 'NONE',  ( 1.507698388325705758E-15, 11.12499999726881761, -24.62258325217400312 ) ) ;
#12478=CARTESIAN_POINT ( 'NONE',  ( 20.75514604977248467, 16.67500000273117777, -28.56700777964554305 ) ) ;
#12479=CARTESIAN_POINT ( 'NONE',  ( -20.08610463437157989, 24.20000000546238184, -27.64615127144129758 ) ) ;
#12481=CARTESIAN_POINT ( 'NONE',  ( 20.08610463437158344, 64.70000000000001705, 27.64615127144129403 ) ) ;
#12485=CARTESIAN_POINT ( 'NONE',  ( -20.75514604977248823, 27.07500000273119412, -28.56700777964554305 ) ) ;
#12486=CARTESIAN_POINT ( 'NONE',  ( 32.50000000000000000, 43.60000000546237686, -10.55989012756945833 ) ) ;
#12489=CARTESIAN_POINT ( 'NONE',  ( 14.47279130897151767, 15.42499999726882898, -19.92008829642072598 ) ) ;
#12490=CARTESIAN_POINT ( 'NONE',  ( -20.08610463437156923, 6.300000000000004263, 27.64615127144130113 ) ) ;
#12493=CARTESIAN_POINT ( 'NONE',  ( -33.58253175000000113, 49.02500000273116854, -10.91162601494193218 ) ) ;
#12495=CARTESIAN_POINT ( 'NONE',  ( -20.75514604977248112, 39.67500000273118133, 28.56700777964554661 ) ) ;
#12499=CARTESIAN_POINT ( 'NONE',  ( 33.58253175000000113, 2.225000002731166937, -10.91162601494193751 ) ) ;
#12503=CARTESIAN_POINT ( 'NONE',  ( -32.50000000000000000, 62.60000000546238397, 10.55989012756946366 ) ) ;
#12505=ADVANCED_FACE ( 'NONE', ( #13053 ), #19973, .T. ) ;
#12506=DIRECTION ( 'NONE',  ( 0.000000000000000000, 0.000000000000000000, -1.000000000000000000 ) ) ;
#12510=CARTESIAN_POINT ( 'NONE',  ( -10.37757302488623701, 29.52500000273117209, 31.93888565452638417 ) ) ;
#12516=CARTESIAN_POINT ( 'NONE',  ( -32.50000000000000000, 16.50000000546236834, 0.000000000000000000 ) ) ;
#12517=ORIENTED_EDGE ( 'NONE', *, *, #1891, .T. ) ;
#12523=CARTESIAN_POINT ( 'NONE',  ( 6.486482029760649416E-15, 31.87500000273119127, 35.31076352940723240 ) ) ;
#12524=CARTESIAN_POINT ( 'NONE',  ( -32.50000000000000000, 44.60000000546237686, 10.55989012756946366 ) ) ;
#12526=CARTESIAN_POINT ( 'NONE',  ( 33.58253175000000113, 20.22500000273117848, -10.91162601494193751 ) ) ;
#12528=CARTESIAN_POINT ( 'NONE',  ( 20.75514604977249178, 50.07500000273120122, 28.56700777964553950 ) ) ;
#12531=CARTESIAN_POINT ( 'NONE',  ( -26.29305231718578995, 28.20000000000000284, 19.10302069950538595 ) ) ;
#12533=CARTESIAN_POINT ( 'NONE',  ( -27.16883889988623935, 75.32500000273117280, 19.73931689729374739 ) ) ;
#12534=CARTESIAN_POINT ( 'NONE',  ( 0.000000000000000000, 0.000000000000000000, 0.000000000000000000 ) ) ;
#12535=CARTESIAN_POINT ( 'NONE',  ( -26.29305231718579350, 20.30000000546239391, -19.10302069950537884 ) ) ;
#12536=CARTESIAN_POINT ( 'NONE',  ( -20.75514604977248823, 59.07500000273120122, -28.56700777964554305 ) ) ;
#12539=CARTESIAN_POINT ( 'NONE',  ( -27.16883889988623935, 21.32500000273118701, 19.73931689729374739 ) ) ;
#12540=CARTESIAN_POINT ( 'NONE',  ( 24.50000000000000355, 9.649999994537628467, 7.960532557706212486 ) ) ;
#12542=CARTESIAN_POINT ( 'NONE',  ( -10.04305231718578462, 26.40000000000000568, 30.90933677959249337 ) ) ;
#12553=CARTESIAN_POINT ( 'NONE',  ( -1.778240108872766143E-15, 53.50000000000000000, -32.49999999999999289 ) ) ;
#12554=CARTESIAN_POINT ( 'NONE',  ( -10.37757302488623701, 1.525000002731202731, 31.93888565452638417 ) ) ;
#12558=ORIENTED_EDGE ( 'NONE', *, *, #22470, .F. ) ;
#12559=CARTESIAN_POINT ( 'NONE',  ( -20.75514604977248112, 73.67500000273120975, 28.56700777964554661 ) ) ;
#12562=CARTESIAN_POINT ( 'NONE',  ( 20.08610463437158344, 61.20000000546237118, 27.64615127144129403 ) ) ;
#12565=CARTESIAN_POINT ( 'NONE',  ( -10.37757302488624411, 40.72500000273118559, -31.93888565452638417 ) ) ;
#12566=CARTESIAN_POINT ( 'NONE',  ( 14.47279130897151767, 16.92499999726880944, -19.92008829642072598 ) ) ;
#12567=CARTESIAN_POINT ( 'NONE',  ( 32.50000000000000000, 5.600000005462384856, -10.55989012756945833 ) ) ;
#12568=CARTESIAN_POINT ( 'NONE',  ( -32.50000000000000000, 8.000000000000007105, 0.000000000000000000 ) ) ;
#12570=CARTESIAN_POINT ( 'NONE',  ( 26.29305231718579350, 46.80000000000001137, 19.10302069950537529 ) ) ;
#12571=DIRECTION ( 'NONE',  ( -0.000000000000000000, -1.000000000000000000, -0.000000000000000000 ) ) ;
#12572=CARTESIAN_POINT ( 'NONE',  ( -2.162160676586881955E-15, 14.87500000273120193, -35.31076352940723240 ) ) ;
#12573=CARTESIAN_POINT ( 'NONE',  ( -10.04305231718579172, 24.10000000546236265, -30.90933677959248982 ) ) ;
#12575=CARTESIAN_POINT ( 'NONE',  ( 4.300734207923761154, 79.97500000273119269, 13.23629886949340495 ) ) ;
#12576=CARTESIAN_POINT ( 'NONE',  ( -10.37757302488624411, 78.97500000273119269, -31.93888565452638417 ) ) ;
#12590=DIRECTION ( 'NONE',  ( -0.000000000000000000, -1.000000000000000000, -0.000000000000000000 ) ) ;
#12592=CARTESIAN_POINT ( 'NONE',  ( 27.16883889988623935, 46.32500000273117990, -19.73931689729374384 ) ) ;
#12596=EDGE_CURVE ( 'NONE', #13948, #26987, #32413, .T. ) ;
#12598=CARTESIAN_POINT ( 'NONE',  ( 5.779280353836490358E-15, 42.49999999999999289, 32.49999999999999289 ) ) ;
#12600=CARTESIAN_POINT ( 'NONE',  ( -20.75514604977248112, 75.67500000273118133, 28.56700777964554661 ) ) ;
#12605=ORIENTED_EDGE ( 'NONE', *, *, #20503, .T. ) ;
#12606=CARTESIAN_POINT ( 'NONE',  ( 0.000000000000000000, 70.00000000000000000, 0.000000000000000000 ) ) ;
#12607=CARTESIAN_POINT ( 'NONE',  ( -10.37757302488624411, 68.72500000273117848, -31.93888565452638417 ) ) ;
#12609=CARTESIAN_POINT ( 'NONE',  ( 24.50000000000000000, 12.00000000000001066, 0.000000000000000000 ) ) ;
#12610=LINE ( 'NONE', #2311, #30862 ) ;
#12611=CARTESIAN_POINT ( 'NONE',  ( 10.37757302488624767, 11.72500000273118914, 31.93888565452638417 ) ) ;
#12614=CARTESIAN_POINT ( 'NONE',  ( 9.270509831248425314, 72.70000000000001705, 12.75976212528059683 ) ) ;
#12619=CARTESIAN_POINT ( 'NONE',  ( -15.00000000000000000, 72.35000000546236265, 4.873795443493597723 ) ) ;
#12621=CARTESIAN_POINT ( 'NONE',  ( 33.58253175000000113, 28.22500000273119269, -10.91162601494193751 ) ) ;
#12624=CARTESIAN_POINT ( 'NONE',  ( -20.75514604977248112, 19.67500000273119909, 28.56700777964554661 ) ) ;
#12625=CARTESIAN_POINT ( 'NONE',  ( -5.147494310547423346, 12.94874572391553258, 32.50000000000000000 ) ) ;
#12626=CARTESIAN_POINT ( 'NONE',  ( -33.58253175000000113, 77.12500000273119838, 0.000000000000000000 ) ) ;
#12629=CARTESIAN_POINT ( 'NONE',  ( 14.47279130897151767, 16.32499999726879736, 19.92008829642072953 ) ) ;
#12630=CARTESIAN_POINT ( 'NONE',  ( 27.16883889988623935, 64.32500000273120122, -19.73931689729374384 ) ) ;
#12633=CARTESIAN_POINT ( 'NONE',  ( -27.16883889988623935, 9.325000002731176352, 19.73931689729374739 ) ) ;
#12634=CARTESIAN_POINT ( 'NONE',  ( -14.47279130897151589, 13.82499999726882045, -19.92008829642072598 ) ) ;
#12643=CARTESIAN_POINT ( 'NONE',  ( 7.236395654485760609, 3.524999997268824181, -22.27133577429736633 ) ) ;
#12644=CARTESIAN_POINT ( 'NONE',  ( 18.94512977948576093, 14.82499999726882933, -13.76444248337722875 ) ) ;
#12645=CARTESIAN_POINT ( 'NONE',  ( -10.37757302488623701, 15.77500000273118808, 31.93888565452638417 ) ) ;
#12646=CARTESIAN_POINT ( 'NONE',  ( -10.04305231718578462, 20.90000000546238113, 30.90933677959249337 ) ) ;
#12647=CARTESIAN_POINT ( 'NONE',  ( -20.08610463437157989, 65.69999999999998863, -27.64615127144129758 ) ) ;
#12648=CARTESIAN_POINT ( 'NONE',  ( 5.779280353836490358E-15, 7.000000005462371000, 32.49999999999999289 ) ) ;
#12651=CARTESIAN_POINT ( 'NONE',  ( 27.16883889988624290, 32.17500000273118843, 19.73931689729373673 ) ) ;
#12652=CARTESIAN_POINT ( 'NONE',  ( -8.960552108402742093E-16, 80.87500000273116996, -14.63369212191046387 ) ) ;
#12655=ADVANCED_FACE ( 'NONE', ( #32071 ), #6158, .T. ) ;
#12656=CARTESIAN_POINT ( 'NONE',  ( -23.41746825000000243, 14.02499999726881263, -7.608796670333730638 ) ) ;
#12657=CARTESIAN_POINT ( 'NONE',  ( 20.08610463437157279, 5.300000000000006928, -27.64615127144129758 ) ) ;
#12660=CARTESIAN_POINT ( 'NONE',  ( -20.75514604977248112, 53.42500000273117422, 28.56700777964554661 ) ) ;
#12662=CARTESIAN_POINT ( 'NONE',  ( -10.37757302488624411, 42.97500000273119269, -31.93888565452638417 ) ) ;
#12665=CARTESIAN_POINT ( 'NONE',  ( -3.880418787951142701, 9.448745718453144704, 24.49999999999999645 ) ) ;
#12666=AXIS2_PLACEMENT_3D ( 'NONE', #20239, #30679, #12506 ) ;
#12667=CARTESIAN_POINT ( 'NONE',  ( -32.50000000000000000, 22.60000000546237331, 10.55989012756946366 ) ) ;
#12670=CARTESIAN_POINT ( 'NONE',  ( 32.50000000000000000, 7.100000000000008527, -10.55989012756945833 ) ) ;
#12671=CYLINDRICAL_SURFACE ( 'NONE', #17750, 24.50000000000000000 ) ;
#12672=DIRECTION ( 'NONE',  ( 0.000000000000000000, 0.000000000000000000, -1.000000000000000000 ) ) ;
#12675=CARTESIAN_POINT ( 'NONE',  ( -7.570916362186215665, 11.14999999453764090, 23.30088464923126423 ) ) ;
#12676=CARTESIAN_POINT ( 'NONE',  ( -33.58253175000000113, 27.22500000273119269, 10.91162601494193929 ) ) ;
#12677=VECTOR ( 'NONE', #32188, 1000.000000000000000 ) ;
#12684=( BOUNDED_CURVE ( )  B_SPLINE_CURVE ( 2, ( #32372, #10954, #21594, #965, #6298, #19352, #471, #29794, #16774, #1126, #26897, #3396, #27234 ),
 .UNSPECIFIED., .F., .T. ) 
 B_SPLINE_CURVE_WITH_KNOTS ( ( 3, 2, 2, 2, 2, 2, 3 ),
 ( 0.3500000000000000333, 0.3599999999999999867, 0.3800000000000000044, 0.4000000000000000222, 0.4199999999999999845, 0.4400000000000000022, 0.4500000000000000111 ),
 .UNSPECIFIED. ) 
 CURVE ( )  GEOMETRIC_REPRESENTATION_ITEM ( )  RATIONAL_B_SPLINE_CURVE ( ( 0.9755282581475768211, 0.9755282581475768211, 1.000000000000000000, 0.9510565162951535312, 1.000000000000000000, 0.9510565162951535312, 1.000000000000000000, 0.9510565162951535312, 1.000000000000000000, 0.9510565162951535312, 1.000000000000000000, 0.9755282581475768211, 0.9755282581475768211 ) ) 
 REPRESENTATION_ITEM ( '' )  );
#12692=CARTESIAN_POINT ( 'NONE',  ( 33.58253175000000823, 36.27500000273119696, 10.91162601494192863 ) ) ;
#12693=CARTESIAN_POINT ( 'NONE',  ( 10.04305231718579705, 43.10000000546237686, 30.90933677959248982 ) ) ;
#12696=CARTESIAN_POINT ( 'NONE',  ( -10.37757302488624411, 22.72500000273119980, -31.93888565452638417 ) ) ;
#12698=CARTESIAN_POINT ( 'NONE',  ( -27.16883889988623935, 49.57500000273118701, 19.73931689729374739 ) ) ;
#12700=CARTESIAN_POINT ( 'NONE',  ( -10.04305231718579172, 29.60000000000001563, -30.90933677959248982 ) ) ;
#12702=CARTESIAN_POINT ( 'NONE',  ( 33.58253175000000113, 70.12500000273119838, -4.112674001490185761E-15 ) ) ;
#12703=CARTESIAN_POINT ( 'NONE',  ( -32.50000000000000000, 70.50000000546238255, 0.000000000000000000 ) ) ;
#12705=CARTESIAN_POINT ( 'NONE',  ( -33.58253175000000113, 61.27500000273118985, -10.91162601494193041 ) ) ;
#12708=CARTESIAN_POINT ( 'NONE',  ( -20.75514604977248112, 9.425000002731202642, 28.56700777964554661 ) ) ;
#12709=CARTESIAN_POINT ( 'NONE',  ( 24.50000000000000355, 11.84999999453761710, -7.960532557706203605 ) ) ;
#12711=CARTESIAN_POINT ( 'NONE',  ( 3.880418787951153803, 7.301254276084462091, 24.49999999999999645 ) ) ;
#12720=CARTESIAN_POINT ( 'NONE',  ( 10.04305231718579705, 62.59999999999998721, 30.90933677959248982 ) ) ;
#12723=CARTESIAN_POINT ( 'NONE',  ( -32.50000000000000000, 76.50000000546236834, 0.000000000000000000 ) ) ;
#12728=ORIENTED_EDGE ( 'NONE', *, *, #18928, .T. ) ;
#12729=CARTESIAN_POINT ( 'NONE',  ( -33.58253175000000113, 73.27500000273118985, -10.91162601494193218 ) ) ;
#12733=CARTESIAN_POINT ( 'NONE',  ( 20.75514604977249178, 54.07500000273118701, 28.56700777964553950 ) ) ;
#12734=CARTESIAN_POINT ( 'NONE',  ( 10.04305231718578817, 61.90000000546235981, -30.90933677959249337 ) ) ;
#12737=CARTESIAN_POINT ( 'NONE',  ( -27.16883889988623935, 45.32500000273117990, 19.73931689729374739 ) ) ;
#12738=CARTESIAN_POINT ( 'NONE',  ( 18.94512977948575738, 18.42499999726882010, 13.76444248337723408 ) ) ;
#12739=CARTESIAN_POINT ( 'NONE',  ( 10.37757302488624767, 65.97500000273120691, 31.93888565452638417 ) ) ;
#12740=CARTESIAN_POINT ( 'NONE',  ( -20.08610463437156923, 4.800000005462381480, 27.64615127144130113 ) ) ;
#12742=CARTESIAN_POINT ( 'NONE',  ( 3.000384657911015469E-15, 70.00000000000000000, -24.50000000000000000 ) ) ;
#12743=CARTESIAN_POINT ( 'NONE',  ( -26.29305231718579350, 45.80000000000000426, -19.10302069950537884 ) ) ;
#12744=FACE_OUTER_BOUND ( 'NONE', #22097, .T. ) ;
#12745=CARTESIAN_POINT ( 'NONE',  ( 33.58253175000000113, 12.47500000273119447, -10.91162601494193751 ) ) ;
#12746=AXIS2_PLACEMENT_3D ( 'NONE', #30214, #4145, #7053 ) ;
#12747=CARTESIAN_POINT ( 'NONE',  ( -15.14183272437242067, 6.699999999999991296, -20.84094480462497856 ) ) ;
#12749=CARTESIAN_POINT ( 'NONE',  ( -11.25946833292375793, 79.57500000273121543, 8.180482586598737171 ) ) ;
#12750=CARTESIAN_POINT ( 'NONE',  ( -20.75514604977248823, 77.07500000273118701, -28.56700777964554305 ) ) ;
#12765=CARTESIAN_POINT ( 'NONE',  ( -1.778240108872766143E-15, 53.50000000000000000, -32.49999999999999289 ) ) ;
#12767=CARTESIAN_POINT ( 'NONE',  ( 6.486482029760648627E-15, 45.62500000273119127, 35.31076352940722529 ) ) ;
#12769=CARTESIAN_POINT ( 'NONE',  ( 5.779280353836490358E-15, 21.00000000546237544, 32.49999999999999289 ) ) ;
#12770=VERTEX_POINT ( 'NONE', #3099 ) ;
#12774=CARTESIAN_POINT ( 'NONE',  ( -27.16883889988624290, 73.17500000273119554, -19.73931689729374028 ) ) ;
#12777=AXIS2_PLACEMENT_3D ( 'NONE', #25952, #4499, #9822 ) ;
#12780=CARTESIAN_POINT ( 'NONE',  ( 26.29305231718579350, 29.30000000546237260, 19.10302069950537529 ) ) ;
#12781=CARTESIAN_POINT ( 'NONE',  ( -27.16883889988623935, 61.32500000273119412, 19.73931689729374739 ) ) ;
#12783=CARTESIAN_POINT ( 'NONE',  ( -7.570916362186215665, 17.39999999999999858, 23.30088464923126423 ) ) ;
#12784=CARTESIAN_POINT ( 'NONE',  ( 23.41746824999999887, 3.124999997268812280, 0.000000000000000000 ) ) ;
#12785=CARTESIAN_POINT ( 'NONE',  ( 27.16883889988623935, 6.325000002731173687, -19.73931689729374384 ) ) ;
#12786=CARTESIAN_POINT ( 'NONE',  ( -24.50000000000000000, 6.649999994537635573, -7.960532557706207157 ) ) ;
#12788=CARTESIAN_POINT ( 'NONE',  ( -15.00000000000000000, 74.10000000000002274, 4.873795443493597723 ) ) ;
#12789=CARTESIAN_POINT ( 'NONE',  ( 0.000000000000000000, 80.00000000000001421, 0.000000000000000000 ) ) ;
#12790=FACE_OUTER_BOUND ( 'NONE', #25212, .T. ) ;
#12793=CARTESIAN_POINT ( 'NONE',  ( -8.601468415847518756, 80.57500000273118701, -11.83890561707634781 ) ) ;
#12796=CARTESIAN_POINT ( 'NONE',  ( 27.16883889988623935, 34.32500000273120122, -19.73931689729374384 ) ) ;
#12799=CARTESIAN_POINT ( 'NONE',  ( 20.75514604977249178, 20.07500000273118701, 28.56700777964553950 ) ) ;
#12802=CARTESIAN_POINT ( 'NONE',  ( -20.75514604977248823, 78.82500000273120122, -28.56700777964554305 ) ) ;
#12805=CARTESIAN_POINT ( 'NONE',  ( -23.41746824999999887, 15.62499999726882294, -2.867812753649727150E-15 ) ) ;
#12806=CARTESIAN_POINT ( 'NONE',  ( -10.37757302488623701, 63.52500000273120406, 31.93888565452638417 ) ) ;
#12809=CARTESIAN_POINT ( 'NONE',  ( -33.58253175000000113, 7.125000002731196602, 0.000000000000000000 ) ) ;
#12810=CARTESIAN_POINT ( 'NONE',  ( 18.94512977948576093, 17.32499999726880446, -13.76444248337722875 ) ) ;
#12812=VERTEX_POINT ( 'NONE', #33075 ) ;
#12814=ORIENTED_EDGE ( 'NONE', *, *, #755, .F. ) ;
#12816=CARTESIAN_POINT ( 'NONE',  ( 3.980102097228898626E-15, 80.00000000000001421, 32.50000000000000000 ) ) ;
#12818=CARTESIAN_POINT ( 'NONE',  ( -10.37757302488624411, 78.72500000273119269, -31.93888565452638417 ) ) ;
#12820=CARTESIAN_POINT ( 'NONE',  ( -14.47279130897152122, 2.424999997268802332, 19.92008829642072243 ) ) ;
#12822=CARTESIAN_POINT ( 'NONE',  ( 1.507698388325705758E-15, 15.12499999726880873, -24.62258325217400312 ) ) ;
#12823=CARTESIAN_POINT ( 'NONE',  ( 33.58253175000000823, 16.27500000273118630, 10.91162601494192863 ) ) ;
#12824=CARTESIAN_POINT ( 'NONE',  ( -26.29305231718578995, 18.70000000546237473, 19.10302069950538595 ) ) ;
#12825=CARTESIAN_POINT ( 'NONE',  ( -32.50000000000000000, 65.89999999999997726, -10.55989012756945478 ) ) ;
#12826=CARTESIAN_POINT ( 'NONE',  ( 3.880418787951134707, 11.30125427608447097, 24.50000000000000000 ) ) ;
#12827=CARTESIAN_POINT ( 'NONE',  ( 5.779280353836490358E-15, 29.00000000546237544, 32.49999999999999289 ) ) ;
#12829=CARTESIAN_POINT ( 'NONE',  ( -26.29305231718579350, 32.30000000546237260, -19.10302069950537884 ) ) ;
#12832=CARTESIAN_POINT ( 'NONE',  ( -18.94512977948575738, 17.92499999726882010, -13.76444248337723231 ) ) ;
#12833=CARTESIAN_POINT ( 'NONE',  ( 26.29305231718578995, 7.199999999999984190, -19.10302069950538240 ) ) ;
#12834=FACE_OUTER_BOUND ( 'NONE', #26978, .T. ) ;
#12835=EDGE_CURVE ( 'NONE', #19940, #5896, #6362, .T. ) ;
#12837=CARTESIAN_POINT ( 'NONE',  ( -33.58253175000000113, 49.12500000273117706, 0.000000000000000000 ) ) ;
#12839=CARTESIAN_POINT ( 'NONE',  ( -33.58253175000000113, 39.37500000273119838, 0.000000000000000000 ) ) ;
#12847=DIRECTION ( 'NONE',  ( -0.000000000000000000, -1.000000000000000000, -0.000000000000000000 ) ) ;
#12851=CARTESIAN_POINT ( 'NONE',  ( -33.04126587500000056, 0.8125000040967722548, 0.000000000000000000 ) ) ;
#12852=CARTESIAN_POINT ( 'NONE',  ( 33.58253175000000113, 26.12500000273118417, -4.112674001490185761E-15 ) ) ;
#12854=EDGE_LOOP ( 'NONE', ( #8622, #5911, #1435, #13033 ) ) ;
#12863=CARTESIAN_POINT ( 'NONE',  ( -27.16883889988624290, 33.17500000273118843, -19.73931689729374028 ) ) ;
#12864=CARTESIAN_POINT ( 'NONE',  ( 32.50000000000000711, 35.40000000546237402, 10.55989012756945122 ) ) ;
#12867=CARTESIAN_POINT ( 'NONE',  ( -27.16883889988624290, 24.92500000273117777, -19.73931689729374028 ) ) ;
#12868=CARTESIAN_POINT ( 'NONE',  ( 15.14183272437242067, 5.449999994537614967, 20.84094480462498211 ) ) ;
#12869=CARTESIAN_POINT ( 'NONE',  ( -10.37757302488624411, 50.97500000273119980, -31.93888565452638417 ) ) ;
#12872=CARTESIAN_POINT ( 'NONE',  ( 20.08610463437158344, 30.69999999999999218, 27.64615127144129403 ) ) ;
#12874=CARTESIAN_POINT ( 'NONE',  ( 6.486482029760649416E-15, 69.62500000273118417, 35.31076352940723240 ) ) ;
#12876=CARTESIAN_POINT ( 'NONE',  ( -1.778240108872766143E-15, 20.00000000546237544, -32.49999999999999289 ) ) ;
#12877=CARTESIAN_POINT ( 'NONE',  ( -27.16883889988624290, 61.17500000273118133, -19.73931689729374028 ) ) ;
#12878=CARTESIAN_POINT ( 'NONE',  ( 10.04305231718579705, 7.100000005462375974, 30.90933677959248982 ) ) ;
#12879=CARTESIAN_POINT ( 'NONE',  ( -33.58253175000000113, 13.22500000273119802, 10.91162601494193929 ) ) ;
#12894=CARTESIAN_POINT ( 'NONE',  ( -32.50000000000000000, 78.50000000546236834, 0.000000000000000000 ) ) ;
#12899=CARTESIAN_POINT ( 'NONE',  ( 33.58253175000000113, 76.47500000273117848, -10.91162601494193751 ) ) ;
#12903=CARTESIAN_POINT ( 'NONE',  ( -10.37757302488624411, 52.97500000273119980, -31.93888565452638417 ) ) ;
#12904=CARTESIAN_POINT ( 'NONE',  ( -32.50000000000000000, 54.50000000546237544, 0.000000000000000000 ) ) ;
#12906=CARTESIAN_POINT ( 'NONE',  ( 3.245314017740486554E-15, 0.000000000000000000, -26.50000000000000355 ) ) ;
#12907=CARTESIAN_POINT ( 'NONE',  ( 33.58253175000000823, 40.02500000273119696, 10.91162601494192863 ) ) ;
#12908=CARTESIAN_POINT ( 'NONE',  ( 2.445080149700053643E-15, 72.75000000546238255, 15.00000000000000000 ) ) ;
#12909=CARTESIAN_POINT ( 'NONE',  ( -10.37757302488623701, 65.77500000273117564, 31.93888565452638417 ) ) ;
#12910=CARTESIAN_POINT ( 'NONE',  ( -32.50000000000000000, 2.600000005462363095, 10.55989012756946366 ) ) ;
#12912=CARTESIAN_POINT ( 'NONE',  ( 26.29305231718578995, 49.19999999999999574, -19.10302069950538240 ) ) ;
#12913=CARTESIAN_POINT ( 'NONE',  ( -20.08610463437156923, 14.29999999999998472, 27.64615127144130113 ) ) ;
#12914=CARTESIAN_POINT ( 'NONE',  ( -27.16883889988623935, 13.57500000273120833, 19.73931689729374739 ) ) ;
#12915=CARTESIAN_POINT ( 'NONE',  ( -32.50000000000000000, 74.10000000000000853, 10.55989012756946366 ) ) ;
#12917=CARTESIAN_POINT ( 'NONE',  ( -11.25946833292375793, 79.17500000273119554, -8.180482586598733619 ) ) ;
#12918=CARTESIAN_POINT ( 'NONE',  ( 27.16883889988623935, 76.57500000273120122, -19.73931689729374384 ) ) ;
#12930=ADVANCED_FACE ( 'NONE', ( #32899 ), #24854, .T. ) ;
#12934=CARTESIAN_POINT ( 'NONE',  ( 33.58253175000000823, 48.02500000273120406, 10.91162601494192685 ) ) ;
#12936=EDGE_CURVE ( 'NONE', #12338, #26701, #30006, .T. ) ;
#12938=DIRECTION ( 'NONE',  ( -0.000000000000000000, -1.000000000000000000, -0.000000000000000000 ) ) ;
#12943=CARTESIAN_POINT ( 'NONE',  ( 10.37757302488624056, 72.77500000273118985, -31.93888565452638417 ) ) ;
#12950=DIRECTION ( 'NONE',  ( -0.000000000000000000, 1.000000000000000000, -0.000000000000000000 ) ) ;
#12951=CARTESIAN_POINT ( 'NONE',  ( -27.16883889988624290, 58.92500000273118133, -19.73931689729374028 ) ) ;
#12953=CARTESIAN_POINT ( 'NONE',  ( 19.82091636218621034, 15.80000000000000782, 14.40073868116559730 ) ) ;
#12954=CARTESIAN_POINT ( 'NONE',  ( 14.47279130897151767, 2.824999997268819119, 19.92008829642072953 ) ) ;
#12955=CARTESIAN_POINT ( 'NONE',  ( -33.58253175000000113, 5.225000002731188253, 10.91162601494193929 ) ) ;
#12956=CARTESIAN_POINT ( 'NONE',  ( 10.04305231718579705, 28.60000000000001563, 30.90933677959248982 ) ) ;
#12958=CARTESIAN_POINT ( 'NONE',  ( 33.58253175000000823, 78.27500000273116143, 10.91162601494192863 ) ) ;
#12960=CARTESIAN_POINT ( 'NONE',  ( -20.08610463437156923, 4.300000000000009592, 27.64615127144130113 ) ) ;
#12964=CARTESIAN_POINT ( 'NONE',  ( -15.00000000000000000, 74.25000000546239676, 0.000000000000000000 ) ) ;
#12966=CARTESIAN_POINT ( 'NONE',  ( -10.37757302488623701, 31.52500000273117564, 31.93888565452638417 ) ) ;
#12969=CARTESIAN_POINT ( 'NONE',  ( -10.37757302488624411, 20.97500000273119625, -31.93888565452638417 ) ) ;
#12970=CARTESIAN_POINT ( 'NONE',  ( -26.29305231718579350, 63.79999999999999716, -19.10302069950537884 ) ) ;
#12972=CARTESIAN_POINT ( 'NONE',  ( 6.486482029760648627E-15, 75.62500000273119838, 35.31076352940722529 ) ) ;
#12973=FACE_OUTER_BOUND ( 'NONE', #18023, .T. ) ;
#12975=CARTESIAN_POINT ( 'NONE',  ( 7.236395654485760609, 15.02499999726880731, -22.27133577429736633 ) ) ;
#12976=CARTESIAN_POINT ( 'NONE',  ( 10.37757302488624056, 64.52500000273120406, -31.93888565452638417 ) ) ;
#12980=CARTESIAN_POINT ( 'NONE',  ( 33.58253175000000823, 8.025000002731188076, 10.91162601494192685 ) ) ;
#12981=CARTESIAN_POINT ( 'NONE',  ( -23.41746824999999887, 16.12499999726882294, -2.867812753649727150E-15 ) ) ;
#12984=VECTOR ( 'NONE', #15699, 1000.000000000000000 ) ;
#12987=( BOUNDED_CURVE ( )  B_SPLINE_CURVE ( 2, ( #13850, #16758, #22075, #32520, #8521, #13685, #8851, #27217, #16431, #21413, #31856, #19501, #3710 ),
 .UNSPECIFIED., .F., .F. ) 
 B_SPLINE_CURVE_WITH_KNOTS ( ( 3, 2, 2, 2, 2, 2, 3 ),
 ( 0.3653846153846153633, 0.3666666666666666408, 0.3692307692307692513, 0.3717948717948718063, 0.3743589743589743613, 0.3769230769230769162, 0.3782051282051281937 ),
 .UNSPECIFIED. ) 
 CURVE ( )  GEOMETRIC_REPRESENTATION_ITEM ( )  RATIONAL_B_SPLINE_CURVE ( ( 0.9755282581475768211, 0.9755282581475768211, 1.000000000000000000, 0.9510565162951535312, 1.000000000000000000, 0.9510565162951535312, 1.000000000000000000, 0.9510565162951535312, 1.000000000000000000, 0.9510565162951535312, 1.000000000000000000, 0.9755282581475768211, 0.9755282581475768211 ) ) 
 REPRESENTATION_ITEM ( '' )  );
#12992=CARTESIAN_POINT ( 'NONE',  ( -4.934616302121927505E-14, 72.50000000000001421, 32.50000000000000000 ) ) ;
#12993=CARTESIAN_POINT ( 'NONE',  ( -23.41746824999999887, 6.124999997268814944, -2.867812753649727150E-15 ) ) ;
#12994=CARTESIAN_POINT ( 'NONE',  ( -7.236395654485757944, 17.22499999726881370, -22.27133577429736988 ) ) ;
#12995=CARTESIAN_POINT ( 'NONE',  ( 33.58253175000000823, 14.27500000273119340, 10.91162601494192863 ) ) ;
#12996=CARTESIAN_POINT ( 'NONE',  ( -10.04305231718578462, 56.40000000000000568, 30.90933677959249337 ) ) ;
#12998=CARTESIAN_POINT ( 'NONE',  ( -1.778240108872766143E-15, 29.50000000000000711, -32.49999999999999289 ) ) ;
#13000=CARTESIAN_POINT ( 'NONE',  ( -8.960552108402742093E-16, 78.87500000273118417, -14.63369212191046387 ) ) ;
#13003=DIRECTION ( 'NONE',  ( 0.000000000000000000, 0.000000000000000000, -1.000000000000000000 ) ) ;
#13004=CARTESIAN_POINT ( 'NONE',  ( 0.000000000000000000, 0.000000000000000000, 0.000000000000000000 ) ) ;
#13005=CARTESIAN_POINT ( 'NONE',  ( -32.50000000000000000, 8.000000000000007105, 0.000000000000000000 ) ) ;
#13008=CARTESIAN_POINT ( 'NONE',  ( -33.58253175000000113, 49.22500000273119269, 10.91162601494193929 ) ) ;
#13010=CARTESIAN_POINT ( 'NONE',  ( 10.37757302488624056, 40.77500000273118275, -31.93888565452638417 ) ) ;
#13011=CYLINDRICAL_SURFACE ( 'NONE', #14541, 32.50000000000000000 ) ;
#13016=CARTESIAN_POINT ( 'NONE',  ( -32.50000000000000000, 28.10000000000001208, 10.55989012756946366 ) ) ;
#13018=CARTESIAN_POINT ( 'NONE',  ( -13.91746824999999532, 81.27500000273120406, -4.522059556121115875 ) ) ;
#13019=CARTESIAN_POINT ( 'NONE',  ( 23.95873412499999944, 18.31249999863440792, 0.000000000000000000 ) ) ;
#13020=CARTESIAN_POINT ( 'NONE',  ( 3.880418787951159132, 10.19874571299079236, -24.49999999999999289 ) ) ;
#13023=CARTESIAN_POINT ( 'NONE',  ( 20.08610463437158344, 10.70000000000001172, 27.64615127144129403 ) ) ;
#13024=CARTESIAN_POINT ( 'NONE',  ( -27.16883889988623935, 25.32500000273119056, 19.73931689729374739 ) ) ;
#13029=ADVANCED_FACE ( 'NONE', ( #33253 ), #9749, .T. ) ;
#13033=ORIENTED_EDGE ( 'NONE', *, *, #2129, .F. ) ;
#13036=LINE ( 'NONE', #23507, #27795 ) ;
#13037=CARTESIAN_POINT ( 'NONE',  ( -10.37757302488623701, 35.77500000273120406, 31.93888565452638417 ) ) ;
#13038=CARTESIAN_POINT ( 'NONE',  ( 10.04305231718579705, 39.10000000546237686, 30.90933677959248982 ) ) ;
#13040=CARTESIAN_POINT ( 'NONE',  ( -26.29305231718578995, 48.19999999999999574, 19.10302069950538595 ) ) ;
#13041=CARTESIAN_POINT ( 'NONE',  ( 33.58253175000000823, 20.02500000273118275, 10.91162601494192863 ) ) ;
#13042=CARTESIAN_POINT ( 'NONE',  ( 6.486482029760649416E-15, 51.87500000273119127, 35.31076352940723240 ) ) ;
#13044=CARTESIAN_POINT ( 'NONE',  ( -32.50000000000000000, 25.89999999999999503, -10.55989012756945478 ) ) ;
#13046=CARTESIAN_POINT ( 'NONE',  ( 6.486482029760649416E-15, 67.62500000273119838, 35.31076352940723240 ) ) ;
#13048=CARTESIAN_POINT ( 'NONE',  ( -5.147494310547430452, 76.94874572391552192, 32.50000000000000000 ) ) ;
#13049=CARTESIAN_POINT ( 'NONE',  ( -2.162160676586882350E-15, 60.87500000273117706, -35.31076352940722529 ) ) ;
#13050=DIRECTION ( 'NONE',  ( -0.000000000000000000, -1.000000000000000000, -0.000000000000000000 ) ) ;
#13051=CARTESIAN_POINT ( 'NONE',  ( -33.58253175000000113, 15.12500000273120371, 0.000000000000000000 ) ) ;
#13053=FACE_OUTER_BOUND ( 'NONE', #2813, .T. ) ;
#13056=CARTESIAN_POINT ( 'NONE',  ( 3.778760231354629433E-15, 0.5000000000000067724, -24.50000000000000355 ) ) ;
#13062=CARTESIAN_POINT ( 'NONE',  ( -1.053607264507113999E-13, 63.00000000546238255, 32.50000000000000711 ) ) ;
#13063=CARTESIAN_POINT ( 'NONE',  ( 32.50000000000000000, 67.60000000546237686, -10.55989012756945833 ) ) ;
#13073=CARTESIAN_POINT ( 'NONE',  ( -27.16883889988624290, 57.17500000273118133, -19.73931689729374028 ) ) ;
#13075=CARTESIAN_POINT ( 'NONE',  ( -26.29305231718579350, 54.30000000546236549, -19.10302069950537884 ) ) ;
#13076=CARTESIAN_POINT ( 'NONE',  ( -15.14183272437242778, 13.04999999453763770, 20.84094480462497856 ) ) ;
#13077=CARTESIAN_POINT ( 'NONE',  ( 27.16883889988624290, 39.92500000273119554, 19.73931689729373673 ) ) ;
#13079=CARTESIAN_POINT ( 'NONE',  ( 10.37757302488624056, 70.77500000273117564, -31.93888565452638417 ) ) ;
#13080=CARTESIAN_POINT ( 'NONE',  ( 10.04305231718578817, 1.900000005462365582, -30.90933677959249337 ) ) ;
#13083=CARTESIAN_POINT ( 'NONE',  ( 20.08610463437158344, 46.70000000000000284, 27.64615127144129403 ) ) ;
#13085=CARTESIAN_POINT ( 'NONE',  ( -27.16883889988624290, 13.17500000273119554, -19.73931689729374028 ) ) ;
#13088=CARTESIAN_POINT ( 'NONE',  ( 11.25946833292375793, 78.17500000273119554, 8.180482586598731842 ) ) ;
#13090=CARTESIAN_POINT ( 'NONE',  ( 0.000000000000000000, 80.00000000000001421, 0.000000000000000000 ) ) ;
#13092=ORIENTED_EDGE ( 'NONE', *, *, #11730, .T. ) ;
#13093=DIRECTION ( 'NONE',  ( -0.000000000000000000, -1.000000000000000000, -0.000000000000000000 ) ) ;
#13104=CARTESIAN_POINT ( 'NONE',  ( -33.58253175000000113, 41.12500000273119838, 0.000000000000000000 ) ) ;
#13107=CARTESIAN_POINT ( 'NONE',  ( -20.08610463437157989, 2.200000005462376063, -27.64615127144129758 ) ) ;
#13110=CARTESIAN_POINT ( 'NONE',  ( -1.778240108872766143E-15, 4.000000005462373664, -32.49999999999999289 ) ) ;
#13112=CARTESIAN_POINT ( 'NONE',  ( -33.58253175000000113, 77.27500000273117564, -10.91162601494193218 ) ) ;
#13118=CARTESIAN_POINT ( 'NONE',  ( -33.58253175000000113, 61.12500000273119127, 0.000000000000000000 ) ) ;
#13120=CARTESIAN_POINT ( 'NONE',  ( -14.47279130897151767, 11.82499999726882578, -19.92008829642072598 ) ) ;
#13121=CARTESIAN_POINT ( 'NONE',  ( 10.37757302488624056, 2.525000002731203619, -31.93888565452638417 ) ) ;
#13124=CARTESIAN_POINT ( 'NONE',  ( 5.779280353836490358E-15, 61.00000000546238255, 32.49999999999999289 ) ) ;
#13130=CARTESIAN_POINT ( 'NONE',  ( 4.300734207923761154, 79.47500000273119269, 13.23629886949340495 ) ) ;
#13132=CARTESIAN_POINT ( 'NONE',  ( 33.58253175000000823, 30.02500000273118985, 10.91162601494192863 ) ) ;
#13135=CARTESIAN_POINT ( 'NONE',  ( -10.37757302488623701, 15.77500000273118808, 31.93888565452638417 ) ) ;
#13138=EDGE_CURVE ( 'NONE', #22725, #15526, #23013, .T. ) ;
#13139=CARTESIAN_POINT ( 'NONE',  ( -27.16883889988623935, 77.32500000273118701, 19.73931689729374739 ) ) ;
#13140=CARTESIAN_POINT ( 'NONE',  ( 19.82091636218621034, 7.800000000000001599, 14.40073868116559730 ) ) ;
#13142=CARTESIAN_POINT ( 'NONE',  ( 18.94512977948575738, 16.42499999726882010, 13.76444248337723408 ) ) ;
#13143=CARTESIAN_POINT ( 'NONE',  ( 33.58253175000000113, 64.12500000273119838, -4.112674001490185761E-15 ) ) ;
#13147=CARTESIAN_POINT ( 'NONE',  ( -20.75514604977248823, 4.825000002731171911, -28.56700777964554305 ) ) ;
#13148=CARTESIAN_POINT ( 'NONE',  ( -18.94512977948575738, 15.92499999726881832, -13.76444248337723231 ) ) ;
#13154=CARTESIAN_POINT ( 'NONE',  ( 5.147494310547434893, 11.05125428700922896, 32.49999999999999289 ) ) ;
#13158=CARTESIAN_POINT ( 'NONE',  ( 15.14183272437242245, 2.299999999999985612, -20.84094480462497856 ) ) ;
#13159=CARTESIAN_POINT ( 'NONE',  ( 33.58253175000000113, 16.47500000273118204, -10.91162601494193751 ) ) ;
#13160=CARTESIAN_POINT ( 'NONE',  ( -20.08610463437156923, 62.29999999999997584, 27.64615127144130113 ) ) ;
#13161=CARTESIAN_POINT ( 'NONE',  ( -4.300734207923755825, 79.27500000273118985, 13.23629886949340673 ) ) ;
#13162=CARTESIAN_POINT ( 'NONE',  ( -5.147494310547423346, 30.44874571845313938, 32.50000000000000000 ) ) ;
#13164=CARTESIAN_POINT ( 'NONE',  ( 11.25946833292375793, 78.57500000273121543, -8.180482586598735395 ) ) ;
#13167=FACE_OUTER_BOUND ( 'NONE', #15847, .T. ) ;
#13168=CARTESIAN_POINT ( 'NONE',  ( 7.570916362186213000, 16.39999999999999858, -23.30088464923126423 ) ) ;
#13169=CARTESIAN_POINT ( 'NONE',  ( 32.50000000000000711, 2.899999999999995470, 10.55989012756945122 ) ) ;
#13170=CARTESIAN_POINT ( 'NONE',  ( -15.00000000000000000, 73.90000000000001990, -4.873795443493594171 ) ) ;
#13172=CARTESIAN_POINT ( 'NONE',  ( 33.58253175000000113, 48.12500000273117706, -4.112674001490185761E-15 ) ) ;
#13175=CARTESIAN_POINT ( 'NONE',  ( 33.58253175000000113, 36.37500000273119838, -4.112674001490185761E-15 ) ) ;
#13176=CARTESIAN_POINT ( 'NONE',  ( 0.000000000000000000, 80.00000000000001421, 0.000000000000000000 ) ) ;
#13182=CARTESIAN_POINT ( 'NONE',  ( -1.778240108872766143E-15, 62.00000000546238255, -32.49999999999999289 ) ) ;
#13183=CARTESIAN_POINT ( 'NONE',  ( 0.000000000000000000, 70.00000000000000000, 0.000000000000000000 ) ) ;
#13184=CARTESIAN_POINT ( 'NONE',  ( 24.50000000000000000, 12.00000000000001066, 0.000000000000000000 ) ) ;
#13187=( BOUNDED_CURVE ( )  B_SPLINE_CURVE ( 2, ( #1532, #17858, #17339, #17173, #22477, #7199, #17680, #27802, #9424, #9605, #25738, #22649, #27630 ),
 .UNSPECIFIED., .F., .T. ) 
 B_SPLINE_CURVE_WITH_KNOTS ( ( 3, 2, 2, 2, 2, 2, 3 ),
 ( 0.6388888888888889506, 0.6444444444444444864, 0.6555555555555555580, 0.6666666666666666297, 0.6777777777777778123, 0.6888888888888888840, 0.6944444444444444198 ),
 .UNSPECIFIED. ) 
 CURVE ( )  GEOMETRIC_REPRESENTATION_ITEM ( )  RATIONAL_B_SPLINE_CURVE ( ( 0.9755282581475768211, 0.9755282581475770431, 1.000000000000000000, 0.9510565162951535312, 1.000000000000000000, 0.9510565162951535312, 1.000000000000000000, 0.9510565162951535312, 1.000000000000000000, 0.9510565162951535312, 1.000000000000000000, 0.9755282581475768211, 0.9755282581475768211 ) ) 
 REPRESENTATION_ITEM ( '' )  );
#13188=CARTESIAN_POINT ( 'NONE',  ( 7.313012447739250820E-14, 17.24999999453762456, 24.50000000000000000 ) ) ;
#13189=CARTESIAN_POINT ( 'NONE',  ( 10.37757302488624767, 25.72500000273120335, 31.93888565452638417 ) ) ;
#13197=CARTESIAN_POINT ( 'NONE',  ( 1.507698388325705758E-15, 1.124999997268814722, -24.62258325217400312 ) ) ;
#13198=CARTESIAN_POINT ( 'NONE',  ( 20.75514604977248467, 32.67500000273118843, -28.56700777964554305 ) ) ;
#13199=CARTESIAN_POINT ( 'NONE',  ( 20.08610463437157279, 35.80000000546235128, -27.64615127144129758 ) ) ;
#13200=CARTESIAN_POINT ( 'NONE',  ( -2.092463501923844636E-15, 77.50000000000000000, -34.17252228774368916 ) ) ;
#13201=CARTESIAN_POINT ( 'NONE',  ( -32.50000000000000000, 47.89999999999999858, -10.55989012756945300 ) ) ;
#13202=CARTESIAN_POINT ( 'NONE',  ( 1.093617666956751375E-13, 61.50000000000000000, -32.50000000000000711 ) ) ;
#13203=CARTESIAN_POINT ( 'NONE',  ( 20.75514604977248467, 46.67500000273118133, -28.56700777964554305 ) ) ;
#13206=CARTESIAN_POINT ( 'NONE',  ( 20.08610463437158344, 24.70000000000000284, 27.64615127144129403 ) ) ;
#13208=CARTESIAN_POINT ( 'NONE',  ( -33.58253175000000113, 69.12500000273119838, 0.000000000000000000 ) ) ;
#13211=CARTESIAN_POINT ( 'NONE',  ( -33.58253175000000113, 63.27500000273118985, -10.91162601494193041 ) ) ;
#13212=CARTESIAN_POINT ( 'NONE',  ( 5.147494310547426899, 39.94874572391552903, -32.50000000000000000 ) ) ;
#13213=CARTESIAN_POINT ( 'NONE',  ( 20.75514604977248467, 10.42500000273120087, -28.56700777964554305 ) ) ;
#13216=CARTESIAN_POINT ( 'NONE',  ( 24.50000000000000000, 1.849999994537612658, -7.960532557706203605 ) ) ;
#13219=DIRECTION ( 'NONE',  ( 0.000000000000000000, 0.000000000000000000, -1.000000000000000000 ) ) ;
#13220=CARTESIAN_POINT ( 'NONE',  ( 26.29305231718578995, 19.19999999999999574, -19.10302069950538240 ) ) ;
#13228=CARTESIAN_POINT ( 'NONE',  ( 23.41746825000000243, 7.024999997268802865, 7.608796670333735079 ) ) ;
#13229=CARTESIAN_POINT ( 'NONE',  ( 32.50000000000000000, 71.60000000546240528, -10.55989012756945833 ) ) ;
#13238=DIRECTION ( 'NONE',  ( -0.000000000000000000, -1.000000000000000000, -0.000000000000000000 ) ) ;
#13239=CARTESIAN_POINT ( 'NONE',  ( -20.75514604977248823, 57.07500000273117280, -28.56700777964554305 ) ) ;
#13240=CARTESIAN_POINT ( 'NONE',  ( 10.04305231718578817, 53.90000000546238113, -30.90933677959249337 ) ) ;
#13243=CARTESIAN_POINT ( 'NONE',  ( -33.58253175000000113, 43.22500000273118559, 10.91162601494193929 ) ) ;
#13244=CARTESIAN_POINT ( 'NONE',  ( 20.08610463437157279, 55.29999999999999716, -27.64615127144129758 ) ) ;
#13246=CARTESIAN_POINT ( 'NONE',  ( -10.37757302488623701, 67.77500000273117564, 31.93888565452638417 ) ) ;
#13247=DIRECTION ( 'NONE',  ( -0.000000000000000000, -1.000000000000000000, -0.000000000000000000 ) ) ;
#13250=CARTESIAN_POINT ( 'NONE',  ( 6.277390505771533514E-15, 48.50000000000000711, 34.17252228774368916 ) ) ;
#13252=CARTESIAN_POINT ( 'NONE',  ( -2.162160676586881955E-15, 10.87500000273118417, -35.31076352940723240 ) ) ;
#13253=FACE_OUTER_BOUND ( 'NONE', #11908, .T. ) ;
#13255=CARTESIAN_POINT ( 'NONE',  ( 13.91746825000000065, 72.27500000273118985, 4.522059556121114987 ) ) ;
#13259=ORIENTED_EDGE ( 'NONE', *, *, #17767, .F. ) ;
#13260=CARTESIAN_POINT ( 'NONE',  ( 0.000000000000000000, 70.00000000000000000, 0.000000000000000000 ) ) ;
#13271=CARTESIAN_POINT ( 'NONE',  ( 20.75514604977248467, 36.42500000273118843, -28.56700777964554305 ) ) ;
#13279=CARTESIAN_POINT ( 'NONE',  ( 10.37757302488624767, 71.97500000273119269, 31.93888565452638417 ) ) ;
#13280=ORIENTED_EDGE ( 'NONE', *, *, #32350, .F. ) ;
#13284=VECTOR ( 'NONE', #3678, 1000.000000000000000 ) ;
#13286=CARTESIAN_POINT ( 'NONE',  ( -27.16883889988624290, 60.92500000273118133, -19.73931689729374028 ) ) ;
#13288=( BOUNDED_CURVE ( )  B_SPLINE_CURVE ( 2, ( #17908, #2273, #22698, #12747, #32973, #12401, #23044, #18074, #22871, #17386, #28523, #5018, #10006 ),
 .UNSPECIFIED., .F., .T. ) 
 B_SPLINE_CURVE_WITH_KNOTS ( ( 3, 2, 2, 2, 2, 2, 3 ),
 ( 0.3611111111111111049, 0.3666666666666666408, 0.3777777777777777679, 0.3888888888888888951, 0.4000000000000000222, 0.4111111111111110938, 0.4166666666666666852 ),
 .UNSPECIFIED. ) 
 CURVE ( )  GEOMETRIC_REPRESENTATION_ITEM ( )  RATIONAL_B_SPLINE_CURVE ( ( 0.9755282581475768211, 0.9755282581475768211, 1.000000000000000000, 0.9510565162951535312, 1.000000000000000000, 0.9510565162951535312, 1.000000000000000000, 0.9510565162951535312, 1.000000000000000000, 0.9510565162951535312, 1.000000000000000000, 0.9755282581475765991, 0.9755282581475767101 ) ) 
 REPRESENTATION_ITEM ( '' )  );
#13290=CARTESIAN_POINT ( 'NONE',  ( 18.94512977948576093, 9.324999997268824004, -13.76444248337722875 ) ) ;
#13291=CARTESIAN_POINT ( 'NONE',  ( 33.58253175000000113, 2.125000002731192161, -4.112674001490185761E-15 ) ) ;
#13292=( BOUNDED_CURVE ( )  B_SPLINE_CURVE ( 2, ( #28914, #20875, #4901, #15556, #20537, #30981, #28748, #31323, #7481, #2502, #15382, #5415, #23610 ),
 .UNSPECIFIED., .F., .F. ) 
 B_SPLINE_CURVE_WITH_KNOTS ( ( 3, 2, 2, 2, 2, 2, 3 ),
 ( 0.1500000000000000222, 0.1600000000000000033, 0.1799999999999999933, 0.2000000000000000111, 0.2200000000000000011, 0.2399999999999999911, 0.2500000000000000000 ),
 .UNSPECIFIED. ) 
 CURVE ( )  GEOMETRIC_REPRESENTATION_ITEM ( )  RATIONAL_B_SPLINE_CURVE ( ( 0.9755282581475768211, 0.9755282581475768211, 1.000000000000000000, 0.9510565162951535312, 1.000000000000000000, 0.9510565162951535312, 1.000000000000000000, 0.9510565162951535312, 1.000000000000000000, 0.9510565162951535312, 1.000000000000000000, 0.9755282581475768211, 0.9755282581475768211 ) ) 
 REPRESENTATION_ITEM ( '' )  );
#13293=CARTESIAN_POINT ( 'NONE',  ( -10.37757302488623701, 29.77500000273120051, 31.93888565452638417 ) ) ;
#13294=CARTESIAN_POINT ( 'NONE',  ( 20.08610463437157279, 5.800000005462378816, -27.64615127144129758 ) ) ;
#13296=DIRECTION ( 'NONE',  ( 0.000000000000000000, 0.000000000000000000, -1.000000000000000000 ) ) ;
#13297=CARTESIAN_POINT ( 'NONE',  ( -32.50000000000000000, 32.10000000000000142, 10.55989012756946366 ) ) ;
#13302=CARTESIAN_POINT ( 'NONE',  ( 15.00000000000000355, 71.15000000546237402, 4.873795443493592394 ) ) ;
#13304=CARTESIAN_POINT ( 'NONE',  ( 20.75514604977249178, 21.82500000273119056, 28.56700777964553950 ) ) ;
#13307=CARTESIAN_POINT ( 'NONE',  ( 20.75514604977248467, 18.67500000273120264, -28.56700777964554305 ) ) ;
#13311=CARTESIAN_POINT ( 'NONE',  ( -27.16883889988624290, 68.92500000273119554, -19.73931689729374028 ) ) ;
#13312=CARTESIAN_POINT ( 'NONE',  ( -20.08610463437157989, 26.20000000546237828, -27.64615127144129758 ) ) ;
#13316=CARTESIAN_POINT ( 'NONE',  ( -33.58253175000000113, 57.22500000273117848, 10.91162601494193929 ) ) ;
#13319=ORIENTED_EDGE ( 'NONE', *, *, #33695, .T. ) ;
#13322=CARTESIAN_POINT ( 'NONE',  ( -14.47279130897152122, 16.42499999726882365, 19.92008829642072243 ) ) ;
#13324=ORIENTED_EDGE ( 'NONE', *, *, #2724, .F. ) ;
#13327=ORIENTED_EDGE ( 'NONE', *, *, #5171, .T. ) ;
#13331=DIRECTION ( 'NONE',  ( -0.000000000000000000, 1.000000000000000000, -0.000000000000000000 ) ) ;
#13333=CARTESIAN_POINT ( 'NONE',  ( -4.523095164977116484E-15, 16.12499999726880873, 24.62258325217400312 ) ) ;
#13334=CARTESIAN_POINT ( 'NONE',  ( 33.58253175000000113, 8.375000002731169957, -4.112674001490185761E-15 ) ) ;
#13335=AXIS2_PLACEMENT_3D ( 'NONE', #9927, #20403, #7346 ) ;
#13336=CARTESIAN_POINT ( 'NONE',  ( -26.29305231718578995, 58.20000000000000284, 19.10302069950538595 ) ) ;
#13337=CARTESIAN_POINT ( 'NONE',  ( 4.300734207923761154, 77.47500000273119269, 13.23629886949340495 ) ) ;
#13338=CARTESIAN_POINT ( 'NONE',  ( 20.08610463437158344, 73.20000000546238539, 27.64615127144129403 ) ) ;
#13340=CARTESIAN_POINT ( 'NONE',  ( 4.300734207923761154, 77.97500000273119269, 13.23629886949340495 ) ) ;
#13342=VECTOR ( 'NONE', #4671, 1000.000000000000000 ) ;
#13343=DIRECTION ( 'NONE',  ( -0.000000000000000000, 1.000000000000000000, -0.000000000000000000 ) ) ;
#13344=CARTESIAN_POINT ( 'NONE',  ( 32.50000000000000000, 65.00000000000000000, -3.980102097228898626E-15 ) ) ;
#13345=CARTESIAN_POINT ( 'NONE',  ( -32.50000000000000000, 4.000000000000003553, 0.000000000000000000 ) ) ;
#13347=CARTESIAN_POINT ( 'NONE',  ( 20.75514604977249178, 41.82500000273119412, 28.56700777964553950 ) ) ;
#13350=CARTESIAN_POINT ( 'NONE',  ( -10.37757302488624411, 36.97500000273118559, -31.93888565452638417 ) ) ;
#13351=FACE_OUTER_BOUND ( 'NONE', #32150, .T. ) ;
#13353=CARTESIAN_POINT ( 'NONE',  ( 26.29305231718578995, 15.70000000546237295, -19.10302069950538240 ) ) ;
#13358=EDGE_CURVE ( 'NONE', #4493, #4016, #31327, .T. ) ;
#13362=CARTESIAN_POINT ( 'NONE',  ( -3.880418787951118276, 10.30125427608447097, -24.50000000000000355 ) ) ;
#13363=CARTESIAN_POINT ( 'NONE',  ( -20.75514604977248112, 27.42500000273118488, 28.56700777964554661 ) ) ;
#13366=EDGE_CURVE ( 'NONE', #29691, #5024, #2238, .T. ) ;
#13370=VERTEX_POINT ( 'NONE', #26266 ) ;
#13376=CARTESIAN_POINT ( 'NONE',  ( 27.16883889988623935, 26.57500000273119056, -19.73931689729374384 ) ) ;
#13377=CARTESIAN_POINT ( 'NONE',  ( 32.50000000000000000, 35.60000000546236976, -10.55989012756945833 ) ) ;
#13378=CARTESIAN_POINT ( 'NONE',  ( -10.04305231718578462, 76.39999999999999147, 30.90933677959249337 ) ) ;
#13379=CARTESIAN_POINT ( 'NONE',  ( -20.08610463437157989, 54.20000000546236407, -27.64615127144129758 ) ) ;
#13380=CARTESIAN_POINT ( 'NONE',  ( 10.04305231718579705, 76.59999999999999432, 30.90933677959248982 ) ) ;
#13381=CARTESIAN_POINT ( 'NONE',  ( 27.16883889988624290, 40.17500000273119554, 19.73931689729373673 ) ) ;
#13383=CARTESIAN_POINT ( 'NONE',  ( 26.29305231718579350, 22.79999999999998650, 19.10302069950537529 ) ) ;
#13385=CARTESIAN_POINT ( 'NONE',  ( 33.58253175000000823, 70.02500000273121827, 10.91162601494192863 ) ) ;
#13389=CARTESIAN_POINT ( 'NONE',  ( -33.58253175000000113, 53.47500000273117848, 10.91162601494193929 ) ) ;
#13390=CARTESIAN_POINT ( 'NONE',  ( 26.29305231718578995, 39.70000000546236407, -19.10302069950538240 ) ) ;
#13391=CARTESIAN_POINT ( 'NONE',  ( -33.58253175000000113, 9.225000002731178483, 10.91162601494193929 ) ) ;
#13406=CARTESIAN_POINT ( 'NONE',  ( 26.29305231718579350, 69.30000000546237970, 19.10302069950537529 ) ) ;
#13415=CARTESIAN_POINT ( 'NONE',  ( 2.445080149700053643E-15, 72.50000000000001421, 15.00000000000000000 ) ) ;
#13416=CARTESIAN_POINT ( 'NONE',  ( 10.37757302488624767, 51.97500000273119980, 31.93888565452638417 ) ) ;
#13417=CARTESIAN_POINT ( 'NONE',  ( 20.08610463437157279, 55.80000000546236549, -27.64615127144129758 ) ) ;
#13419=CARTESIAN_POINT ( 'NONE',  ( 0.000000000000000000, 80.00000000000001421, -32.50000000000000000 ) ) ;
#13420=CARTESIAN_POINT ( 'NONE',  ( 6.486482029760649416E-15, 37.62500000273118417, 35.31076352940723240 ) ) ;
#13422=CARTESIAN_POINT ( 'NONE',  ( 10.37757302488624056, 66.77500000273117564, -31.93888565452638417 ) ) ;
#13425=CARTESIAN_POINT ( 'NONE',  ( 26.29305231718578995, 43.20000000000001705, -19.10302069950538240 ) ) ;
#13427=CARTESIAN_POINT ( 'NONE',  ( 10.37757302488624767, 9.975000002731187365, 31.93888565452638417 ) ) ;
#13430=CARTESIAN_POINT ( 'NONE',  ( 13.91746824999999887, 74.37500000273116996, -1.704398294459741270E-15 ) ) ;
#13431=CARTESIAN_POINT ( 'NONE',  ( 27.16883889988624290, 76.17500000273119554, 19.73931689729373673 ) ) ;
#13434=ORIENTED_EDGE ( 'NONE', *, *, #21544, .F. ) ;
#13435=( BOUNDED_CURVE ( )  B_SPLINE_CURVE ( 2, ( #11708, #6229, #5903, #1060, #11541, #22023, #19281, #16541, #13961, #16380, #11383, #24268, #3655 ),
 .UNSPECIFIED., .F., .T. ) 
 B_SPLINE_CURVE_WITH_KNOTS ( ( 3, 2, 2, 2, 2, 2, 3 ),
 ( 0.7500000000000000000, 0.7555555555555555358, 0.7666666666666667185, 0.7777777777777777901, 0.7888888888888888618, 0.8000000000000000444, 0.8055555555555555802 ),
 .UNSPECIFIED. ) 
 CURVE ( )  GEOMETRIC_REPRESENTATION_ITEM ( )  RATIONAL_B_SPLINE_CURVE ( ( 0.9755282581475768211, 0.9755282581475768211, 1.000000000000000000, 0.9510565162951535312, 1.000000000000000000, 0.9510565162951535312, 1.000000000000000000, 0.9510565162951535312, 1.000000000000000000, 0.9510565162951535312, 1.000000000000000000, 0.9755282581475768211, 0.9755282581475768211 ) ) 
 REPRESENTATION_ITEM ( '' )  );
#13447=CARTESIAN_POINT ( 'NONE',  ( -33.58253175000000113, 37.22500000273119980, 10.91162601494193929 ) ) ;
#13450=CARTESIAN_POINT ( 'NONE',  ( -4.405589869732278832E-13, 9.000000005462366559, 32.50000000000000000 ) ) ;
#13451=ORIENTED_EDGE ( 'NONE', *, *, #14403, .T. ) ;
#13456=CARTESIAN_POINT ( 'NONE',  ( -10.37757302488624411, 70.97500000273119269, -31.93888565452638417 ) ) ;
#13463=DIRECTION ( 'NONE',  ( 0.000000000000000000, -1.000000000000000000, 0.000000000000000000 ) ) ;
#13464=CARTESIAN_POINT ( 'NONE',  ( -10.37757302488623701, 63.52500000273120406, 31.93888565452638417 ) ) ;
#13466=ADVANCED_FACE ( 'NONE', ( #23185 ), #7901, .T. ) ;
#13467=CARTESIAN_POINT ( 'NONE',  ( 32.50000000000000000, 19.50000000546236834, -3.980102097228898626E-15 ) ) ;
#13468=CARTESIAN_POINT ( 'NONE',  ( 19.82091636218621034, 17.80000000000001137, 14.40073868116559730 ) ) ;
#13469=CARTESIAN_POINT ( 'NONE',  ( -4.523095164977117273E-15, 8.624999997268810503, 24.62258325217400312 ) ) ;
#13470=CARTESIAN_POINT ( 'NONE',  ( -20.75514604977248823, 4.825000002731171023, -28.56700777964554305 ) ) ;
#13471=CARTESIAN_POINT ( 'NONE',  ( 10.37757302488624056, 28.77500000273120051, -31.93888565452638417 ) ) ;
#13472=LINE ( 'NONE', #572, #26951 ) ;
#13474=CARTESIAN_POINT ( 'NONE',  ( 2.667360163309149608E-15, 78.00000000546238255, -32.50000000000000000 ) ) ;
#13475=CARTESIAN_POINT ( 'NONE',  ( -8.601468415847515203, 79.17500000273120975, 11.83890561707634959 ) ) ;
#13476=CARTESIAN_POINT ( 'NONE',  ( 26.29305231718578995, 75.70000000546239960, -19.10302069950538240 ) ) ;
#13480=CARTESIAN_POINT ( 'NONE',  ( -13.91746824999999532, 72.97500000273117848, 4.522059556121122093 ) ) ;
#13482=CARTESIAN_POINT ( 'NONE',  ( -33.58253175000000113, 27.12500000273118772, 0.000000000000000000 ) ) ;
#13485=CARTESIAN_POINT ( 'NONE',  ( -33.58253175000000113, 17.47500000273118204, 10.91162601494193929 ) ) ;
#13487=CARTESIAN_POINT ( 'NONE',  ( 6.486482029760648627E-15, 69.62500000273118417, 35.31076352940722529 ) ) ;
#13488=CARTESIAN_POINT ( 'NONE',  ( 20.08610463437157279, 3.800000005462383257, -27.64615127144129758 ) ) ;
#13491=CARTESIAN_POINT ( 'NONE',  ( 27.16883889988624290, 59.92500000273118133, 19.73931689729373673 ) ) ;
#13493=ORIENTED_EDGE ( 'NONE', *, *, #33800, .T. ) ;
#13495=CARTESIAN_POINT ( 'NONE',  ( 6.486482029760648627E-15, 1.625000002731185944, 35.31076352940722529 ) ) ;
#13497=CARTESIAN_POINT ( 'NONE',  ( 18.94512977948576093, 0.8249999972688160099, -13.76444248337722875 ) ) ;
#13499=( BOUNDED_CURVE ( )  B_SPLINE_CURVE ( 2, ( #5148, #21451, #23686, #26594, #15458, #151, #16140, #2583, #25914, #3091, #10307, #31894, #20785 ),
 .UNSPECIFIED., .F., .T. ) 
 B_SPLINE_CURVE_WITH_KNOTS ( ( 3, 2, 2, 2, 2, 2, 3 ),
 ( 0.01923076923076923184, 0.02051282051282051280, 0.02307692307692307820, 0.02564102564102564014, 0.02820512820512820554, 0.03076923076923077094, 0.03205128205128205537 ),
 .UNSPECIFIED. ) 
 CURVE ( )  GEOMETRIC_REPRESENTATION_ITEM ( )  RATIONAL_B_SPLINE_CURVE ( ( 0.9755282581475768211, 0.9755282581475768211, 1.000000000000000000, 0.9510565162951535312, 1.000000000000000000, 0.9510565162951535312, 1.000000000000000000, 0.9510565162951535312, 1.000000000000000000, 0.9510565162951535312, 1.000000000000000000, 0.9755282581475767101, 0.9755282581475768211 ) ) 
 REPRESENTATION_ITEM ( '' )  );
#13506=CARTESIAN_POINT ( 'NONE',  ( 5.779280353836490358E-15, 4.500000000000003553, 32.49999999999999289 ) ) ;
#13508=CARTESIAN_POINT ( 'NONE',  ( 32.50000000000000000, 27.50000000546237544, -3.980102097228898626E-15 ) ) ;
#13510=CARTESIAN_POINT ( 'NONE',  ( -23.41746825000000598, 17.72499999726881725, 7.608796670333726198 ) ) ;
#13511=CARTESIAN_POINT ( 'NONE',  ( -27.16883889988623935, 7.575000002731202997, 19.73931689729374739 ) ) ;
#13512=CARTESIAN_POINT ( 'NONE',  ( -26.29305231718579350, 61.79999999999999716, -19.10302069950537884 ) ) ;
#13513=CARTESIAN_POINT ( 'NONE',  ( -11.25946833292375793, 78.67500000273119554, -8.180482586598733619 ) ) ;
#13514=LINE ( 'NONE', #448, #15408 ) ;
#13516=CARTESIAN_POINT ( 'NONE',  ( 13.91746824999999887, 78.37500000273116996, -1.704398294459741270E-15 ) ) ;
#13519=CARTESIAN_POINT ( 'NONE',  ( 20.08610463437157279, 65.29999999999999716, -27.64615127144129758 ) ) ;
#13520=CARTESIAN_POINT ( 'NONE',  ( -20.08610463437156923, 2.299999999999985612, 27.64615127144130113 ) ) ;
#13521=CARTESIAN_POINT ( 'NONE',  ( 5.147494310547426899, 17.94874572391552547, -32.50000000000000000 ) ) ;
#13523=CARTESIAN_POINT ( 'NONE',  ( -27.16883889988624290, 44.92500000273119554, -19.73931689729374028 ) ) ;
#13526=CARTESIAN_POINT ( 'NONE',  ( -27.16883889988624290, 33.17500000273118843, -19.73931689729374028 ) ) ;
#13531=CARTESIAN_POINT ( 'NONE',  ( -1.778240108872766143E-15, 44.00000000546238255, -32.49999999999999289 ) ) ;
#13534=CARTESIAN_POINT ( 'NONE',  ( -14.47279130897152299, 3.924999997268813878, 19.92008829642072243 ) ) ;
#13535=CARTESIAN_POINT ( 'NONE',  ( 3.445340210940985210E-14, 9.249999994537636994, 24.50000000000000000 ) ) ;
#13538=CARTESIAN_POINT ( 'NONE',  ( -33.58253175000000113, 19.12500000273118062, 0.000000000000000000 ) ) ;
#13540=ORIENTED_EDGE ( 'NONE', *, *, #9492, .T. ) ;
#13546=ORIENTED_EDGE ( 'NONE', *, *, #18413, .F. ) ;
#13547=DIRECTION ( 'NONE',  ( -0.000000000000000000, -1.000000000000000000, -0.000000000000000000 ) ) ;
#13549=CARTESIAN_POINT ( 'NONE',  ( -33.58253175000000113, 31.37500000273119127, 0.000000000000000000 ) ) ;
#13550=CARTESIAN_POINT ( 'NONE',  ( 26.29305231718579350, 35.30000000546237970, 19.10302069950537529 ) ) ;
#13552=CARTESIAN_POINT ( 'NONE',  ( 32.50000000000000000, 33.60000000546236976, -10.55989012756945833 ) ) ;
#13553=CARTESIAN_POINT ( 'NONE',  ( 2.445080149700053643E-15, 72.50000000000001421, 15.00000000000000000 ) ) ;
#13554=CARTESIAN_POINT ( 'NONE',  ( -20.75514604977248112, 43.67500000273119554, 28.56700777964554661 ) ) ;
#13559=CARTESIAN_POINT ( 'NONE',  ( -26.29305231718579350, 19.79999999999998295, -19.10302069950537884 ) ) ;
#13561=CARTESIAN_POINT ( 'NONE',  ( 20.75514604977249178, 61.82500000273116569, 28.56700777964553950 ) ) ;
#13564=CARTESIAN_POINT ( 'NONE',  ( -10.37757302488624411, 50.97500000273119980, -31.93888565452638417 ) ) ;
#13566=EDGE_CURVE ( 'NONE', #27363, #3936, #32244, .T. ) ;
#13567=CARTESIAN_POINT ( 'NONE',  ( 20.75514604977248467, 6.425000002731179549, -28.56700777964554305 ) ) ;
#13572=CARTESIAN_POINT ( 'NONE',  ( 2.445080149700053643E-15, 70.75000000546236834, 15.00000000000000000 ) ) ;
#13573=CARTESIAN_POINT ( 'NONE',  ( -5.147494310547423346, 58.94874572391553613, 32.50000000000000000 ) ) ;
#13582=CARTESIAN_POINT ( 'NONE',  ( -26.29305231718578995, 66.70000000546238539, 19.10302069950538595 ) ) ;
#13589=CARTESIAN_POINT ( 'NONE',  ( 33.58253175000000113, 48.37500000273120548, -4.112674001490185761E-15 ) ) ;
#13590=CARTESIAN_POINT ( 'NONE',  ( 26.29305231718579350, 59.30000000546237260, 19.10302069950537529 ) ) ;
#13592=CARTESIAN_POINT ( 'NONE',  ( 33.58253175000000113, 34.22500000273117848, -10.91162601494193751 ) ) ;
#13593=CARTESIAN_POINT ( 'NONE',  ( 15.00000000000000000, 73.35000000546237686, -4.873795443493596835 ) ) ;
#13594=CARTESIAN_POINT ( 'NONE',  ( -20.75514604977248112, 61.67500000273117422, 28.56700777964554661 ) ) ;
#13598=CARTESIAN_POINT ( 'NONE',  ( 10.04305231718578817, 41.39999999999999147, -30.90933677959249337 ) ) ;
#13601=CARTESIAN_POINT ( 'NONE',  ( -27.16883889988624290, 5.175000002731189319, -19.73931689729374028 ) ) ;
#13602=CARTESIAN_POINT ( 'NONE',  ( 32.50000000000000000, 35.50000000546238255, -3.980102097228898626E-15 ) ) ;
#13603=CARTESIAN_POINT ( 'NONE',  ( 8.601468415847520532, 72.07500000273120122, 11.83890561707634781 ) ) ;
#13604=CARTESIAN_POINT ( 'NONE',  ( -33.58253175000000113, 71.47500000273120691, 10.91162601494193929 ) ) ;
#13605=DIRECTION ( 'NONE',  ( 0.000000000000000000, 0.000000000000000000, -1.000000000000000000 ) ) ;
#13619=CARTESIAN_POINT ( 'NONE',  ( -2.162160676586882350E-15, 40.62500000273120548, -35.31076352940722529 ) ) ;
#13622=FACE_OUTER_BOUND ( 'NONE', #6742, .T. ) ;
#13623=ORIENTED_EDGE ( 'NONE', *, *, #8918, .T. ) ;
#13625=CARTESIAN_POINT ( 'NONE',  ( -26.29305231718579350, 50.30000000546236549, -19.10302069950537884 ) ) ;
#13628=CARTESIAN_POINT ( 'NONE',  ( 27.16883889988623935, 72.57500000273120122, -19.73931689729374384 ) ) ;
#13629=EDGE_LOOP ( 'NONE', ( #17159, #17849, #27786, #18779 ) ) ;
#13632=ORIENTED_EDGE ( 'NONE', *, *, #29589, .T. ) ;
#13633=CARTESIAN_POINT ( 'NONE',  ( 0.000000000000000000, 80.00000000000001421, 0.000000000000000000 ) ) ;
#13634=CARTESIAN_POINT ( 'NONE',  ( -2.162160676586881955E-15, 54.62500000273116996, -35.31076352940723240 ) ) ;
#13636=CARTESIAN_POINT ( 'NONE',  ( -32.50000000000000000, 20.40000000546238113, -10.55989012756945478 ) ) ;
#13638=CARTESIAN_POINT ( 'NONE',  ( -23.41746824999999887, 6.024999997268805529, -7.608796670333730638 ) ) ;
#13639=CARTESIAN_POINT ( 'NONE',  ( -33.58253175000000113, 27.37500000273118772, 0.000000000000000000 ) ) ;
#13640=CARTESIAN_POINT ( 'NONE',  ( -12.13525491562421088, 78.05000000546239391, -8.816778784387096835 ) ) ;
#13642=CARTESIAN_POINT ( 'NONE',  ( -8.601468415847518756, 80.57500000273118701, -11.83890561707634781 ) ) ;
#13643=CARTESIAN_POINT ( 'NONE',  ( -32.50000000000000000, 3.899999999999992806, -10.55989012756945300 ) ) ;
#13647=CARTESIAN_POINT ( 'NONE',  ( 13.91746824999999532, 75.97500000273119269, -4.522059556121118540 ) ) ;
#13649=CARTESIAN_POINT ( 'NONE',  ( -33.58253175000000113, 25.22500000273119625, 10.91162601494193929 ) ) ;
#13652=CARTESIAN_POINT ( 'NONE',  ( -27.16883889988623935, 17.57500000273118346, 19.73931689729374739 ) ) ;
#13654=CARTESIAN_POINT ( 'NONE',  ( 20.75514604977249178, 67.82500000273118701, 28.56700777964553950 ) ) ;
#13655=CARTESIAN_POINT ( 'NONE',  ( 0.000000000000000000, 80.00000000000001421, 0.000000000000000000 ) ) ;
#13656=EDGE_CURVE ( 'NONE', #14202, #6637, #32407, .T. ) ;
#13659=CARTESIAN_POINT ( 'NONE',  ( -20.75514604977248112, 59.42500000273118843, 28.56700777964554661 ) ) ;
#13662=ORIENTED_EDGE ( 'NONE', *, *, #27334, .T. ) ;
#13665=CARTESIAN_POINT ( 'NONE',  ( -4.523095164977116484E-15, 6.124999997268802510, 24.62258325217400312 ) ) ;
#13667=ORIENTED_EDGE ( 'NONE', *, *, #4651, .F. ) ;
#13669=CARTESIAN_POINT ( 'NONE',  ( -32.50000000000000000, 42.40000000546238823, -10.55989012756945300 ) ) ;
#13670=ORIENTED_EDGE ( 'NONE', *, *, #25723, .T. ) ;
#13674=CARTESIAN_POINT ( 'NONE',  ( 27.16883889988623935, 74.32500000273117280, -19.73931689729374384 ) ) ;
#13676=CARTESIAN_POINT ( 'NONE',  ( 7.570916362186207671, 1.599999999999990319, 23.30088464923126779 ) ) ;
#13677=CARTESIAN_POINT ( 'NONE',  ( 27.16883889988624290, 12.17500000273119554, 19.73931689729373673 ) ) ;
#13678=CARTESIAN_POINT ( 'NONE',  ( 20.75514604977248467, 20.42500000273120619, -28.56700777964554305 ) ) ;
#13679=CARTESIAN_POINT ( 'NONE',  ( 10.04305231718579705, 57.10000000546239107, 30.90933677959248982 ) ) ;
#13682=CARTESIAN_POINT ( 'NONE',  ( -4.300734207923755825, 73.77500000273118985, 13.23629886949340673 ) ) ;
#13685=CARTESIAN_POINT ( 'NONE',  ( 32.50000000000000000, 49.60000000546239107, -10.55989012756945833 ) ) ;
#13687=CARTESIAN_POINT ( 'NONE',  ( -27.16883889988623935, 41.32500000273120122, 19.73931689729374739 ) ) ;
#13690=CARTESIAN_POINT ( 'NONE',  ( 20.75514604977248467, 34.67500000273118843, -28.56700777964554305 ) ) ;
#13693=CARTESIAN_POINT ( 'NONE',  ( -1.778240108872766143E-15, 11.49999999999999112, -32.49999999999999289 ) ) ;
#13694=CARTESIAN_POINT ( 'NONE',  ( 26.29305231718579350, 30.79999999999999361, 19.10302069950537529 ) ) ;
#13697=CARTESIAN_POINT ( 'NONE',  ( -23.41746824999999887, 1.524999997268801755, -7.608796670333730638 ) ) ;
#13698=( BOUNDED_CURVE ( )  B_SPLINE_CURVE ( 2, ( #720, #9119, #24738, #11368, #16364, #26819, #14448, #32289, #21678, #8621, #19103, #29541, #29883 ),
 .UNSPECIFIED., .F., .T. ) 
 B_SPLINE_CURVE_WITH_KNOTS ( ( 3, 2, 2, 2, 2, 2, 3 ),
 ( 0.8269230769230769829, 0.8282051282051282604, 0.8307692307692308153, 0.8333333333333333703, 0.8358974358974359253, 0.8384615384615384803, 0.8397435897435897578 ),
 .UNSPECIFIED. ) 
 CURVE ( )  GEOMETRIC_REPRESENTATION_ITEM ( )  RATIONAL_B_SPLINE_CURVE ( ( 0.9755282581475768211, 0.9755282581475778203, 1.000000000000000000, 0.9510565162951535312, 1.000000000000000000, 0.9510565162951535312, 1.000000000000000000, 0.9510565162951535312, 1.000000000000000000, 0.9510565162951535312, 1.000000000000000000, 0.9755282581475768211, 0.9755282581475768211 ) ) 
 REPRESENTATION_ITEM ( '' )  );
#13699=CARTESIAN_POINT ( 'NONE',  ( -1.778240108872766143E-15, 52.00000000546237544, -32.49999999999999289 ) ) ;
#13701=CARTESIAN_POINT ( 'NONE',  ( 27.16883889988623935, 22.32500000273118701, -19.73931689729374384 ) ) ;
#13709=ORIENTED_EDGE ( 'NONE', *, *, #17076, .F. ) ;
#13710=LINE ( 'NONE', #21106, #19063 ) ;
#13711=CARTESIAN_POINT ( 'NONE',  ( 20.75514604977249178, 30.07500000273118701, 28.56700777964553950 ) ) ;
#13712=CARTESIAN_POINT ( 'NONE',  ( -32.50000000000000000, 30.50000000546237899, 0.000000000000000000 ) ) ;
#13713=CARTESIAN_POINT ( 'NONE',  ( -26.29305231718579350, 79.79999999999998295, -19.10302069950537884 ) ) ;
#13714=CARTESIAN_POINT ( 'NONE',  ( 32.50000000000000000, 52.99999999999999289, -3.980102097228898626E-15 ) ) ;
#13715=CARTESIAN_POINT ( 'NONE',  ( 9.270509831248421762, 73.29999999999996874, -12.75976212528059861 ) ) ;
#13716=CARTESIAN_POINT ( 'NONE',  ( -10.37757302488623701, 43.77500000273118275, 31.93888565452638417 ) ) ;
#13717=CARTESIAN_POINT ( 'NONE',  ( 26.29305231718578995, 61.20000000000000284, -19.10302069950538240 ) ) ;
#13720=CARTESIAN_POINT ( 'NONE',  ( -32.50000000000000000, 22.09999999999999787, 10.55989012756946366 ) ) ;
#13722=CARTESIAN_POINT ( 'NONE',  ( 33.58253175000000823, 60.02500000273116854, 10.91162601494192863 ) ) ;
#13724=CARTESIAN_POINT ( 'NONE',  ( -10.37757302488624411, 54.97500000273119980, -31.93888565452638417 ) ) ;
#13727=CARTESIAN_POINT ( 'NONE',  ( -10.37757302488623701, 7.525000002731207616, 31.93888565452638417 ) ) ;
#13731=CARTESIAN_POINT ( 'NONE',  ( -10.04305231718578462, 18.90000000546238113, 30.90933677959249337 ) ) ;
#13736=( NAMED_UNIT ( * ) SI_UNIT ( $, .STERADIAN. ) SOLID_ANGLE_UNIT ( ) );
#13738=EDGE_LOOP ( 'NONE', ( #5261, #28047, #31609, #5848 ) ) ;
#13742=ORIENTED_EDGE ( 'NONE', *, *, #16488, .T. ) ;
#13747=CARTESIAN_POINT ( 'NONE',  ( 20.75514604977249178, 50.07500000273120122, 28.56700777964553950 ) ) ;
#13748=CARTESIAN_POINT ( 'NONE',  ( 10.04305231718579705, 49.10000000546238397, 30.90933677959248982 ) ) ;
#13751=CARTESIAN_POINT ( 'NONE',  ( -2.162160676586881955E-15, 32.62500000273119838, -35.31076352940723240 ) ) ;
#13753=CARTESIAN_POINT ( 'NONE',  ( 20.75514604977249178, 64.07500000273120122, 28.56700777964553950 ) ) ;
#13755=CARTESIAN_POINT ( 'NONE',  ( -20.08610463437157989, 37.70000000000000995, -27.64615127144129758 ) ) ;
#13757=CARTESIAN_POINT ( 'NONE',  ( 10.37757302488624056, 6.775000002731179194, -31.93888565452638417 ) ) ;
#13758=CARTESIAN_POINT ( 'NONE',  ( -32.50000000000000000, 70.60000000546236265, 10.55989012756946366 ) ) ;
#13759=AXIS2_PLACEMENT_3D ( 'NONE', #14008, #22356, #24922 ) ;
#13760=CARTESIAN_POINT ( 'NONE',  ( -8.960552108402742093E-16, 74.87500000273116996, -14.63369212191046387 ) ) ;
#13761=CARTESIAN_POINT ( 'NONE',  ( 33.58253175000000113, 70.47500000273119269, -10.91162601494193574 ) ) ;
#13762=CARTESIAN_POINT ( 'NONE',  ( 0.000000000000000000, 80.00000000000001421, 0.000000000000000000 ) ) ;
#13764=EDGE_LOOP ( 'NONE', ( #3400, #7625, #24337, #26406 ) ) ;
#13765=DIRECTION ( 'NONE',  ( -0.000000000000000000, -1.000000000000000000, -0.000000000000000000 ) ) ;
#13776=EDGE_CURVE ( 'NONE', #6044, #33570, #33528, .T. ) ;
#13778=CARTESIAN_POINT ( 'NONE',  ( 33.58253175000000823, 42.02500000273118985, 10.91162601494192685 ) ) ;
#13781=CARTESIAN_POINT ( 'NONE',  ( 5.147494310547426899, 59.44874571845315359, -32.50000000000000000 ) ) ;
#13784=CARTESIAN_POINT ( 'NONE',  ( 0.000000000000000000, 80.00000000000001421, -32.50000000000000000 ) ) ;
#13785=VECTOR ( 'NONE', #20658, 1000.000000000000000 ) ;
#13787=CARTESIAN_POINT ( 'NONE',  ( -33.58253175000000113, 71.27500000273118985, -10.91162601494193218 ) ) ;
#13788=VERTEX_POINT ( 'NONE', #13572 ) ;
#13793=( BOUNDED_CURVE ( )  B_SPLINE_CURVE ( 2, ( #30797, #33018, #22568, #6781, #33374, #4719, #27722, #1453, #9869, #17259, #4210, #28062, #14682 ),
 .UNSPECIFIED., .F., .T. ) 
 B_SPLINE_CURVE_WITH_KNOTS ( ( 3, 2, 2, 2, 2, 2, 3 ),
 ( 0.7243589743589743390, 0.7256410256410256165, 0.7282051282051281715, 0.7307692307692307265, 0.7333333333333332815, 0.7358974358974359475, 0.7371794871794872250 ),
 .UNSPECIFIED. ) 
 CURVE ( )  GEOMETRIC_REPRESENTATION_ITEM ( )  RATIONAL_B_SPLINE_CURVE ( ( 0.9755282581475768211, 0.9755282581475768211, 1.000000000000000000, 0.9510565162951535312, 1.000000000000000000, 0.9510565162951535312, 1.000000000000000000, 0.9510565162951535312, 1.000000000000000000, 0.9510565162951535312, 1.000000000000000000, 0.9755282581475768211, 0.9755282581475768211 ) ) 
 REPRESENTATION_ITEM ( '' )  );
#13794=ORIENTED_EDGE ( 'NONE', *, *, #2759, .T. ) ;
#13795=CARTESIAN_POINT ( 'NONE',  ( -5.147494310547430452, 48.05125428700922185, -32.49999999999999289 ) ) ;
#13796=CARTESIAN_POINT ( 'NONE',  ( 10.37757302488624056, 56.52500000273119696, -31.93888565452638417 ) ) ;
#13798=CARTESIAN_POINT ( 'NONE',  ( -20.08610463437156923, 20.80000000546236549, 27.64615127144130113 ) ) ;
#13799=CARTESIAN_POINT ( 'NONE',  ( -5.147494310547377161, 66.05125428700922896, -32.50000000000002132 ) ) ;
#13800=CARTESIAN_POINT ( 'NONE',  ( 23.41746824999999887, 11.12499999726881938, 0.000000000000000000 ) ) ;
#13801=CARTESIAN_POINT ( 'NONE',  ( 33.58253175000000113, 22.37500000273118417, -4.112674001490185761E-15 ) ) ;
#13804=CARTESIAN_POINT ( 'NONE',  ( -11.25946833292375793, 79.07500000273121543, 8.180482586598737171 ) ) ;
#13805=CARTESIAN_POINT ( 'NONE',  ( -1.778240108872766143E-15, 28.00000000546237544, -32.49999999999999289 ) ) ;
#13809=CARTESIAN_POINT ( 'NONE',  ( -4.300734207923759378, 78.47500000273119269, -13.23629886949340495 ) ) ;
#13811=CARTESIAN_POINT ( 'NONE',  ( -33.58253175000000113, 23.12500000273118417, 0.000000000000000000 ) ) ;
#13816=CARTESIAN_POINT ( 'NONE',  ( -20.75514604977248112, 13.67500000273118310, 28.56700777964554661 ) ) ;
#13818=CARTESIAN_POINT ( 'NONE',  ( -10.37757302488623701, 69.52500000273120406, 31.93888565452638417 ) ) ;
#13819=DIRECTION ( 'NONE',  ( 0.000000000000000000, 0.000000000000000000, -1.000000000000000000 ) ) ;
#13820=CARTESIAN_POINT ( 'NONE',  ( -11.25946833292375793, 77.57500000273121543, 8.180482586598737171 ) ) ;
#13823=CARTESIAN_POINT ( 'NONE',  ( -33.58253175000000113, 61.22500000273119269, 10.91162601494193929 ) ) ;
#13825=ORIENTED_EDGE ( 'NONE', *, *, #16600, .T. ) ;
#13827=CARTESIAN_POINT ( 'NONE',  ( -33.58253175000000113, 3.025000002731199622, -10.91162601494193041 ) ) ;
#13828=CARTESIAN_POINT ( 'NONE',  ( -18.94512977948575738, 9.424999997268812990, -13.76444248337723231 ) ) ;
#13832=CARTESIAN_POINT ( 'NONE',  ( -32.50000000000000000, 42.60000000546236976, 10.55989012756946366 ) ) ;
#13836=DIRECTION ( 'NONE',  ( 0.000000000000000000, 0.000000000000000000, 1.000000000000000000 ) ) ;
#13837=CARTESIAN_POINT ( 'NONE',  ( -10.37757302488623701, 75.52500000273118985, 31.93888565452638417 ) ) ;
#13839=CARTESIAN_POINT ( 'NONE',  ( -19.82091636218621389, 3.200000000000008171, 14.40073868116558842 ) ) ;
#13840=CARTESIAN_POINT ( 'NONE',  ( 20.75514604977249178, 12.07500000273120655, 28.56700777964553950 ) ) ;
#13841=EDGE_CURVE ( 'NONE', #14813, #24433, #641, .T. ) ;
#13842=CARTESIAN_POINT ( 'NONE',  ( -10.37757302488623701, 13.52500000273118630, 31.93888565452638417 ) ) ;
#13843=CARTESIAN_POINT ( 'NONE',  ( -13.91746824999999532, 78.77500000273117564, -4.522059556121115875 ) ) ;
#13846=CARTESIAN_POINT ( 'NONE',  ( -15.00000000000000000, 77.90000000000001990, -4.873795443493594171 ) ) ;
#13848=EDGE_CURVE ( 'NONE', #390, #1865, #14234, .T. ) ;
#13849=DIRECTION ( 'NONE',  ( 0.000000000000000000, 0.000000000000000000, -1.000000000000000000 ) ) ;
#13850=CARTESIAN_POINT ( 'NONE',  ( -1.778240108872766143E-15, 50.00000000546237544, -32.49999999999999289 ) ) ;
#13852=CARTESIAN_POINT ( 'NONE',  ( 27.16883889988624290, 43.92500000273119554, 19.73931689729373673 ) ) ;
#13855=CARTESIAN_POINT ( 'NONE',  ( 6.486482029760648627E-15, 37.87500000273117706, 35.31076352940722529 ) ) ;
#13857=AXIS2_PLACEMENT_3D ( 'NONE', #21854, #13463, #32136 ) ;
#13860=LINE ( 'NONE', #11604, #10194 ) ;
#13863=CARTESIAN_POINT ( 'NONE',  ( -14.47279130897151767, 5.324999997268798246, -19.92008829642072598 ) ) ;
#13864=CARTESIAN_POINT ( 'NONE',  ( 3.880418787951140036, 12.44874571845315714, -24.49999999999999645 ) ) ;
#13867=CARTESIAN_POINT ( 'NONE',  ( 10.37757302488624767, 21.72500000273119980, 31.93888565452638417 ) ) ;
#13868=CARTESIAN_POINT ( 'NONE',  ( 14.47279130897151767, 5.424999997268823648, -19.92008829642072598 ) ) ;
#13870=ORIENTED_EDGE ( 'NONE', *, *, #1325, .F. ) ;
#13872=EDGE_LOOP ( 'NONE', ( #32606, #3895, #23668, #12040 ) ) ;
#13876=CARTESIAN_POINT ( 'NONE',  ( 26.29305231718578995, 39.20000000000000995, -19.10302069950538240 ) ) ;
#13877=AXIS2_PLACEMENT_3D ( 'NONE', #8842, #19325, #30101 ) ;
#13878=CARTESIAN_POINT ( 'NONE',  ( -23.41746824999999887, 7.624999997268816720, -2.867812753649727150E-15 ) ) ;
#13879=CARTESIAN_POINT ( 'NONE',  ( -10.37757302488623701, 27.77500000273119696, 31.93888565452638417 ) ) ;
#13880=CARTESIAN_POINT ( 'NONE',  ( 10.04305231718578817, 33.90000000546239534, -30.90933677959249337 ) ) ;
#13881=ADVANCED_FACE ( 'NONE', ( #25028 ), #30677, .T. ) ;
#13882=CARTESIAN_POINT ( 'NONE',  ( 10.04305231718579705, 76.59999999999999432, 30.90933677959248982 ) ) ;
#13883=CARTESIAN_POINT ( 'NONE',  ( 10.04305231718578817, 33.90000000546239534, -30.90933677959249337 ) ) ;
#13884=CARTESIAN_POINT ( 'NONE',  ( 2.375766604868046361, 72.55125428154683220, 14.99999999999999822 ) ) ;
#13885=CARTESIAN_POINT ( 'NONE',  ( 33.58253175000000113, 44.47500000273119269, -10.91162601494193751 ) ) ;
#13886=EDGE_CURVE ( 'NONE', #27323, #30686, #12330, .T. ) ;
#13888=CARTESIAN_POINT ( 'NONE',  ( 32.50000000000000711, 22.90000000000000568, 10.55989012756945122 ) ) ;
#13890=CARTESIAN_POINT ( 'NONE',  ( 33.58253175000000113, 66.22500000273120691, -10.91162601494193751 ) ) ;
#13891=CARTESIAN_POINT ( 'NONE',  ( 33.58253175000000823, 56.27500000273117564, 10.91162601494192685 ) ) ;
#13894=CARTESIAN_POINT ( 'NONE',  ( 20.75514604977249178, 3.825000002731174575, 28.56700777964553950 ) ) ;
#13900=CARTESIAN_POINT ( 'NONE',  ( -4.223320258572819786E-15, 15.24999999453762278, 24.50000000000000000 ) ) ;
#13910=FACE_OUTER_BOUND ( 'NONE', #25813, .T. ) ;
#13915=DIRECTION ( 'NONE',  ( 0.000000000000000000, 0.000000000000000000, -1.000000000000000000 ) ) ;
#13916=CARTESIAN_POINT ( 'NONE',  ( 33.58253175000000113, 46.37500000273120548, -4.112674001490185761E-15 ) ) ;
#13917=CARTESIAN_POINT ( 'NONE',  ( 32.50000000000000000, 51.50000000546239676, -3.980102097228898626E-15 ) ) ;
#13919=CARTESIAN_POINT ( 'NONE',  ( 33.58253175000000113, 38.12500000273119838, -4.112674001490185761E-15 ) ) ;
#13921=VECTOR ( 'NONE', #30850, 1000.000000000000000 ) ;
#13922=CARTESIAN_POINT ( 'NONE',  ( -10.37757302488624411, 60.97500000273120691, -31.93888565452638417 ) ) ;
#13924=CARTESIAN_POINT ( 'NONE',  ( -26.29305231718578995, 40.20000000000001705, 19.10302069950538595 ) ) ;
#13926=CARTESIAN_POINT ( 'NONE',  ( 33.58253175000000113, 6.475000002731178483, -10.91162601494193751 ) ) ;
#13927=CARTESIAN_POINT ( 'NONE',  ( 5.147494310547434893, 12.55125428154683753, 32.49999999999999289 ) ) ;
#13928=CARTESIAN_POINT ( 'NONE',  ( -13.91746824999999887, 71.37500000273119838, 0.000000000000000000 ) ) ;
#13929=CARTESIAN_POINT ( 'NONE',  ( 33.58253175000000113, 74.47500000273117848, -10.91162601494193574 ) ) ;
#13930=CARTESIAN_POINT ( 'NONE',  ( -3.880418787951124493, 5.448745718453149145, 24.50000000000000355 ) ) ;
#13932=VERTEX_POINT ( 'NONE', #14908 ) ;
#13933=CARTESIAN_POINT ( 'NONE',  ( 19.82091636218621389, 1.949999994537626735, -14.40073868116559197 ) ) ;
#13935=CARTESIAN_POINT ( 'NONE',  ( -1.778240108872766143E-15, 43.50000000000000000, -32.49999999999999289 ) ) ;
#13948=VERTEX_POINT ( 'NONE', #22130 ) ;
#13952=CARTESIAN_POINT ( 'NONE',  ( 6.486482029760649416E-15, 69.87500000273121259, 35.31076352940723240 ) ) ;
#13953=ORIENTED_EDGE ( 'NONE', *, *, #20502, .F. ) ;
#13956=ORIENTED_EDGE ( 'NONE', *, *, #846, .T. ) ;
#13957=DIRECTION ( 'NONE',  ( 0.000000000000000000, 0.000000000000000000, -1.000000000000000000 ) ) ;
#13958=CARTESIAN_POINT ( 'NONE',  ( -27.16883889988623935, 53.32500000273118701, 19.73931689729374739 ) ) ;
#13960=CARTESIAN_POINT ( 'NONE',  ( -10.04305231718578462, 14.90000000546237757, 30.90933677959249337 ) ) ;
#13961=CARTESIAN_POINT ( 'NONE',  ( 19.82091636218621389, 15.94999999453763984, -14.40073868116559197 ) ) ;
#13962=CARTESIAN_POINT ( 'NONE',  ( 1.507698388325705758E-15, 17.62499999726881938, -24.62258325217400312 ) ) ;
#13964=CARTESIAN_POINT ( 'NONE',  ( 20.75514604977249178, 26.07500000273119767, 28.56700777964553950 ) ) ;
#13966=FACE_OUTER_BOUND ( 'NONE', #7081, .T. ) ;
#13970=VERTEX_POINT ( 'NONE', #25372 ) ;
#13972=CARTESIAN_POINT ( 'NONE',  ( -13.91746824999999532, 74.97500000273115006, 4.522059556121122093 ) ) ;
#13974=CARTESIAN_POINT ( 'NONE',  ( 6.486482029760649416E-15, 25.62500000273118772, 35.31076352940723240 ) ) ;
#13978=CARTESIAN_POINT ( 'NONE',  ( 27.16883889988624290, 8.175000002731191984, 19.73931689729373673 ) ) ;
#13980=ADVANCED_FACE ( 'NONE', ( #1851, #4094 ), #27777, .T. ) ;
#13981=CARTESIAN_POINT ( 'NONE',  ( -2.162160676586882350E-15, 70.62500000273118417, -35.31076352940722529 ) ) ;
#13984=CARTESIAN_POINT ( 'NONE',  ( -13.91746824999999887, 75.37500000273116996, 0.000000000000000000 ) ) ;
#13986=CARTESIAN_POINT ( 'NONE',  ( -2.375766604868041476, 72.69874572391553613, 14.99999999999999822 ) ) ;
#13987=CARTESIAN_POINT ( 'NONE',  ( 10.37757302488624767, 51.72500000273119980, 31.93888565452638417 ) ) ;
#13990=ORIENTED_EDGE ( 'NONE', *, *, #28667, .F. ) ;
#13994=CARTESIAN_POINT ( 'NONE',  ( -23.41746825000000243, 5.524999997268821517, -7.608796670333730638 ) ) ;
#13998=ORIENTED_EDGE ( 'NONE', *, *, #427, .T. ) ;
#14000=CARTESIAN_POINT ( 'NONE',  ( 6.486482029760649416E-15, 61.87500000273117706, 35.31076352940723240 ) ) ;
#14001=CARTESIAN_POINT ( 'NONE',  ( 10.04305231718578817, 69.90000000546237402, -30.90933677959249337 ) ) ;
#14002=CARTESIAN_POINT ( 'NONE',  ( -33.58253175000000113, 71.22500000273117848, 10.91162601494193929 ) ) ;
#14004=CARTESIAN_POINT ( 'NONE',  ( -15.14183272437242600, 9.299999999999998934, 20.84094480462497856 ) ) ;
#14005=CARTESIAN_POINT ( 'NONE',  ( 33.58253175000000113, 6.475000002731178483, -10.91162601494193751 ) ) ;
#14006=CARTESIAN_POINT ( 'NONE',  ( -10.37757302488624411, 18.72500000273119625, -31.93888565452638417 ) ) ;
#14007=CARTESIAN_POINT ( 'NONE',  ( 11.25946833292375793, 73.67500000273119554, 8.180482586598731842 ) ) ;
#14008=CARTESIAN_POINT ( 'NONE',  ( 0.000000000000000000, 82.00000000000001421, 0.000000000000000000 ) ) ;
#14010=CARTESIAN_POINT ( 'NONE',  ( -4.635254915624211769, 77.60000000000000853, -14.26584774442730286 ) ) ;
#14015=CARTESIAN_POINT ( 'NONE',  ( 33.58253175000000113, 46.12500000273117706, -4.112674001490185761E-15 ) ) ;
#14018=CARTESIAN_POINT ( 'NONE',  ( -27.16883889988624290, 27.17500000273118133, -19.73931689729374028 ) ) ;
#14021=CARTESIAN_POINT ( 'NONE',  ( 5.334720326618300005E-14, 73.50000000000001421, -32.50000000000000000 ) ) ;
#14026=CARTESIAN_POINT ( 'NONE',  ( 14.47279130897151944, 6.924999997268805885, -19.92008829642072598 ) ) ;
#14031=CARTESIAN_POINT ( 'NONE',  ( -20.75514604977248112, 17.42500000273117777, 28.56700777964554661 ) ) ;
#14032=CARTESIAN_POINT ( 'NONE',  ( 23.41746825000000243, 5.024999997268808194, 7.608796670333735079 ) ) ;
#14034=ORIENTED_EDGE ( 'NONE', *, *, #16488, .F. ) ;
#14037=ORIENTED_EDGE ( 'NONE', *, *, #30596, .T. ) ;
#14041=CARTESIAN_POINT ( 'NONE',  ( -19.82091636218621034, 16.54999999453762882, -14.40073868116559552 ) ) ;
#14042=CARTESIAN_POINT ( 'NONE',  ( 14.47279130897151767, 4.924999997268811214, -19.92008829642072598 ) ) ;
#14043=CARTESIAN_POINT ( 'NONE',  ( 27.16883889988624290, 26.17500000273118133, 19.73931689729373673 ) ) ;
#14044=CARTESIAN_POINT ( 'NONE',  ( -32.50000000000000000, 30.40000000546238823, -10.55989012756945478 ) ) ;
#14045=AXIS2_PLACEMENT_3D ( 'NONE', #9301, #9480, #19785 ) ;
#14046=CARTESIAN_POINT ( 'NONE',  ( -32.50000000000000000, 69.90000000000000568, -10.55989012756945478 ) ) ;
#14047=CARTESIAN_POINT ( 'NONE',  ( 32.50000000000000711, 52.89999999999999147, 10.55989012756945122 ) ) ;
#14048=CARTESIAN_POINT ( 'NONE',  ( 9.270509831248425314, 72.70000000000000284, 12.75976212528059683 ) ) ;
#14050=CARTESIAN_POINT ( 'NONE',  ( -10.37757302488624411, 44.97500000273119269, -31.93888565452638417 ) ) ;
#14052=CARTESIAN_POINT ( 'NONE',  ( -23.41746825000000598, 12.22499999726881370, 7.608796670333726198 ) ) ;
#14053=CARTESIAN_POINT ( 'NONE',  ( -26.29305231718578995, 14.19999999999999041, 19.10302069950538595 ) ) ;
#14056=CARTESIAN_POINT ( 'NONE',  ( 10.37757302488624056, 64.52500000273120406, -31.93888565452638417 ) ) ;
#14057=CARTESIAN_POINT ( 'NONE',  ( -27.16883889988624290, 49.17500000273117422, -19.73931689729374028 ) ) ;
#14060=CARTESIAN_POINT ( 'NONE',  ( -27.16883889988623935, 3.325000002731171023, 19.73931689729374739 ) ) ;
#14064=UNCERTAINTY_MEASURE_WITH_UNIT (LENGTH_MEASURE( 1.000000000000000082E-05 ), #361, 'distance_accuracy_value', 'NONE');
#14066=DIRECTION ( 'NONE',  ( -0.000000000000000000, -1.000000000000000000, -0.000000000000000000 ) ) ;
#14071=EDGE_CURVE ( 'NONE', #10540, #2121, #30001, .T. ) ;
#14072=CARTESIAN_POINT ( 'NONE',  ( 0.000000000000000000, 80.00000000000001421, 0.000000000000000000 ) ) ;
#14073=CARTESIAN_POINT ( 'NONE',  ( 0.000000000000000000, 82.00000000000001421, 0.000000000000000000 ) ) ;
#14075=ADVANCED_FACE ( 'NONE', ( #9233 ), #1337, .T. ) ;
#14078=CYLINDRICAL_SURFACE ( 'NONE', #18560, 15.00000000000000000 ) ;
#14079=ORIENTED_EDGE ( 'NONE', *, *, #5392, .F. ) ;
#14082=AXIS2_PLACEMENT_3D ( 'NONE', #30347, #30690, #17845 ) ;
#14084=CARTESIAN_POINT ( 'NONE',  ( -20.08610463437156923, 64.80000000546237970, 27.64615127144130113 ) ) ;
#14085=CARTESIAN_POINT ( 'NONE',  ( -33.58253175000000113, 45.47500000273119980, 10.91162601494193929 ) ) ;
#14086=CARTESIAN_POINT ( 'NONE',  ( 6.277390505771533514E-15, 49.00000000546238965, 34.17252228774368916 ) ) ;
#14089=CARTESIAN_POINT ( 'NONE',  ( 27.16883889988623935, 34.32500000273120122, -19.73931689729374384 ) ) ;
#14091=CARTESIAN_POINT ( 'NONE',  ( 10.37757302488624767, 59.97500000273120691, 31.93888565452638417 ) ) ;
#14094=CARTESIAN_POINT ( 'NONE',  ( 10.04305231718578817, 37.39999999999999147, -30.90933677959249337 ) ) ;
#14096=CARTESIAN_POINT ( 'NONE',  ( -20.75514604977248112, 1.675000002731184434, 28.56700777964554661 ) ) ;
#14097=CARTESIAN_POINT ( 'NONE',  ( 32.50000000000000711, 12.90000000000000036, 10.55989012756945122 ) ) ;
#14099=CARTESIAN_POINT ( 'NONE',  ( -10.37757302488624411, 74.97500000273119269, -31.93888565452638417 ) ) ;
#14100=CARTESIAN_POINT ( 'NONE',  ( -24.50000000000000000, 18.64999999453763380, -7.960532557706207157 ) ) ;
#14103=CARTESIAN_POINT ( 'NONE',  ( -4.732186688966233175E-15, 5.249999994537621895, 25.76082449383753925 ) ) ;
#14105=CARTESIAN_POINT ( 'NONE',  ( 9.270509831248421762, 75.30000000000001137, -12.75976212528059861 ) ) ;
#14118=ORIENTED_EDGE ( 'NONE', *, *, #26858, .F. ) ;
#14120=CARTESIAN_POINT ( 'NONE',  ( -10.04305231718578462, 76.39999999999999147, 30.90933677959249337 ) ) ;
#14123=ORIENTED_EDGE ( 'NONE', *, *, #19915, .T. ) ;
#14126=ORIENTED_EDGE ( 'NONE', *, *, #6826, .F. ) ;
#14128=CARTESIAN_POINT ( 'NONE',  ( 20.08610463437158344, 65.20000000546235697, 27.64615127144129403 ) ) ;
#14129=CARTESIAN_POINT ( 'NONE',  ( -33.58253175000000113, 53.02500000273118985, -10.91162601494193218 ) ) ;
#14131=CARTESIAN_POINT ( 'NONE',  ( -20.08610463437156923, 14.80000000546238503, 27.64615127144130113 ) ) ;
#14132=CARTESIAN_POINT ( 'NONE',  ( -26.29305231718579350, 66.30000000546237970, -19.10302069950537884 ) ) ;
#14133=CARTESIAN_POINT ( 'NONE',  ( 23.41746824999999887, 15.02499999726881086, 7.608796670333735079 ) ) ;
#14134=CARTESIAN_POINT ( 'NONE',  ( 20.08610463437157279, 57.29999999999999005, -27.64615127144129758 ) ) ;
#14135=CARTESIAN_POINT ( 'NONE',  ( 33.58253175000000113, 22.47500000273119625, -10.91162601494193751 ) ) ;
#14137=CARTESIAN_POINT ( 'NONE',  ( 4.300734207923757602, 76.27500000273118985, -13.23629886949340673 ) ) ;
#14138=CARTESIAN_POINT ( 'NONE',  ( 15.14183272437242422, 16.30000000000000782, -20.84094480462497856 ) ) ;
#14139=CARTESIAN_POINT ( 'NONE',  ( 10.04305231718578817, 15.39999999999999680, -30.90933677959249337 ) ) ;
#14143=CARTESIAN_POINT ( 'NONE',  ( 4.300734207923757602, 78.27500000273118985, -13.23629886949340673 ) ) ;
#14145=CARTESIAN_POINT ( 'NONE',  ( 10.37757302488624056, 16.52500000273118985, -31.93888565452638417 ) ) ;
#14149=CARTESIAN_POINT ( 'NONE',  ( 10.37757302488624056, 8.775000002731180970, -31.93888565452638417 ) ) ;
#14152=CARTESIAN_POINT ( 'NONE',  ( 13.91746824999999532, 80.47500000273119269, -4.522059556121118540 ) ) ;
#14154=CARTESIAN_POINT ( 'NONE',  ( 26.29305231718578995, 63.20000000000000284, -19.10302069950538240 ) ) ;
#14155=CARTESIAN_POINT ( 'NONE',  ( 27.16883889988624290, 53.92500000273120264, 19.73931689729373673 ) ) ;
#14158=EDGE_LOOP ( 'NONE', ( #16449, #10959, #7249, #306 ) ) ;
#14160=FACE_OUTER_BOUND ( 'NONE', #10919, .T. ) ;
#14161=CARTESIAN_POINT ( 'NONE',  ( -23.41746825000000598, 5.724999997268815477, 7.608796670333726198 ) ) ;
#14163=VERTEX_POINT ( 'NONE', #30336 ) ;
#14165=CARTESIAN_POINT ( 'NONE',  ( 0.000000000000000000, 80.00000000000001421, -32.50000000000000000 ) ) ;
#14166=ORIENTED_EDGE ( 'NONE', *, *, #11970, .F. ) ;
#14168=CARTESIAN_POINT ( 'NONE',  ( 20.75514604977248467, 60.67500000273118133, -28.56700777964554305 ) ) ;
#14170=CARTESIAN_POINT ( 'NONE',  ( -33.58253175000000113, 75.02500000273117564, -10.91162601494193218 ) ) ;
#14172=CARTESIAN_POINT ( 'NONE',  ( -15.14183272437241889, 6.699999999999991296, -20.84094480462497856 ) ) ;
#14173=CARTESIAN_POINT ( 'NONE',  ( -27.16883889988624290, 3.175000002731187543, -19.73931689729374028 ) ) ;
#14174=CARTESIAN_POINT ( 'NONE',  ( -27.16883889988624290, 16.92500000273117067, -19.73931689729374028 ) ) ;
#14175=CARTESIAN_POINT ( 'NONE',  ( -11.25946833292375793, 71.07500000273120122, 8.180482586598737171 ) ) ;
#14177=CARTESIAN_POINT ( 'NONE',  ( 15.00000000000000000, 79.00000000000001421, -1.836970198721029589E-15 ) ) ;
#14180=CARTESIAN_POINT ( 'NONE',  ( -5.147494310547423346, 38.94874572391552192, 32.50000000000000000 ) ) ;
#14182=CARTESIAN_POINT ( 'NONE',  ( -27.16883889988624290, 36.92500000273118843, -19.73931689729374028 ) ) ;
#14185=CARTESIAN_POINT ( 'NONE',  ( -33.58253175000000113, 25.47500000273118914, 10.91162601494193929 ) ) ;
#14186=CARTESIAN_POINT ( 'NONE',  ( 1.555960095263670572E-15, 16.24999999453762101, -24.50000000000000000 ) ) ;
#14190=( BOUNDED_CURVE ( )  B_SPLINE_CURVE ( 2, ( #21093, #8033, #18519, #297, #28965, #5461, #15942, #26398, #19020, #13697, #21919, #5631, #18850, #29298, #3723, #32036, #14193, #802, #24162, #16770, #632, #8534, #1122, #8362, #16115, #11122, #26567, #29461, #32369, #3063, #5796, #8863, #21590, #13534, #19348, #19182, #23997, #5964, #3393, #11284, #16442, #21762, #26894, #16278, #3229, #8198, #26736, #13863, #8699, #24328, #32205, #29620, #6123, #468, #11442, #10951, #21427, #16607, #29790, #27060, #3553, #6294, #29128, #14026, #24489, #31868, #962, #24648, #27229, #21261, #31706, #18689, #27735, #6465, #30464, #27564, #6962, #16939, #32698, #1468, #27396, #11944, #4223, #25155, #19839, #9710, #14697, #20018, #14525, #25506, #17612, #17272, #1631, #20192, #22413, #12109, #14864, #22581, #14358, #28074, #24985, #30292, #30635, #17447, #6793, #4050, #33032, #11775, #9536, #7132, #27908, #4390, #4563, #25329, #1807, #22255, #12283, #19512, #19677, #22757, #33207, #3885, #9192, #32861, #24816, #9358, #32533, #9033, #11607, #15041, #22089, #29960, #1293, #30123, #6626, #17105, #23615, #2155, #15733, #26187, #7303, #12460, #20718, #30809, #12975, #31499, #17966, #31159, #17787, #21050, #12805, #2683, #30986, #33386, #7486, #20541, #28415, #12629, #13142, #33562, #1985, #28247, #4905, #15211, #28581, #84, #18137, #15386, #10571, #10401, #25842, #10061, #7991, #15563, #20880, #26015, #33742, #10237, #2330, #18476, #20362 ),
 .UNSPECIFIED., .F., .T. ) 
 B_SPLINE_CURVE_WITH_KNOTS ( ( 3, 2, 2, 2, 2, 2, 2, 2, 2, 2, 2, 2, 2, 2, 2, 2, 2, 2, 2, 2, 2, 2, 2, 2, 2, 2, 2, 2, 2, 2, 2, 2, 2, 2, 2, 2, 2, 2, 2, 2, 2, 2, 2, 2, 2, 2, 2, 2, 2, 2, 2, 2, 2, 2, 2, 2, 2, 2, 2, 2, 2, 2, 2, 2, 2, 2, 2, 2, 2, 2, 2, 2, 2, 2, 2, 2, 2, 2, 2, 2, 2, 2, 2, 2, 2, 2, 2, 2, 2, 2, 3 ),
 ( 0.000000000000000000, 0.01111111111111111154, 0.02222222222222222307, 0.03333333333333333287, 0.04444444444444444614, 0.05555555555555555247, 0.06666666666666666574, 0.07777777777777777901, 0.08888888888888889228, 0.1000000000000000056, 0.1111111111111111049, 0.1222222222222222182, 0.1333333333333333315, 0.1444444444444444309, 0.1555555555555555580, 0.1666666666666666574, 0.1777777777777777846, 0.1888888888888888840, 0.2000000000000000111, 0.2111111111111111105, 0.2222222222222222099, 0.2333333333333333370, 0.2444444444444444364, 0.2555555555555555358, 0.2666666666666666630, 0.2777777777777777901, 0.2888888888888888618, 0.2999999999999999889, 0.3111111111111111160, 0.3222222222222222432, 0.3333333333333333148, 0.3444444444444444420, 0.3555555555555555691, 0.3666666666666666408, 0.3777777777777777679, 0.3888888888888888951, 0.4000000000000000222, 0.4111111111111110938, 0.4222222222222222210, 0.4333333333333333481, 0.4444444444444444198, 0.4555555555555555469, 0.4666666666666666741, 0.4777777777777778012, 0.4888888888888888729, 0.5000000000000000000, 0.5111111111111110716, 0.5222222222222222543, 0.5333333333333333259, 0.5444444444444443976, 0.5555555555555555802, 0.5666666666666666519, 0.5777777777777777235, 0.5888888888888889062, 0.5999999999999999778, 0.6111111111111111605, 0.6222222222222222321, 0.6333333333333333037, 0.6444444444444444864, 0.6555555555555555580, 0.6666666666666666297, 0.6777777777777778123, 0.6888888888888888840, 0.6999999999999999556, 0.7111111111111111382, 0.7222222222222222099, 0.7333333333333332815, 0.7444444444444444642, 0.7555555555555555358, 0.7666666666666667185, 0.7777777777777777901, 0.7888888888888888618, 0.8000000000000000444, 0.8111111111111111160, 0.8222222222222221877, 0.8333333333333333703, 0.8444444444444444420, 0.8555555555555555136, 0.8666666666666666963, 0.8777777777777777679, 0.8888888888888888395, 0.9000000000000000222, 0.9111111111111110938, 0.9222222222222222765, 0.9333333333333333481, 0.9444444444444444198, 0.9555555555555556024, 0.9666666666666666741, 0.9777777777777777457, 0.9888888888888889284, 1.000000000000000000 ),
 .UNSPECIFIED. ) 
 CURVE ( )  GEOMETRIC_REPRESENTATION_ITEM ( )  RATIONAL_B_SPLINE_CURVE ( ( 1.000000000000000000, 0.9510565162951535312, 1.000000000000000000, 0.9510565162951535312, 1.000000000000000000, 0.9510565162951535312, 1.000000000000000000, 0.9510565162951535312, 1.000000000000000000, 0.9510565162951535312, 1.000000000000000000, 0.9510565162951535312, 1.000000000000000000, 0.9510565162951535312, 1.000000000000000000, 0.9510565162951535312, 1.000000000000000000, 0.9510565162951535312, 1.000000000000000000, 0.9510565162951535312, 1.000000000000000000, 0.9510565162951535312, 1.000000000000000000, 0.9510565162951535312, 1.000000000000000000, 0.9510565162951535312, 1.000000000000000000, 0.9510565162951535312, 1.000000000000000000, 0.9510565162951535312, 1.000000000000000000, 0.9510565162951535312, 1.000000000000000000, 0.9510565162951535312, 1.000000000000000000, 0.9510565162951535312, 1.000000000000000000, 0.9510565162951535312, 1.000000000000000000, 0.9510565162951535312, 1.000000000000000000, 0.9510565162951535312, 1.000000000000000000, 0.9510565162951535312, 1.000000000000000000, 0.9510565162951535312, 1.000000000000000000, 0.9510565162951535312, 1.000000000000000000, 0.9510565162951535312, 1.000000000000000000, 0.9510565162951535312, 1.000000000000000000, 0.9510565162951535312, 1.000000000000000000, 0.9510565162951535312, 1.000000000000000000, 0.9510565162951535312, 1.000000000000000000, 0.9510565162951535312, 1.000000000000000000, 0.9510565162951535312, 1.000000000000000000, 0.9510565162951535312, 1.000000000000000000, 0.9510565162951535312, 1.000000000000000000, 0.9510565162951535312, 1.000000000000000000, 0.9510565162951535312, 1.000000000000000000, 0.9510565162951535312, 1.000000000000000000, 0.9510565162951535312, 1.000000000000000000, 0.9510565162951535312, 1.000000000000000000, 0.9510565162951535312, 1.000000000000000000, 0.9510565162951535312, 1.000000000000000000, 0.9510565162951535312, 1.000000000000000000, 0.9510565162951535312, 1.000000000000000000, 0.9510565162951535312, 1.000000000000000000, 0.9510565162951535312, 1.000000000000000000, 0.9510565162951535312, 1.000000000000000000, 0.9510565162951535312, 1.000000000000000000, 0.9510565162951535312, 1.000000000000000000, 0.9510565162951535312, 1.000000000000000000, 0.9510565162951535312, 1.000000000000000000, 0.9510565162951535312, 1.000000000000000000, 0.9510565162951535312, 1.000000000000000000, 0.9510565162951535312, 1.000000000000000000, 0.9510565162951535312, 1.000000000000000000, 0.9510565162951535312, 1.000000000000000000, 0.9510565162951535312, 1.000000000000000000, 0.9510565162951535312, 1.000000000000000000, 0.9510565162951535312, 1.000000000000000000, 0.9510565162951535312, 1.000000000000000000, 0.9510565162951535312, 1.000000000000000000, 0.9510565162951535312, 1.000000000000000000, 0.9510565162951535312, 1.000000000000000000, 0.9510565162951535312, 1.000000000000000000, 0.9510565162951535312, 1.000000000000000000, 0.9510565162951535312, 1.000000000000000000, 0.9510565162951535312, 1.000000000000000000, 0.9510565162951535312, 1.000000000000000000, 0.9510565162951535312, 1.000000000000000000, 0.9510565162951535312, 1.000000000000000000, 0.9510565162951535312, 1.000000000000000000, 0.9510565162951535312, 1.000000000000000000, 0.9510565162951535312, 1.000000000000000000, 0.9510565162951535312, 1.000000000000000000, 0.9510565162951535312, 1.000000000000000000, 0.9510565162951535312, 1.000000000000000000, 0.9510565162951535312, 1.000000000000000000, 0.9510565162951535312, 1.000000000000000000, 0.9510565162951535312, 1.000000000000000000, 0.9510565162951535312, 1.000000000000000000, 0.9510565162951535312, 1.000000000000000000, 0.9510565162951535312, 1.000000000000000000, 0.9510565162951535312, 1.000000000000000000, 0.9510565162951535312, 1.000000000000000000, 0.9510565162951535312, 1.000000000000000000, 0.9510565162951535312, 1.000000000000000000, 0.9510565162951535312, 1.000000000000000000, 0.9510565162951535312, 1.000000000000000000, 0.9510565162951535312, 1.000000000000000000, 0.9510565162951535312, 1.000000000000000000, 0.9510565162951535312, 1.000000000000000000, 0.9510565162951535312, 1.000000000000000000 ) ) 
 REPRESENTATION_ITEM ( '' )  );
#14193=CARTESIAN_POINT ( 'NONE',  ( 7.236395654485755280, 2.224999997268800378, 22.27133577429736988 ) ) ;
#14197=EDGE_CURVE ( 'NONE', #33960, #10375, #11184, .T. ) ;
#14198=CYLINDRICAL_SURFACE ( 'NONE', #10149, 32.50000000000000000 ) ;
#14199=CARTESIAN_POINT ( 'NONE',  ( 20.75514604977249178, 21.82500000273118346, 28.56700777964553950 ) ) ;
#14200=CARTESIAN_POINT ( 'NONE',  ( -18.94512977948575738, 3.924999997268807661, -13.76444248337723231 ) ) ;
#14202=VERTEX_POINT ( 'NONE', #17831 ) ;
#14208=CARTESIAN_POINT ( 'NONE',  ( -20.08610463437156923, 10.29999999999999361, 27.64615127144130113 ) ) ;
#14209=CARTESIAN_POINT ( 'NONE',  ( 7.570916362186207671, 13.34999999453762065, 23.30088464923126779 ) ) ;
#14210=CARTESIAN_POINT ( 'NONE',  ( -4.523095164977116484E-15, 4.124999997268806951, 24.62258325217400312 ) ) ;
#14211=CARTESIAN_POINT ( 'NONE',  ( -10.37757302488623701, 23.77500000273119340, 31.93888565452638417 ) ) ;
#14212=CARTESIAN_POINT ( 'NONE',  ( 26.29305231718579350, 31.30000000546237615, 19.10302069950537529 ) ) ;
#14213=CARTESIAN_POINT ( 'NONE',  ( 20.08610463437158344, 74.70000000000000284, 27.64615127144129403 ) ) ;
#14214=CARTESIAN_POINT ( 'NONE',  ( 32.50000000000000000, 47.50000000546239676, -3.980102097228898626E-15 ) ) ;
#14215=CARTESIAN_POINT ( 'NONE',  ( 0.000000000000000000, 80.00000000000001421, 0.000000000000000000 ) ) ;
#14217=CARTESIAN_POINT ( 'NONE',  ( 10.37757302488624767, 37.97500000273118559, 31.93888565452638417 ) ) ;
#14221=CARTESIAN_POINT ( 'NONE',  ( -18.94512977948575738, 11.92499999726881477, -13.76444248337723231 ) ) ;
#14222=CARTESIAN_POINT ( 'NONE',  ( 26.29305231718579350, 16.79999999999998295, 19.10302069950537529 ) ) ;
#14225=CARTESIAN_POINT ( 'NONE',  ( -27.16883889988624290, 60.92500000273118133, -19.73931689729374028 ) ) ;
#14226=CARTESIAN_POINT ( 'NONE',  ( -33.58253175000000113, 45.47500000273119980, 10.91162601494193929 ) ) ;
#14229=CARTESIAN_POINT ( 'NONE',  ( -33.58253175000000113, 5.225000002731188253, 10.91162601494193929 ) ) ;
#14231=CARTESIAN_POINT ( 'NONE',  ( 32.50000000000000000, 25.60000000546239107, -10.55989012756945833 ) ) ;
#14232=CARTESIAN_POINT ( 'NONE',  ( -32.50000000000000000, 41.89999999999998437, -10.55989012756945300 ) ) ;
#14234=LINE ( 'NONE', #3927, #20444 ) ;
#14241=VERTEX_POINT ( 'NONE', #15774 ) ;
#14249=CARTESIAN_POINT ( 'NONE',  ( 5.147494310547434893, 56.55125428154683220, 32.49999999999999289 ) ) ;
#14250=CARTESIAN_POINT ( 'NONE',  ( 20.75514604977249178, 46.07500000273117280, 28.56700777964553950 ) ) ;
#14251=CARTESIAN_POINT ( 'NONE',  ( 26.29305231718578995, 51.70000000546237828, -19.10302069950538240 ) ) ;
#14253=CARTESIAN_POINT ( 'NONE',  ( 20.75514604977248467, 28.42500000273118133, -28.56700777964554305 ) ) ;
#14255=CARTESIAN_POINT ( 'NONE',  ( 6.486482029760649416E-15, 59.87500000273117706, 35.31076352940723240 ) ) ;
#14257=CARTESIAN_POINT ( 'NONE',  ( 32.50000000000000711, 36.89999999999999858, 10.55989012756945122 ) ) ;
#14259=EDGE_CURVE ( 'NONE', #1603, #32300, #25379, .T. ) ;
#14260=CARTESIAN_POINT ( 'NONE',  ( 10.37757302488624056, 2.775000002731176085, -31.93888565452638417 ) ) ;
#14261=DIRECTION ( 'NONE',  ( -0.000000000000000000, -1.000000000000000000, -0.000000000000000000 ) ) ;
#14263=CARTESIAN_POINT ( 'NONE',  ( 6.486482029760648627E-15, 65.87500000273119838, 35.31076352940722529 ) ) ;
#14264=CARTESIAN_POINT ( 'NONE',  ( 3.445340210940985210E-14, 5.499999999999997335, 24.50000000000000000 ) ) ;
#14268=CARTESIAN_POINT ( 'NONE',  ( 15.14183272437241889, 7.449999994537639836, 20.84094480462498211 ) ) ;
#14280=DIRECTION ( 'NONE',  ( 0.000000000000000000, 0.000000000000000000, -1.000000000000000000 ) ) ;
#14281=CARTESIAN_POINT ( 'NONE',  ( 5.779280353836490358E-15, 53.00000000546238255, 32.49999999999999289 ) ) ;
#14284=( BOUNDED_CURVE ( )  B_SPLINE_CURVE ( 2, ( #23193, #2600, #10325, #18227, #2078, #31246, #28840, #4824, #23537, #25931, #26103, #25425, #12553 ),
 .UNSPECIFIED., .F., .T. ) 
 B_SPLINE_CURVE_WITH_KNOTS ( ( 3, 2, 2, 2, 2, 2, 3 ),
 ( 0.3269230769230769273, 0.3282051282051282048, 0.3307692307692307598, 0.3333333333333333148, 0.3358974358974358698, 0.3384615384615384803, 0.3397435897435897578 ),
 .UNSPECIFIED. ) 
 CURVE ( )  GEOMETRIC_REPRESENTATION_ITEM ( )  RATIONAL_B_SPLINE_CURVE ( ( 0.9755282581475768211, 0.9755282581475768211, 1.000000000000000000, 0.9510565162951535312, 1.000000000000000000, 0.9510565162951535312, 1.000000000000000000, 0.9510565162951535312, 1.000000000000000000, 0.9510565162951535312, 1.000000000000000000, 0.9755282581475768211, 0.9755282581475768211 ) ) 
 REPRESENTATION_ITEM ( '' )  );
#14287=ORIENTED_EDGE ( 'NONE', *, *, #17553, .F. ) ;
#14289=ORIENTED_EDGE ( 'NONE', *, *, #24568, .T. ) ;
#14292=CARTESIAN_POINT ( 'NONE',  ( -10.37757302488624411, 52.72500000273119980, -31.93888565452638417 ) ) ;
#14294=CARTESIAN_POINT ( 'NONE',  ( -10.04305231718578462, 8.900000005462372243, 30.90933677959249337 ) ) ;
#14295=LINE ( 'NONE', #569, #2654 ) ;
#14296=CARTESIAN_POINT ( 'NONE',  ( -23.41746825000000243, 14.22499999726880837, 7.608796670333725309 ) ) ;
#14297=CARTESIAN_POINT ( 'NONE',  ( -32.50000000000000000, 56.10000000000000853, 10.55989012756946366 ) ) ;
#14299=CARTESIAN_POINT ( 'NONE',  ( 27.16883889988623935, 26.57500000273119056, -19.73931689729374384 ) ) ;
#14300=CARTESIAN_POINT ( 'NONE',  ( 32.50000000000000000, 5.500000005462357677, -3.980102097228898626E-15 ) ) ;
#14302=CARTESIAN_POINT ( 'NONE',  ( 2.688165632520823219E-15, 75.37500000273118417, 14.63369212191046387 ) ) ;
#14303=CARTESIAN_POINT ( 'NONE',  ( -4.223320258572819786E-15, 13.50000000000000355, 24.50000000000000000 ) ) ;
#14306=VERTEX_POINT ( 'NONE', #2373 ) ;
#14308=CARTESIAN_POINT ( 'NONE',  ( 11.25946833292375793, 71.67500000273119554, 8.180482586598731842 ) ) ;
#14314=CARTESIAN_POINT ( 'NONE',  ( 33.58253175000000113, 10.47500000273119802, -10.91162601494193574 ) ) ;
#14317=CARTESIAN_POINT ( 'NONE',  ( 4.300734207923757602, 78.77500000273118985, -13.23629886949340673 ) ) ;
#14319=VECTOR ( 'NONE', #30264, 1000.000000000000000 ) ;
#14320=CARTESIAN_POINT ( 'NONE',  ( -1.778240108872766143E-15, 63.50000000000000000, -32.49999999999999289 ) ) ;
#14321=CARTESIAN_POINT ( 'NONE',  ( 27.16883889988623935, 52.32500000273118701, -19.73931689729374384 ) ) ;
#14323=ORIENTED_EDGE ( 'NONE', *, *, #7038, .T. ) ;
#14325=CARTESIAN_POINT ( 'NONE',  ( 20.08610463437158344, 16.69999999999999574, 27.64615127144129403 ) ) ;
#14326=CARTESIAN_POINT ( 'NONE',  ( -18.94512977948575738, 3.424999997268807217, -13.76444248337723231 ) ) ;
#14333=CARTESIAN_POINT ( 'NONE',  ( 33.58253175000000113, 60.47500000273118559, -10.91162601494193751 ) ) ;
#14334=CARTESIAN_POINT ( 'NONE',  ( 5.779280353836490358E-15, 17.00000000546237899, 32.49999999999999289 ) ) ;
#14335=CARTESIAN_POINT ( 'NONE',  ( 20.75514604977249178, 73.82500000273121543, 28.56700777964553950 ) ) ;
#14337=CARTESIAN_POINT ( 'NONE',  ( -4.732186688966233175E-15, 5.500000000000000888, 25.76082449383753925 ) ) ;
#14338=CARTESIAN_POINT ( 'NONE',  ( -27.16883889988623935, 5.575000002731201221, 19.73931689729374739 ) ) ;
#14339=CARTESIAN_POINT ( 'NONE',  ( -33.58253175000000113, 15.12500000273120371, 0.000000000000000000 ) ) ;
#14340=CARTESIAN_POINT ( 'NONE',  ( 4.300734207923757602, 72.27500000273117564, -13.23629886949340673 ) ) ;
#14343=CARTESIAN_POINT ( 'NONE',  ( -15.00000000000000000, 80.10000000000000853, 4.873795443493597723 ) ) ;
#14346=CARTESIAN_POINT ( 'NONE',  ( 0.000000000000000000, 82.00000000000001421, 0.000000000000000000 ) ) ;
#14349=CARTESIAN_POINT ( 'NONE',  ( -2.162160676586881955E-15, 40.62500000273120548, -35.31076352940723240 ) ) ;
#14352=CARTESIAN_POINT ( 'NONE',  ( -33.58253175000000113, 29.47500000273117848, 10.91162601494193929 ) ) ;
#14355=CARTESIAN_POINT ( 'NONE',  ( -3.880418787951136483, 14.30125427608446920, -24.50000000000000000 ) ) ;
#14358=CARTESIAN_POINT ( 'NONE',  ( 18.94512977948575738, 10.42499999726881299, 13.76444248337723408 ) ) ;
#14362=CARTESIAN_POINT ( 'NONE',  ( 0.000000000000000000, 80.00000000000001421, 0.000000000000000000 ) ) ;
#14363=CARTESIAN_POINT ( 'NONE',  ( -20.75514604977248112, 15.42500000273118665, 28.56700777964554661 ) ) ;
#14364=CARTESIAN_POINT ( 'NONE',  ( 1.507698388325705758E-15, 7.624999997268814056, -24.62258325217400312 ) ) ;
#14372=CARTESIAN_POINT ( 'NONE',  ( 7.570916362186207671, 19.34999999453762598, 23.30088464923126779 ) ) ;
#14373=CARTESIAN_POINT ( 'NONE',  ( 1.507698388325705758E-15, 5.124999997268805174, -24.62258325217400312 ) ) ;
#14374=CARTESIAN_POINT ( 'NONE',  ( -27.16883889988623935, 23.57500000273119056, 19.73931689729374739 ) ) ;
#14375=CARTESIAN_POINT ( 'NONE',  ( 32.50000000000000000, 29.60000000546238041, -10.55989012756945833 ) ) ;
#14376=CARTESIAN_POINT ( 'NONE',  ( -10.04305231718579172, 71.59999999999999432, -30.90933677959248982 ) ) ;
#14377=CARTESIAN_POINT ( 'NONE',  ( 0.000000000000000000, 70.00000000000000000, 0.000000000000000000 ) ) ;
#14380=CARTESIAN_POINT ( 'NONE',  ( 6.486482029760649416E-15, 33.87500000273118417, 35.31076352940723240 ) ) ;
#14383=( BOUNDED_CURVE ( )  B_SPLINE_CURVE ( 2, ( #2006, #22951, #7671, #28268, #4754, #15231, #18157, #25694, #28599, #33930, #7504, #7840, #10421 ),
 .UNSPECIFIED., .F., .T. ) 
 B_SPLINE_CURVE_WITH_KNOTS ( ( 3, 2, 2, 2, 2, 2, 3 ),
 ( 0.2500000000000000000, 0.2600000000000000089, 0.2800000000000000266, 0.2999999999999999889, 0.3200000000000000067, 0.3400000000000000244, 0.3500000000000000333 ),
 .UNSPECIFIED. ) 
 CURVE ( )  GEOMETRIC_REPRESENTATION_ITEM ( )  RATIONAL_B_SPLINE_CURVE ( ( 0.9755282581475768211, 0.9755282581475768211, 1.000000000000000000, 0.9510565162951535312, 1.000000000000000000, 0.9510565162951535312, 1.000000000000000000, 0.9510565162951535312, 1.000000000000000000, 0.9510565162951535312, 1.000000000000000000, 0.9755282581475767101, 0.9755282581475768211 ) ) 
 REPRESENTATION_ITEM ( '' )  );
#14386=CARTESIAN_POINT ( 'NONE',  ( -7.236395654485763274, 8.524999997268800200, 22.27133577429736633 ) ) ;
#14387=CARTESIAN_POINT ( 'NONE',  ( 20.08610463437158344, 12.70000000000000639, 27.64615127144129403 ) ) ;
#14390=( BOUNDED_CURVE ( )  B_SPLINE_CURVE ( 2, ( #18078, #22162, #3626, #6194, #32605, #29368, #29525, #16506, #24556, #6538, #8937, #13930, #14264 ),
 .UNSPECIFIED., .F., .T. ) 
 B_SPLINE_CURVE_WITH_KNOTS ( ( 3, 2, 2, 2, 2, 2, 3 ),
 ( 0.2499999999999999722, 0.2555555555555555358, 0.2666666666666666630, 0.2777777777777777901, 0.2888888888888888618, 0.2999999999999999889, 0.3055555555555555802 ),
 .UNSPECIFIED. ) 
 CURVE ( )  GEOMETRIC_REPRESENTATION_ITEM ( )  RATIONAL_B_SPLINE_CURVE ( ( 0.9755282581475768211, 0.9755282581475768211, 1.000000000000000000, 0.9510565162951535312, 1.000000000000000000, 0.9510565162951535312, 1.000000000000000000, 0.9510565162951535312, 1.000000000000000000, 0.9510565162951535312, 1.000000000000000000, 0.9755282581475765991, 0.9755282581475767101 ) ) 
 REPRESENTATION_ITEM ( '' )  );
#14391=CARTESIAN_POINT ( 'NONE',  ( 27.16883889988624290, 59.92500000273118133, 19.73931689729373673 ) ) ;
#14392=CARTESIAN_POINT ( 'NONE',  ( -27.16883889988623935, 45.57500000273117990, 19.73931689729374739 ) ) ;
#14395=DIRECTION ( 'NONE',  ( 0.000000000000000000, -1.000000000000000000, 0.000000000000000000 ) ) ;
#14396=CARTESIAN_POINT ( 'NONE',  ( -1.778240108872766143E-15, 49.50000000000000000, -32.49999999999999289 ) ) ;
#14399=CARTESIAN_POINT ( 'NONE',  ( -10.04305231718578462, 42.39999999999999147, 30.90933677959249337 ) ) ;
#14401=CARTESIAN_POINT ( 'NONE',  ( 3.980102097228898626E-15, 80.00000000000001421, 32.50000000000000000 ) ) ;
#14403=EDGE_CURVE ( 'NONE', #29888, #9319, #6560, .T. ) ;
#14404=CARTESIAN_POINT ( 'NONE',  ( -32.50000000000000000, 30.50000000546237899, 0.000000000000000000 ) ) ;
#14405=ADVANCED_FACE ( 'NONE', ( #15603 ), #4604, .T. ) ;
#14408=CARTESIAN_POINT ( 'NONE',  ( 10.37757302488624767, 33.72500000273117848, 31.93888565452638417 ) ) ;
#14419=CARTESIAN_POINT ( 'NONE',  ( 20.08610463437157279, 21.29999999999999716, -27.64615127144129758 ) ) ;
#14420=CARTESIAN_POINT ( 'NONE',  ( -10.37757302488623701, 43.77500000273118275, 31.93888565452638417 ) ) ;
#14421=CARTESIAN_POINT ( 'NONE',  ( -26.29305231718579350, 48.30000000546236549, -19.10302069950537884 ) ) ;
#14423=CARTESIAN_POINT ( 'NONE',  ( -33.58253175000000113, 31.12500000273119127, 0.000000000000000000 ) ) ;
#14425=CARTESIAN_POINT ( 'NONE',  ( 20.75514604977249178, 54.07500000273118701, 28.56700777964553950 ) ) ;
#14427=CARTESIAN_POINT ( 'NONE',  ( -10.04305231718579172, 35.59999999999999432, -30.90933677959248982 ) ) ;
#14429=CARTESIAN_POINT ( 'NONE',  ( 10.37757302488624767, 73.72500000273119269, 31.93888565452638417 ) ) ;
#14430=LINE ( 'NONE', #8934, #23905 ) ;
#14432=CARTESIAN_POINT ( 'NONE',  ( 27.16883889988624290, 64.17500000273118133, 19.73931689729373673 ) ) ;
#14435=CARTESIAN_POINT ( 'NONE',  ( -33.58253175000000113, 1.250000002731177506, 0.000000000000000000 ) ) ;
#14448=CARTESIAN_POINT ( 'NONE',  ( 32.50000000000000000, 13.50000000546236478, -3.980102097228898626E-15 ) ) ;
#14449=ORIENTED_EDGE ( 'NONE', *, *, #9343, .F. ) ;
#14450=EDGE_CURVE ( 'NONE', #33174, #17621, #9873, .T. ) ;
#14452=CYLINDRICAL_SURFACE ( 'NONE', #16829, 32.50000000000000000 ) ;
#14454=VERTEX_POINT ( 'NONE', #12765 ) ;
#14457=ORIENTED_EDGE ( 'NONE', *, *, #805, .T. ) ;
#14458=CARTESIAN_POINT ( 'NONE',  ( -24.50000000000000000, 12.74999999453763166, -3.000384657911015469E-15 ) ) ;
#14459=CARTESIAN_POINT ( 'NONE',  ( 6.486482029760649416E-15, 47.62500000273118417, 35.31076352940723240 ) ) ;
#14462=CARTESIAN_POINT ( 'NONE',  ( 20.08610463437158344, 9.200000005462387165, 27.64615127144129403 ) ) ;
#14464=CARTESIAN_POINT ( 'NONE',  ( 23.41746824999999887, 13.02499999726881619, 7.608796670333735079 ) ) ;
#14465=CARTESIAN_POINT ( 'NONE',  ( -32.50000000000000000, 51.99999999999999289, 0.000000000000000000 ) ) ;
#14466=CARTESIAN_POINT ( 'NONE',  ( 27.16883889988624290, 22.17500000273120264, 19.73931689729373673 ) ) ;
#14467=CARTESIAN_POINT ( 'NONE',  ( 5.779280353836490358E-15, 25.00000000546237899, 32.49999999999999289 ) ) ;
#14469=CARTESIAN_POINT ( 'NONE',  ( 13.91746824999999887, 75.87500000273116996, -1.704398294459741270E-15 ) ) ;
#14470=LINE ( 'NONE', #17047, #20079 ) ;
#14471=CARTESIAN_POINT ( 'NONE',  ( -26.29305231718579350, 33.79999999999999716, -19.10302069950537884 ) ) ;
#14473=EDGE_LOOP ( 'NONE', ( #4703, #22141, #22100, #13324 ) ) ;
#14475=CARTESIAN_POINT ( 'NONE',  ( 26.29305231718578995, 71.70000000546239960, -19.10302069950538240 ) ) ;
#14481=CARTESIAN_POINT ( 'NONE',  ( 10.37757302488624056, 10.77500000273118275, -31.93888565452638417 ) ) ;
#14484=( BOUNDED_CURVE ( )  B_SPLINE_CURVE ( 2, ( #14186, #27730, #22752, #14520, #4218, #12279, #23093, #27903, #14692, #33027, #6621, #33556, #1627 ),
 .UNSPECIFIED., .F., .T. ) 
 B_SPLINE_CURVE_WITH_KNOTS ( ( 3, 2, 2, 2, 2, 2, 3 ),
 ( 0.8055555555555555802, 0.8111111111111111160, 0.8222222222222221877, 0.8333333333333333703, 0.8444444444444444420, 0.8555555555555555136, 0.8611111111111111605 ),
 .UNSPECIFIED. ) 
 CURVE ( )  GEOMETRIC_REPRESENTATION_ITEM ( )  RATIONAL_B_SPLINE_CURVE ( ( 0.9755282581475768211, 0.9755282581475768211, 1.000000000000000000, 0.9510565162951535312, 1.000000000000000000, 0.9510565162951535312, 1.000000000000000000, 0.9510565162951535312, 1.000000000000000000, 0.9510565162951535312, 1.000000000000000000, 0.9755282581475765991, 0.9755282581475768211 ) ) 
 REPRESENTATION_ITEM ( '' )  );
#14485=CARTESIAN_POINT ( 'NONE',  ( 11.25946833292375793, 80.17500000273119554, 8.180482586598731842 ) ) ;
#14487=CARTESIAN_POINT ( 'NONE',  ( 10.04305231718578817, 63.40000000000001279, -30.90933677959249337 ) ) ;
#14488=CARTESIAN_POINT ( 'NONE',  ( 33.58253175000000823, 54.02500000273118985, 10.91162601494192685 ) ) ;
#14490=ORIENTED_EDGE ( 'NONE', *, *, #24987, .F. ) ;
#14492=DIRECTION ( 'NONE',  ( -0.000000000000000000, -1.000000000000000000, -0.000000000000000000 ) ) ;
#14493=CARTESIAN_POINT ( 'NONE',  ( 14.47279130897151589, 12.32499999726880802, 19.92008829642072953 ) ) ;
#14495=EDGE_CURVE ( 'NONE', #33570, #8435, #12420, .T. ) ;
#14496=VERTEX_POINT ( 'NONE', #25116 ) ;
#14498=CARTESIAN_POINT ( 'NONE',  ( 5.779280353836490358E-15, 35.00000000546238255, 32.49999999999999289 ) ) ;
#14501=CARTESIAN_POINT ( 'NONE',  ( 33.58253175000000113, 62.37500000273119127, -4.112674001490185761E-15 ) ) ;
#14502=CARTESIAN_POINT ( 'NONE',  ( 1.836970198721029589E-15, 82.00000000000001421, 15.00000000000000000 ) ) ;
#14503=CARTESIAN_POINT ( 'NONE',  ( -33.58253175000000113, 69.02500000273118985, -10.91162601494193218 ) ) ;
#14505=CARTESIAN_POINT ( 'NONE',  ( -24.50000000000000355, 14.89999999999999680, -7.960532557706207157 ) ) ;
#14507=CARTESIAN_POINT ( 'NONE',  ( -33.58253175000000113, 19.12500000273118062, 0.000000000000000000 ) ) ;
#14508=CARTESIAN_POINT ( 'NONE',  ( 13.91746825000000065, 71.77500000273120406, 4.522059556121115875 ) ) ;
#14510=CARTESIAN_POINT ( 'NONE',  ( 9.270509831248425314, 78.70000000000000284, 12.75976212528059683 ) ) ;
#14514=CARTESIAN_POINT ( 'NONE',  ( 15.00000000000000355, 75.15000000546237402, 4.873795443493592394 ) ) ;
#14516=CARTESIAN_POINT ( 'NONE',  ( 20.75514604977249178, 37.82500000273117280, 28.56700777964553950 ) ) ;
#14519=CARTESIAN_POINT ( 'NONE',  ( 33.58253175000000113, 30.37500000273119127, -4.112674001490185761E-15 ) ) ;
#14520=CARTESIAN_POINT ( 'NONE',  ( -15.14183272437242067, 16.44999999453761674, -20.84094480462497856 ) ) ;
#14521=CARTESIAN_POINT ( 'NONE',  ( -32.50000000000000000, 8.500000005462361230, 0.000000000000000000 ) ) ;
#14523=CARTESIAN_POINT ( 'NONE',  ( 9.270509831248421762, 81.29999999999999716, -12.75976212528059861 ) ) ;
#14525=CARTESIAN_POINT ( 'NONE',  ( -18.94512977948575738, 9.424999997268812990, -13.76444248337723231 ) ) ;
#14530=CARTESIAN_POINT ( 'NONE',  ( 20.75514604977248467, 16.42500000273118133, -28.56700777964554305 ) ) ;
#14531=CARTESIAN_POINT ( 'NONE',  ( 14.47279130897151589, 10.82499999726880091, 19.92008829642072953 ) ) ;
#14536=EDGE_CURVE ( 'NONE', #30261, #10957, #4154, .T. ) ;
#14537=EDGE_CURVE ( 'NONE', #7360, #11875, #14687, .T. ) ;
#14538=ORIENTED_EDGE ( 'NONE', *, *, #10848, .F. ) ;
#14541=AXIS2_PLACEMENT_3D ( 'NONE', #13176, #2545, #18171 ) ;
#14542=CARTESIAN_POINT ( 'NONE',  ( -26.29305231718579350, 9.800000000000002487, -19.10302069950537884 ) ) ;
#14543=CARTESIAN_POINT ( 'NONE',  ( -15.14183272437242600, 17.04999999453762527, 20.84094480462497856 ) ) ;
#14544=CARTESIAN_POINT ( 'NONE',  ( 23.41746825000000243, 4.724999997268818142, -7.608796670333727974 ) ) ;
#14545=CARTESIAN_POINT ( 'NONE',  ( 27.16883889988624290, 20.17500000273120264, 19.73931689729373673 ) ) ;
#14546=CARTESIAN_POINT ( 'NONE',  ( -2.092463501923844636E-15, 24.00000000546238610, -34.17252228774368916 ) ) ;
#14547=CARTESIAN_POINT ( 'NONE',  ( -32.50000000000000000, 72.09999999999999432, 10.55989012756946366 ) ) ;
#14548=CARTESIAN_POINT ( 'NONE',  ( 5.147494310547434893, 33.05125428700922185, 32.49999999999999289 ) ) ;
#14551=CARTESIAN_POINT ( 'NONE',  ( -27.16883889988624290, 39.17500000273118843, -19.73931689729374028 ) ) ;
#14554=CARTESIAN_POINT ( 'NONE',  ( 23.41746825000000243, 13.22499999726881192, -7.608796670333727974 ) ) ;
#14555=CARTESIAN_POINT ( 'NONE',  ( -20.08610463437156923, 14.29999999999998472, 27.64615127144130113 ) ) ;
#14557=EDGE_CURVE ( 'NONE', #5893, #5805, #30597, .T. ) ;
#14559=CARTESIAN_POINT ( 'NONE',  ( -33.58253175000000113, 55.12500000273118417, 0.000000000000000000 ) ) ;
#14560=AXIS2_PLACEMENT_3D ( 'NONE', #9826, #4334, #14807 ) ;
#14561=CARTESIAN_POINT ( 'NONE',  ( 33.58253175000000113, 48.37500000273120548, -4.112674001490185761E-15 ) ) ;
#14568=CARTESIAN_POINT ( 'NONE',  ( 10.04305231718579705, 66.59999999999999432, 30.90933677959248982 ) ) ;
#14570=CARTESIAN_POINT ( 'NONE',  ( -20.08610463437157989, 78.20000000546235697, -27.64615127144129758 ) ) ;
#14573=CARTESIAN_POINT ( 'NONE',  ( 15.00000000000000355, 71.15000000546237402, 4.873795443493592394 ) ) ;
#14574=CARTESIAN_POINT ( 'NONE',  ( -27.16883889988623935, 33.32500000273120122, 19.73931689729374739 ) ) ;
#14576=ORIENTED_EDGE ( 'NONE', *, *, #8939, .F. ) ;
#14579=CARTESIAN_POINT ( 'NONE',  ( 3.980102097228898626E-15, 80.00000000000001421, 32.50000000000000000 ) ) ;
#14582=AXIS2_PLACEMENT_3D ( 'NONE', #5200, #24074, #21168 ) ;
#14584=( BOUNDED_CURVE ( )  B_SPLINE_CURVE ( 2, ( #3389, #10947, #24324, #30120, #32695, #6623, #25326, #11769, #1804, #3882, #19674, #9029, #12280 ),
 .UNSPECIFIED., .F., .T. ) 
 B_SPLINE_CURVE_WITH_KNOTS ( ( 3, 2, 2, 2, 2, 2, 3 ),
 ( 0.7884615384615384359, 0.7897435897435897134, 0.7923076923076922684, 0.7948717948717948234, 0.7974358974358974894, 0.8000000000000000444, 0.8012820512820513219 ),
 .UNSPECIFIED. ) 
 CURVE ( )  GEOMETRIC_REPRESENTATION_ITEM ( )  RATIONAL_B_SPLINE_CURVE ( ( 0.9755282581475768211, 0.9755282581475768211, 1.000000000000000000, 0.9510565162951535312, 1.000000000000000000, 0.9510565162951535312, 1.000000000000000000, 0.9510565162951535312, 1.000000000000000000, 0.9510565162951535312, 1.000000000000000000, 0.9755282581475768211, 0.9755282581475768211 ) ) 
 REPRESENTATION_ITEM ( '' )  );
#14586=CARTESIAN_POINT ( 'NONE',  ( 32.50000000000000000, 57.10000000000000142, -10.55989012756945833 ) ) ;
#14587=CARTESIAN_POINT ( 'NONE',  ( 27.16883889988624290, 44.17500000273119554, 19.73931689729373673 ) ) ;
#14588=CARTESIAN_POINT ( 'NONE',  ( -10.04305231718578462, 46.90000000546238113, 30.90933677959249337 ) ) ;
#14589=( BOUNDED_CURVE ( )  B_SPLINE_CURVE ( 2, ( #20960, #18221, #2755, #23529, #13220, #23186, #18556, #10145, #7564, #18048, #28492, #4989, #10482 ),
 .UNSPECIFIED., .F., .T. ) 
 B_SPLINE_CURVE_WITH_KNOTS ( ( 3, 2, 2, 2, 2, 2, 3 ),
 ( 0.7756410256410256610, 0.7769230769230769384, 0.7794871794871794934, 0.7820512820512820484, 0.7846153846153846034, 0.7871794871794871584, 0.7884615384615384359 ),
 .UNSPECIFIED. ) 
 CURVE ( )  GEOMETRIC_REPRESENTATION_ITEM ( )  RATIONAL_B_SPLINE_CURVE ( ( 0.9755282581475768211, 0.9755282581475768211, 1.000000000000000000, 0.9510565162951535312, 1.000000000000000000, 0.9510565162951535312, 1.000000000000000000, 0.9510565162951535312, 1.000000000000000000, 0.9510565162951535312, 1.000000000000000000, 0.9755282581475768211, 0.9755282581475768211 ) ) 
 REPRESENTATION_ITEM ( '' )  );
#14591=CARTESIAN_POINT ( 'NONE',  ( 6.486482029760649416E-15, 31.62500000273119483, 35.31076352940723240 ) ) ;
#14592=CARTESIAN_POINT ( 'NONE',  ( 32.50000000000000711, 31.40000000546238468, 10.55989012756945122 ) ) ;
#14593=CARTESIAN_POINT ( 'NONE',  ( 20.75514604977248467, 58.67500000273118843, -28.56700777964554305 ) ) ;
#14597=CARTESIAN_POINT ( 'NONE',  ( -20.08610463437157989, 35.70000000000000995, -27.64615127144129758 ) ) ;
#14599=CARTESIAN_POINT ( 'NONE',  ( -10.37757302488623701, 75.52500000273118985, 31.93888565452638417 ) ) ;
#14602=CARTESIAN_POINT ( 'NONE',  ( 10.37757302488624056, 68.77500000273117564, -31.93888565452638417 ) ) ;
#14604=ADVANCED_FACE ( 'NONE', ( #15522 ), #2467, .T. ) ;
#14605=ORIENTED_EDGE ( 'NONE', *, *, #24113, .T. ) ;
#14606=CARTESIAN_POINT ( 'NONE',  ( -24.50000000000000000, 4.749999994537623671, -3.000384657911015469E-15 ) ) ;
#14608=CARTESIAN_POINT ( 'NONE',  ( -26.29305231718579350, 25.79999999999999005, -19.10302069950537884 ) ) ;
#14618=CARTESIAN_POINT ( 'NONE',  ( -32.50000000000000000, 0.5000000054623809920, 0.000000000000000000 ) ) ;
#14626=CARTESIAN_POINT ( 'NONE',  ( 10.04305231718579705, 65.10000000546240528, 30.90933677959248982 ) ) ;
#14628=CARTESIAN_POINT ( 'NONE',  ( 20.08610463437157279, 27.29999999999997939, -27.64615127144129758 ) ) ;
#14629=CARTESIAN_POINT ( 'NONE',  ( -27.16883889988623935, 51.32500000273118701, 19.73931689729374739 ) ) ;
#14630=CARTESIAN_POINT ( 'NONE',  ( 32.50000000000000711, 55.40000000546238113, 10.55989012756945122 ) ) ;
#14632=CARTESIAN_POINT ( 'NONE',  ( 32.50000000000000711, 11.40000000546237580, 10.55989012756945122 ) ) ;
#14633=AXIS2_PLACEMENT_3D ( 'NONE', #28579, #23448, #26185 ) ;
#14634=CARTESIAN_POINT ( 'NONE',  ( -14.47279130897151767, 17.82499999726881157, -19.92008829642072598 ) ) ;
#14635=CARTESIAN_POINT ( 'NONE',  ( 32.50000000000000711, 54.90000000000001279, 10.55989012756945122 ) ) ;
#14636=CARTESIAN_POINT ( 'NONE',  ( 3.880418787951139592, 1.551254281546846192, 24.50000000000000000 ) ) ;
#14637=CARTESIAN_POINT ( 'NONE',  ( 10.37757302488624056, 16.77500000273118985, -31.93888565452638417 ) ) ;
#14640=CARTESIAN_POINT ( 'NONE',  ( -8.960552108402742093E-16, 72.37500000273116996, -14.63369212191046387 ) ) ;
#14642=CARTESIAN_POINT ( 'NONE',  ( -26.29305231718578995, 22.19999999999999574, 19.10302069950538595 ) ) ;
#14643=AXIS2_PLACEMENT_3D ( 'NONE', #11659, #1008, #32585 ) ;
#14648=CARTESIAN_POINT ( 'NONE',  ( 26.29305231718579350, 71.30000000546237970, 19.10302069950537529 ) ) ;
#14653=CARTESIAN_POINT ( 'NONE',  ( 33.58253175000000823, 4.275000002731189852, 10.91162601494192685 ) ) ;
#14656=CARTESIAN_POINT ( 'NONE',  ( -8.960552108402744065E-16, 72.87500000273115575, -14.63369212191046209 ) ) ;
#14658=CARTESIAN_POINT ( 'NONE',  ( -27.16883889988623935, 51.32500000273118701, 19.73931689729374739 ) ) ;
#14662=CARTESIAN_POINT ( 'NONE',  ( -20.08610463437156923, 2.299999999999985612, 27.64615127144130113 ) ) ;
#14663=CARTESIAN_POINT ( 'NONE',  ( 7.236395654485755280, 10.22499999726880837, 22.27133577429736988 ) ) ;
#14667=CARTESIAN_POINT ( 'NONE',  ( -26.29305231718578995, 34.70000000546239249, 19.10302069950538595 ) ) ;
#14668=ORIENTED_EDGE ( 'NONE', *, *, #31598, .T. ) ;
#14670=CARTESIAN_POINT ( 'NONE',  ( -33.58253175000000113, 59.47500000273118559, 10.91162601494193929 ) ) ;
#14672=CARTESIAN_POINT ( 'NONE',  ( -20.75514604977248823, 68.82500000273118701, -28.56700777964554305 ) ) ;
#14674=CARTESIAN_POINT ( 'NONE',  ( -24.50000000000000355, 12.90000000000000036, -7.960532557706207157 ) ) ;
#14675=CARTESIAN_POINT ( 'NONE',  ( -33.58253175000000113, 3.275000002731191628, -10.91162601494193218 ) ) ;
#14676=CARTESIAN_POINT ( 'NONE',  ( 20.75514604977249178, 11.82500000273118346, 28.56700777964553950 ) ) ;
#14677=CARTESIAN_POINT ( 'NONE',  ( 4.300734207923761154, 71.47500000273119269, 13.23629886949340495 ) ) ;
#14679=CARTESIAN_POINT ( 'NONE',  ( -15.00000000000000000, 76.00000000000001421, 0.000000000000000000 ) ) ;
#14681=DIRECTION ( 'NONE',  ( 0.000000000000000000, 0.000000000000000000, -1.000000000000000000 ) ) ;
#14682=CARTESIAN_POINT ( 'NONE',  ( 5.779280353836490358E-15, 22.49999999999999645, 32.49999999999999289 ) ) ;
#14684=CARTESIAN_POINT ( 'NONE',  ( 15.00000000000000000, 77.25000000546239676, -1.836970198721029589E-15 ) ) ;
#14686=EDGE_CURVE ( 'NONE', #4188, #16901, #27612, .T. ) ;
#14687=( BOUNDED_CURVE ( )  B_SPLINE_CURVE ( 2, ( #9495, #19977, #25467, #30423, #22720, #6922, #1944, #7262, #25290, #28207, #1762, #4693, #20152 ),
 .UNSPECIFIED., .F., .T. ) 
 B_SPLINE_CURVE_WITH_KNOTS ( ( 3, 2, 2, 2, 2, 2, 3 ),
 ( 0.1346153846153846090, 0.1358974358974358865, 0.1384615384615384692, 0.1410256410256410242, 0.1435897435897435792, 0.1461538461538461620, 0.1474358974358974395 ),
 .UNSPECIFIED. ) 
 CURVE ( )  GEOMETRIC_REPRESENTATION_ITEM ( )  RATIONAL_B_SPLINE_CURVE ( ( 0.9755282581475768211, 0.9755282581475768211, 1.000000000000000000, 0.9510565162951535312, 1.000000000000000000, 0.9510565162951535312, 1.000000000000000000, 0.9510565162951535312, 1.000000000000000000, 0.9510565162951535312, 1.000000000000000000, 0.9755282581475768211, 0.9755282581475768211 ) ) 
 REPRESENTATION_ITEM ( '' )  );
#14688=CARTESIAN_POINT ( 'NONE',  ( 20.75514604977248467, 40.42500000273117422, -28.56700777964554305 ) ) ;
#14691=CARTESIAN_POINT ( 'NONE',  ( 33.58253175000000823, 26.27500000273119340, 10.91162601494192685 ) ) ;
#14692=CARTESIAN_POINT ( 'NONE',  ( -19.82091636218621389, 16.94999999453761319, 14.40073868116558842 ) ) ;
#14693=EDGE_CURVE ( 'NONE', #1732, #7660, #11202, .T. ) ;
#14695=CARTESIAN_POINT ( 'NONE',  ( 32.50000000000000000, 79.00000000000001421, -3.980102097228898626E-15 ) ) ;
#14697=CARTESIAN_POINT ( 'NONE',  ( -7.236395654485757944, 9.224999997268806595, -22.27133577429736988 ) ) ;
#14702=CARTESIAN_POINT ( 'NONE',  ( 27.16883889988624290, 13.92500000273116889, 19.73931689729373673 ) ) ;
#14703=CARTESIAN_POINT ( 'NONE',  ( -23.41746825000000243, 12.02499999726881974, -7.608796670333730638 ) ) ;
#14712=CARTESIAN_POINT ( 'NONE',  ( 19.82091636218621389, 17.94999999453761319, -14.40073868116559197 ) ) ;
#14713=CARTESIAN_POINT ( 'NONE',  ( -14.47279130897151589, 13.32499999726880624, -19.92008829642072598 ) ) ;
#14714=CARTESIAN_POINT ( 'NONE',  ( -10.37757302488623701, 19.77500000273118985, 31.93888565452638417 ) ) ;
#14715=CARTESIAN_POINT ( 'NONE',  ( 26.29305231718578995, 21.70000000546237828, -19.10302069950538240 ) ) ;
#14716=CARTESIAN_POINT ( 'NONE',  ( -20.08610463437156923, 72.30000000000002558, 27.64615127144130113 ) ) ;
#14717=CARTESIAN_POINT ( 'NONE',  ( -1.778240108872766143E-15, 6.000000005462371888, -32.49999999999999289 ) ) ;
#14720=CARTESIAN_POINT ( 'NONE',  ( -2.162160676586881955E-15, 34.87500000273117706, -35.31076352940723240 ) ) ;
#14724=CARTESIAN_POINT ( 'NONE',  ( 18.94512977948576093, 11.32499999726882578, -13.76444248337722875 ) ) ;
#14725=CARTESIAN_POINT ( 'NONE',  ( -20.08610463437156923, 16.29999999999997584, 27.64615127144130113 ) ) ;
#14726=CARTESIAN_POINT ( 'NONE',  ( 32.50000000000000711, 9.400000005462381125, 10.55989012756945122 ) ) ;
#14728=CARTESIAN_POINT ( 'NONE',  ( -10.37757302488623701, 59.52500000273119696, 31.93888565452638417 ) ) ;
#14729=CARTESIAN_POINT ( 'NONE',  ( 33.58253175000000113, 46.47500000273119269, -10.91162601494193574 ) ) ;
#14731=CARTESIAN_POINT ( 'NONE',  ( -15.00000000000000000, 70.25000000546238255, 0.000000000000000000 ) ) ;
#14734=CARTESIAN_POINT ( 'NONE',  ( 2.205017735002230837E-13, 56.00000000546238255, -32.50000000000000000 ) ) ;
#14737=DIRECTION ( 'NONE',  ( -0.000000000000000000, -1.000000000000000000, -0.000000000000000000 ) ) ;
#14739=CARTESIAN_POINT ( 'NONE',  ( -1.778240108872766143E-15, 42.00000000546236834, -32.49999999999999289 ) ) ;
#14742=CARTESIAN_POINT ( 'NONE',  ( 12.13525491562421088, 71.05000000546237970, 8.816778784387095058 ) ) ;
#14743=CARTESIAN_POINT ( 'NONE',  ( -20.75514604977248112, 31.42500000273120619, 28.56700777964554661 ) ) ;
#14744=CARTESIAN_POINT ( 'NONE',  ( 6.486482029760649416E-15, 63.87500000273119127, 35.31076352940723240 ) ) ;
#14749=CARTESIAN_POINT ( 'NONE',  ( -5.147494310547423346, 16.94874572391552903, 32.50000000000000000 ) ) ;
#14750=ORIENTED_EDGE ( 'NONE', *, *, #3983, .F. ) ;
#14756=CARTESIAN_POINT ( 'NONE',  ( -2.162160676586881955E-15, 38.87500000273120548, -35.31076352940723240 ) ) ;
#14757=CARTESIAN_POINT ( 'NONE',  ( -32.50000000000000000, 42.60000000546238397, 10.55989012756946366 ) ) ;
#14759=CARTESIAN_POINT ( 'NONE',  ( -20.75514604977248112, 27.42500000273118488, 28.56700777964554661 ) ) ;
#14760=DIRECTION ( 'NONE',  ( 0.000000000000000000, 1.000000000000000000, 0.000000000000000000 ) ) ;
#14761=CARTESIAN_POINT ( 'NONE',  ( 20.75514604977248467, 54.67500000273119554, -28.56700777964554305 ) ) ;
#14764=CARTESIAN_POINT ( 'NONE',  ( 26.29305231718579350, 32.79999999999999716, 19.10302069950537529 ) ) ;
#14766=CARTESIAN_POINT ( 'NONE',  ( -33.58253175000000113, 73.22500000273117848, 10.91162601494193929 ) ) ;
#14768=CARTESIAN_POINT ( 'NONE',  ( -32.50000000000000000, 38.09999999999998010, 10.55989012756946366 ) ) ;
#14769=CARTESIAN_POINT ( 'NONE',  ( -33.58253175000000113, 67.27500000273117564, -10.91162601494193041 ) ) ;
#14771=DIRECTION ( 'NONE',  ( -0.000000000000000000, -1.000000000000000000, -0.000000000000000000 ) ) ;
#14772=CARTESIAN_POINT ( 'NONE',  ( 27.16883889988623935, 18.32500000273118346, -19.73931689729374384 ) ) ;
#14773=CARTESIAN_POINT ( 'NONE',  ( -24.50000000000000000, 10.74999999453762811, -3.000384657911015469E-15 ) ) ;
#14775=CARTESIAN_POINT ( 'NONE',  ( 32.50000000000000000, 47.09999999999999432, -10.55989012756945833 ) ) ;
#14784=( BOUNDED_CURVE ( )  B_SPLINE_CURVE ( 2, ( #3315, #13781, #32125, #16524, #22007, #27486, #16692, #19266, #30215, #30048, #3976, #19435, #6043 ),
 .UNSPECIFIED., .F., .T. ) 
 B_SPLINE_CURVE_WITH_KNOTS ( ( 3, 2, 2, 2, 2, 2, 3 ),
 ( 0.2628205128205128305, 0.2641025641025641080, 0.2666666666666666630, 0.2692307692307692180, 0.2717948717948717730, 0.2743589743589743835, 0.2756410256410256610 ),
 .UNSPECIFIED. ) 
 CURVE ( )  GEOMETRIC_REPRESENTATION_ITEM ( )  RATIONAL_B_SPLINE_CURVE ( ( 0.9755282581475768211, 0.9755282581475768211, 1.000000000000000000, 0.9510565162951535312, 1.000000000000000000, 0.9510565162951535312, 1.000000000000000000, 0.9510565162951535312, 1.000000000000000000, 0.9510565162951535312, 1.000000000000000000, 0.9755282581475768211, 0.9755282581475768211 ) ) 
 REPRESENTATION_ITEM ( '' )  );
#14786=CARTESIAN_POINT ( 'NONE',  ( -26.29305231718579350, 76.30000000546239391, -19.10302069950537884 ) ) ;
#14790=ORIENTED_EDGE ( 'NONE', *, *, #9027, .T. ) ;
#14791=CARTESIAN_POINT ( 'NONE',  ( 33.58253175000000823, 72.27500000273118985, 10.91162601494192863 ) ) ;
#14795=CARTESIAN_POINT ( 'NONE',  ( 10.04305231718578817, 65.90000000546237402, -30.90933677959249337 ) ) ;
#14797=CARTESIAN_POINT ( 'NONE',  ( -19.82091636218621034, 12.54999999453762527, -14.40073868116559552 ) ) ;
#14798=CARTESIAN_POINT ( 'NONE',  ( 20.75514604977248467, 46.42500000273119554, -28.56700777964554305 ) ) ;
#14799=CARTESIAN_POINT ( 'NONE',  ( 1.507698388325705758E-15, 15.12499999726880873, -24.62258325217400312 ) ) ;
#14801=CARTESIAN_POINT ( 'NONE',  ( -32.50000000000000000, 2.500000005462382546, 0.000000000000000000 ) ) ;
#14802=CARTESIAN_POINT ( 'NONE',  ( 5.779280353836490358E-15, 8.500000000000000000, 32.49999999999999289 ) ) ;
#14804=CARTESIAN_POINT ( 'NONE',  ( -32.50000000000000000, 55.99999999999999289, 0.000000000000000000 ) ) ;
#14805=FACE_OUTER_BOUND ( 'NONE', #28924, .T. ) ;
#14806=CARTESIAN_POINT ( 'NONE',  ( 27.16883889988624290, 18.17500000273120264, 19.73931689729373673 ) ) ;
#14807=DIRECTION ( 'NONE',  ( 0.000000000000000000, 0.000000000000000000, 1.000000000000000000 ) ) ;
#14810=CARTESIAN_POINT ( 'NONE',  ( 11.25946833292375793, 76.07500000273120122, -8.180482586598735395 ) ) ;
#14813=VERTEX_POINT ( 'NONE', #11691 ) ;
#14815=CARTESIAN_POINT ( 'NONE',  ( 10.04305231718579705, 71.10000000546237686, 30.90933677959248982 ) ) ;
#14817=ADVANCED_FACE ( 'NONE', ( #19598, #6381 ), #32619, .F. ) ;
#14821=CARTESIAN_POINT ( 'NONE',  ( 20.75514604977249178, 4.075000002731195892, 28.56700777964553950 ) ) ;
#14826=CARTESIAN_POINT ( 'NONE',  ( 8.601468415847520532, 72.07500000273120122, 11.83890561707634603 ) ) ;
#14828=CARTESIAN_POINT ( 'NONE',  ( -33.58253175000000113, 43.02500000273118275, -10.91162601494193041 ) ) ;
#14832=ORIENTED_EDGE ( 'NONE', *, *, #8117, .F. ) ;
#14834=CARTESIAN_POINT ( 'NONE',  ( -1.778240108872766143E-15, 41.49999999999999289, -32.49999999999999289 ) ) ;
#14835=CARTESIAN_POINT ( 'NONE',  ( -14.47279130897152122, 11.92499999726882010, 19.92008829642072243 ) ) ;
#14841=CARTESIAN_POINT ( 'NONE',  ( 32.50000000000000000, 69.60000000546237686, -10.55989012756945833 ) ) ;
#14842=CARTESIAN_POINT ( 'NONE',  ( -20.75514604977248823, 66.82500000273118701, -28.56700777964554305 ) ) ;
#14844=CARTESIAN_POINT ( 'NONE',  ( 1.577395562988744260E-15, 12.50000000000001243, -25.76082449383753925 ) ) ;
#14845=LINE ( 'NONE', #3866, #21019 ) ;
#14846=CARTESIAN_POINT ( 'NONE',  ( -33.58253175000000113, 9.025000002731184523, -10.91162601494193218 ) ) ;
#14849=CARTESIAN_POINT ( 'NONE',  ( 15.00000000000000000, 73.09999999999996589, -4.873795443493596835 ) ) ;
#14854=CARTESIAN_POINT ( 'NONE',  ( -9.657523855033125146E-16, 77.75000000546238255, -15.77193336357400710 ) ) ;
#14856=CARTESIAN_POINT ( 'NONE',  ( -10.37757302488623701, 35.52500000273117564, 31.93888565452638417 ) ) ;
#14859=CARTESIAN_POINT ( 'NONE',  ( 10.37757302488624767, 23.97500000273117138, 31.93888565452638417 ) ) ;
#14861=CARTESIAN_POINT ( 'NONE',  ( -7.570916362186215665, 15.14999999453761603, 23.30088464923126423 ) ) ;
#14862=CARTESIAN_POINT ( 'NONE',  ( 15.00000000000000000, 81.00000000000001421, -1.836970198721029589E-15 ) ) ;
#14864=CARTESIAN_POINT ( 'NONE',  ( 7.236395654485755280, 10.22499999726880837, 22.27133577429736988 ) ) ;
#14868=AXIS2_PLACEMENT_3D ( 'NONE', #23037, #20652, #15320 ) ;
#14870=CARTESIAN_POINT ( 'NONE',  ( 6.486482029760648627E-15, 15.62500000273118062, 35.31076352940722529 ) ) ;
#14871=CARTESIAN_POINT ( 'NONE',  ( 23.41746825000000243, 11.22499999726881548, -7.608796670333727974 ) ) ;
#14873=ORIENTED_EDGE ( 'NONE', *, *, #11926, .T. ) ;
#14883=CARTESIAN_POINT ( 'NONE',  ( -14.47279130897152122, 4.424999997268826313, 19.92008829642072243 ) ) ;
#14884=CARTESIAN_POINT ( 'NONE',  ( 23.41746825000000243, 12.72499999726882436, -7.608796670333727974 ) ) ;
#14885=CARTESIAN_POINT ( 'NONE',  ( 27.16883889988623935, 22.57500000273118701, -19.73931689729374384 ) ) ;
#14886=CARTESIAN_POINT ( 'NONE',  ( 32.50000000000000000, 27.50000000546237544, -3.980102097228898626E-15 ) ) ;
#14887=( BOUNDED_CURVE ( )  B_SPLINE_CURVE ( 2, ( #7130, #11942, #4048, #14523, #30462, #22253, #14862, #22928, #17610, #9030, #11772, #19510, #24814 ),
 .UNSPECIFIED., .F., .T. ) 
 B_SPLINE_CURVE_WITH_KNOTS ( ( 3, 2, 2, 2, 2, 2, 3 ),
 ( 0.05000000000000000278, 0.05999999999999999778, 0.08000000000000000167, 0.1000000000000000056, 0.1199999999999999956, 0.1400000000000000133, 0.1500000000000000222 ),
 .UNSPECIFIED. ) 
 CURVE ( )  GEOMETRIC_REPRESENTATION_ITEM ( )  RATIONAL_B_SPLINE_CURVE ( ( 0.9755282581475768211, 0.9755282581475768211, 1.000000000000000000, 0.9510565162951535312, 1.000000000000000000, 0.9510565162951535312, 1.000000000000000000, 0.9510565162951535312, 1.000000000000000000, 0.9510565162951535312, 1.000000000000000000, 0.9755282581475767101, 0.9755282581475768211 ) ) 
 REPRESENTATION_ITEM ( '' )  );
#14888=CARTESIAN_POINT ( 'NONE',  ( -10.04305231718578462, 66.40000000000001990, 30.90933677959249337 ) ) ;
#14889=DIRECTION ( 'NONE',  ( -0.8660254037844410391, -0.4999999999999958367, -0.000000000000000000 ) ) ;
#14892=CARTESIAN_POINT ( 'NONE',  ( -20.75514604977248112, 37.67500000273118133, 28.56700777964554661 ) ) ;
#14893=DIRECTION ( 'NONE',  ( 0.000000000000000000, 0.000000000000000000, -1.000000000000000000 ) ) ;
#14895=CARTESIAN_POINT ( 'NONE',  ( -2.092463501923844636E-15, 11.49999999999998579, -34.17252228774368916 ) ) ;
#14898=CARTESIAN_POINT ( 'NONE',  ( -33.58253175000000113, 57.12500000273118417, 0.000000000000000000 ) ) ;
#14900=CARTESIAN_POINT ( 'NONE',  ( -27.16883889988624290, 43.17500000273119554, -19.73931689729374028 ) ) ;
#14901=CARTESIAN_POINT ( 'NONE',  ( 20.08610463437158344, 44.69999999999998153, 27.64615127144129403 ) ) ;
#14902=CARTESIAN_POINT ( 'NONE',  ( 15.14183272437242422, 10.29999999999999361, -20.84094480462497856 ) ) ;
#14906=CARTESIAN_POINT ( 'NONE',  ( 19.82091636218621034, 3.799999999999998046, 14.40073868116559730 ) ) ;
#14908=CARTESIAN_POINT ( 'NONE',  ( 2.489536152421872915E-14, 76.00000000546238255, -32.49999999999999289 ) ) ;
#14910=DIRECTION ( 'NONE',  ( 0.000000000000000000, 0.000000000000000000, -1.000000000000000000 ) ) ;
#14913=DIRECTION ( 'NONE',  ( -0.000000000000000000, -1.000000000000000000, -0.000000000000000000 ) ) ;
#14914=CARTESIAN_POINT ( 'NONE',  ( -10.37757302488624411, 32.72500000273117848, -31.93888565452638417 ) ) ;
#14919=EDGE_CURVE ( 'NONE', #14306, #33710, #24205, .T. ) ;
#14920=CARTESIAN_POINT ( 'NONE',  ( -20.08610463437156923, 16.80000000546237970, 27.64615127144130113 ) ) ;
#14921=EDGE_LOOP ( 'NONE', ( #8132, #20416, #27616, #1645 ) ) ;
#14925=EDGE_CURVE ( 'NONE', #17393, #30686, #15807, .T. ) ;
#14927=CARTESIAN_POINT ( 'NONE',  ( -32.50000000000000000, 45.90000000000000568, -10.55989012756945300 ) ) ;
#14928=CARTESIAN_POINT ( 'NONE',  ( 6.486482029760649416E-15, 43.87500000273118417, 35.31076352940723240 ) ) ;
#14929=CARTESIAN_POINT ( 'NONE',  ( 32.50000000000000000, 41.50000000546238965, -3.980102097228898626E-15 ) ) ;
#14931=CARTESIAN_POINT ( 'NONE',  ( -10.37757302488623701, 27.52500000273119696, 31.93888565452638417 ) ) ;
#14932=CARTESIAN_POINT ( 'NONE',  ( -1.778240108872766143E-15, 23.49999999999999645, -32.49999999999999289 ) ) ;
#14933=CARTESIAN_POINT ( 'NONE',  ( 33.58253175000000113, 56.37500000273118417, -4.112674001490185761E-15 ) ) ;
#14936=CARTESIAN_POINT ( 'NONE',  ( 32.50000000000000000, 33.10000000000000853, -10.55989012756945833 ) ) ;
#14938=CARTESIAN_POINT ( 'NONE',  ( -10.37757302488624411, 78.72500000273119269, -31.93888565452638417 ) ) ;
#14940=CARTESIAN_POINT ( 'NONE',  ( -19.82091636218621034, 14.80000000000000782, -14.40073868116559552 ) ) ;
#14941=CARTESIAN_POINT ( 'NONE',  ( -27.16883889988624290, 69.17500000273119554, -19.73931689729374028 ) ) ;
#14943=VERTEX_POINT ( 'NONE', #26934 ) ;
#14944=CARTESIAN_POINT ( 'NONE',  ( -33.58253175000000113, 21.02500000273117919, -10.91162601494193218 ) ) ;
#14945=CARTESIAN_POINT ( 'NONE',  ( 24.50000000000000355, 9.849999994537622428, -7.960532557706203605 ) ) ;
#14947=CARTESIAN_POINT ( 'NONE',  ( -2.165007332552593587E-13, 46.50000000000000711, 32.50000000000000000 ) ) ;
#14960=CARTESIAN_POINT ( 'NONE',  ( -20.08610463437156923, 74.80000000546239391, 27.64615127144130113 ) ) ;
#14964=ORIENTED_EDGE ( 'NONE', *, *, #10945, .T. ) ;
#14965=CARTESIAN_POINT ( 'NONE',  ( -10.37757302488623701, 73.77500000273118985, 31.93888565452638417 ) ) ;
#14968=CARTESIAN_POINT ( 'NONE',  ( -26.29305231718578995, 62.70000000546238539, 19.10302069950538595 ) ) ;
#14969=ORIENTED_EDGE ( 'NONE', *, *, #32764, .F. ) ;
#14970=CARTESIAN_POINT ( 'NONE',  ( -10.04305231718579172, 55.59999999999998010, -30.90933677959248982 ) ) ;
#14971=CARTESIAN_POINT ( 'NONE',  ( 27.16883889988624290, 45.92500000273119554, 19.73931689729373673 ) ) ;
#14972=CARTESIAN_POINT ( 'NONE',  ( -23.41746825000000598, 15.72499999726882081, 7.608796670333726198 ) ) ;
#14973=CARTESIAN_POINT ( 'NONE',  ( 32.50000000000000000, 7.500000005462359454, -3.980102097228898626E-15 ) ) ;
#14974=CARTESIAN_POINT ( 'NONE',  ( -10.04305231718579172, 7.599999999999996092, -30.90933677959248982 ) ) ;
#14976=CARTESIAN_POINT ( 'NONE',  ( -10.04305231718578462, 50.39999999999999858, 30.90933677959249337 ) ) ;
#14977=CARTESIAN_POINT ( 'NONE',  ( -33.58253175000000113, 19.27500000273117919, -10.91162601494193218 ) ) ;
#14978=DIRECTION ( 'NONE',  ( -0.000000000000000000, -1.000000000000000000, -0.000000000000000000 ) ) ;
#14980=CARTESIAN_POINT ( 'NONE',  ( 4.300734207923757602, 80.77500000273118985, -13.23629886949340673 ) ) ;
#14982=CARTESIAN_POINT ( 'NONE',  ( -26.29305231718579350, 43.80000000000000426, -19.10302069950537884 ) ) ;
#14988=ADVANCED_FACE ( 'NONE', ( #3432 ), #842, .T. ) ;
#14993=CARTESIAN_POINT ( 'NONE',  ( -2.162160676586882350E-15, 4.875000002731200155, -35.31076352940722529 ) ) ;
#14997=CARTESIAN_POINT ( 'NONE',  ( 32.50000000000000711, 2.899999999999995470, 10.55989012756945122 ) ) ;
#14999=CARTESIAN_POINT ( 'NONE',  ( -27.16883889988624290, 44.92500000273119554, -19.73931689729374028 ) ) ;
#15003=ORIENTED_EDGE ( 'NONE', *, *, #480, .F. ) ;
#15005=CARTESIAN_POINT ( 'NONE',  ( 5.779280353836490358E-15, 19.00000000546237544, 32.49999999999999289 ) ) ;
#15006=CARTESIAN_POINT ( 'NONE',  ( -18.94512977948576093, 13.82499999726882756, 13.76444248337722698 ) ) ;
#15008=ORIENTED_EDGE ( 'NONE', *, *, #14495, .T. ) ;
#15011=ORIENTED_EDGE ( 'NONE', *, *, #27745, .F. ) ;
#15013=CARTESIAN_POINT ( 'NONE',  ( 6.486482029760649416E-15, 69.62500000273118417, 35.31076352940723240 ) ) ;
#15015=ADVANCED_FACE ( 'NONE', ( #3046 ), #23305, .T. ) ;
#15016=CARTESIAN_POINT ( 'NONE',  ( 19.82091636218621034, 13.80000000000000604, 14.40073868116559730 ) ) ;
#15017=CARTESIAN_POINT ( 'NONE',  ( -7.236395654485757944, 3.724999997268802154, -22.27133577429736988 ) ) ;
#15018=CARTESIAN_POINT ( 'NONE',  ( 33.58253175000000823, 8.025000002731188076, 10.91162601494192863 ) ) ;
#15019=CARTESIAN_POINT ( 'NONE',  ( -24.50000000000000000, 6.749999994537625447, -3.000384657911015469E-15 ) ) ;
#15021=CARTESIAN_POINT ( 'NONE',  ( -12.13525491562420910, 74.19999999999998863, 8.816778784387098611 ) ) ;
#15024=CARTESIAN_POINT ( 'NONE',  ( -5.147494310547450880, 70.44874571845318201, 32.49999999999999289 ) ) ;
#15026=EDGE_CURVE ( 'NONE', #28636, #30070, #453, .T. ) ;
#15028=CARTESIAN_POINT ( 'NONE',  ( 5.779280353836490358E-15, 54.49999999999999289, 32.49999999999999289 ) ) ;
#15030=CARTESIAN_POINT ( 'NONE',  ( 2.897257156509938333E-15, 76.75000000546238255, 15.77193336357400710 ) ) ;
#15032=CARTESIAN_POINT ( 'NONE',  ( 27.16883889988623935, 30.32500000273119412, -19.73931689729374384 ) ) ;
#15035=CARTESIAN_POINT ( 'NONE',  ( 6.486482029760648627E-15, 19.87500000273118772, 35.31076352940722529 ) ) ;
#15036=CARTESIAN_POINT ( 'NONE',  ( -5.147494310547423346, 68.44874571845316780, 32.50000000000000000 ) ) ;
#15039=CARTESIAN_POINT ( 'NONE',  ( 5.147494310547217289, 32.55125428154683931, 32.50000000000007105 ) ) ;
#15041=CARTESIAN_POINT ( 'NONE',  ( -23.41746824999999887, 13.52499999726880198, -7.608796670333730638 ) ) ;
#15042=CARTESIAN_POINT ( 'NONE',  ( -33.58253175000000113, 67.22500000273117848, 10.91162601494193929 ) ) ;
#15046=CARTESIAN_POINT ( 'NONE',  ( 20.75514604977249178, 5.825000002731198556, 28.56700777964553950 ) ) ;
#15047=CARTESIAN_POINT ( 'NONE',  ( -4.523095164977116484E-15, 10.62499999726880695, 24.62258325217400312 ) ) ;
#15055=CARTESIAN_POINT ( 'NONE',  ( -26.29305231718579350, 79.79999999999998295, -19.10302069950537884 ) ) ;
#15056=CARTESIAN_POINT ( 'NONE',  ( -26.29305231718579350, 72.30000000546237970, -19.10302069950537884 ) ) ;
#15057=CARTESIAN_POINT ( 'NONE',  ( 14.47279130897151589, 6.824999997268808904, 19.92008829642072953 ) ) ;
#15058=CARTESIAN_POINT ( 'NONE',  ( 7.236395654485760609, 13.02499999726880375, -22.27133577429736633 ) ) ;
#15059=CARTESIAN_POINT ( 'NONE',  ( -2.162160676586881955E-15, 16.87500000273120193, -35.31076352940723240 ) ) ;
#15060=CARTESIAN_POINT ( 'NONE',  ( -32.50000000000000000, 22.50000000546237189, 0.000000000000000000 ) ) ;
#15061=CARTESIAN_POINT ( 'NONE',  ( 10.04305231718578817, 63.40000000000001279, -30.90933677959249337 ) ) ;
#15064=CARTESIAN_POINT ( 'NONE',  ( -27.16883889988624290, 27.17500000273118133, -19.73931689729374028 ) ) ;
#15065=CARTESIAN_POINT ( 'NONE',  ( 13.91746824999999887, 80.37500000273118417, -1.704398294459741270E-15 ) ) ;
#15067=CARTESIAN_POINT ( 'NONE',  ( -23.41746825000000598, 18.22499999726879949, 7.608796670333726198 ) ) ;
#15068=CARTESIAN_POINT ( 'NONE',  ( 26.29305231718579350, 6.800000000000000711, 19.10302069950537529 ) ) ;
#15069=CIRCLE ( 'NONE', #23848, 15.00000000000000000 ) ;
#15070=CARTESIAN_POINT ( 'NONE',  ( -2.165007332552593587E-13, 52.50000000000000711, 32.50000000000000000 ) ) ;
#15072=CARTESIAN_POINT ( 'NONE',  ( 33.58253175000000113, 54.12500000273118417, -4.112674001490185761E-15 ) ) ;
#15074=CARTESIAN_POINT ( 'NONE',  ( 10.37757302488624767, 41.97500000273118559, 31.93888565452638417 ) ) ;
#15076=PLANE ( 'NONE',  #21065 ) ;
#15077=CARTESIAN_POINT ( 'NONE',  ( -20.08610463437157989, 49.70000000000000284, -27.64615127144129758 ) ) ;
#15079=CARTESIAN_POINT ( 'NONE',  ( -20.08610463437157989, 27.69999999999999929, -27.64615127144129758 ) ) ;
#15081=CARTESIAN_POINT ( 'NONE',  ( -26.29305231718579350, 62.30000000546237260, -19.10302069950537884 ) ) ;
#15083=CARTESIAN_POINT ( 'NONE',  ( -13.91746824999999887, 71.12500000273119838, 0.000000000000000000 ) ) ;
#15087=CARTESIAN_POINT ( 'NONE',  ( -10.37757302488623701, 35.52500000273117564, 31.93888565452638417 ) ) ;
#15089=ORIENTED_EDGE ( 'NONE', *, *, #13841, .F. ) ;
#15096=ORIENTED_EDGE ( 'NONE', *, *, #25723, .F. ) ;
#15099=ORIENTED_EDGE ( 'NONE', *, *, #1803, .T. ) ;
#15102=CARTESIAN_POINT ( 'NONE',  ( -10.04305231718579172, 45.60000000000000142, -30.90933677959248982 ) ) ;
#15103=CARTESIAN_POINT ( 'NONE',  ( -27.16883889988623935, 43.57500000273117990, 19.73931689729374739 ) ) ;
#15104=CARTESIAN_POINT ( 'NONE',  ( 20.08610463437157279, 43.80000000546237970, -27.64615127144129758 ) ) ;
#15106=CARTESIAN_POINT ( 'NONE',  ( -10.37757302488623701, 21.52500000273119340, 31.93888565452638417 ) ) ;
#15107=CARTESIAN_POINT ( 'NONE',  ( -20.08610463437156923, 24.29999999999999005, 27.64615127144130113 ) ) ;
#15108=CARTESIAN_POINT ( 'NONE',  ( 33.58253175000000113, 46.37500000273120548, -4.112674001490185761E-15 ) ) ;
#15111=CARTESIAN_POINT ( 'NONE',  ( -32.50000000000000000, 27.99999999999999645, 0.000000000000000000 ) ) ;
#15113=CARTESIAN_POINT ( 'NONE',  ( 20.75514604977249178, 75.82500000273118701, 28.56700777964553950 ) ) ;
#15115=CARTESIAN_POINT ( 'NONE',  ( -24.50000000000000711, 15.09999999999998899, 7.960532557706201828 ) ) ;
#15116=CARTESIAN_POINT ( 'NONE',  ( 33.58253175000000113, 60.37500000273119127, -4.112674001490185761E-15 ) ) ;
#15119=CARTESIAN_POINT ( 'NONE',  ( -33.58253175000000113, 17.12500000273120548, 0.000000000000000000 ) ) ;
#15120=CARTESIAN_POINT ( 'NONE',  ( 24.50000000000000000, 9.749999994537628112, 0.000000000000000000 ) ) ;
#15123=CARTESIAN_POINT ( 'NONE',  ( -1.778240108872766143E-15, 25.50000000000000711, -32.49999999999999289 ) ) ;
#15128=EDGE_CURVE ( 'NONE', #22201, #7013, #31187, .T. ) ;
#15135=DIRECTION ( 'NONE',  ( -0.000000000000000000, -1.000000000000000000, -0.000000000000000000 ) ) ;
#15136=CARTESIAN_POINT ( 'NONE',  ( 10.04305231718579705, 75.10000000546237686, 30.90933677959248982 ) ) ;
#15141=CARTESIAN_POINT ( 'NONE',  ( -20.75514604977248112, 77.67500000273119554, 28.56700777964554661 ) ) ;
#15144=CARTESIAN_POINT ( 'NONE',  ( 32.50000000000000711, 63.40000000546236691, 10.55989012756945122 ) ) ;
#15146=CARTESIAN_POINT ( 'NONE',  ( 3.445340210940985210E-14, 7.499999999999994671, 24.50000000000000000 ) ) ;
#15147=CARTESIAN_POINT ( 'NONE',  ( 33.58253175000000823, 46.02500000273118275, 10.91162601494192863 ) ) ;
#15148=CARTESIAN_POINT ( 'NONE',  ( -7.236395654485763274, 18.02499999726880731, 22.27133577429736633 ) ) ;
#15149=CARTESIAN_POINT ( 'NONE',  ( 6.277390505771533514E-15, 7.000000005462369224, 34.17252228774368916 ) ) ;
#15151=FACE_OUTER_BOUND ( 'NONE', #9765, .T. ) ;
#15152=CARTESIAN_POINT ( 'NONE',  ( 20.08610463437157279, 49.29999999999998295, -27.64615127144129758 ) ) ;
#15153=CARTESIAN_POINT ( 'NONE',  ( 5.779280353836490358E-15, 28.50000000000000355, 32.49999999999999289 ) ) ;
#15154=CARTESIAN_POINT ( 'NONE',  ( -27.16883889988624290, 15.17500000273119909, -19.73931689729374028 ) ) ;
#15155=CARTESIAN_POINT ( 'NONE',  ( 3.778760231354629433E-15, 0.5000000000000067724, -24.50000000000000355 ) ) ;
#15157=CARTESIAN_POINT ( 'NONE',  ( -8.601468415847515203, 75.67500000273118133, 11.83890561707634959 ) ) ;
#15158=FACE_OUTER_BOUND ( 'NONE', #13764, .T. ) ;
#15159=CARTESIAN_POINT ( 'NONE',  ( -5.147494310547430452, 43.55125428154684641, -32.49999999999999289 ) ) ;
#15171=EDGE_CURVE ( 'NONE', #1581, #1179, #21410, .T. ) ;
#15173=CARTESIAN_POINT ( 'NONE',  ( 5.147494310547434893, 2.551254281546845082, 32.49999999999999289 ) ) ;
#15175=CARTESIAN_POINT ( 'NONE',  ( 33.58253175000000113, 48.22500000273119269, -10.91162601494193574 ) ) ;
#15182=ADVANCED_FACE ( 'NONE', ( #28949 ), #20744, .T. ) ;
#15183=CARTESIAN_POINT ( 'NONE',  ( -27.16883889988623935, 73.57500000273120122, 19.73931689729374739 ) ) ;
#15189=CARTESIAN_POINT ( 'NONE',  ( -2.162160676586881955E-15, 66.62500000273118417, -35.31076352940723240 ) ) ;
#15192=CARTESIAN_POINT ( 'NONE',  ( -15.14183272437242600, 11.29999999999999361, 20.84094480462497856 ) ) ;
#15193=CARTESIAN_POINT ( 'NONE',  ( 14.47279130897151944, 1.424999997268804997, -19.92008829642072598 ) ) ;
#15194=CARTESIAN_POINT ( 'NONE',  ( -33.58253175000000113, 13.12500000273120193, 0.000000000000000000 ) ) ;
#15196=CARTESIAN_POINT ( 'NONE',  ( 4.635254915624212657, 74.59999999999999432, 14.26584774442730286 ) ) ;
#15198=CARTESIAN_POINT ( 'NONE',  ( -32.50000000000000000, 70.09999999999999432, 10.55989012756946366 ) ) ;
#15199=CARTESIAN_POINT ( 'NONE',  ( 26.29305231718579350, 61.30000000546237260, 19.10302069950537529 ) ) ;
#15201=CARTESIAN_POINT ( 'NONE',  ( -8.960552108402742093E-16, 80.37500000273115575, -14.63369212191046387 ) ) ;
#15203=CARTESIAN_POINT ( 'NONE',  ( -27.16883889988623935, 31.32500000273119412, 19.73931689729374739 ) ) ;
#15206=CARTESIAN_POINT ( 'NONE',  ( -2.162160676586882350E-15, 22.87500000273118062, -35.31076352940722529 ) ) ;
#15207=CARTESIAN_POINT ( 'NONE',  ( -10.04305231718578462, 68.40000000000001990, 30.90933677959249337 ) ) ;
#15208=CARTESIAN_POINT ( 'NONE',  ( -10.37757302488624411, 78.72500000273119269, -31.93888565452638417 ) ) ;
#15209=CARTESIAN_POINT ( 'NONE',  ( 3.880418787951159132, 8.448745718453144704, -24.49999999999999289 ) ) ;
#15211=CARTESIAN_POINT ( 'NONE',  ( 14.47279130897151944, 16.92499999726880944, -19.92008829642072598 ) ) ;
#15212=CARTESIAN_POINT ( 'NONE',  ( 20.75514604977248467, 64.42500000273116711, -28.56700777964554305 ) ) ;
#15216=CARTESIAN_POINT ( 'NONE',  ( 27.16883889988624290, 7.925000002731191984, 19.73931689729373673 ) ) ;
#15217=CARTESIAN_POINT ( 'NONE',  ( -18.94512977948575738, 13.92499999726881654, -13.76444248337723231 ) ) ;
#15219=EDGE_LOOP ( 'NONE', ( #20933, #8378, #22017, #23879 ) ) ;
#15221=ORIENTED_EDGE ( 'NONE', *, *, #30248, .T. ) ;
#15225=DIRECTION ( 'NONE',  ( -0.000000000000000000, -1.000000000000000000, -0.000000000000000000 ) ) ;
#15226=CARTESIAN_POINT ( 'NONE',  ( -23.41746824999999887, 4.124999997268813168, -2.867812753649727150E-15 ) ) ;
#15227=CARTESIAN_POINT ( 'NONE',  ( -23.41746825000000598, 11.72499999726882614, 7.608796670333726198 ) ) ;
#15228=CARTESIAN_POINT ( 'NONE',  ( -20.75514604977248112, 15.67500000273117600, 28.56700777964554661 ) ) ;
#15229=CARTESIAN_POINT ( 'NONE',  ( 20.08610463437157279, 17.80000000546237615, -27.64615127144129758 ) ) ;
#15230=CARTESIAN_POINT ( 'NONE',  ( 32.50000000000000711, 64.89999999999997726, 10.55989012756945122 ) ) ;
#15231=CARTESIAN_POINT ( 'NONE',  ( 15.00000000000000000, 77.35000000546237686, -4.873795443493596835 ) ) ;
#15232=CARTESIAN_POINT ( 'NONE',  ( -33.04126587500000056, 79.68750000136559208, 0.000000000000000000 ) ) ;
#15234=CARTESIAN_POINT ( 'NONE',  ( 20.75514604977248467, 28.67500000273117777, -28.56700777964554305 ) ) ;
#15235=CARTESIAN_POINT ( 'NONE',  ( 8.601468415847520532, 80.07500000273118701, 11.83890561707634781 ) ) ;
#15238=CARTESIAN_POINT ( 'NONE',  ( -7.236395654485757944, 15.72499999726881192, -22.27133577429736988 ) ) ;
#15239=CARTESIAN_POINT ( 'NONE',  ( -20.08610463437156923, 10.29999999999999361, 27.64615127144130113 ) ) ;
#15240=VECTOR ( 'NONE', #5792, 1000.000000000000000 ) ;
#15243=CARTESIAN_POINT ( 'NONE',  ( -33.58253175000000113, 47.22500000273117138, 10.91162601494193929 ) ) ;
#15245=CARTESIAN_POINT ( 'NONE',  ( -20.75514604977248112, 43.67500000273119554, 28.56700777964554661 ) ) ;
#15248=CARTESIAN_POINT ( 'NONE',  ( -15.14183272437242067, 8.699999999999986855, -20.84094480462497856 ) ) ;
#15249=ADVANCED_FACE ( 'NONE', ( #33936 ), #10598, .F. ) ;
#15250=CARTESIAN_POINT ( 'NONE',  ( 5.147494310547327423, 51.05125428700922896, 32.50000000000003553 ) ) ;
#15253=CARTESIAN_POINT ( 'NONE',  ( 20.08610463437158344, 6.699999999999991296, 27.64615127144129403 ) ) ;
#15255=CARTESIAN_POINT ( 'NONE',  ( 5.147494310547426899, 41.94874572391552192, -32.50000000000000000 ) ) ;
#15258=CARTESIAN_POINT ( 'NONE',  ( -1.778240108872766143E-15, 11.49999999999999112, -32.49999999999999289 ) ) ;
#15259=CARTESIAN_POINT ( 'NONE',  ( -20.75514604977248823, 24.82500000273117635, -28.56700777964554305 ) ) ;
#15266=ORIENTED_EDGE ( 'NONE', *, *, #17014, .F. ) ;
#15272=LINE ( 'NONE', #28137, #26165 ) ;
#15273=CARTESIAN_POINT ( 'NONE',  ( 33.58253175000000823, 34.27500000273116854, 10.91162601494192863 ) ) ;
#15274=CARTESIAN_POINT ( 'NONE',  ( -32.50000000000000000, 44.40000000546238823, -10.55989012756945478 ) ) ;
#15276=CARTESIAN_POINT ( 'NONE',  ( -10.37757302488623701, 23.52500000273119340, 31.93888565452638417 ) ) ;
#15278=CARTESIAN_POINT ( 'NONE',  ( -10.37757302488623701, 51.77500000273118985, 31.93888565452638417 ) ) ;
#15281=CARTESIAN_POINT ( 'NONE',  ( -26.29305231718578995, 30.20000000000000284, 19.10302069950538595 ) ) ;
#15283=CARTESIAN_POINT ( 'NONE',  ( 33.58253175000000823, 68.02500000273117564, 10.91162601494192863 ) ) ;
#15286=CARTESIAN_POINT ( 'NONE',  ( 33.58253175000000113, 60.47500000273118559, -10.91162601494193574 ) ) ;
#15288=CARTESIAN_POINT ( 'NONE',  ( 20.08610463437157279, 39.80000000546238681, -27.64615127144129758 ) ) ;
#15289=CARTESIAN_POINT ( 'NONE',  ( 20.75514604977249178, 17.82500000273120122, 28.56700777964553950 ) ) ;
#15290=CARTESIAN_POINT ( 'NONE',  ( -4.732186688966233175E-15, 9.249999994537640546, 25.76082449383753925 ) ) ;
#15292=DIRECTION ( 'NONE',  ( -0.000000000000000000, -1.000000000000000000, -0.000000000000000000 ) ) ;
#15297=DIRECTION ( 'NONE',  ( 1.000000000000000000, 0.000000000000000000, 0.000000000000000000 ) ) ;
#15302=CARTESIAN_POINT ( 'NONE',  ( -1.778240108872766143E-15, 33.50000000000000000, -32.49999999999999289 ) ) ;
#15304=CARTESIAN_POINT ( 'NONE',  ( -18.94512977948575738, 1.924999997268805885, -13.76444248337723231 ) ) ;
#15305=CARTESIAN_POINT ( 'NONE',  ( 26.29305231718579350, 75.30000000546237970, 19.10302069950537529 ) ) ;
#15310=CARTESIAN_POINT ( 'NONE',  ( 27.16883889988623935, 76.57500000273120122, -19.73931689729374384 ) ) ;
#15314=CARTESIAN_POINT ( 'NONE',  ( -20.75514604977248823, 53.07500000273118701, -28.56700777964554305 ) ) ;
#15315=CARTESIAN_POINT ( 'NONE',  ( -10.04305231718579172, 64.10000000546240528, -30.90933677959248982 ) ) ;
#15317=VERTEX_POINT ( 'NONE', #26041 ) ;
#15319=CARTESIAN_POINT ( 'NONE',  ( 20.75514604977249178, 43.82500000273119412, 28.56700777964553950 ) ) ;
#15320=DIRECTION ( 'NONE',  ( 0.000000000000000000, 0.000000000000000000, -1.000000000000000000 ) ) ;
#15321=CARTESIAN_POINT ( 'NONE',  ( 20.75514604977249178, 66.07500000273118701, 28.56700777964553950 ) ) ;
#15322=EDGE_CURVE ( 'NONE', #27023, #25888, #20106, .T. ) ;
#15323=CARTESIAN_POINT ( 'NONE',  ( -32.50000000000000000, 4.400000005462393560, -10.55989012756945478 ) ) ;
#15325=FACE_OUTER_BOUND ( 'NONE', #21891, .T. ) ;
#15326=CARTESIAN_POINT ( 'NONE',  ( 32.50000000000000711, 44.90000000000001279, 10.55989012756945122 ) ) ;
#15327=CARTESIAN_POINT ( 'NONE',  ( -1.778240108872766143E-15, 13.50000000000000355, -32.49999999999999289 ) ) ;
#15328=CARTESIAN_POINT ( 'NONE',  ( -10.37757302488624411, 14.97500000273119269, -31.93888565452638417 ) ) ;
#15329=CARTESIAN_POINT ( 'NONE',  ( 5.779280353836490358E-15, 74.50000000000001421, 32.49999999999999289 ) ) ;
#15331=CARTESIAN_POINT ( 'NONE',  ( -8.601468415847515203, 79.67500000273118133, 11.83890561707634959 ) ) ;
#15333=CARTESIAN_POINT ( 'NONE',  ( -5.147494310547423346, 22.44874571845314648, 32.50000000000000000 ) ) ;
#15347=CARTESIAN_POINT ( 'NONE',  ( -8.601468415847515203, 71.67500000273118133, 11.83890561707634959 ) ) ;
#15349=CARTESIAN_POINT ( 'NONE',  ( 33.58253175000000823, 46.02500000273118275, 10.91162601494192685 ) ) ;
#15357=CARTESIAN_POINT ( 'NONE',  ( -2.162160676586881955E-15, 78.87500000273118417, -35.31076352940723240 ) ) ;
#15358=ORIENTED_EDGE ( 'NONE', *, *, #11041, .T. ) ;
#15361=EDGE_CURVE ( 'NONE', #25643, #12120, #26213, .T. ) ;
#15364=CARTESIAN_POINT ( 'NONE',  ( -2.162160676586881955E-15, 62.62500000273116996, -35.31076352940723240 ) ) ;
#15368=CARTESIAN_POINT ( 'NONE',  ( 33.58253175000000113, 8.225000002731182036, -10.91162601494193751 ) ) ;
#15370=CARTESIAN_POINT ( 'NONE',  ( 9.270509831248425314, 76.70000000000000284, 12.75976212528059683 ) ) ;
#15375=CARTESIAN_POINT ( 'NONE',  ( -15.00000000000000000, 74.15000000546237402, -4.873795443493594171 ) ) ;
#15377=CARTESIAN_POINT ( 'NONE',  ( -20.75514604977248112, 33.42500000273120264, 28.56700777964554661 ) ) ;
#15381=CARTESIAN_POINT ( 'NONE',  ( -2.162160676586882350E-15, 24.87500000273117706, -35.31076352940722529 ) ) ;
#15382=CARTESIAN_POINT ( 'NONE',  ( -4.635254915624211769, 79.60000000000000853, -14.26584774442730286 ) ) ;
#15383=CARTESIAN_POINT ( 'NONE',  ( 10.37757302488624056, 74.52500000273118985, -31.93888565452638417 ) ) ;
#15384=CARTESIAN_POINT ( 'NONE',  ( 32.50000000000000000, 59.60000000546236976, -10.55989012756945833 ) ) ;
#15386=CARTESIAN_POINT ( 'NONE',  ( -14.47279130897151767, 17.32499999726882578, -19.92008829642072598 ) ) ;
#15387=CARTESIAN_POINT ( 'NONE',  ( 33.58253175000000113, 62.22500000273119269, -10.91162601494193574 ) ) ;
#15390=CARTESIAN_POINT ( 'NONE',  ( -20.75514604977248112, 7.425000002731177773, 28.56700777964554661 ) ) ;
#15391=CARTESIAN_POINT ( 'NONE',  ( 18.94512977948575738, 18.92499999726882010, 13.76444248337723408 ) ) ;
#15393=VERTEX_POINT ( 'NONE', #23815 ) ;
#15395=( BOUNDED_CURVE ( )  B_SPLINE_CURVE ( 2, ( #24671, #5820, #981, #8384, #9054, #29814, #21611, #488, #32228, #1145, #16793, #24181, #8717 ),
 .UNSPECIFIED., .F., .T. ) 
 B_SPLINE_CURVE_WITH_KNOTS ( ( 3, 2, 2, 2, 2, 2, 3 ),
 ( 0.5833333333333332593, 0.5888888888888889062, 0.5999999999999999778, 0.6111111111111111605, 0.6222222222222222321, 0.6333333333333333037, 0.6388888888888889506 ),
 .UNSPECIFIED. ) 
 CURVE ( )  GEOMETRIC_REPRESENTATION_ITEM ( )  RATIONAL_B_SPLINE_CURVE ( ( 0.9755282581475768211, 0.9755282581475765991, 1.000000000000000000, 0.9510565162951535312, 1.000000000000000000, 0.9510565162951535312, 1.000000000000000000, 0.9510565162951535312, 1.000000000000000000, 0.9510565162951535312, 1.000000000000000000, 0.9755282581475765991, 0.9755282581475768211 ) ) 
 REPRESENTATION_ITEM ( '' )  );
#15400=CARTESIAN_POINT ( 'NONE',  ( -32.50000000000000000, 72.09999999999999432, 10.55989012756946366 ) ) ;
#15401=CARTESIAN_POINT ( 'NONE',  ( 18.94512977948576093, 3.324999997268818230, -13.76444248337722875 ) ) ;
#15402=CARTESIAN_POINT ( 'NONE',  ( 18.94512977948575738, 12.42499999726881477, 13.76444248337723408 ) ) ;
#15403=CARTESIAN_POINT ( 'NONE',  ( -33.58253175000000113, 15.47500000273118381, 10.91162601494193929 ) ) ;
#15404=CARTESIAN_POINT ( 'NONE',  ( -10.04305231718578462, 18.90000000546238113, 30.90933677959249337 ) ) ;
#15405=CARTESIAN_POINT ( 'NONE',  ( 20.08610463437157279, 63.30000000000001137, -27.64615127144129758 ) ) ;
#15407=CYLINDRICAL_SURFACE ( 'NONE', #1684, 24.50000000000000000 ) ;
#15408=VECTOR ( 'NONE', #3212, 1000.000000000000000 ) ;
#15410=CARTESIAN_POINT ( 'NONE',  ( -10.04305231718579172, 32.10000000546236976, -30.90933677959248982 ) ) ;
#15413=DIRECTION ( 'NONE',  ( 0.000000000000000000, 0.000000000000000000, 1.000000000000000000 ) ) ;
#15414=CARTESIAN_POINT ( 'NONE',  ( 23.41746825000000243, 17.22499999726880304, -7.608796670333727974 ) ) ;
#15415=CARTESIAN_POINT ( 'NONE',  ( 10.04305231718578817, 11.39999999999999325, -30.90933677959249337 ) ) ;
#15416=CARTESIAN_POINT ( 'NONE',  ( -12.13525491562421088, 73.80000000000001137, -8.816778784387096835 ) ) ;
#15418=CARTESIAN_POINT ( 'NONE',  ( 33.58253175000000113, 52.12500000273118417, -4.112674001490185761E-15 ) ) ;
#15420=CARTESIAN_POINT ( 'NONE',  ( -33.58253175000000113, 39.47500000273117848, 10.91162601494193929 ) ) ;
#15423=CARTESIAN_POINT ( 'NONE',  ( -20.08610463437156923, 62.29999999999998295, 27.64615127144130113 ) ) ;
#15424=CARTESIAN_POINT ( 'NONE',  ( -26.29305231718579350, 22.30000000546239391, -19.10302069950537884 ) ) ;
#15432=CARTESIAN_POINT ( 'NONE',  ( 7.890940483122900408E-14, 18.24999999453761745, -24.50000000000000000 ) ) ;
#15433=CARTESIAN_POINT ( 'NONE',  ( 6.486482029760648627E-15, 23.62500000273119127, 35.31076352940722529 ) ) ;
#15434=VECTOR ( 'NONE', #29433, 1000.000000000000000 ) ;
#15436=ORIENTED_EDGE ( 'NONE', *, *, #27277, .F. ) ;
#15446=CARTESIAN_POINT ( 'NONE',  ( 20.75514604977248467, 36.67500000273118843, -28.56700777964554305 ) ) ;
#15447=CARTESIAN_POINT ( 'NONE',  ( -32.50000000000000000, 38.40000000546235981, -10.55989012756945478 ) ) ;
#15449=CARTESIAN_POINT ( 'NONE',  ( -32.50000000000000000, 48.09999999999998721, 10.55989012756946366 ) ) ;
#15450=CARTESIAN_POINT ( 'NONE',  ( -33.58253175000000113, 25.22500000273119625, 10.91162601494193929 ) ) ;
#15451=CARTESIAN_POINT ( 'NONE',  ( 8.891200544363830713E-16, 79.75000000546236834, -15.00000000000000000 ) ) ;
#15452=CARTESIAN_POINT ( 'NONE',  ( -33.58253175000000113, 51.27500000273118275, -10.91162601494193218 ) ) ;
#15455=CARTESIAN_POINT ( 'NONE',  ( -32.50000000000000000, 28.10000000000001208, 10.55989012756946366 ) ) ;
#15457=CARTESIAN_POINT ( 'NONE',  ( 20.75514604977249178, 67.82500000273120122, 28.56700777964553950 ) ) ;
#15458=CARTESIAN_POINT ( 'NONE',  ( -26.29305231718578995, 78.19999999999998863, 19.10302069950538595 ) ) ;
#15460=CARTESIAN_POINT ( 'NONE',  ( -10.04305231718578462, 38.39999999999999147, 30.90933677959249337 ) ) ;
#15461=CARTESIAN_POINT ( 'NONE',  ( 27.16883889988624290, 62.17500000273118133, 19.73931689729373673 ) ) ;
#15462=ADVANCED_FACE ( 'NONE', ( #13167 ), #23645, .F. ) ;
#15464=CARTESIAN_POINT ( 'NONE',  ( 32.50000000000000000, 39.60000000546235555, -10.55989012756945833 ) ) ;
#15465=CARTESIAN_POINT ( 'NONE',  ( 33.58253175000000823, 14.02500000273117209, 10.91162601494192863 ) ) ;
#15470=FACE_OUTER_BOUND ( 'NONE', #16883, .T. ) ;
#15471=ADVANCED_FACE ( 'NONE', ( #29448 ), #3216, .F. ) ;
#15478=CARTESIAN_POINT ( 'NONE',  ( 10.04305231718578817, 63.90000000546236691, -30.90933677959249337 ) ) ;
#15479=CARTESIAN_POINT ( 'NONE',  ( 32.50000000000000711, 73.40000000546234560, 10.55989012756945122 ) ) ;
#15484=CARTESIAN_POINT ( 'NONE',  ( -33.58253175000000113, 73.37500000273116996, 0.000000000000000000 ) ) ;
#15488=CARTESIAN_POINT ( 'NONE',  ( -33.58253175000000113, 55.27500000273120406, -10.91162601494193218 ) ) ;
#15489=CARTESIAN_POINT ( 'NONE',  ( 20.08610463437158344, 55.20000000546238539, 27.64615127144129403 ) ) ;
#15491=CARTESIAN_POINT ( 'NONE',  ( -33.58253175000000113, 41.12500000273119838, 0.000000000000000000 ) ) ;
#15492=CARTESIAN_POINT ( 'NONE',  ( -9.270509831248419985, 72.30000000000001137, 12.75976212528060039 ) ) ;
#15493=CARTESIAN_POINT ( 'NONE',  ( -33.58253175000000113, 67.47500000273117848, 10.91162601494193929 ) ) ;
#15494=CARTESIAN_POINT ( 'NONE',  ( 10.04305231718579705, 5.100000005462374197, 30.90933677959248982 ) ) ;
#15496=CARTESIAN_POINT ( 'NONE',  ( 18.94512977948575738, 18.92499999726882010, 13.76444248337723408 ) ) ;
#15497=CARTESIAN_POINT ( 'NONE',  ( -20.08610463437156923, 46.29999999999999716, 27.64615127144130113 ) ) ;
#15499=CARTESIAN_POINT ( 'NONE',  ( 27.16883889988624290, 10.17500000273119376, 19.73931689729373673 ) ) ;
#15503=CARTESIAN_POINT ( 'NONE',  ( -4.300734207923755825, 71.27500000273117564, 13.23629886949340673 ) ) ;
#15504=CARTESIAN_POINT ( 'NONE',  ( -27.16883889988624290, 79.17500000273119554, -19.73931689729374028 ) ) ;
#15505=FACE_OUTER_BOUND ( 'NONE', #12854, .T. ) ;
#15507=AXIS2_PLACEMENT_3D ( 'NONE', #4366, #12436, #22906 ) ;
#15509=ORIENTED_EDGE ( 'NONE', *, *, #7163, .F. ) ;
#15513=( BOUNDED_CURVE ( )  B_SPLINE_CURVE ( 2, ( #17549, #6561, #11704, #12041, #22187, #4494, #29892, #32963, #27839, #30056, #14970, #4323, #17036 ),
 .UNSPECIFIED., .F., .T. ) 
 B_SPLINE_CURVE_WITH_KNOTS ( ( 3, 2, 2, 2, 2, 2, 3 ),
 ( 0.3012820512820512664, 0.3025641025641025439, 0.3051282051282051544, 0.3076923076923077094, 0.3102564102564102644, 0.3128205128205128194, 0.3141025641025640969 ),
 .UNSPECIFIED. ) 
 CURVE ( )  GEOMETRIC_REPRESENTATION_ITEM ( )  RATIONAL_B_SPLINE_CURVE ( ( 0.9755282581475768211, 0.9755282581475768211, 1.000000000000000000, 0.9510565162951535312, 1.000000000000000000, 0.9510565162951535312, 1.000000000000000000, 0.9510565162951535312, 1.000000000000000000, 0.9510565162951535312, 1.000000000000000000, 0.9755282581475768211, 0.9755282581475768211 ) ) 
 REPRESENTATION_ITEM ( '' )  );
#15522=FACE_OUTER_BOUND ( 'NONE', #13629, .T. ) ;
#15523=CARTESIAN_POINT ( 'NONE',  ( 33.58253175000000113, 44.12500000273117706, -4.112674001490185761E-15 ) ) ;
#15525=CARTESIAN_POINT ( 'NONE',  ( 9.270509831248425314, 78.69999999999998863, 12.75976212528059683 ) ) ;
#15526=VERTEX_POINT ( 'NONE', #32518 ) ;
#15530=CARTESIAN_POINT ( 'NONE',  ( 6.486482029760649416E-15, 73.87500000273119838, 35.31076352940723240 ) ) ;
#15537=CARTESIAN_POINT ( 'NONE',  ( -33.58253175000000113, 63.02500000273118985, -10.91162601494193218 ) ) ;
#15539=CARTESIAN_POINT ( 'NONE',  ( 7.570916362186207671, 17.60000000000000497, 23.30088464923126779 ) ) ;
#15540=CARTESIAN_POINT ( 'NONE',  ( 1.507698388325705758E-15, 5.624999997268818497, -24.62258325217400312 ) ) ;
#15541=CARTESIAN_POINT ( 'NONE',  ( 27.16883889988623935, 4.325000002731171911, -19.73931689729374384 ) ) ;
#15542=CARTESIAN_POINT ( 'NONE',  ( -19.82091636218621034, 6.549999994537619941, -14.40073868116559552 ) ) ;
#15544=CARTESIAN_POINT ( 'NONE',  ( -2.162160676586881955E-15, 78.87500000273118417, -35.31076352940723240 ) ) ;
#15546=CARTESIAN_POINT ( 'NONE',  ( -32.50000000000000000, 70.00000000000000000, 0.000000000000000000 ) ) ;
#15550=CARTESIAN_POINT ( 'NONE',  ( -4.300734207923759378, 80.47500000273119269, -13.23629886949340495 ) ) ;
#15552=CARTESIAN_POINT ( 'NONE',  ( -33.58253175000000113, 33.02500000273118275, -10.91162601494193218 ) ) ;
#15553=CYLINDRICAL_SURFACE ( 'NONE', #29201, 32.50000000000000000 ) ;
#15555=CARTESIAN_POINT ( 'NONE',  ( 27.16883889988623935, 20.57500000273118701, -19.73931689729374384 ) ) ;
#15556=CARTESIAN_POINT ( 'NONE',  ( -9.270509831248419985, 80.29999999999999716, 12.75976212528060039 ) ) ;
#15558=AXIS2_PLACEMENT_3D ( 'NONE', #24692, #8400, #3764 ) ;
#15559=CARTESIAN_POINT ( 'NONE',  ( -33.58253175000000113, 77.22500000273117848, 10.91162601494193929 ) ) ;
#15563=CARTESIAN_POINT ( 'NONE',  ( -14.47279130897152299, 17.92499999726880588, 19.92008829642072243 ) ) ;
#15564=CARTESIAN_POINT ( 'NONE',  ( -10.37757302488624411, 62.72500000273117848, -31.93888565452638417 ) ) ;
#15565=EDGE_CURVE ( 'NONE', #9328, #30741, #12274, .T. ) ;
#15568=CARTESIAN_POINT ( 'NONE',  ( 33.58253175000000113, 6.125000002731195714, -4.112674001490185761E-15 ) ) ;
#15569=CARTESIAN_POINT ( 'NONE',  ( 23.41746825000000243, 17.02499999726880731, 7.608796670333735079 ) ) ;
#15571=EDGE_LOOP ( 'NONE', ( #19191, #30348, #32545, #25609, #18819, #16074, #5808, #31446, #14166, #19030, #29304, #16416, #13667, #13259, #25562, #29227, #16207, #18951, #28219, #19477, #29054, #28932 ) ) ;
#15577=CARTESIAN_POINT ( 'NONE',  ( -1.778240108872766143E-15, 28.00000000546237544, -32.49999999999999289 ) ) ;
#15579=CARTESIAN_POINT ( 'NONE',  ( 14.47279130897151767, 5.424999997268823648, -19.92008829642072598 ) ) ;
#15580=AXIS2_PLACEMENT_3D ( 'NONE', #28, #2627, #3132 ) ;
#15581=CARTESIAN_POINT ( 'NONE',  ( -18.94512977948575738, 17.42499999726882010, -13.76444248337723231 ) ) ;
#15582=CARTESIAN_POINT ( 'NONE',  ( 10.37757302488624056, 18.77500000273118985, -31.93888565452638417 ) ) ;
#15583=CARTESIAN_POINT ( 'NONE',  ( -32.50000000000000000, 64.10000000000000853, 10.55989012756946366 ) ) ;
#15585=CARTESIAN_POINT ( 'NONE',  ( 0.000000000000000000, 0.000000000000000000, 0.000000000000000000 ) ) ;
#15587=CARTESIAN_POINT ( 'NONE',  ( 13.91746824999999887, 76.37500000273116996, -1.704398294459741270E-15 ) ) ;
#15590=CARTESIAN_POINT ( 'NONE',  ( 18.94512977948575738, 18.92499999726882010, 13.76444248337723408 ) ) ;
#15591=CARTESIAN_POINT ( 'NONE',  ( 10.04305231718578817, 5.400000000000016342, -30.90933677959249337 ) ) ;
#15594=CARTESIAN_POINT ( 'NONE',  ( -10.37757302488623701, 51.52500000273118985, 31.93888565452638417 ) ) ;
#15596=CARTESIAN_POINT ( 'NONE',  ( -27.16883889988623935, 43.57500000273117990, 19.73931689729374739 ) ) ;
#15599=CARTESIAN_POINT ( 'NONE',  ( 4.023268246324634798E-14, 8.499999999999992895, -24.50000000000000355 ) ) ;
#15600=CARTESIAN_POINT ( 'NONE',  ( 26.29305231718579350, 51.30000000546236549, 19.10302069950537529 ) ) ;
#15603=FACE_OUTER_BOUND ( 'NONE', #16532, .T. ) ;
#15605=CARTESIAN_POINT ( 'NONE',  ( 24.50000000000000000, 11.90000000000000213, 7.960532557706212486 ) ) ;
#15610=( BOUNDED_CURVE ( )  B_SPLINE_CURVE ( 2, ( #25151, #6957, #17100, #20186, #12105, #6789, #25501, #22576, #1462, #4385, #11940, #9532, #27558 ),
 .UNSPECIFIED., .F., .F. ) 
 B_SPLINE_CURVE_WITH_KNOTS ( ( 3, 2, 2, 2, 2, 2, 3 ),
 ( 0.4935897435897436125, 0.4948717948717948900, 0.4974358974358974450, 0.5000000000000000000, 0.5025641025641025550, 0.5051282051282051100, 0.5064102564102563875 ),
 .UNSPECIFIED. ) 
 CURVE ( )  GEOMETRIC_REPRESENTATION_ITEM ( )  RATIONAL_B_SPLINE_CURVE ( ( 0.9755282581475768211, 0.9755282581475768211, 1.000000000000000000, 0.9510565162951535312, 1.000000000000000000, 0.9510565162951535312, 1.000000000000000000, 0.9510565162951535312, 1.000000000000000000, 0.9510565162951535312, 1.000000000000000000, 0.9755282581475768211, 0.9755282581475768211 ) ) 
 REPRESENTATION_ITEM ( '' )  );
#15611=CARTESIAN_POINT ( 'NONE',  ( -19.82091636218621034, 10.54999999453762349, -14.40073868116559552 ) ) ;
#15612=CARTESIAN_POINT ( 'NONE',  ( -10.37757302488624411, 28.72500000273120335, -31.93888565452638417 ) ) ;
#15614=VERTEX_POINT ( 'NONE', #30279 ) ;
#15617=ORIENTED_EDGE ( 'NONE', *, *, #9950, .F. ) ;
#15621=FACE_OUTER_BOUND ( 'NONE', #7960, .T. ) ;
#15622=CARTESIAN_POINT ( 'NONE',  ( -27.16883889988623935, 33.57500000273120122, 19.73931689729374739 ) ) ;
#15624=CARTESIAN_POINT ( 'NONE',  ( 6.277390505771533514E-15, 37.00000000546237544, 34.17252228774368916 ) ) ;
#15625=EDGE_CURVE ( 'NONE', #3936, #30562, #13793, .T. ) ;
#15628=CARTESIAN_POINT ( 'NONE',  ( 27.16883889988623935, 20.32500000273118701, -19.73931689729374384 ) ) ;
#15629=CARTESIAN_POINT ( 'NONE',  ( 0.000000000000000000, 0.000000000000000000, 26.50000000000000355 ) ) ;
#15630=CARTESIAN_POINT ( 'NONE',  ( -27.16883889988623935, 47.57500000273117990, 19.73931689729374739 ) ) ;
#15632=CARTESIAN_POINT ( 'NONE',  ( -20.08610463437157989, 27.69999999999999929, -27.64615127144129758 ) ) ;
#15634=CARTESIAN_POINT ( 'NONE',  ( -10.37757302488623701, 69.52500000273120406, 31.93888565452638417 ) ) ;
#15637=CARTESIAN_POINT ( 'NONE',  ( -27.16883889988623935, 57.57500000273119412, 19.73931689729374739 ) ) ;
#15639=CARTESIAN_POINT ( 'NONE',  ( -2.162160676586881955E-15, 14.62500000273118239, -35.31076352940723240 ) ) ;
#15642=CARTESIAN_POINT ( 'NONE',  ( -20.75514604977248112, 1.675000002731184212, 28.56700777964554661 ) ) ;
#15644=CARTESIAN_POINT ( 'NONE',  ( 10.04305231718579705, 45.10000000546238397, 30.90933677959248982 ) ) ;
#15645=LINE ( 'NONE', #25923, #16647 ) ;
#15653=FACE_OUTER_BOUND ( 'NONE', #29972, .T. ) ;
#15654=CARTESIAN_POINT ( 'NONE',  ( -10.04305231718579172, 72.10000000546237686, -30.90933677959248982 ) ) ;
#15661=EDGE_CURVE ( 'NONE', #10375, #4234, #26321, .T. ) ;
#15664=CARTESIAN_POINT ( 'NONE',  ( 20.75514604977248467, 54.67500000273119554, -28.56700777964554305 ) ) ;
#15665=CARTESIAN_POINT ( 'NONE',  ( 32.50000000000000000, 55.60000000546238397, -10.55989012756945833 ) ) ;
#15667=CARTESIAN_POINT ( 'NONE',  ( -33.58253175000000113, 41.02500000273118985, -10.91162601494193218 ) ) ;
#15669=CARTESIAN_POINT ( 'NONE',  ( 33.58253175000000113, 70.47500000273117848, -10.91162601494193751 ) ) ;
#15670=CARTESIAN_POINT ( 'NONE',  ( 32.50000000000000000, 1.600000005462365760, -10.55989012756945833 ) ) ;
#15674=( GEOMETRIC_REPRESENTATION_CONTEXT ( 3 ) GLOBAL_UNCERTAINTY_ASSIGNED_CONTEXT ( ( #23234 ) ) GLOBAL_UNIT_ASSIGNED_CONTEXT ( ( #9258, #1190, #1362 ) ) REPRESENTATION_CONTEXT ( 'NONE', 'WORKASPACE' ) );
#15675=CARTESIAN_POINT ( 'NONE',  ( 32.50000000000000000, 48.99999999999998579, -3.980102097228898626E-15 ) ) ;
#15677=CARTESIAN_POINT ( 'NONE',  ( -10.37757302488623701, 13.77500000273118630, 31.93888565452638417 ) ) ;
#15679=CARTESIAN_POINT ( 'NONE',  ( -4.300734207923755825, 79.77500000273118985, 13.23629886949340673 ) ) ;
#15680=CARTESIAN_POINT ( 'NONE',  ( 12.13525491562421088, 75.05000000546237970, 8.816778784387095058 ) ) ;
#15681=CYLINDRICAL_SURFACE ( 'NONE', #24812, 32.50000000000000000 ) ;
#15683=ORIENTED_EDGE ( 'NONE', *, *, #26732, .T. ) ;
#15694=CARTESIAN_POINT ( 'NONE',  ( -10.37757302488623701, 41.52500000273118275, 31.93888565452638417 ) ) ;
#15699=DIRECTION ( 'NONE',  ( -0.000000000000000000, -1.000000000000000000, -0.000000000000000000 ) ) ;
#15701=CARTESIAN_POINT ( 'NONE',  ( 33.58253175000000113, 76.47500000273117848, -10.91162601494193751 ) ) ;
#15702=VERTEX_POINT ( 'NONE', #15028 ) ;
#15705=EDGE_LOOP ( 'NONE', ( #24953, #5729, #23618, #27741 ) ) ;
#15706=CARTESIAN_POINT ( 'NONE',  ( -26.29305231718578995, 14.70000000546237118, 19.10302069950538595 ) ) ;
#15707=CARTESIAN_POINT ( 'NONE',  ( -20.75514604977248823, 60.82500000273121543, -28.56700777964554305 ) ) ;
#15709=( BOUNDED_CURVE ( )  B_SPLINE_CURVE ( 2, ( #19645, #22219, #17070, #7100, #20160, #22897, #17583, #4530, #7271, #28385, #28213, #1953, #12598 ),
 .UNSPECIFIED., .F., .T. ) 
 B_SPLINE_CURVE_WITH_KNOTS ( ( 3, 2, 2, 2, 2, 2, 3 ),
 ( 0.4679487179487179516, 0.4692307692307692291, 0.4717948717948717841, 0.4743589743589743390, 0.4769230769230769496, 0.4794871794871795045, 0.4807692307692307820 ),
 .UNSPECIFIED. ) 
 CURVE ( )  GEOMETRIC_REPRESENTATION_ITEM ( )  RATIONAL_B_SPLINE_CURVE ( ( 0.9755282581475768211, 0.9755282581475768211, 1.000000000000000000, 0.9510565162951535312, 1.000000000000000000, 0.9510565162951535312, 1.000000000000000000, 0.9510565162951535312, 1.000000000000000000, 0.9510565162951535312, 1.000000000000000000, 0.9755282581475768211, 0.9755282581475768211 ) ) 
 REPRESENTATION_ITEM ( '' )  );
#15711=CARTESIAN_POINT ( 'NONE',  ( 14.47279130897151944, 3.424999997268799667, -19.92008829642072598 ) ) ;
#15712=CARTESIAN_POINT ( 'NONE',  ( 20.75514604977249178, 3.825000002731174575, 28.56700777964553950 ) ) ;
#15713=( BOUNDED_CURVE ( )  B_SPLINE_CURVE ( 2, ( #2666, #28565, #29069, #10386, #7974, #21369, #18118, #31484, #24107, #10553, #2829, #33894, #575 ),
 .UNSPECIFIED., .F., .F. ) 
 B_SPLINE_CURVE_WITH_KNOTS ( ( 3, 2, 2, 2, 2, 2, 3 ),
 ( 0.9038461538461538547, 0.9051282051282051322, 0.9076923076923076872, 0.9102564102564102422, 0.9128205128205127972, 0.9153846153846153522, 0.9166666666666666297 ),
 .UNSPECIFIED. ) 
 CURVE ( )  GEOMETRIC_REPRESENTATION_ITEM ( )  RATIONAL_B_SPLINE_CURVE ( ( 0.9755282581475768211, 0.9755282581475768211, 1.000000000000000000, 0.9510565162951535312, 1.000000000000000000, 0.9510565162951535312, 1.000000000000000000, 0.9510565162951535312, 1.000000000000000000, 0.9510565162951535312, 1.000000000000000000, 0.9755282581475768211, 0.9755282581475768211 ) ) 
 REPRESENTATION_ITEM ( '' )  );
#15714=DIRECTION ( 'NONE',  ( -0.000000000000000000, -1.000000000000000000, -0.000000000000000000 ) ) ;
#15718=CARTESIAN_POINT ( 'NONE',  ( -26.29305231718579350, 69.79999999999999716, -19.10302069950537884 ) ) ;
#15722=CARTESIAN_POINT ( 'NONE',  ( -12.13525491562420910, 70.45000000546237118, 8.816778784387098611 ) ) ;
#15724=CARTESIAN_POINT ( 'NONE',  ( 10.37757302488624767, 29.72500000273120691, 31.93888565452638417 ) ) ;
#15727=CARTESIAN_POINT ( 'NONE',  ( -33.58253175000000113, 17.37500000273117706, 0.000000000000000000 ) ) ;
#15730=CARTESIAN_POINT ( 'NONE',  ( -27.16883889988624290, 74.92500000273119554, -19.73931689729374028 ) ) ;
#15731=CARTESIAN_POINT ( 'NONE',  ( -1.778240108872766143E-15, 65.50000000000000000, -32.49999999999999289 ) ) ;
#15733=CARTESIAN_POINT ( 'NONE',  ( 18.94512977948575738, 14.42499999726881654, 13.76444248337723408 ) ) ;
#15734=CARTESIAN_POINT ( 'NONE',  ( -27.16883889988624290, 62.92500000273118843, -19.73931689729374028 ) ) ;
#15737=CARTESIAN_POINT ( 'NONE',  ( 27.16883889988624290, 5.925000002731190207, 19.73931689729373673 ) ) ;
#15738=CARTESIAN_POINT ( 'NONE',  ( 14.47279130897151767, 0.9249999972688209837, -19.92008829642072598 ) ) ;
#15741=VECTOR ( 'NONE', #19731, 1000.000000000000000 ) ;
#15747=CARTESIAN_POINT ( 'NONE',  ( -26.29305231718578995, 72.19999999999998863, 19.10302069950538595 ) ) ;
#15749=CARTESIAN_POINT ( 'NONE',  ( 24.50000000000000000, 2.000000000000001776, 0.000000000000000000 ) ) ;
#15750=CARTESIAN_POINT ( 'NONE',  ( -33.58253175000000113, 13.47500000273118914, 10.91162601494193929 ) ) ;
#15752=CARTESIAN_POINT ( 'NONE',  ( -20.08610463437156923, 60.29999999999998295, 27.64615127144130113 ) ) ;
#15753=CARTESIAN_POINT ( 'NONE',  ( 1.555960095263670572E-15, 8.249999994537619230, -24.50000000000000000 ) ) ;
#15754=FACE_OUTER_BOUND ( 'NONE', #1641, .T. ) ;
#15756=CARTESIAN_POINT ( 'NONE',  ( -11.25946833292375793, 73.17500000273119554, -8.180482586598733619 ) ) ;
#15759=EDGE_CURVE ( 'NONE', #1581, #26581, #10081, .T. ) ;
#15761=CARTESIAN_POINT ( 'NONE',  ( -15.14183272437242067, 12.70000000000000639, -20.84094480462497856 ) ) ;
#15762=CARTESIAN_POINT ( 'NONE',  ( -20.75514604977248823, 79.07500000273121543, -28.56700777964554305 ) ) ;
#15765=CARTESIAN_POINT ( 'NONE',  ( -20.75514604977248112, 49.42500000273118133, 28.56700777964554661 ) ) ;
#15767=CARTESIAN_POINT ( 'NONE',  ( 27.16883889988623935, 34.57500000273120122, -19.73931689729374384 ) ) ;
#15768=VECTOR ( 'NONE', #25900, 1000.000000000000000 ) ;
#15770=CARTESIAN_POINT ( 'NONE',  ( -32.50000000000000000, 62.09999999999998721, 10.55989012756946366 ) ) ;
#15771=CARTESIAN_POINT ( 'NONE',  ( 0.000000000000000000, 0.000000000000000000, 0.000000000000000000 ) ) ;
#15772=CARTESIAN_POINT ( 'NONE',  ( -5.147494310547213736, 27.55125428154684997, -32.50000000000007105 ) ) ;
#15774=CARTESIAN_POINT ( 'NONE',  ( 5.334720326618300005E-14, 72.00000000546238255, -32.50000000000000000 ) ) ;
#15775=DIRECTION ( 'NONE',  ( 0.000000000000000000, -0.000000000000000000, -1.000000000000000000 ) ) ;
#15776=CARTESIAN_POINT ( 'NONE',  ( 3.880418787951153803, 9.301254276084472750, 24.49999999999999645 ) ) ;
#15779=DIRECTION ( 'NONE',  ( -0.000000000000000000, -1.000000000000000000, -0.000000000000000000 ) ) ;
#15780=CARTESIAN_POINT ( 'NONE',  ( 10.37757302488624767, 23.72500000273119980, 31.93888565452638417 ) ) ;
#15782=ORIENTED_EDGE ( 'NONE', *, *, #22470, .T. ) ;
#15789=DIRECTION ( 'NONE',  ( -0.8660254037844398178, 0.4999999999999979461, -0.000000000000000000 ) ) ;
#15790=CARTESIAN_POINT ( 'NONE',  ( -2.162160676586881955E-15, 32.87500000273118417, -35.31076352940723240 ) ) ;
#15791=CARTESIAN_POINT ( 'NONE',  ( 32.50000000000000000, 39.50000000546238965, -3.980102097228898626E-15 ) ) ;
#15794=PLANE ( 'NONE',  #15980 ) ;
#15795=CARTESIAN_POINT ( 'NONE',  ( 19.82091636218621034, 5.549999994537619052, 14.40073868116559730 ) ) ;
#15796=CARTESIAN_POINT ( 'NONE',  ( 27.16883889988624290, 48.17500000273117422, 19.73931689729373673 ) ) ;
#15798=CARTESIAN_POINT ( 'NONE',  ( 32.50000000000000000, 25.09999999999999432, -10.55989012756945833 ) ) ;
#15800=CARTESIAN_POINT ( 'NONE',  ( 20.75514604977249178, 71.82500000273118701, 28.56700777964553950 ) ) ;
#15803=CARTESIAN_POINT ( 'NONE',  ( 20.75514604977248467, 58.67500000273118843, -28.56700777964554305 ) ) ;
#15804=CARTESIAN_POINT ( 'NONE',  ( 20.08610463437157279, 73.29999999999996874, -27.64615127144129758 ) ) ;
#15805=CARTESIAN_POINT ( 'NONE',  ( 6.486482029760649416E-15, 13.62500000273118417, 35.31076352940723240 ) ) ;
#15807=( BOUNDED_CURVE ( )  B_SPLINE_CURVE ( 2, ( #8405, #16651, #10995, #29341, #26778, #32412, #24041, #21468, #29839, #16478, #3267, #674, #29500 ),
 .UNSPECIFIED., .F., .T. ) 
 B_SPLINE_CURVE_WITH_KNOTS ( ( 3, 2, 2, 2, 2, 2, 3 ),
 ( 0.3910256410256410242, 0.3923076923076923017, 0.3948717948717948567, 0.3974358974358974117, 0.4000000000000000222, 0.4025641025641025772, 0.4038461538461538547 ),
 .UNSPECIFIED. ) 
 CURVE ( )  GEOMETRIC_REPRESENTATION_ITEM ( )  RATIONAL_B_SPLINE_CURVE ( ( 0.9755282581475768211, 0.9755282581475768211, 1.000000000000000000, 0.9510565162951535312, 1.000000000000000000, 0.9510565162951535312, 1.000000000000000000, 0.9510565162951535312, 1.000000000000000000, 0.9510565162951535312, 1.000000000000000000, 0.9755282581475768211, 0.9755282581475768211 ) ) 
 REPRESENTATION_ITEM ( '' )  );
#15809=CARTESIAN_POINT ( 'NONE',  ( 6.486482029760648627E-15, 3.875000002731201931, 35.31076352940722529 ) ) ;
#15820=CARTESIAN_POINT ( 'NONE',  ( 18.94512977948576093, 3.324999997268818230, -13.76444248337722875 ) ) ;
#15821=CARTESIAN_POINT ( 'NONE',  ( -20.08610463437156923, 68.80000000546236549, 27.64615127144130113 ) ) ;
#15830=CARTESIAN_POINT ( 'NONE',  ( -33.58253175000000113, 53.47500000273117848, 10.91162601494193929 ) ) ;
#15831=CARTESIAN_POINT ( 'NONE',  ( -26.29305231718578995, 58.70000000546238539, 19.10302069950538595 ) ) ;
#15833=CARTESIAN_POINT ( 'NONE',  ( 33.58253175000000823, 42.02500000273118985, 10.91162601494192863 ) ) ;
#15834=CARTESIAN_POINT ( 'NONE',  ( 33.58253175000000113, 68.37500000273119838, -4.112674001490185761E-15 ) ) ;
#15838=CARTESIAN_POINT ( 'NONE',  ( 32.50000000000000711, 46.90000000000000568, 10.55989012756945122 ) ) ;
#15840=CARTESIAN_POINT ( 'NONE',  ( 27.16883889988623935, 8.575000002731202997, -19.73931689729374384 ) ) ;
#15843=CARTESIAN_POINT ( 'NONE',  ( 11.25946833292375793, 72.57500000273120122, -8.180482586598735395 ) ) ;
#15844=CARTESIAN_POINT ( 'NONE',  ( 27.16883889988624290, 78.17500000273119554, 19.73931689729373673 ) ) ;
#15845=DIRECTION ( 'NONE',  ( -0.000000000000000000, -1.000000000000000000, -0.000000000000000000 ) ) ;
#15847=EDGE_LOOP ( 'NONE', ( #11055, #435, #13327, #1350 ) ) ;
#15848=( BOUNDED_SURFACE ( )  B_SPLINE_SURFACE ( 1, 2, ( 
 ( #11137, #21606, #20937, #31386, #7876, #13197, #23674, #29142, #5646, #138, #10629, #26582, #482, #32049, #8550, #28639, #5135, #31550, #28979, #19528, #11622, #29809, #3739, #27580, #26907, #6137, #22105, #16955, #3904, #24666, #6310, #3571, #32550, #19195, #29978, #14210, #1310, #16455, #6483, #29634, #11297, #14544, #32713, #14042, #30139, #14373, #9210, #6643, #977, #9049, #24832, #1140, #17123, #27414, #11792, #19693, #22271, #3406, #4069, #25003, #1485, #19366, #22430, #11959, #32877, #19035, #29473, #816, #32385, #5978, #13878, #24345, #21776, #32223, #8712, #16622, #11461, #27076, #16788, #24503, #21935, #8880, #27246, #19857, #33227, #17806, #6981, #33405, #2171, #17631, #28432, #4922, #28264, #22775, #1651, #20212, #20034, #9726, #17984, #6809, #30480, #30828, #17464, #30652, #7322, #12477, #4750, #27751, #30312, #28092, #7149, #15227, #9556, #27924, #4581, #4407, #25171, #1825, #15402, #9902, #22598, #14884, #31003, #7500, #15058, #17288, #22947, #14713, #23115, #33052, #4239, #12126, #25345, #12303, #25525, #10077, #2002, #20379, #23293, #33578, #20557, #25690, #12644, #25858, #2347, #12822, #9376, #8173, #10418, #2864, #5094, #31516, #28938, #33927, #20895, #13333, #21067, #8010, #18495, #10253, #5437, #31344, #16091, #7666, #20734, #26542, #12994, #3037, #15581, #7836, #31176, #13510, #18153, #23973, #28595, #18829, #29274, #5775, #2698, #21237, #10926 ),
 ( #10589, #15918, #26374, #23807, #272, #26032, #2525, #443, #23634, #23465, #16255, #21400, #5267, #18326, #26711, #3208, #13676, #10759, #31846, #28771, #15749, #31680, #33761, #13158, #26204, #100, #18664, #29102, #5607, #8339, #19657, #1102, #13839, #29940, #6444, #16916, #3700, #24467, #8841, #24306, #21897, #8678, #6273, #32677, #9173, #19160, #11752, #3532, #32510, #29766, #24793, #942, #27037, #4030, #3865, #14337, #16750, #780, #32347, #9011, #29440, #1272, #19491, #11262, #27208, #5941, #19324, #14172, #21738, #32183, #24629, #11422, #11585, #22066, #607, #27376, #29599, #22233, #32013, #11099, #30100, #3369, #6606, #16422, #6101, #21568, #17083, #8509, #27543, #18996, #24140, #26874, #16582, #14004, #1965, #25655, #28225, #30789, #28054, #32843, #25310, #27886, #1783, #20171, #12260, #4542, #22737, #11924, #9335, #17765, #4369, #4202, #30964, #15192, #19996, #19820, #7463, #10042, #17946, #7110, #12609, #33010, #30444, #30614, #28395, #14844, #17253, #1446, #25486, #14674, #17592, #12440, #20519, #22910, #25134, #20339, #7282, #4711, #15016, #33187, #9690, #1611, #33366, #9515, #9862, #23078, #33539, #6942, #2134, #14505, #24964, #22394, #30272, #6772, #27714, #12089, #22558, #17425, #12953, #20696, #31303, #403, #5399, #18110, #5055, #26502, #2995, #28731, #25820, #7968, #10216, #18625, #28559, #2310, #12783, #31138, #15539, #21027, #13468, #23934, #33887 ) ),
 .UNSPECIFIED., .F., .F., .F. ) 
 B_SPLINE_SURFACE_WITH_KNOTS ( ( 2, 2 ),
 ( 3, 2, 2, 2, 2, 2, 2, 2, 2, 2, 2, 2, 2, 2, 2, 2, 2, 2, 2, 2, 2, 2, 2, 2, 2, 2, 2, 2, 2, 2, 2, 2, 2, 2, 2, 2, 2, 2, 2, 2, 2, 2, 2, 2, 2, 2, 2, 2, 2, 2, 2, 2, 2, 2, 2, 2, 2, 2, 2, 2, 2, 2, 2, 2, 2, 2, 2, 2, 2, 2, 2, 2, 2, 2, 2, 2, 2, 2, 2, 2, 2, 2, 2, 2, 2, 2, 2, 2, 2, 2, 3 ),
 ( 0.000000000000000000, 1.000000000000000000 ),
 ( 0.000000000000000000, 0.01111111111111111154, 0.02222222222222222307, 0.03333333333333333287, 0.04444444444444444614, 0.05555555555555555247, 0.06666666666666666574, 0.07777777777777777901, 0.08888888888888889228, 0.1000000000000000056, 0.1111111111111111049, 0.1222222222222222182, 0.1333333333333333315, 0.1444444444444444309, 0.1555555555555555580, 0.1666666666666666574, 0.1777777777777777846, 0.1888888888888888840, 0.2000000000000000111, 0.2111111111111111105, 0.2222222222222222099, 0.2333333333333333370, 0.2444444444444444364, 0.2555555555555555358, 0.2666666666666666630, 0.2777777777777777901, 0.2888888888888888618, 0.2999999999999999889, 0.3111111111111111160, 0.3222222222222222432, 0.3333333333333333148, 0.3444444444444444420, 0.3555555555555555691, 0.3666666666666666408, 0.3777777777777777679, 0.3888888888888888951, 0.4000000000000000222, 0.4111111111111110938, 0.4222222222222222210, 0.4333333333333333481, 0.4444444444444444198, 0.4555555555555555469, 0.4666666666666666741, 0.4777777777777778012, 0.4888888888888888729, 0.5000000000000000000, 0.5111111111111110716, 0.5222222222222222543, 0.5333333333333333259, 0.5444444444444443976, 0.5555555555555555802, 0.5666666666666666519, 0.5777777777777777235, 0.5888888888888889062, 0.5999999999999999778, 0.6111111111111111605, 0.6222222222222222321, 0.6333333333333333037, 0.6444444444444444864, 0.6555555555555555580, 0.6666666666666666297, 0.6777777777777778123, 0.6888888888888888840, 0.6999999999999999556, 0.7111111111111111382, 0.7222222222222222099, 0.7333333333333332815, 0.7444444444444444642, 0.7555555555555555358, 0.7666666666666667185, 0.7777777777777777901, 0.7888888888888888618, 0.8000000000000000444, 0.8111111111111111160, 0.8222222222222221877, 0.8333333333333333703, 0.8444444444444444420, 0.8555555555555555136, 0.8666666666666666963, 0.8777777777777777679, 0.8888888888888888395, 0.9000000000000000222, 0.9111111111111110938, 0.9222222222222222765, 0.9333333333333333481, 0.9444444444444444198, 0.9555555555555556024, 0.9666666666666666741, 0.9777777777777777457, 0.9888888888888889284, 1.000000000000000000 ),
 .UNSPECIFIED. ) 
 GEOMETRIC_REPRESENTATION_ITEM ( )  RATIONAL_B_SPLINE_SURFACE ( (
 ( 1.000000000000000000, 0.9510565162951535312, 1.000000000000000000, 0.9510565162951535312, 1.000000000000000000, 0.9510565162951535312, 1.000000000000000000, 0.9510565162951535312, 1.000000000000000000, 0.9510565162951535312, 1.000000000000000000, 0.9510565162951535312, 1.000000000000000000, 0.9510565162951535312, 1.000000000000000000, 0.9510565162951535312, 1.000000000000000000, 0.9510565162951535312, 1.000000000000000000, 0.9510565162951535312, 1.000000000000000000, 0.9510565162951535312, 1.000000000000000000, 0.9510565162951535312, 1.000000000000000000, 0.9510565162951535312, 1.000000000000000000, 0.9510565162951535312, 1.000000000000000000, 0.9510565162951535312, 1.000000000000000000, 0.9510565162951535312, 1.000000000000000000, 0.9510565162951535312, 1.000000000000000000, 0.9510565162951535312, 1.000000000000000000, 0.9510565162951535312, 1.000000000000000000, 0.9510565162951535312, 1.000000000000000000, 0.9510565162951535312, 1.000000000000000000, 0.9510565162951535312, 1.000000000000000000, 0.9510565162951535312, 1.000000000000000000, 0.9510565162951535312, 1.000000000000000000, 0.9510565162951535312, 1.000000000000000000, 0.9510565162951535312, 1.000000000000000000, 0.9510565162951535312, 1.000000000000000000, 0.9510565162951535312, 1.000000000000000000, 0.9510565162951535312, 1.000000000000000000, 0.9510565162951535312, 1.000000000000000000, 0.9510565162951535312, 1.000000000000000000, 0.9510565162951535312, 1.000000000000000000, 0.9510565162951535312, 1.000000000000000000, 0.9510565162951535312, 1.000000000000000000, 0.9510565162951535312, 1.000000000000000000, 0.9510565162951535312, 1.000000000000000000, 0.9510565162951535312, 1.000000000000000000, 0.9510565162951535312, 1.000000000000000000, 0.9510565162951535312, 1.000000000000000000, 0.9510565162951535312, 1.000000000000000000, 0.9510565162951535312, 1.000000000000000000, 0.9510565162951535312, 1.000000000000000000, 0.9510565162951535312, 1.000000000000000000, 0.9510565162951535312, 1.000000000000000000, 0.9510565162951535312, 1.000000000000000000, 0.9510565162951535312, 1.000000000000000000, 0.9510565162951535312, 1.000000000000000000, 0.9510565162951535312, 1.000000000000000000, 0.9510565162951535312, 1.000000000000000000, 0.9510565162951535312, 1.000000000000000000, 0.9510565162951535312, 1.000000000000000000, 0.9510565162951535312, 1.000000000000000000, 0.9510565162951535312, 1.000000000000000000, 0.9510565162951535312, 1.000000000000000000, 0.9510565162951535312, 1.000000000000000000, 0.9510565162951535312, 1.000000000000000000, 0.9510565162951535312, 1.000000000000000000, 0.9510565162951535312, 1.000000000000000000, 0.9510565162951535312, 1.000000000000000000, 0.9510565162951535312, 1.000000000000000000, 0.9510565162951535312, 1.000000000000000000, 0.9510565162951535312, 1.000000000000000000, 0.9510565162951535312, 1.000000000000000000, 0.9510565162951535312, 1.000000000000000000, 0.9510565162951535312, 1.000000000000000000, 0.9510565162951535312, 1.000000000000000000, 0.9510565162951535312, 1.000000000000000000, 0.9510565162951535312, 1.000000000000000000, 0.9510565162951535312, 1.000000000000000000, 0.9510565162951535312, 1.000000000000000000, 0.9510565162951535312, 1.000000000000000000, 0.9510565162951535312, 1.000000000000000000, 0.9510565162951535312, 1.000000000000000000, 0.9510565162951535312, 1.000000000000000000, 0.9510565162951535312, 1.000000000000000000, 0.9510565162951535312, 1.000000000000000000, 0.9510565162951535312, 1.000000000000000000, 0.9510565162951535312, 1.000000000000000000, 0.9510565162951535312, 1.000000000000000000, 0.9510565162951535312, 1.000000000000000000, 0.9510565162951535312, 1.000000000000000000, 0.9510565162951535312, 1.000000000000000000, 0.9510565162951535312, 1.000000000000000000, 0.9510565162951535312, 1.000000000000000000, 0.9510565162951535312, 1.000000000000000000, 0.9510565162951535312, 1.000000000000000000, 0.9510565162951535312, 1.000000000000000000, 0.9510565162951535312, 1.000000000000000000, 0.9510565162951535312, 1.000000000000000000, 0.9510565162951535312, 1.000000000000000000),
 ( 1.000000000000000000, 0.9510565162951535312, 1.000000000000000000, 0.9510565162951535312, 1.000000000000000000, 0.9510565162951535312, 1.000000000000000000, 0.9510565162951535312, 1.000000000000000000, 0.9510565162951535312, 1.000000000000000000, 0.9510565162951535312, 1.000000000000000000, 0.9510565162951535312, 1.000000000000000000, 0.9510565162951535312, 1.000000000000000000, 0.9510565162951535312, 1.000000000000000000, 0.9510565162951535312, 1.000000000000000000, 0.9510565162951535312, 1.000000000000000000, 0.9510565162951535312, 1.000000000000000000, 0.9510565162951535312, 1.000000000000000000, 0.9510565162951535312, 1.000000000000000000, 0.9510565162951535312, 1.000000000000000000, 0.9510565162951535312, 1.000000000000000000, 0.9510565162951535312, 1.000000000000000000, 0.9510565162951535312, 1.000000000000000000, 0.9510565162951535312, 1.000000000000000000, 0.9510565162951535312, 1.000000000000000000, 0.9510565162951535312, 1.000000000000000000, 0.9510565162951535312, 1.000000000000000000, 0.9510565162951535312, 1.000000000000000000, 0.9510565162951535312, 1.000000000000000000, 0.9510565162951535312, 1.000000000000000000, 0.9510565162951535312, 1.000000000000000000, 0.9510565162951535312, 1.000000000000000000, 0.9510565162951535312, 1.000000000000000000, 0.9510565162951535312, 1.000000000000000000, 0.9510565162951535312, 1.000000000000000000, 0.9510565162951535312, 1.000000000000000000, 0.9510565162951535312, 1.000000000000000000, 0.9510565162951535312, 1.000000000000000000, 0.9510565162951535312, 1.000000000000000000, 0.9510565162951535312, 1.000000000000000000, 0.9510565162951535312, 1.000000000000000000, 0.9510565162951535312, 1.000000000000000000, 0.9510565162951535312, 1.000000000000000000, 0.9510565162951535312, 1.000000000000000000, 0.9510565162951535312, 1.000000000000000000, 0.9510565162951535312, 1.000000000000000000, 0.9510565162951535312, 1.000000000000000000, 0.9510565162951535312, 1.000000000000000000, 0.9510565162951535312, 1.000000000000000000, 0.9510565162951535312, 1.000000000000000000, 0.9510565162951535312, 1.000000000000000000, 0.9510565162951535312, 1.000000000000000000, 0.9510565162951535312, 1.000000000000000000, 0.9510565162951535312, 1.000000000000000000, 0.9510565162951535312, 1.000000000000000000, 0.9510565162951535312, 1.000000000000000000, 0.9510565162951535312, 1.000000000000000000, 0.9510565162951535312, 1.000000000000000000, 0.9510565162951535312, 1.000000000000000000, 0.9510565162951535312, 1.000000000000000000, 0.9510565162951535312, 1.000000000000000000, 0.9510565162951535312, 1.000000000000000000, 0.9510565162951535312, 1.000000000000000000, 0.9510565162951535312, 1.000000000000000000, 0.9510565162951535312, 1.000000000000000000, 0.9510565162951535312, 1.000000000000000000, 0.9510565162951535312, 1.000000000000000000, 0.9510565162951535312, 1.000000000000000000, 0.9510565162951535312, 1.000000000000000000, 0.9510565162951535312, 1.000000000000000000, 0.9510565162951535312, 1.000000000000000000, 0.9510565162951535312, 1.000000000000000000, 0.9510565162951535312, 1.000000000000000000, 0.9510565162951535312, 1.000000000000000000, 0.9510565162951535312, 1.000000000000000000, 0.9510565162951535312, 1.000000000000000000, 0.9510565162951535312, 1.000000000000000000, 0.9510565162951535312, 1.000000000000000000, 0.9510565162951535312, 1.000000000000000000, 0.9510565162951535312, 1.000000000000000000, 0.9510565162951535312, 1.000000000000000000, 0.9510565162951535312, 1.000000000000000000, 0.9510565162951535312, 1.000000000000000000, 0.9510565162951535312, 1.000000000000000000, 0.9510565162951535312, 1.000000000000000000, 0.9510565162951535312, 1.000000000000000000, 0.9510565162951535312, 1.000000000000000000, 0.9510565162951535312, 1.000000000000000000, 0.9510565162951535312, 1.000000000000000000, 0.9510565162951535312, 1.000000000000000000, 0.9510565162951535312, 1.000000000000000000, 0.9510565162951535312, 1.000000000000000000, 0.9510565162951535312, 1.000000000000000000, 0.9510565162951535312, 1.000000000000000000, 0.9510565162951535312, 1.000000000000000000) ) ) 
 REPRESENTATION_ITEM ( '' )  SURFACE ( )  );
#15859=CARTESIAN_POINT ( 'NONE',  ( -33.58253175000000113, 37.02500000273116854, -10.91162601494193041 ) ) ;
#15862=CARTESIAN_POINT ( 'NONE',  ( -10.04305231718578462, 2.900000005462366470, 30.90933677959249337 ) ) ;
#15867=CARTESIAN_POINT ( 'NONE',  ( -20.75514604977248823, 71.07500000273117280, -28.56700777964554305 ) ) ;
#15871=EDGE_LOOP ( 'NONE', ( #21495, #25163, #32628, #9642 ) ) ;
#15872=CARTESIAN_POINT ( 'NONE',  ( 3.980102097228898626E-15, 80.00000000000001421, 32.50000000000000000 ) ) ;
#15873=CARTESIAN_POINT ( 'NONE',  ( -33.58253175000000113, 63.22500000273119269, 10.91162601494193929 ) ) ;
#15876=CARTESIAN_POINT ( 'NONE',  ( -7.236395654485757944, 5.724999997268803931, -22.27133577429736988 ) ) ;
#15877=CARTESIAN_POINT ( 'NONE',  ( 6.486482029760649416E-15, 1.625000002731185944, 35.31076352940723240 ) ) ;
#15878=CARTESIAN_POINT ( 'NONE',  ( -33.58253175000000113, 31.37500000273119127, 0.000000000000000000 ) ) ;
#15882=CARTESIAN_POINT ( 'NONE',  ( 8.601468415847516980, 78.17500000273118133, -11.83890561707634781 ) ) ;
#15883=CARTESIAN_POINT ( 'NONE',  ( 5.147494310547434893, 75.05125428700921475, 32.49999999999999289 ) ) ;
#15884=EDGE_CURVE ( 'NONE', #25987, #1179, #4358, .T. ) ;
#15888=CARTESIAN_POINT ( 'NONE',  ( -9.270509831248421762, 72.55000000546236549, 12.75976212528060039 ) ) ;
#15890=CARTESIAN_POINT ( 'NONE',  ( 10.37757302488624767, 25.72500000273120335, 31.93888565452638417 ) ) ;
#15893=CARTESIAN_POINT ( 'NONE',  ( 27.16883889988624290, 14.17500000273119731, 19.73931689729373673 ) ) ;
#15894=CARTESIAN_POINT ( 'NONE',  ( -32.50000000000000000, 64.10000000000000853, 10.55989012756946366 ) ) ;
#15896=CARTESIAN_POINT ( 'NONE',  ( -10.37757302488624411, 76.72500000273119269, -31.93888565452638417 ) ) ;
#15898=FACE_OUTER_BOUND ( 'NONE', #9944, .T. ) ;
#15900=CARTESIAN_POINT ( 'NONE',  ( 5.779280353836490358E-15, 26.50000000000000711, 32.49999999999999289 ) ) ;
#15901=CARTESIAN_POINT ( 'NONE',  ( 6.486482029760648627E-15, 55.62500000273119838, 35.31076352940722529 ) ) ;
#15906=CARTESIAN_POINT ( 'NONE',  ( 7.236395654485760609, 1.024999997268821739, -22.27133577429736633 ) ) ;
#15908=( BOUNDED_CURVE ( )  B_SPLINE_CURVE ( 2, ( #30386, #1395, #14120, #11371, #6555, #9122, #27831, #1217, #22504, #29711, #22181, #24909, #32457 ),
 .UNSPECIFIED., .F., .F. ) 
 B_SPLINE_CURVE_WITH_KNOTS ( ( 3, 2, 2, 2, 2, 2, 3 ),
 ( 0.04487179487179487197, 0.04615384615384615641, 0.04871794871794871834, 0.05128205128205128027, 0.05384615384615384914, 0.05641025641025641107, 0.05769230769230769551 ),
 .UNSPECIFIED. ) 
 CURVE ( )  GEOMETRIC_REPRESENTATION_ITEM ( )  RATIONAL_B_SPLINE_CURVE ( ( 0.9755282581475768211, 0.9755282581475768211, 1.000000000000000000, 0.9510565162951535312, 1.000000000000000000, 0.9510565162951535312, 1.000000000000000000, 0.9510565162951535312, 1.000000000000000000, 0.9510565162951535312, 1.000000000000000000, 0.9755282581475767101, 0.9755282581475768211 ) ) 
 REPRESENTATION_ITEM ( '' )  );
#15909=ORIENTED_EDGE ( 'NONE', *, *, #14536, .T. ) ;
#15911=CARTESIAN_POINT ( 'NONE',  ( -10.04305231718578462, 16.90000000546237757, 30.90933677959249337 ) ) ;
#15916=CARTESIAN_POINT ( 'NONE',  ( -10.04305231718578462, 72.40000000000001990, 30.90933677959249337 ) ) ;
#15918=CARTESIAN_POINT ( 'NONE',  ( 24.50000000000000355, 0.09999999999999684142, -7.960532557706203605 ) ) ;
#15919=CARTESIAN_POINT ( 'NONE',  ( 33.58253175000000823, 12.27500000273116854, 10.91162601494192863 ) ) ;
#15920=CARTESIAN_POINT ( 'NONE',  ( 20.08610463437158344, 62.69999999999999574, 27.64615127144129403 ) ) ;
#15921=CARTESIAN_POINT ( 'NONE',  ( -13.91746824999999887, 80.87500000273118417, 0.000000000000000000 ) ) ;
#15924=CARTESIAN_POINT ( 'NONE',  ( -8.601468415847518756, 79.07500000273121543, -11.83890561707634781 ) ) ;
#15928=CARTESIAN_POINT ( 'NONE',  ( 26.29305231718578995, 65.20000000000000284, -19.10302069950538240 ) ) ;
#15929=CARTESIAN_POINT ( 'NONE',  ( 32.50000000000000000, 3.099999999999989875, -10.55989012756945833 ) ) ;
#15930=CARTESIAN_POINT ( 'NONE',  ( 5.779280353836490358E-15, 35.00000000546238255, 32.49999999999999289 ) ) ;
#15932=CARTESIAN_POINT ( 'NONE',  ( 6.486482029760649416E-15, 51.62500000273120548, 35.31076352940723240 ) ) ;
#15935=CARTESIAN_POINT ( 'NONE',  ( -27.16883889988623935, 31.57500000273119767, 19.73931689729374739 ) ) ;
#15936=FACE_OUTER_BOUND ( 'NONE', #31831, .T. ) ;
#15939=CARTESIAN_POINT ( 'NONE',  ( 26.29305231718578995, 51.70000000546237828, -19.10302069950538240 ) ) ;
#15942=CARTESIAN_POINT ( 'NONE',  ( -7.236395654485757944, 1.224999997268799712, -22.27133577429736988 ) ) ;
#15947=CARTESIAN_POINT ( 'NONE',  ( -32.50000000000000000, 12.00000000000001066, 0.000000000000000000 ) ) ;
#15948=CARTESIAN_POINT ( 'NONE',  ( 33.58253175000000113, 26.22500000273119625, -10.91162601494193574 ) ) ;
#15956=VERTEX_POINT ( 'NONE', #1202 ) ;
#15957=CARTESIAN_POINT ( 'NONE',  ( 0.000000000000000000, 80.00000000000001421, 0.000000000000000000 ) ) ;
#15958=CARTESIAN_POINT ( 'NONE',  ( 33.58253175000000113, 36.37500000273119838, -4.112674001490185761E-15 ) ) ;
#15959=CARTESIAN_POINT ( 'NONE',  ( 26.29305231718579350, 39.30000000546237970, 19.10302069950537529 ) ) ;
#15961=CARTESIAN_POINT ( 'NONE',  ( 0.000000000000000000, 80.00000000000001421, -32.50000000000000000 ) ) ;
#15962=CARTESIAN_POINT ( 'NONE',  ( 7.570916362186207671, 5.349999994537613546, 23.30088464923126779 ) ) ;
#15963=CARTESIAN_POINT ( 'NONE',  ( 33.58253175000000823, 40.27500000273118985, 10.91162601494192863 ) ) ;
#15966=CARTESIAN_POINT ( 'NONE',  ( -32.50000000000000000, 19.99999999999998934, 0.000000000000000000 ) ) ;
#15968=CARTESIAN_POINT ( 'NONE',  ( 33.58253175000000823, 72.02500000273118985, 10.91162601494192863 ) ) ;
#15970=CARTESIAN_POINT ( 'NONE',  ( -20.08610463437157989, 37.70000000000000284, -27.64615127144129758 ) ) ;
#15971=CARTESIAN_POINT ( 'NONE',  ( 10.37757302488624767, 51.97500000273119980, 31.93888565452638417 ) ) ;
#15972=CARTESIAN_POINT ( 'NONE',  ( 5.147494310547426899, 7.948745723915522809, -32.50000000000000000 ) ) ;
#15973=CARTESIAN_POINT ( 'NONE',  ( -33.58253175000000113, 11.22500000273120335, 10.91162601494193929 ) ) ;
#15980=AXIS2_PLACEMENT_3D ( 'NONE', #26250, #17209, #6898 ) ;
#15981=DIRECTION ( 'NONE',  ( 0.000000000000000000, 0.000000000000000000, 1.000000000000000000 ) ) ;
#15989=CARTESIAN_POINT ( 'NONE',  ( -32.50000000000000000, 72.50000000546236834, 0.000000000000000000 ) ) ;
#15993=VERTEX_POINT ( 'NONE', #11515 ) ;
#15997=CARTESIAN_POINT ( 'NONE',  ( 26.29305231718579350, 74.80000000000001137, 19.10302069950537529 ) ) ;
#15998=CARTESIAN_POINT ( 'NONE',  ( 27.16883889988623935, 54.57500000273118701, -19.73931689729374384 ) ) ;
#15999=CARTESIAN_POINT ( 'NONE',  ( 32.50000000000000000, 53.60000000546238397, -10.55989012756945833 ) ) ;
#16001=CARTESIAN_POINT ( 'NONE',  ( 33.58253175000000823, 36.02500000273117564, 10.91162601494192863 ) ) ;
#16004=CARTESIAN_POINT ( 'NONE',  ( -20.75514604977248823, 67.07500000273118701, -28.56700777964554305 ) ) ;
#16008=CARTESIAN_POINT ( 'NONE',  ( 10.04305231718578817, 39.39999999999999147, -30.90933677959249337 ) ) ;
#16011=CARTESIAN_POINT ( 'NONE',  ( -33.58253175000000113, 11.47500000273119625, 10.91162601494193929 ) ) ;
#16012=CARTESIAN_POINT ( 'NONE',  ( 24.50000000000000000, 19.64999999453763024, 7.960532557706212486 ) ) ;
#16014=CARTESIAN_POINT ( 'NONE',  ( -11.25946833292375793, 71.57500000273120122, 8.180482586598737171 ) ) ;
#16015=CARTESIAN_POINT ( 'NONE',  ( 33.58253175000000823, 70.27500000273118985, 10.91162601494192685 ) ) ;
#16016=LINE ( 'NONE', #26470, #33564 ) ;
#16018=VERTEX_POINT ( 'NONE', #29374 ) ;
#16029=CARTESIAN_POINT ( 'NONE',  ( 6.486482029760648627E-15, 39.62500000273117706, 35.31076352940722529 ) ) ;
#16032=DIRECTION ( 'NONE',  ( 0.000000000000000000, 0.000000000000000000, -1.000000000000000000 ) ) ;
#16037=CARTESIAN_POINT ( 'NONE',  ( 10.37757302488624056, 68.77500000273117564, -31.93888565452638417 ) ) ;
#16041=ORIENTED_EDGE ( 'NONE', *, *, #12835, .F. ) ;
#16043=CARTESIAN_POINT ( 'NONE',  ( 20.08610463437157279, 65.80000000546237970, -27.64615127144129758 ) ) ;
#16044=CARTESIAN_POINT ( 'NONE',  ( -33.58253175000000113, 61.22500000273118559, 10.91162601494193929 ) ) ;
#16046=CARTESIAN_POINT ( 'NONE',  ( 20.08610463437158344, 17.20000000546236762, 27.64615127144129403 ) ) ;
#16047=CARTESIAN_POINT ( 'NONE',  ( -32.50000000000000000, 66.50000000546238255, 0.000000000000000000 ) ) ;
#16048=CARTESIAN_POINT ( 'NONE',  ( -7.236395654485757944, 7.724999997268805707, -22.27133577429736988 ) ) ;
#16049=EDGE_CURVE ( 'NONE', #20206, #28550, #16680, .T. ) ;
#16050=CARTESIAN_POINT ( 'NONE',  ( 6.486482029760649416E-15, 5.625000002731175286, 35.31076352940723240 ) ) ;
#16051=CARTESIAN_POINT ( 'NONE',  ( 20.75514604977248467, 30.67500000273119909, -28.56700777964554305 ) ) ;
#16054=FACE_OUTER_BOUND ( 'NONE', #19267, .T. ) ;
#16055=CARTESIAN_POINT ( 'NONE',  ( -10.04305231718578462, 32.39999999999998437, 30.90933677959249337 ) ) ;
#16059=CARTESIAN_POINT ( 'NONE',  ( 13.91746824999999532, 73.97500000273119269, -4.522059556121118540 ) ) ;
#16061=CARTESIAN_POINT ( 'NONE',  ( -10.37757302488623701, 25.52500000273119696, 31.93888565452638417 ) ) ;
#16064=CARTESIAN_POINT ( 'NONE',  ( 33.58253175000000113, 12.37500000273117351, -4.112674001490185761E-15 ) ) ;
#16066=CARTESIAN_POINT ( 'NONE',  ( 33.58253175000000113, 70.12500000273119838, -4.112674001490185761E-15 ) ) ;
#16067=CARTESIAN_POINT ( 'NONE',  ( -1.778240108872766143E-15, 4.000000005462373664, -32.49999999999999289 ) ) ;
#16070=CARTESIAN_POINT ( 'NONE',  ( 9.270509831248425314, 78.95000000546239960, 12.75976212528059683 ) ) ;
#16071=CARTESIAN_POINT ( 'NONE',  ( -2.162160676586882350E-15, 60.62500000273118417, -35.31076352940722529 ) ) ;
#16074=ORIENTED_EDGE ( 'NONE', *, *, #11926, .F. ) ;
#16077=CARTESIAN_POINT ( 'NONE',  ( -7.236395654485763274, 2.024999997268822405, 22.27133577429736633 ) ) ;
#16082=CARTESIAN_POINT ( 'NONE',  ( -10.04305231718578462, 42.90000000546237402, 30.90933677959249337 ) ) ;
#16083=VERTEX_POINT ( 'NONE', #17015 ) ;
#16091=CARTESIAN_POINT ( 'NONE',  ( 18.94512977948576093, 16.82499999726880091, -13.76444248337722875 ) ) ;
#16092=CARTESIAN_POINT ( 'NONE',  ( 10.37757302488624056, 8.775000002731180970, -31.93888565452638417 ) ) ;
#16093=CARTESIAN_POINT ( 'NONE',  ( 32.50000000000000000, 59.00000000000000000, -3.980102097228898626E-15 ) ) ;
#16094=CARTESIAN_POINT ( 'NONE',  ( 11.25946833292375793, 79.67500000273119554, 8.180482586598731842 ) ) ;
#16095=FACE_OUTER_BOUND ( 'NONE', #2279, .T. ) ;
#16097=CARTESIAN_POINT ( 'NONE',  ( -8.960552108402742093E-16, 74.87500000273116996, -14.63369212191046387 ) ) ;
#16102=CARTESIAN_POINT ( 'NONE',  ( 26.29305231718579350, 2.799999999999997158, 19.10302069950537529 ) ) ;
#16105=CARTESIAN_POINT ( 'NONE',  ( -27.16883889988624290, 40.92500000273119554, -19.73931689729374028 ) ) ;
#16108=CARTESIAN_POINT ( 'NONE',  ( -33.58253175000000113, 33.37500000273119127, 0.000000000000000000 ) ) ;
#16112=CARTESIAN_POINT ( 'NONE',  ( -2.375766604868045029, 75.55125428154684641, -14.99999999999999822 ) ) ;
#16115=CARTESIAN_POINT ( 'NONE',  ( 7.236395654485760609, 3.024999997268823293, -22.27133577429736633 ) ) ;
#16117=DIRECTION ( 'NONE',  ( -0.8660254037844402619, 0.4999999999999970579, -0.000000000000000000 ) ) ;
#16118=CARTESIAN_POINT ( 'NONE',  ( 10.37757302488624056, 22.52500000273119340, -31.93888565452638417 ) ) ;
#16121=VERTEX_POINT ( 'NONE', #26807 ) ;
#16127=ORIENTED_EDGE ( 'NONE', *, *, #29282, .T. ) ;
#16129=CARTESIAN_POINT ( 'NONE',  ( 20.75514604977249178, 26.07500000273119767, 28.56700777964553950 ) ) ;
#16130=CARTESIAN_POINT ( 'NONE',  ( 32.50000000000000711, 37.40000000546236691, 10.55989012756945122 ) ) ;
#16131=CARTESIAN_POINT ( 'NONE',  ( -26.29305231718579350, 75.80000000000001137, -19.10302069950537884 ) ) ;
#16132=CARTESIAN_POINT ( 'NONE',  ( 26.29305231718578995, 33.70000000546238539, -19.10302069950538240 ) ) ;
#16133=CARTESIAN_POINT ( 'NONE',  ( 32.50000000000000711, 76.89999999999999147, 10.55989012756945122 ) ) ;
#16134=CARTESIAN_POINT ( 'NONE',  ( 10.37757302488624767, 43.97500000273119269, 31.93888565452638417 ) ) ;
#16137=CARTESIAN_POINT ( 'NONE',  ( -26.29305231718579350, 21.79999999999998650, -19.10302069950537884 ) ) ;
#16139=CARTESIAN_POINT ( 'NONE',  ( 6.486482029760649416E-15, 63.62500000273117706, 35.31076352940723240 ) ) ;
#16140=CARTESIAN_POINT ( 'NONE',  ( -32.50000000000000000, 78.00000000000001421, 0.000000000000000000 ) ) ;
#16141=VECTOR ( 'NONE', #8565, 1000.000000000000000 ) ;
#16142=CARTESIAN_POINT ( 'NONE',  ( -32.50000000000000000, 76.50000000546236834, 0.000000000000000000 ) ) ;
#16143=CARTESIAN_POINT ( 'NONE',  ( 33.58253175000000113, 52.47500000273117848, -10.91162601494193574 ) ) ;
#16146=CARTESIAN_POINT ( 'NONE',  ( 10.37757302488624056, 10.52500000273118275, -31.93888565452638417 ) ) ;
#16148=CARTESIAN_POINT ( 'NONE',  ( 7.570916362186213000, 2.149999994537632464, -23.30088464923126423 ) ) ;
#16158=CARTESIAN_POINT ( 'NONE',  ( 20.08610463437158344, 69.20000000546235697, 27.64615127144129403 ) ) ;
#16162=ORIENTED_EDGE ( 'NONE', *, *, #29484, .F. ) ;
#16166=CARTESIAN_POINT ( 'NONE',  ( -26.29305231718578995, 36.20000000000000995, 19.10302069950538595 ) ) ;
#16167=CARTESIAN_POINT ( 'NONE',  ( -10.37757302488624411, 46.97500000273119269, -31.93888565452638417 ) ) ;
#16168=CARTESIAN_POINT ( 'NONE',  ( -10.04305231718579172, 56.10000000546239107, -30.90933677959248982 ) ) ;
#16170=CARTESIAN_POINT ( 'NONE',  ( -33.58253175000000113, 35.22500000273119980, 10.91162601494193929 ) ) ;
#16172=CARTESIAN_POINT ( 'NONE',  ( 33.58253175000000113, 62.47500000273118559, -10.91162601494193751 ) ) ;
#16176=CARTESIAN_POINT ( 'NONE',  ( -32.50000000000000000, 42.00000000000000711, 0.000000000000000000 ) ) ;
#16179=CARTESIAN_POINT ( 'NONE',  ( 20.75514604977249178, 6.075000002731190563, 28.56700777964553950 ) ) ;
#16182=CARTESIAN_POINT ( 'NONE',  ( 33.58253175000000823, 74.27500000273118985, 10.91162601494192685 ) ) ;
#16183=CARTESIAN_POINT ( 'NONE',  ( 0.000000000000000000, 80.00000000000001421, 0.000000000000000000 ) ) ;
#16186=ORIENTED_EDGE ( 'NONE', *, *, #24194, .F. ) ;
#16188=AXIS2_PLACEMENT_3D ( 'NONE', #24331, #3727, #806 ) ;
#16198=CARTESIAN_POINT ( 'NONE',  ( 10.37757302488624056, 38.52500000273118275, -31.93888565452638417 ) ) ;
#16204=CARTESIAN_POINT ( 'NONE',  ( -5.147494310547430452, 50.05125428700922185, -32.49999999999999289 ) ) ;
#16206=CARTESIAN_POINT ( 'NONE',  ( 20.75514604977249178, 70.07500000273120122, 28.56700777964553950 ) ) ;
#16207=ORIENTED_EDGE ( 'NONE', *, *, #26245, .F. ) ;
#16210=( GEOMETRIC_REPRESENTATION_CONTEXT ( 3 ) GLOBAL_UNCERTAINTY_ASSIGNED_CONTEXT ( ( #14064 ) ) GLOBAL_UNIT_ASSIGNED_CONTEXT ( ( #361, #21982, #29858 ) ) REPRESENTATION_CONTEXT ( 'NONE', 'WORKASPACE' ) );
#16212=( BOUNDED_CURVE ( )  B_SPLINE_CURVE ( 2, ( #21775, #26906, #29975, #14208, #19363, #32548, #32383, #16785, #14542, #27578, #29472, #4067, #815 ),
 .UNSPECIFIED., .F., .T. ) 
 B_SPLINE_CURVE_WITH_KNOTS ( ( 3, 2, 2, 2, 2, 2, 3 ),
 ( 0.8910256410256410797, 0.8923076923076923572, 0.8948717948717949122, 0.8974358974358974672, 0.9000000000000000222, 0.9025641025641025772, 0.9038461538461538547 ),
 .UNSPECIFIED. ) 
 CURVE ( )  GEOMETRIC_REPRESENTATION_ITEM ( )  RATIONAL_B_SPLINE_CURVE ( ( 0.9755282581475768211, 0.9755282581475778203, 1.000000000000000000, 0.9510565162951535312, 1.000000000000000000, 0.9510565162951535312, 1.000000000000000000, 0.9510565162951535312, 1.000000000000000000, 0.9510565162951535312, 1.000000000000000000, 0.9755282581475768211, 0.9755282581475768211 ) ) 
 REPRESENTATION_ITEM ( '' )  );
#16214=CARTESIAN_POINT ( 'NONE',  ( 6.486482029760649416E-15, 55.62500000273119838, 35.31076352940723240 ) ) ;
#16216=CARTESIAN_POINT ( 'NONE',  ( 20.08610463437157279, 15.80000000546238326, -27.64615127144129758 ) ) ;
#16217=DIRECTION ( 'NONE',  ( -0.000000000000000000, -1.000000000000000000, -0.000000000000000000 ) ) ;
#16218=CARTESIAN_POINT ( 'NONE',  ( 7.236395654485755280, 10.72499999726880837, 22.27133577429736988 ) ) ;
#16219=CARTESIAN_POINT ( 'NONE',  ( 20.75514604977249178, 32.07500000273117990, 28.56700777964553950 ) ) ;
#16222=CARTESIAN_POINT ( 'NONE',  ( -4.405589869732278832E-13, 32.49999999999997868, 32.50000000000000000 ) ) ;
#16224=CARTESIAN_POINT ( 'NONE',  ( 2.489536152421872915E-14, 76.00000000546238255, -32.49999999999999289 ) ) ;
#16228=CARTESIAN_POINT ( 'NONE',  ( 4.300734207923757602, 76.27500000273118985, -13.23629886949340673 ) ) ;
#16230=CARTESIAN_POINT ( 'NONE',  ( -27.16883889988623935, 25.32500000273119056, 19.73931689729374739 ) ) ;
#16233=CARTESIAN_POINT ( 'NONE',  ( -20.75514604977248823, 17.07500000273119412, -28.56700777964554305 ) ) ;
#16235=CARTESIAN_POINT ( 'NONE',  ( 33.58253175000000823, 68.02500000273117564, 10.91162601494192685 ) ) ;
#16236=FACE_OUTER_BOUND ( 'NONE', #224, .T. ) ;
#16238=CARTESIAN_POINT ( 'NONE',  ( 20.75514604977248467, 56.42500000273120264, -28.56700777964554305 ) ) ;
#16240=ORIENTED_EDGE ( 'NONE', *, *, #7756, .T. ) ;
#16242=CARTESIAN_POINT ( 'NONE',  ( 33.58253175000000823, 2.025000002731202287, 10.91162601494192685 ) ) ;
#16244=CARTESIAN_POINT ( 'NONE',  ( -23.41746825000000598, 3.724999997268819918, 7.608796670333726198 ) ) ;
#16246=ORIENTED_EDGE ( 'NONE', *, *, #27184, .F. ) ;
#16251=CARTESIAN_POINT ( 'NONE',  ( -4.223320258572819786E-15, 17.50000000000000000, 24.50000000000000000 ) ) ;
#16252=CARTESIAN_POINT ( 'NONE',  ( -19.82091636218621389, 3.200000000000008171, 14.40073868116558842 ) ) ;
#16253=CARTESIAN_POINT ( 'NONE',  ( -27.16883889988623935, 75.32500000273117280, 19.73931689729374739 ) ) ;
#16255=CARTESIAN_POINT ( 'NONE',  ( -24.50000000000000000, 1.000000000000000888, -3.000384657911015469E-15 ) ) ;
#16256=CARTESIAN_POINT ( 'NONE',  ( 27.16883889988624290, 8.175000002731191984, 19.73931689729373673 ) ) ;
#16257=CARTESIAN_POINT ( 'NONE',  ( 33.58253175000000823, 26.02500000273120406, 10.91162601494192863 ) ) ;
#16258=CARTESIAN_POINT ( 'NONE',  ( 13.91746824999999887, 79.87500000273118417, -1.704398294459741270E-15 ) ) ;
#16259=CARTESIAN_POINT ( 'NONE',  ( 7.890940483122900408E-14, 18.24999999453761745, -24.50000000000000000 ) ) ;
#16261=CARTESIAN_POINT ( 'NONE',  ( 8.601468415847520532, 74.07500000273120122, 11.83890561707634781 ) ) ;
#16265=CARTESIAN_POINT ( 'NONE',  ( 5.147494310547408247, 70.55125428154684641, 32.50000000000000711 ) ) ;
#16267=CARTESIAN_POINT ( 'NONE',  ( 20.75514604977248467, 42.42500000273117422, -28.56700777964554305 ) ) ;
#16270=CARTESIAN_POINT ( 'NONE',  ( -20.75514604977248823, 33.07500000273118701, -28.56700777964554305 ) ) ;
#16275=CARTESIAN_POINT ( 'NONE',  ( 20.08610463437157279, 31.30000000000000071, -27.64615127144129758 ) ) ;
#16278=CARTESIAN_POINT ( 'NONE',  ( 14.47279130897151944, 4.924999997268811214, -19.92008829642072598 ) ) ;
#16279=CARTESIAN_POINT ( 'NONE',  ( -32.50000000000000000, 52.60000000546235555, 10.55989012756946366 ) ) ;
#16282=CARTESIAN_POINT ( 'NONE',  ( 20.75514604977249178, 17.82500000273119767, 28.56700777964553950 ) ) ;
#16286=VERTEX_POINT ( 'NONE', #13935 ) ;
#16290=ORIENTED_EDGE ( 'NONE', *, *, #8518, .T. ) ;
#16292=CARTESIAN_POINT ( 'NONE',  ( -33.58253175000000113, 29.47500000273117848, 10.91162601494193929 ) ) ;
#16293=CARTESIAN_POINT ( 'NONE',  ( -26.29305231718578995, 32.70000000546238539, 19.10302069950538595 ) ) ;
#16294=CARTESIAN_POINT ( 'NONE',  ( 10.04305231718578817, 77.39999999999999147, -30.90933677959249337 ) ) ;
#16295=CARTESIAN_POINT ( 'NONE',  ( 5.779280353836490358E-15, 25.00000000546237899, 32.49999999999999289 ) ) ;
#16296=CARTESIAN_POINT ( 'NONE',  ( 15.00000000000000000, 73.00000000000001421, -1.836970198721029589E-15 ) ) ;
#16297=CARTESIAN_POINT ( 'NONE',  ( 10.37757302488624056, 42.77500000273118275, -31.93888565452638417 ) ) ;
#16301=CARTESIAN_POINT ( 'NONE',  ( 26.29305231718578995, 23.19999999999999929, -19.10302069950538240 ) ) ;
#16304=CARTESIAN_POINT ( 'NONE',  ( 33.58253175000000113, 60.12500000273119127, -4.112674001490185761E-15 ) ) ;
#16307=CARTESIAN_POINT ( 'NONE',  ( -20.75514604977248112, 51.67500000273117422, 28.56700777964554661 ) ) ;
#16310=CARTESIAN_POINT ( 'NONE',  ( 10.37757302488624767, 5.725000002731183812, 31.93888565452638417 ) ) ;
#16312=CARTESIAN_POINT ( 'NONE',  ( 4.445600272181915325E-13, 26.00000000546237189, -32.50000000000000000 ) ) ;
#16313=DIRECTION ( 'NONE',  ( -0.000000000000000000, -1.000000000000000000, -0.000000000000000000 ) ) ;
#16317=CARTESIAN_POINT ( 'NONE',  ( 5.779280353836490358E-15, 1.000000005462375885, 32.49999999999999289 ) ) ;
#16323=AXIS2_PLACEMENT_3D ( 'NONE', #18864, #31883, #18704 ) ;
#16324=CARTESIAN_POINT ( 'NONE',  ( -26.29305231718579350, 68.30000000546237970, -19.10302069950537884 ) ) ;
#16331=CARTESIAN_POINT ( 'NONE',  ( 10.04305231718579705, 74.59999999999999432, 30.90933677959248982 ) ) ;
#16332=CARTESIAN_POINT ( 'NONE',  ( -20.75514604977248823, 47.07500000273117990, -28.56700777964554305 ) ) ;
#16333=CARTESIAN_POINT ( 'NONE',  ( 32.50000000000000711, 49.40000000546236691, 10.55989012756945122 ) ) ;
#16335=CARTESIAN_POINT ( 'NONE',  ( -33.58253175000000113, 33.12500000273119127, 0.000000000000000000 ) ) ;
#16337=CARTESIAN_POINT ( 'NONE',  ( 27.16883889988623935, 60.57500000273119412, -19.73931689729374384 ) ) ;
#16340=CARTESIAN_POINT ( 'NONE',  ( -32.50000000000000000, 38.00000000000000711, 0.000000000000000000 ) ) ;
#16342=CARTESIAN_POINT ( 'NONE',  ( -2.162160676586881955E-15, 6.875000002731195714, -35.31076352940723240 ) ) ;
#16343=CARTESIAN_POINT ( 'NONE',  ( 26.29305231718579350, 35.30000000546237970, 19.10302069950537529 ) ) ;
#16344=CARTESIAN_POINT ( 'NONE',  ( -13.91746824999999887, 73.37500000273119838, 0.000000000000000000 ) ) ;
#16345=CARTESIAN_POINT ( 'NONE',  ( 27.16883889988623935, 72.57500000273120122, -19.73931689729374384 ) ) ;
#16346=CARTESIAN_POINT ( 'NONE',  ( -3.880418787951142701, 19.19874571299078525, 24.49999999999999645 ) ) ;
#16349=FACE_OUTER_BOUND ( 'NONE', #6680, .T. ) ;
#16360=CARTESIAN_POINT ( 'NONE',  ( 2.205017735002230837E-13, 56.00000000546238255, -32.50000000000000000 ) ) ;
#16361=CARTESIAN_POINT ( 'NONE',  ( 20.75514604977249178, 41.82500000273120122, 28.56700777964553950 ) ) ;
#16364=CARTESIAN_POINT ( 'NONE',  ( 26.29305231718578995, 13.70000000546239782, -19.10302069950538240 ) ) ;
#16366=EDGE_CURVE ( 'NONE', #17243, #32915, #26524, .T. ) ;
#16368=CARTESIAN_POINT ( 'NONE',  ( 10.04305231718579705, 50.60000000000000853, 30.90933677959248982 ) ) ;
#16370=CARTESIAN_POINT ( 'NONE',  ( -10.37757302488623701, 67.77500000273117564, 31.93888565452638417 ) ) ;
#16371=EDGE_CURVE ( 'NONE', #31469, #16121, #18216, .T. ) ;
#16372=ORIENTED_EDGE ( 'NONE', *, *, #2433, .F. ) ;
#16376=CARTESIAN_POINT ( 'NONE',  ( 10.04305231718579705, 65.10000000546240528, 30.90933677959248982 ) ) ;
#16377=CARTESIAN_POINT ( 'NONE',  ( -33.58253175000000113, 55.22500000273117848, 10.91162601494193929 ) ) ;
#16379=CARTESIAN_POINT ( 'NONE',  ( 32.50000000000000711, 15.40000000546236514, 10.55989012756945122 ) ) ;
#16380=CARTESIAN_POINT ( 'NONE',  ( 15.14183272437242422, 16.04999999453762882, -20.84094480462497856 ) ) ;
#16381=CARTESIAN_POINT ( 'NONE',  ( 14.47279130897151767, 10.82499999726879913, 19.92008829642072953 ) ) ;
#16382=CARTESIAN_POINT ( 'NONE',  ( 27.16883889988623935, 24.57500000273119056, -19.73931689729374384 ) ) ;
#16385=CARTESIAN_POINT ( 'NONE',  ( -8.601468415847518756, 78.57500000273120122, -11.83890561707634781 ) ) ;
#16386=CARTESIAN_POINT ( 'NONE',  ( 26.29305231718578995, 15.19999999999999218, -19.10302069950538240 ) ) ;
#16388=ORIENTED_EDGE ( 'NONE', *, *, #32529, .F. ) ;
#16390=CARTESIAN_POINT ( 'NONE',  ( -8.960552108402742093E-16, 72.37500000273116996, -14.63369212191046387 ) ) ;
#16392=CARTESIAN_POINT ( 'NONE',  ( -2.162160676586881955E-15, 24.62500000273118772, -35.31076352940723240 ) ) ;
#16396=CARTESIAN_POINT ( 'NONE',  ( -27.16883889988623935, 15.57500000273118168, 19.73931689729374739 ) ) ;
#16398=CARTESIAN_POINT ( 'NONE',  ( 10.37757302488624767, 69.72500000273117848, 31.93888565452638417 ) ) ;
#16399=CYLINDRICAL_SURFACE ( 'NONE', #30994, 32.50000000000000000 ) ;
#16400=CARTESIAN_POINT ( 'NONE',  ( -11.25946833292375793, 75.57500000273120122, 8.180482586598737171 ) ) ;
#16402=CARTESIAN_POINT ( 'NONE',  ( -1.778240108872766143E-15, 63.50000000000000000, -32.49999999999999289 ) ) ;
#16403=CARTESIAN_POINT ( 'NONE',  ( 27.16883889988624290, 55.92500000273120975, 19.73931689729373673 ) ) ;
#16405=EDGE_CURVE ( 'NONE', #7955, #7360, #20443, .T. ) ;
#16409=CARTESIAN_POINT ( 'NONE',  ( 33.58253175000000113, 2.125000002731192161, -4.112674001490185761E-15 ) ) ;
#16410=CARTESIAN_POINT ( 'NONE',  ( -7.236395654485757944, 7.224999997268804819, -22.27133577429736988 ) ) ;
#16413=VERTEX_POINT ( 'NONE', #27817 ) ;
#16416=ORIENTED_EDGE ( 'NONE', *, *, #655, .F. ) ;
#16420=CARTESIAN_POINT ( 'NONE',  ( 27.16883889988624290, 75.92500000273119554, 19.73931689729373673 ) ) ;
#16422=CARTESIAN_POINT ( 'NONE',  ( 15.14183272437242245, 8.300000000000000711, -20.84094480462497856 ) ) ;
#16423=CARTESIAN_POINT ( 'NONE',  ( -33.58253175000000113, 7.275000002731181858, -10.91162601494193218 ) ) ;
#16424=CARTESIAN_POINT ( 'NONE',  ( -33.58253175000000113, 19.02500000273118630, -10.91162601494193218 ) ) ;
#16425=CARTESIAN_POINT ( 'NONE',  ( 13.91746825000000065, 79.77500000273118985, 4.522059556121115875 ) ) ;
#16426=CARTESIAN_POINT ( 'NONE',  ( 5.779280353836490358E-15, 65.00000000546236834, 32.49999999999999289 ) ) ;
#16428=CARTESIAN_POINT ( 'NONE',  ( -15.00000000000000000, 78.10000000000000853, 4.873795443493597723 ) ) ;
#16430=CARTESIAN_POINT ( 'NONE',  ( -3.880418787951136483, 8.301254276084460315, -24.50000000000000000 ) ) ;
#16431=CARTESIAN_POINT ( 'NONE',  ( 26.29305231718579350, 49.30000000546236549, 19.10302069950537529 ) ) ;
#16433=CARTESIAN_POINT ( 'NONE',  ( 33.58253175000000113, 42.12500000273116996, -4.112674001490185761E-15 ) ) ;
#16436=CARTESIAN_POINT ( 'NONE',  ( -2.162160676586882350E-15, 34.87500000273117706, -35.31076352940722529 ) ) ;
#16442=CARTESIAN_POINT ( 'NONE',  ( 23.41746824999999887, 4.624999997268814056, 0.000000000000000000 ) ) ;
#16445=CARTESIAN_POINT ( 'NONE',  ( -26.29305231718579350, 59.79999999999999005, -19.10302069950537884 ) ) ;
#16446=CARTESIAN_POINT ( 'NONE',  ( 27.16883889988624290, 17.92500000273117422, 19.73931689729373673 ) ) ;
#16447=CARTESIAN_POINT ( 'NONE',  ( -14.47279130897152122, 8.424999997268816543, 19.92008829642072243 ) ) ;
#16449=ORIENTED_EDGE ( 'NONE', *, *, #26976, .F. ) ;
#16455=CARTESIAN_POINT ( 'NONE',  ( 14.47279130897151589, 4.324999997268801799, 19.92008829642072953 ) ) ;
#16456=CARTESIAN_POINT ( 'NONE',  ( -27.16883889988623935, 31.57500000273119767, 19.73931689729374739 ) ) ;
#16457=CARTESIAN_POINT ( 'NONE',  ( 20.08610463437158344, 33.20000000546238539, 27.64615127144129403 ) ) ;
#16458=CARTESIAN_POINT ( 'NONE',  ( 32.50000000000000711, 78.89999999999999147, 10.55989012756945122 ) ) ;
#16459=CARTESIAN_POINT ( 'NONE',  ( 0.000000000000000000, 82.00000000000001421, 0.000000000000000000 ) ) ;
#16461=CARTESIAN_POINT ( 'NONE',  ( -33.58253175000000113, 41.47500000273117138, 10.91162601494193929 ) ) ;
#16463=CARTESIAN_POINT ( 'NONE',  ( 10.04305231718579705, 18.60000000000000497, 30.90933677959248982 ) ) ;
#16465=CARTESIAN_POINT ( 'NONE',  ( 27.16883889988623935, 62.32500000273119412, -19.73931689729374384 ) ) ;
#16466=CARTESIAN_POINT ( 'NONE',  ( 27.16883889988624290, 52.17500000273117422, 19.73931689729373673 ) ) ;
#16469=CARTESIAN_POINT ( 'NONE',  ( 10.37757302488624056, 4.525000002731205839, -31.93888565452638417 ) ) ;
#16475=CARTESIAN_POINT ( 'NONE',  ( -10.04305231718579172, 30.10000000546236976, -30.90933677959248982 ) ) ;
#16478=CARTESIAN_POINT ( 'NONE',  ( 20.08610463437158344, 48.70000000000000284, 27.64615127144129403 ) ) ;
#16485=ORIENTED_EDGE ( 'NONE', *, *, #31598, .F. ) ;
#16488=EDGE_CURVE ( 'NONE', #26696, #9328, #20408, .T. ) ;
#16490=CARTESIAN_POINT ( 'NONE',  ( -5.147494310547423346, 36.44874571845313227, 32.50000000000000000 ) ) ;
#16491=CARTESIAN_POINT ( 'NONE',  ( 33.58253175000000113, 50.47500000273117848, -10.91162601494193751 ) ) ;
#16492=CARTESIAN_POINT ( 'NONE',  ( -26.29305231718578995, 50.70000000546237828, 19.10302069950538595 ) ) ;
#16493=( BOUNDED_CURVE ( )  B_SPLINE_CURVE ( 2, ( #9662, #30587, #1242, #17567, #14475, #3834, #11720, #1417, #14648, #30072, #14815, #28024, #25280 ),
 .UNSPECIFIED., .F., .F. ) 
 B_SPLINE_CURVE_WITH_KNOTS ( ( 3, 2, 2, 2, 2, 2, 3 ),
 ( 0.08333333333333334259, 0.08461538461538462008, 0.08717948717948717507, 0.08974358974358974395, 0.09230769230769231282, 0.09487179487179486781, 0.09615384615384615918 ),
 .UNSPECIFIED. ) 
 CURVE ( )  GEOMETRIC_REPRESENTATION_ITEM ( )  RATIONAL_B_SPLINE_CURVE ( ( 0.9755282581475767101, 0.9755282581475768211, 1.000000000000000000, 0.9510565162951535312, 1.000000000000000000, 0.9510565162951535312, 1.000000000000000000, 0.9510565162951535312, 1.000000000000000000, 0.9510565162951535312, 1.000000000000000000, 0.9755282581475765991, 0.9755282581475767101 ) ) 
 REPRESENTATION_ITEM ( '' )  );
#16495=CARTESIAN_POINT ( 'NONE',  ( -33.58253175000000113, 33.02500000273118275, -10.91162601494193218 ) ) ;
#16497=CARTESIAN_POINT ( 'NONE',  ( -2.162160676586881955E-15, 60.87500000273116996, -35.31076352940723240 ) ) ;
#16498=SURFACE_STYLE_FILL_AREA ( #17003 ) ;
#16499=EDGE_CURVE ( 'NONE', #13970, #29891, #19926, .T. ) ;
#16500=CARTESIAN_POINT ( 'NONE',  ( 20.08610463437158344, 40.69999999999999574, 27.64615127144129403 ) ) ;
#16502=CARTESIAN_POINT ( 'NONE',  ( 20.75514604977248467, 2.675000002731181770, -28.56700777964554305 ) ) ;
#16503=CARTESIAN_POINT ( 'NONE',  ( 10.04305231718578817, 13.39999999999999503, -30.90933677959249337 ) ) ;
#16504=CARTESIAN_POINT ( 'NONE',  ( 4.300734207923757602, 72.77500000273118985, -13.23629886949340673 ) ) ;
#16505=CARTESIAN_POINT ( 'NONE',  ( 27.16883889988623935, 70.57500000273120122, -19.73931689729374384 ) ) ;
#16506=CARTESIAN_POINT ( 'NONE',  ( -24.50000000000000711, 5.100000000000012967, 7.960532557706201828 ) ) ;
#16509=ORIENTED_EDGE ( 'NONE', *, *, #18928, .F. ) ;
#16510=CARTESIAN_POINT ( 'NONE',  ( -15.14183272437242600, 7.049999994537622605, 20.84094480462497856 ) ) ;
#16524=CARTESIAN_POINT ( 'NONE',  ( 20.08610463437157279, 59.30000000000001847, -27.64615127144129758 ) ) ;
#16527=DIRECTION ( 'NONE',  ( 0.000000000000000000, -1.000000000000000000, 0.000000000000000000 ) ) ;
#16531=CARTESIAN_POINT ( 'NONE',  ( 33.58253175000000113, 72.37500000273116996, -4.112674001490185761E-15 ) ) ;
#16532=EDGE_LOOP ( 'NONE', ( #2207, #22987, #22164, #25604 ) ) ;
#16535=EDGE_LOOP ( 'NONE', ( #6634, #3360, #3523, #20640, #33266, #30090 ) ) ;
#16538=CARTESIAN_POINT ( 'NONE',  ( 10.37757302488624767, 53.72500000273117138, 31.93888565452638417 ) ) ;
#16540=CARTESIAN_POINT ( 'NONE',  ( -26.29305231718579350, 12.30000000546238681, -19.10302069950537884 ) ) ;
#16541=CARTESIAN_POINT ( 'NONE',  ( 24.50000000000000000, 15.84999999453763664, -7.960532557706203605 ) ) ;
#16542=CARTESIAN_POINT ( 'NONE',  ( 7.236395654485760609, 7.524999997268800200, -22.27133577429736633 ) ) ;
#16543=CARTESIAN_POINT ( 'NONE',  ( 10.37757302488624767, 23.97500000273117138, 31.93888565452638417 ) ) ;
#16546=CARTESIAN_POINT ( 'NONE',  ( -10.04305231718579172, 31.59999999999999076, -30.90933677959248982 ) ) ;
#16547=CARTESIAN_POINT ( 'NONE',  ( 20.08610463437158344, 14.70000000000000107, 27.64615127144129403 ) ) ;
#16551=CARTESIAN_POINT ( 'NONE',  ( 11.25946833292375793, 73.67500000273119554, 8.180482586598731842 ) ) ;
#16554=CARTESIAN_POINT ( 'NONE',  ( 6.486482029760649416E-15, 27.62500000273118062, 35.31076352940723240 ) ) ;
#16558=CARTESIAN_POINT ( 'NONE',  ( -33.58253175000000113, 7.275000002731180970, -10.91162601494193041 ) ) ;
#16560=CARTESIAN_POINT ( 'NONE',  ( -10.37757302488624411, 72.72500000273119269, -31.93888565452638417 ) ) ;
#16562=CARTESIAN_POINT ( 'NONE',  ( 3.980102097228898626E-15, 80.00000000000001421, 32.50000000000000000 ) ) ;
#16563=CARTESIAN_POINT ( 'NONE',  ( -13.91746824999999887, 77.37500000273116996, 0.000000000000000000 ) ) ;
#16566=CARTESIAN_POINT ( 'NONE',  ( 10.37757302488624767, 57.72500000273117848, 31.93888565452638417 ) ) ;
#16568=ORIENTED_EDGE ( 'NONE', *, *, #22998, .F. ) ;
#16570=CARTESIAN_POINT ( 'NONE',  ( -27.16883889988623935, 3.325000002731171023, 19.73931689729374739 ) ) ;
#16571=CARTESIAN_POINT ( 'NONE',  ( -18.94512977948576093, 5.824999997268820451, 13.76444248337722698 ) ) ;
#16573=ORIENTED_EDGE ( 'NONE', *, *, #31799, .F. ) ;
#16575=CARTESIAN_POINT ( 'NONE',  ( -5.147494310547430452, 68.05125428700922896, -32.49999999999999289 ) ) ;
#16576=ORIENTED_EDGE ( 'NONE', *, *, #22664, .T. ) ;
#16578=CARTESIAN_POINT ( 'NONE',  ( 20.75514604977249178, 60.07500000273119412, 28.56700777964553950 ) ) ;
#16580=CARTESIAN_POINT ( 'NONE',  ( -10.37757302488623701, 71.52500000273120406, 31.93888565452638417 ) ) ;
#16582=CARTESIAN_POINT ( 'NONE',  ( -19.82091636218621389, 9.199999999999985079, 14.40073868116558842 ) ) ;
#16583=CARTESIAN_POINT ( 'NONE',  ( 33.58253175000000113, 12.37500000273117351, -4.112674001490185761E-15 ) ) ;
#16584=CARTESIAN_POINT ( 'NONE',  ( 10.37757302488624056, 16.52500000273118985, -31.93888565452638417 ) ) ;
#16585=CARTESIAN_POINT ( 'NONE',  ( 5.779280353836490358E-15, 57.00000000546238965, 32.49999999999999289 ) ) ;
#16588=CARTESIAN_POINT ( 'NONE',  ( 8.601468415847520532, 72.07500000273120122, 11.83890561707634781 ) ) ;
#16591=CARTESIAN_POINT ( 'NONE',  ( -32.50000000000000000, 38.50000000546238965, 0.000000000000000000 ) ) ;
#16593=ADVANCED_FACE ( 'NONE', ( #31236 ), #18551, .F. ) ;
#16594=CARTESIAN_POINT ( 'NONE',  ( 33.58253175000000113, 46.22500000273119269, -10.91162601494193751 ) ) ;
#16598=CARTESIAN_POINT ( 'NONE',  ( 27.16883889988623935, 28.57500000273119412, -19.73931689729374384 ) ) ;
#16600=EDGE_CURVE ( 'NONE', #10964, #28042, #19303, .T. ) ;
#16601=AXIS2_PLACEMENT_3D ( 'NONE', #12606, #5224, #33536 ) ;
#16603=CARTESIAN_POINT ( 'NONE',  ( -15.00000000000000000, 76.10000000000000853, 4.873795443493597723 ) ) ;
#16604=( BOUNDED_CURVE ( )  B_SPLINE_CURVE ( 2, ( #23802, #3365, #26539, #21062, #24303, #24136, #31512, #3033, #8335, #5771, #5603, #10585, #13506 ),
 .UNSPECIFIED., .F., .T. ) 
 B_SPLINE_CURVE_WITH_KNOTS ( ( 3, 2, 2, 2, 2, 2, 3 ),
 ( 0.9551282051282051766, 0.9564102564102564541, 0.9589743589743590091, 0.9615384615384615641, 0.9641025641025641191, 0.9666666666666666741, 0.9679487179487179516 ),
 .UNSPECIFIED. ) 
 CURVE ( )  GEOMETRIC_REPRESENTATION_ITEM ( )  RATIONAL_B_SPLINE_CURVE ( ( 0.9755282581475768211, 0.9755282581475768211, 1.000000000000000000, 0.9510565162951535312, 1.000000000000000000, 0.9510565162951535312, 1.000000000000000000, 0.9510565162951535312, 1.000000000000000000, 0.9510565162951535312, 1.000000000000000000, 0.9755282581475768211, 0.9755282581475768211 ) ) 
 REPRESENTATION_ITEM ( '' )  );
#16607=CARTESIAN_POINT ( 'NONE',  ( 14.47279130897151767, 6.324999997268824892, 19.92008829642072953 ) ) ;
#16611=CARTESIAN_POINT ( 'NONE',  ( 20.75514604977248467, 18.42500000273117777, -28.56700777964554305 ) ) ;
#16612=CARTESIAN_POINT ( 'NONE',  ( -18.94512977948576093, 6.324999997268820451, 13.76444248337722698 ) ) ;
#16614=ORIENTED_EDGE ( 'NONE', *, *, #28032, .F. ) ;
#16616=ORIENTED_EDGE ( 'NONE', *, *, #757, .T. ) ;
#16621=CARTESIAN_POINT ( 'NONE',  ( 19.82091636218621389, 15.94999999453763984, -14.40073868116559197 ) ) ;
#16622=CARTESIAN_POINT ( 'NONE',  ( -4.523095164977116484E-15, 8.124999997268826490, 24.62258325217400312 ) ) ;
#16623=CARTESIAN_POINT ( 'NONE',  ( -27.16883889988624290, 29.17500000273118133, -19.73931689729374028 ) ) ;
#16624=CARTESIAN_POINT ( 'NONE',  ( 32.50000000000000000, 33.50000000546238255, -3.980102097228898626E-15 ) ) ;
#16625=CARTESIAN_POINT ( 'NONE',  ( 32.50000000000000711, 72.90000000000000568, 10.55989012756945122 ) ) ;
#16627=DIRECTION ( 'NONE',  ( -0.000000000000000000, -1.000000000000000000, -0.000000000000000000 ) ) ;
#16629=CARTESIAN_POINT ( 'NONE',  ( 10.37757302488624056, 40.77500000273118275, -31.93888565452638417 ) ) ;
#16630=CARTESIAN_POINT ( 'NONE',  ( -23.41746825000000243, 8.024999997268801977, -7.608796670333730638 ) ) ;
#16631=CARTESIAN_POINT ( 'NONE',  ( -32.50000000000000000, 18.00000000000001421, 0.000000000000000000 ) ) ;
#16634=CARTESIAN_POINT ( 'NONE',  ( -20.75514604977248823, 64.82500000273120122, -28.56700777964554305 ) ) ;
#16635=CARTESIAN_POINT ( 'NONE',  ( 6.486482029760648627E-15, 51.87500000273119127, 35.31076352940722529 ) ) ;
#16637=CARTESIAN_POINT ( 'NONE',  ( 20.08610463437158344, 39.20000000546237118, 27.64615127144129403 ) ) ;
#16638=CARTESIAN_POINT ( 'NONE',  ( 33.58253175000000823, 4.025000002731196957, 10.91162601494192863 ) ) ;
#16646=CARTESIAN_POINT ( 'NONE',  ( -32.50000000000000000, 58.60000000546236265, 10.55989012756946366 ) ) ;
#16647=VECTOR ( 'NONE', #23361, 1000.000000000000000 ) ;
#16648=CARTESIAN_POINT ( 'NONE',  ( 19.82091636218621034, 13.80000000000000604, 14.40073868116559730 ) ) ;
#16651=CARTESIAN_POINT ( 'NONE',  ( 5.147494310547426899, 49.44874571845315359, -32.50000000000000000 ) ) ;
#16661=CARTESIAN_POINT ( 'NONE',  ( -20.08610463437156923, 46.80000000546235839, 27.64615127144130113 ) ) ;
#16662=CARTESIAN_POINT ( 'NONE',  ( 10.37757302488624767, 47.97500000273119269, 31.93888565452638417 ) ) ;
#16663=CARTESIAN_POINT ( 'NONE',  ( 10.04305231718578817, 47.90000000546238113, -30.90933677959249337 ) ) ;
#16665=CARTESIAN_POINT ( 'NONE',  ( -33.58253175000000113, 37.02500000273117564, -10.91162601494193218 ) ) ;
#16667=CARTESIAN_POINT ( 'NONE',  ( 33.58253175000000113, 60.47500000273118559, -10.91162601494193751 ) ) ;
#16668=AXIS2_PLACEMENT_3D ( 'NONE', #33194, #9697, #14681 ) ;
#16669=CARTESIAN_POINT ( 'NONE',  ( 32.50000000000000711, 40.89999999999998437, 10.55989012756945122 ) ) ;
#16671=CARTESIAN_POINT ( 'NONE',  ( -10.37757302488623701, 1.775000002731175197, 31.93888565452638417 ) ) ;
#16674=CARTESIAN_POINT ( 'NONE',  ( 10.37757302488624056, 72.77500000273118985, -31.93888565452638417 ) ) ;
#16675=CARTESIAN_POINT ( 'NONE',  ( 0.000000000000000000, 80.00000000000001421, 0.000000000000000000 ) ) ;
#16677=ORIENTED_EDGE ( 'NONE', *, *, #15026, .T. ) ;
#16678=CARTESIAN_POINT ( 'NONE',  ( -19.82091636218621034, 4.549999994537618164, -14.40073868116559552 ) ) ;
#16680=LINE ( 'NONE', #22167, #24485 ) ;
#16692=CARTESIAN_POINT ( 'NONE',  ( 32.50000000000000000, 59.00000000000000000, -3.980102097228898626E-15 ) ) ;
#16693=ORIENTED_EDGE ( 'NONE', *, *, #29548, .F. ) ;
#16695=( BOUNDED_CURVE ( )  B_SPLINE_CURVE ( 2, ( #32742, #838, #19057, #26775, #16648, #1339, #24859, #29496, #11320, #19556, #27102, #3264, #6508 ),
 .UNSPECIFIED., .F., .T. ) 
 B_SPLINE_CURVE_WITH_KNOTS ( ( 3, 2, 2, 2, 2, 2, 3 ),
 ( 0.7500000000000000000, 0.7555555555555555358, 0.7666666666666667185, 0.7777777777777777901, 0.7888888888888888618, 0.8000000000000000444, 0.8055555555555555802 ),
 .UNSPECIFIED. ) 
 CURVE ( )  GEOMETRIC_REPRESENTATION_ITEM ( )  RATIONAL_B_SPLINE_CURVE ( ( 0.9755282581475768211, 0.9755282581475768211, 1.000000000000000000, 0.9510565162951535312, 1.000000000000000000, 0.9510565162951535312, 1.000000000000000000, 0.9510565162951535312, 1.000000000000000000, 0.9510565162951535312, 1.000000000000000000, 0.9755282581475768211, 0.9755282581475768211 ) ) 
 REPRESENTATION_ITEM ( '' )  );
#16703=ORIENTED_EDGE ( 'NONE', *, *, #24751, .T. ) ;
#16704=DIRECTION ( 'NONE',  ( 0.8660254037844402619, 0.4999999999999970579, -0.000000000000000000 ) ) ;
#16705=CARTESIAN_POINT ( 'NONE',  ( -33.58253175000000113, 53.22500000273118559, 10.91162601494193929 ) ) ;
#16707=CARTESIAN_POINT ( 'NONE',  ( -2.092463501923844636E-15, 14.00000000546237899, -34.17252228774368916 ) ) ;
#16708=CARTESIAN_POINT ( 'NONE',  ( -1.778240108872766143E-15, 45.49999999999999289, -32.49999999999999289 ) ) ;
#16709=CARTESIAN_POINT ( 'NONE',  ( 14.47279130897151767, 12.82499999726882400, 19.92008829642072953 ) ) ;
#16710=( GEOMETRIC_REPRESENTATION_CONTEXT ( 3 ) GLOBAL_UNCERTAINTY_ASSIGNED_CONTEXT ( ( #3100 ) ) GLOBAL_UNIT_ASSIGNED_CONTEXT ( ( #27441, #19393, #13736 ) ) REPRESENTATION_CONTEXT ( 'NONE', 'WORKASPACE' ) );
#16711=CARTESIAN_POINT ( 'NONE',  ( -32.50000000000000000, 57.99999999999999289, 0.000000000000000000 ) ) ;
#16712=CARTESIAN_POINT ( 'NONE',  ( -20.75514604977248823, 25.07500000273120122, -28.56700777964554305 ) ) ;
#16713=CARTESIAN_POINT ( 'NONE',  ( -32.50000000000000000, 24.60000000546236620, 10.55989012756946366 ) ) ;
#16715=CARTESIAN_POINT ( 'NONE',  ( -4.300734207923759378, 76.47500000273119269, -13.23629886949340495 ) ) ;
#16716=CARTESIAN_POINT ( 'NONE',  ( -1.778240108872766143E-15, 65.50000000000000000, -32.49999999999999289 ) ) ;
#16717=CARTESIAN_POINT ( 'NONE',  ( -26.29305231718578995, 28.70000000546238539, 19.10302069950538595 ) ) ;
#16721=CARTESIAN_POINT ( 'NONE',  ( -13.91746824999999532, 74.77500000273117564, -4.522059556121115875 ) ) ;
#16723=CARTESIAN_POINT ( 'NONE',  ( 20.75514604977249178, 15.82500000273117102, 28.56700777964553950 ) ) ;
#16727=CARTESIAN_POINT ( 'NONE',  ( 33.58253175000000113, 6.375000002731168181, -4.112674001490185761E-15 ) ) ;
#16730=LINE ( 'NONE', #6251, #13284 ) ;
#16731=CARTESIAN_POINT ( 'NONE',  ( 4.300734207923757602, 74.77500000273118985, -13.23629886949340673 ) ) ;
#16733=CARTESIAN_POINT ( 'NONE',  ( 32.50000000000000000, 63.10000000000001563, -10.55989012756945833 ) ) ;
#16734=CARTESIAN_POINT ( 'NONE',  ( 10.37757302488624056, 48.52500000273118985, -31.93888565452638417 ) ) ;
#16736=ORIENTED_EDGE ( 'NONE', *, *, #9990, .T. ) ;
#16738=CARTESIAN_POINT ( 'NONE',  ( -10.04305231718578462, 2.400000000000013234, 30.90933677959249337 ) ) ;
#16739=CARTESIAN_POINT ( 'NONE',  ( 7.236395654485760609, 7.024999997268799312, -22.27133577429736633 ) ) ;
#16743=CARTESIAN_POINT ( 'NONE',  ( -26.29305231718579350, 42.30000000546238681, -19.10302069950537884 ) ) ;
#16746=CARTESIAN_POINT ( 'NONE',  ( -20.75514604977248823, 59.07500000273119412, -28.56700777964554305 ) ) ;
#16748=CARTESIAN_POINT ( 'NONE',  ( 33.58253175000000113, 76.12500000273119838, -4.112674001490185761E-15 ) ) ;
#16750=CARTESIAN_POINT ( 'NONE',  ( 7.570916362186207671, 5.599999999999994316, 23.30088464923126779 ) ) ;
#16751=CARTESIAN_POINT ( 'NONE',  ( 33.58253175000000113, 4.475000002731183812, -10.91162601494193751 ) ) ;
#16752=CARTESIAN_POINT ( 'NONE',  ( -10.37757302488623701, 17.52500000273118985, 31.93888565452638417 ) ) ;
#16753=DIRECTION ( 'NONE',  ( 0.000000000000000000, -1.000000000000000000, 0.000000000000000000 ) ) ;
#16755=CARTESIAN_POINT ( 'NONE',  ( -4.300734207923759378, 72.97500000273119269, -13.23629886949340495 ) ) ;
#16758=CARTESIAN_POINT ( 'NONE',  ( 5.147494310547426899, 49.94874572391552903, -32.50000000000000000 ) ) ;
#16760=CARTESIAN_POINT ( 'NONE',  ( -20.75514604977248823, 34.82500000273118701, -28.56700777964554305 ) ) ;
#16763=CARTESIAN_POINT ( 'NONE',  ( 20.75514604977249178, 30.07500000273118701, 28.56700777964553950 ) ) ;
#16767=CARTESIAN_POINT ( 'NONE',  ( -4.635254915624211769, 75.59999999999999432, -14.26584774442730286 ) ) ;
#16770=CARTESIAN_POINT ( 'NONE',  ( 23.41746824999999887, 2.524999997268799312, 7.608796670333735079 ) ) ;
#16774=CARTESIAN_POINT ( 'NONE',  ( -12.13525491562421088, 76.05000000546239391, -8.816778784387096835 ) ) ;
#16775=CARTESIAN_POINT ( 'NONE',  ( -20.75514604977248823, 20.82500000273119056, -28.56700777964554305 ) ) ;
#16776=CARTESIAN_POINT ( 'NONE',  ( 18.94512977948576093, 5.324999997268820451, -13.76444248337722875 ) ) ;
#16781=EDGE_CURVE ( 'NONE', #7065, #8583, #11378, .T. ) ;
#16785=CARTESIAN_POINT ( 'NONE',  ( -32.50000000000000000, 9.899999999999979039, -10.55989012756945300 ) ) ;
#16786=CARTESIAN_POINT ( 'NONE',  ( 7.570916362186213000, 14.14999999453761603, -23.30088464923126423 ) ) ;
#16787=ADVANCED_FACE ( 'NONE', ( #6157 ), #21458, .T. ) ;
#16788=CARTESIAN_POINT ( 'NONE',  ( 18.94512977948575738, 8.424999997268811214, 13.76444248337723408 ) ) ;
#16789=CARTESIAN_POINT ( 'NONE',  ( 27.16883889988623935, 30.57500000273119412, -19.73931689729374384 ) ) ;
#16790=CARTESIAN_POINT ( 'NONE',  ( 10.04305231718579705, 33.10000000546236976, 30.90933677959248982 ) ) ;
#16791=CARTESIAN_POINT ( 'NONE',  ( 6.277390505771533514E-15, 74.50000000000000000, 34.17252228774368916 ) ) ;
#16792=CARTESIAN_POINT ( 'NONE',  ( -10.04305231718578462, 6.900000005462370467, 30.90933677959249337 ) ) ;
#16793=CARTESIAN_POINT ( 'NONE',  ( -7.570916362186215665, 11.39999999999999325, 23.30088464923126423 ) ) ;
#16795=CARTESIAN_POINT ( 'NONE',  ( -2.162160676586881955E-15, 38.87500000273120548, -35.31076352940723240 ) ) ;
#16797=( BOUNDED_CURVE ( )  B_SPLINE_CURVE ( 2, ( #15599, #31364, #5115, #15248, #2191, #21087, #7687, #7521, #292, #18515, #23316, #12665, #2887 ),
 .UNSPECIFIED., .F., .T. ) 
 B_SPLINE_CURVE_WITH_KNOTS ( ( 3, 2, 2, 2, 2, 2, 3 ),
 ( 0.4722222222222222099, 0.4777777777777778012, 0.4888888888888888729, 0.5000000000000000000, 0.5111111111111110716, 0.5222222222222222543, 0.5277777777777777901 ),
 .UNSPECIFIED. ) 
 CURVE ( )  GEOMETRIC_REPRESENTATION_ITEM ( )  RATIONAL_B_SPLINE_CURVE ( ( 0.9755282581475765991, 0.9755282581475765991, 1.000000000000000000, 0.9510565162951535312, 1.000000000000000000, 0.9510565162951535312, 1.000000000000000000, 0.9510565162951535312, 1.000000000000000000, 0.9510565162951535312, 1.000000000000000000, 0.9755282581475768211, 0.9755282581475768211 ) ) 
 REPRESENTATION_ITEM ( '' )  );
#16799=CARTESIAN_POINT ( 'NONE',  ( -23.41746825000000598, 8.224999997268824359, 7.608796670333726198 ) ) ;
#16800=CARTESIAN_POINT ( 'NONE',  ( 26.29305231718578995, 17.19999999999999218, -19.10302069950538240 ) ) ;
#16804=CARTESIAN_POINT ( 'NONE',  ( -20.75514604977248112, 63.42500000273118133, 28.56700777964554661 ) ) ;
#16805=CARTESIAN_POINT ( 'NONE',  ( -33.58253175000000113, 45.27500000273117564, -10.91162601494193041 ) ) ;
#16808=CARTESIAN_POINT ( 'NONE',  ( 20.75514604977248467, 8.425000002731204418, -28.56700777964554305 ) ) ;
#16810=CARTESIAN_POINT ( 'NONE',  ( 26.29305231718578995, 25.70000000546238184, -19.10302069950538240 ) ) ;
#16814=CARTESIAN_POINT ( 'NONE',  ( -5.147494310547423346, 18.94874572391552903, 32.50000000000000000 ) ) ;
#16816=FACE_OUTER_BOUND ( 'NONE', #26828, .T. ) ;
#16821=ORIENTED_EDGE ( 'NONE', *, *, #23007, .F. ) ;
#16826=VERTEX_POINT ( 'NONE', #1505 ) ;
#16829=AXIS2_PLACEMENT_3D ( 'NONE', #32292, #9458, #8786 ) ;
#16831=CARTESIAN_POINT ( 'NONE',  ( -10.04305231718579172, 46.10000000546238397, -30.90933677959248982 ) ) ;
#16832=CARTESIAN_POINT ( 'NONE',  ( -10.37757302488623701, 49.77500000273118985, 31.93888565452638417 ) ) ;
#16833=CARTESIAN_POINT ( 'NONE',  ( -20.08610463437156923, 48.80000000546235128, 27.64615127144130113 ) ) ;
#16835=CARTESIAN_POINT ( 'NONE',  ( -20.75514604977248112, 31.42500000273120619, 28.56700777964554661 ) ) ;
#16837=CARTESIAN_POINT ( 'NONE',  ( 33.58253175000000113, 62.37500000273119127, -4.112674001490185761E-15 ) ) ;
#16839=CARTESIAN_POINT ( 'NONE',  ( -32.50000000000000000, 36.10000000000000142, 10.55989012756946366 ) ) ;
#16841=CARTESIAN_POINT ( 'NONE',  ( -2.162160676586881955E-15, 4.875000002731200155, -35.31076352940723240 ) ) ;
#16844=CARTESIAN_POINT ( 'NONE',  ( -2.162160676586882350E-15, 64.87500000273119838, -35.31076352940722529 ) ) ;
#16845=LINE ( 'NONE', #11349, #18788 ) ;
#16848=CARTESIAN_POINT ( 'NONE',  ( 15.14183272437242245, 6.049999994537625270, -20.84094480462497856 ) ) ;
#16850=CARTESIAN_POINT ( 'NONE',  ( 9.270509831248425314, 74.70000000000000284, 12.75976212528059683 ) ) ;
#16858=CARTESIAN_POINT ( 'NONE',  ( 0.000000000000000000, 0.000000000000000000, 0.000000000000000000 ) ) ;
#16860=CARTESIAN_POINT ( 'NONE',  ( 0.000000000000000000, 0.000000000000000000, 0.000000000000000000 ) ) ;
#16869=CARTESIAN_POINT ( 'NONE',  ( -26.29305231718578995, 74.70000000546239960, 19.10302069950538595 ) ) ;
#16870=CARTESIAN_POINT ( 'NONE',  ( 33.58253175000000823, 58.02500000273117564, 10.91162601494192863 ) ) ;
#16872=CARTESIAN_POINT ( 'NONE',  ( 32.50000000000000000, 11.60000000546236798, -10.55989012756945833 ) ) ;
#16874=CARTESIAN_POINT ( 'NONE',  ( 1.507698388325705758E-15, 13.62499999726882649, -24.62258325217400312 ) ) ;
#16875=CARTESIAN_POINT ( 'NONE',  ( -10.04305231718578462, 62.40000000000001279, 30.90933677959249337 ) ) ;
#16876=CARTESIAN_POINT ( 'NONE',  ( 27.16883889988623935, 20.57500000273118701, -19.73931689729374384 ) ) ;
#16879=CARTESIAN_POINT ( 'NONE',  ( -4.300734207923755825, 75.27500000273118985, 13.23629886949340673 ) ) ;
#16881=CARTESIAN_POINT ( 'NONE',  ( 20.08610463437157279, 15.29999999999998472, -27.64615127144129758 ) ) ;
#16883=EDGE_LOOP ( 'NONE', ( #16485, #3667, #32087, #24948 ) ) ;
#16885=FACE_OUTER_BOUND ( 'NONE', #25341, .T. ) ;
#16887=CARTESIAN_POINT ( 'NONE',  ( 27.16883889988624290, 15.92500000273117067, 19.73931689729373673 ) ) ;
#16891=CARTESIAN_POINT ( 'NONE',  ( 20.75514604977249178, 10.07500000273117990, 28.56700777964553950 ) ) ;
#16895=( BOUNDED_CURVE ( )  B_SPLINE_CURVE ( 2, ( #10781, #31703, #8030, #10610, #18346, #12667, #18516, #31198, #15424, #23317, #28790, #7522, #118 ),
 .UNSPECIFIED., .F., .T. ) 
 B_SPLINE_CURVE_WITH_KNOTS ( ( 3, 2, 2, 2, 2, 2, 3 ),
 ( 0.7115384615384615641, 0.7128205128205128416, 0.7153846153846153966, 0.7179487179487179516, 0.7205128205128205066, 0.7230769230769230616, 0.7243589743589743390 ),
 .UNSPECIFIED. ) 
 CURVE ( )  GEOMETRIC_REPRESENTATION_ITEM ( )  RATIONAL_B_SPLINE_CURVE ( ( 0.9755282581475768211, 0.9755282581475768211, 1.000000000000000000, 0.9510565162951535312, 1.000000000000000000, 0.9510565162951535312, 1.000000000000000000, 0.9510565162951535312, 1.000000000000000000, 0.9510565162951535312, 1.000000000000000000, 0.9755282581475768211, 0.9755282581475768211 ) ) 
 REPRESENTATION_ITEM ( '' )  );
#16896=CARTESIAN_POINT ( 'NONE',  ( 13.91746824999999532, 74.47500000273117848, -4.522059556121118540 ) ) ;
#16898=CARTESIAN_POINT ( 'NONE',  ( -15.14183272437242778, 3.049999994537633263, 20.84094480462497856 ) ) ;
#16899=CARTESIAN_POINT ( 'NONE',  ( -33.58253175000000113, 51.12500000273117706, 0.000000000000000000 ) ) ;
#16901=VERTEX_POINT ( 'NONE', #14734 ) ;
#16903=CARTESIAN_POINT ( 'NONE',  ( -5.147494310547423346, 2.448745718453165132, 32.50000000000000000 ) ) ;
#16904=CARTESIAN_POINT ( 'NONE',  ( 14.47279130897151589, 8.324999997268818674, 19.92008829642072953 ) ) ;
#16911=CARTESIAN_POINT ( 'NONE',  ( -10.37757302488623701, 59.77500000273119696, 31.93888565452638417 ) ) ;
#16912=CARTESIAN_POINT ( 'NONE',  ( 20.08610463437158344, 69.20000000546237118, 27.64615127144129403 ) ) ;
#16913=CARTESIAN_POINT ( 'NONE',  ( 27.16883889988624290, 73.92500000273119554, 19.73931689729373673 ) ) ;
#16916=CARTESIAN_POINT ( 'NONE',  ( -4.732186688966233175E-15, 3.500000000000005329, 25.76082449383753925 ) ) ;
#16917=CARTESIAN_POINT ( 'NONE',  ( 27.16883889988623935, 4.575000002731199444, -19.73931689729374384 ) ) ;
#16918=CARTESIAN_POINT ( 'NONE',  ( 33.58253175000000113, 16.22500000273118914, -10.91162601494193751 ) ) ;
#16919=CARTESIAN_POINT ( 'NONE',  ( 8.601468415847516980, 74.17500000273119554, -11.83890561707634603 ) ) ;
#16921=CARTESIAN_POINT ( 'NONE',  ( 11.25946833292375793, 72.57500000273120122, -8.180482586598735395 ) ) ;
#16927=CARTESIAN_POINT ( 'NONE',  ( -1.778240108872766143E-15, 71.50000000000001421, -32.49999999999999289 ) ) ;
#16929=CARTESIAN_POINT ( 'NONE',  ( -2.162160676586881955E-15, 38.62500000273118417, -35.31076352940723240 ) ) ;
#16932=CARTESIAN_POINT ( 'NONE',  ( -10.37757302488623701, 29.77500000273120051, 31.93888565452638417 ) ) ;
#16937=CARTESIAN_POINT ( 'NONE',  ( 26.29305231718579350, 78.79999999999998295, 19.10302069950537529 ) ) ;
#16939=CARTESIAN_POINT ( 'NONE',  ( 14.47279130897151767, 8.324999997268818674, 19.92008829642072953 ) ) ;
#16941=CARTESIAN_POINT ( 'NONE',  ( -20.08610463437156923, 52.80000000546237260, 27.64615127144130113 ) ) ;
#16944=CARTESIAN_POINT ( 'NONE',  ( -27.16883889988623935, 11.32500000273117813, 19.73931689729374739 ) ) ;
#16945=CARTESIAN_POINT ( 'NONE',  ( -14.47279130897152122, 4.424999997268826313, 19.92008829642072243 ) ) ;
#16954=CARTESIAN_POINT ( 'NONE',  ( -15.14183272437242600, 19.04999999453762172, 20.84094480462497856 ) ) ;
#16955=CARTESIAN_POINT ( 'NONE',  ( -14.47279130897151589, 3.324999997268803131, -19.92008829642072598 ) ) ;
#16956=CARTESIAN_POINT ( 'NONE',  ( 33.58253175000000113, 22.47500000273119625, -10.91162601494193751 ) ) ;
#16957=CARTESIAN_POINT ( 'NONE',  ( -10.04305231718579172, 30.10000000546236976, -30.90933677959248982 ) ) ;
#16958=CARTESIAN_POINT ( 'NONE',  ( -32.50000000000000000, 73.90000000000003411, -10.55989012756945478 ) ) ;
#16959=CARTESIAN_POINT ( 'NONE',  ( 32.50000000000000711, 47.40000000546237402, 10.55989012756945122 ) ) ;
#16960=CARTESIAN_POINT ( 'NONE',  ( 12.13525491562420910, 73.19999999999998863, -8.816778784387098611 ) ) ;
#16962=CARTESIAN_POINT ( 'NONE',  ( 33.58253175000000823, 38.27500000273118985, 10.91162601494192863 ) ) ;
#16965=CARTESIAN_POINT ( 'NONE',  ( 7.236395654485755280, 10.72499999726880837, 22.27133577429736988 ) ) ;
#16966=CARTESIAN_POINT ( 'NONE',  ( 32.50000000000000000, 17.00000000000001421, -3.980102097228898626E-15 ) ) ;
#16969=CARTESIAN_POINT ( 'NONE',  ( 10.37757302488624767, 53.72500000273117138, 31.93888565452638417 ) ) ;
#16970=CARTESIAN_POINT ( 'NONE',  ( 20.75514604977248467, 44.67500000273118843, -28.56700777964554305 ) ) ;
#16972=CARTESIAN_POINT ( 'NONE',  ( 26.29305231718578995, 67.70000000546238539, -19.10302069950538240 ) ) ;
#16973=CARTESIAN_POINT ( 'NONE',  ( 10.37757302488624056, 8.525000002731180970, -31.93888565452638417 ) ) ;
#16975=EDGE_CURVE ( 'NONE', #19688, #33879, #16895, .T. ) ;
#16979=CARTESIAN_POINT ( 'NONE',  ( 32.50000000000000000, 67.10000000000000853, -10.55989012756945833 ) ) ;
#16980=FACE_OUTER_BOUND ( 'NONE', #32753, .T. ) ;
#16984=FILL_AREA_STYLE ('',( #32414 ) ) ;
#16985=CARTESIAN_POINT ( 'NONE',  ( -27.16883889988623935, 31.32500000273119412, 19.73931689729374739 ) ) ;
#16990=ORIENTED_EDGE ( 'NONE', *, *, #16405, .T. ) ;
#16995=CARTESIAN_POINT ( 'NONE',  ( 10.04305231718579705, 20.60000000000000853, 30.90933677959248982 ) ) ;
#16996=CARTESIAN_POINT ( 'NONE',  ( 33.58253175000000113, 42.37500000273119838, -4.112674001490185761E-15 ) ) ;
#16997=CARTESIAN_POINT ( 'NONE',  ( -26.29305231718578995, 52.70000000546237828, 19.10302069950538595 ) ) ;
#16998=( BOUNDED_CURVE ( )  B_SPLINE_CURVE ( 2, ( #21826, #1198, #29866, #24722, #29688, #14100, #27131, #32273, #5868, #24070, #8766, #16346, #11510 ),
 .UNSPECIFIED., .F., .T. ) 
 B_SPLINE_CURVE_WITH_KNOTS ( ( 3, 2, 2, 2, 2, 2, 3 ),
 ( 0.9166666666666666297, 0.9222222222222222765, 0.9333333333333333481, 0.9444444444444444198, 0.9555555555555556024, 0.9666666666666666741, 0.9722222222222222099 ),
 .UNSPECIFIED. ) 
 CURVE ( )  GEOMETRIC_REPRESENTATION_ITEM ( )  RATIONAL_B_SPLINE_CURVE ( ( 0.9755282581475768211, 0.9755282581475765991, 1.000000000000000000, 0.9510565162951535312, 1.000000000000000000, 0.9510565162951535312, 1.000000000000000000, 0.9510565162951535312, 1.000000000000000000, 0.9510565162951535312, 1.000000000000000000, 0.9755282581475768211, 0.9755282581475768211 ) ) 
 REPRESENTATION_ITEM ( '' )  );
#17000=CARTESIAN_POINT ( 'NONE',  ( 27.16883889988623935, 32.32500000273119412, -19.73931689729374384 ) ) ;
#17002=CARTESIAN_POINT ( 'NONE',  ( 33.58253175000000113, 54.37500000273118417, -4.112674001490185761E-15 ) ) ;
#17003=FILL_AREA_STYLE ('',( #21652 ) ) ;
#17005=CARTESIAN_POINT ( 'NONE',  ( -2.092463501923844636E-15, 31.49999999999999289, -34.17252228774368916 ) ) ;
#17007=CARTESIAN_POINT ( 'NONE',  ( -10.37757302488623701, 73.52500000273121827, 31.93888565452638417 ) ) ;
#17008=CARTESIAN_POINT ( 'NONE',  ( 0.000000000000000000, 80.00000000000001421, 0.000000000000000000 ) ) ;
#17010=CARTESIAN_POINT ( 'NONE',  ( -20.75514604977248112, 65.67500000273116711, 28.56700777964554661 ) ) ;
#17011=CARTESIAN_POINT ( 'NONE',  ( 2.067204126564591252E-14, 4.249999994537631665, -24.50000000000000000 ) ) ;
#17012=CARTESIAN_POINT ( 'NONE',  ( -19.82091636218621034, 2.549999994537616388, -14.40073868116559552 ) ) ;
#17014=EDGE_CURVE ( 'NONE', #14163, #29502, #2568, .T. ) ;
#17015=CARTESIAN_POINT ( 'NONE',  ( 5.779280353836490358E-15, 11.00000000546238077, 32.49999999999999289 ) ) ;
#17026=CARTESIAN_POINT ( 'NONE',  ( -20.08610463437157989, 57.70000000000000995, -27.64615127144129758 ) ) ;
#17027=CARTESIAN_POINT ( 'NONE',  ( -15.14183272437242067, 4.449999994537617631, -20.84094480462497856 ) ) ;
#17028=ORIENTED_EDGE ( 'NONE', *, *, #1791, .F. ) ;
#17032=VERTEX_POINT ( 'NONE', #20915 ) ;
#17036=CARTESIAN_POINT ( 'NONE',  ( -1.778240108872766143E-15, 55.49999999999999289, -32.49999999999999289 ) ) ;
#17037=CARTESIAN_POINT ( 'NONE',  ( 33.58253175000000113, 50.12500000273117706, -4.112674001490185761E-15 ) ) ;
#17039=CARTESIAN_POINT ( 'NONE',  ( 32.50000000000000000, 11.50000000546236301, -3.980102097228898626E-15 ) ) ;
#17040=CARTESIAN_POINT ( 'NONE',  ( -10.04305231718578462, 8.400000000000018119, 30.90933677959249337 ) ) ;
#17041=CARTESIAN_POINT ( 'NONE',  ( -7.236395654485763274, 14.52499999726880553, 22.27133577429736633 ) ) ;
#17042=CARTESIAN_POINT ( 'NONE',  ( 20.08610463437158344, 52.69999999999998863, 27.64615127144129403 ) ) ;
#17043=CARTESIAN_POINT ( 'NONE',  ( 27.16883889988624290, 26.17500000273118133, 19.73931689729373673 ) ) ;
#17046=CARTESIAN_POINT ( 'NONE',  ( -11.25946833292375793, 75.07500000273120122, 8.180482586598737171 ) ) ;
#17047=CARTESIAN_POINT ( 'NONE',  ( 0.000000000000000000, 80.00000000000001421, -32.50000000000000000 ) ) ;
#17052=DIRECTION ( 'NONE',  ( 0.000000000000000000, 0.000000000000000000, -1.000000000000000000 ) ) ;
#17053=AXIS2_PLACEMENT_3D ( 'NONE', #31370, #18010, #4948 ) ;
#17058=CARTESIAN_POINT ( 'NONE',  ( 20.75514604977249178, 8.075000002731185234, 28.56700777964553950 ) ) ;
#17062=CARTESIAN_POINT ( 'NONE',  ( -4.300734207923755825, 77.77500000273118985, 13.23629886949340673 ) ) ;
#17066=CARTESIAN_POINT ( 'NONE',  ( -10.37757302488623701, 49.52500000273118985, 31.93888565452638417 ) ) ;
#17070=CARTESIAN_POINT ( 'NONE',  ( 10.04305231718578817, 43.39999999999999147, -30.90933677959249337 ) ) ;
#17071=CARTESIAN_POINT ( 'NONE',  ( -4.523095164977116484E-15, 14.12499999726881050, 24.62258325217400312 ) ) ;
#17073=ORIENTED_EDGE ( 'NONE', *, *, #4845, .T. ) ;
#17075=DIRECTION ( 'NONE',  ( 0.000000000000000000, 1.000000000000000000, 0.000000000000000000 ) ) ;
#17076=EDGE_CURVE ( 'NONE', #31503, #10494, #27816, .T. ) ;
#17077=ORIENTED_EDGE ( 'NONE', *, *, #27400, .T. ) ;
#17079=CARTESIAN_POINT ( 'NONE',  ( 10.37757302488624056, 58.77500000273119696, -31.93888565452638417 ) ) ;
#17081=CARTESIAN_POINT ( 'NONE',  ( -20.75514604977248823, 64.82500000273120122, -28.56700777964554305 ) ) ;
#17083=CARTESIAN_POINT ( 'NONE',  ( -7.570916362186210335, 8.599999999999996092, -23.30088464923126779 ) ) ;
#17084=CARTESIAN_POINT ( 'NONE',  ( 27.16883889988623935, 2.575000002731198112, -19.73931689729374384 ) ) ;
#17085=CARTESIAN_POINT ( 'NONE',  ( 33.58253175000000823, 14.02500000273117209, 10.91162601494192863 ) ) ;
#17086=CARTESIAN_POINT ( 'NONE',  ( -4.300734207923759378, 72.47500000273119269, -13.23629886949340495 ) ) ;
#17089=CARTESIAN_POINT ( 'NONE',  ( -11.25946833292375793, 71.57500000273120122, 8.180482586598737171 ) ) ;
#17091=CARTESIAN_POINT ( 'NONE',  ( -12.13525491562421088, 74.05000000546237970, -8.816778784387096835 ) ) ;
#17093=CARTESIAN_POINT ( 'NONE',  ( -12.13525491562421088, 78.05000000546239391, -8.816778784387096835 ) ) ;
#17096=CARTESIAN_POINT ( 'NONE',  ( 10.37757302488624056, 40.52500000273118275, -31.93888565452638417 ) ) ;
#17099=CARTESIAN_POINT ( 'NONE',  ( -33.58253175000000113, 29.27500000273118630, -10.91162601494193041 ) ) ;
#17100=CARTESIAN_POINT ( 'NONE',  ( 10.04305231718578817, 41.39999999999999147, -30.90933677959249337 ) ) ;
#17102=DIRECTION ( 'NONE',  ( 0.000000000000000000, 0.000000000000000000, -1.000000000000000000 ) ) ;
#17105=CARTESIAN_POINT ( 'NONE',  ( -4.523095164977117273E-15, 14.12499999726881050, 24.62258325217400312 ) ) ;
#17110=CARTESIAN_POINT ( 'NONE',  ( -20.75514604977248823, 10.82500000273118701, -28.56700777964554305 ) ) ;
#17111=CARTESIAN_POINT ( 'NONE',  ( -18.94512977948576093, 14.32499999726882756, 13.76444248337722698 ) ) ;
#17113=ADVANCED_FACE ( 'NONE', ( #2192 ), #33602, .F. ) ;
#17117=EDGE_LOOP ( 'NONE', ( #310, #3441, #13493, #3436 ) ) ;
#17120=CARTESIAN_POINT ( 'NONE',  ( 32.50000000000000711, 38.89999999999999147, 10.55989012756945122 ) ) ;
#17121=CARTESIAN_POINT ( 'NONE',  ( 24.50000000000000355, 15.84999999453763664, -7.960532557706203605 ) ) ;
#17123=CARTESIAN_POINT ( 'NONE',  ( -18.94512977948576093, 5.824999997268820451, 13.76444248337722698 ) ) ;
#17124=CARTESIAN_POINT ( 'NONE',  ( 33.58253175000000823, 24.27500000273120051, 10.91162601494192863 ) ) ;
#17125=CARTESIAN_POINT ( 'NONE',  ( -32.50000000000000000, 26.40000000546236336, -10.55989012756945478 ) ) ;
#17126=VECTOR ( 'NONE', #4265, 1000.000000000000000 ) ;
#17127=CARTESIAN_POINT ( 'NONE',  ( 32.50000000000000000, 75.09999999999999432, -10.55989012756945833 ) ) ;
#17131=CARTESIAN_POINT ( 'NONE',  ( -27.16883889988623935, 39.57500000273117280, 19.73931689729374739 ) ) ;
#17135=EDGE_CURVE ( 'NONE', #7428, #29891, #5269, .T. ) ;
#17137=CARTESIAN_POINT ( 'NONE',  ( 14.47279130897151589, 12.82499999726882400, 19.92008829642072953 ) ) ;
#17138=CARTESIAN_POINT ( 'NONE',  ( -32.50000000000000000, 15.89999999999999147, -10.55989012756945478 ) ) ;
#17141=CARTESIAN_POINT ( 'NONE',  ( 33.58253175000000113, 56.12500000273118417, -4.112674001490185761E-15 ) ) ;
#17142=CARTESIAN_POINT ( 'NONE',  ( 6.486482029760648627E-15, 47.87500000273117706, 35.31076352940722529 ) ) ;
#17144=CARTESIAN_POINT ( 'NONE',  ( 26.29305231718579350, 67.30000000546237970, 19.10302069950537529 ) ) ;
#17145=CARTESIAN_POINT ( 'NONE',  ( -10.04305231718578462, 50.39999999999999858, 30.90933677959249337 ) ) ;
#17151=CARTESIAN_POINT ( 'NONE',  ( 2.667360163309149608E-15, 78.00000000546238255, -32.50000000000000000 ) ) ;
#17154=CARTESIAN_POINT ( 'NONE',  ( 5.147494310547426899, 35.44874571845313227, -32.50000000000000000 ) ) ;
#17155=VECTOR ( 'NONE', #14737, 1000.000000000000000 ) ;
#17156=CARTESIAN_POINT ( 'NONE',  ( 33.58253175000000113, 32.12500000273119127, -4.112674001490185761E-15 ) ) ;
#17157=CARTESIAN_POINT ( 'NONE',  ( -33.58253175000000113, 65.47500000273117848, 10.91162601494193929 ) ) ;
#17159=ORIENTED_EDGE ( 'NONE', *, *, #17836, .T. ) ;
#17160=VECTOR ( 'NONE', #21201, 1000.000000000000000 ) ;
#17169=CARTESIAN_POINT ( 'NONE',  ( -33.58253175000000113, 41.47500000273117138, 10.91162601494193929 ) ) ;
#17170=CARTESIAN_POINT ( 'NONE',  ( -20.08610463437156923, 44.80000000546235839, 27.64615127144130113 ) ) ;
#17172=CARTESIAN_POINT ( 'NONE',  ( 20.75514604977249178, 29.82500000273119767, 28.56700777964553950 ) ) ;
#17173=CARTESIAN_POINT ( 'NONE',  ( 15.14183272437242067, 13.44999999453762385, 20.84094480462498211 ) ) ;
#17174=CARTESIAN_POINT ( 'NONE',  ( 10.37757302488624056, 52.77500000273118985, -31.93888565452638417 ) ) ;
#17176=CARTESIAN_POINT ( 'NONE',  ( 26.29305231718578995, 31.20000000000000639, -19.10302069950538240 ) ) ;
#17178=CARTESIAN_POINT ( 'NONE',  ( 10.37757302488624767, 77.72500000273119269, 31.93888565452638417 ) ) ;
#17181=CARTESIAN_POINT ( 'NONE',  ( -27.16883889988623935, 63.57500000273119412, 19.73931689729374739 ) ) ;
#17184=ORIENTED_EDGE ( 'NONE', *, *, #14259, .F. ) ;
#17185=CARTESIAN_POINT ( 'NONE',  ( 24.50000000000000355, 3.649999994537613812, 7.960532557706212486 ) ) ;
#17197=( BOUNDED_CURVE ( )  B_SPLINE_CURVE ( 2, ( #10668, #31757, #21147, #5688, #31589, #18575, #29016, #5852, #15997, #26621, #16331, #3117, #26787 ),
 .UNSPECIFIED., .F., .T. ) 
 B_SPLINE_CURVE_WITH_KNOTS ( ( 3, 2, 2, 2, 2, 2, 3 ),
 ( 0.05769230769230769551, 0.05897435897435897301, 0.06153846153846154188, 0.06410256410256409687, 0.06666666666666666574, 0.06923076923076923461, 0.07051282051282051211 ),
 .UNSPECIFIED. ) 
 CURVE ( )  GEOMETRIC_REPRESENTATION_ITEM ( )  RATIONAL_B_SPLINE_CURVE ( ( 0.9755282581475768211, 0.9755282581475768211, 1.000000000000000000, 0.9510565162951535312, 1.000000000000000000, 0.9510565162951535312, 1.000000000000000000, 0.9510565162951535312, 1.000000000000000000, 0.9510565162951535312, 1.000000000000000000, 0.9755282581475768211, 0.9755282581475768211 ) ) 
 REPRESENTATION_ITEM ( '' )  );
#17198=CARTESIAN_POINT ( 'NONE',  ( -26.29305231718578995, 58.20000000000000284, 19.10302069950538595 ) ) ;
#17201=CARTESIAN_POINT ( 'NONE',  ( 7.890940483122900408E-14, 16.49999999999999645, -24.50000000000000000 ) ) ;
#17203=EDGE_LOOP ( 'NONE', ( #32497, #3684, #14969, #14449, #27444, #7062, #29804, #5302, #28391, #2303, #18737, #14079, #16821, #16614, #29049, #2793, #26328, #9832, #29842, #33491, #26161, #29629, #14490, #16162, #13870, #5048, #16186, #26493, #8168, #18943, #18901, #31719, #16246, #25061, #20728, #26941, #21022, #6302, #20309, #14118, #13434, #3848, #6553, #21732, #30472, #20997, #14750, #20071, #561, #3324, #14576, #11718, #11618, #22060, #13709, #24623, #15096, #26304, #13953, #9506, #24419, #19520, #17719, #16388, #27238, #22008, #7995, #32218, #11407, #3500, #21358, #26537, #398, #6591, #10184, #27409, #27194, #15011, #17372, #16693, #7579, #31383 ) ) ;
#17206=ORIENTED_EDGE ( 'NONE', *, *, #2377, .F. ) ;
#17207=CARTESIAN_POINT ( 'NONE',  ( -2.162160676586881955E-15, 50.62500000273118417, -35.31076352940723240 ) ) ;
#17208=CARTESIAN_POINT ( 'NONE',  ( 26.29305231718578995, 55.70000000546237828, -19.10302069950538240 ) ) ;
#17209=DIRECTION ( 'NONE',  ( -0.000000000000000000, 0.000000000000000000, -1.000000000000000000 ) ) ;
#17211=CARTESIAN_POINT ( 'NONE',  ( -10.04305231718578462, 12.90000000546237580, 30.90933677959249337 ) ) ;
#17213=CARTESIAN_POINT ( 'NONE',  ( 23.41746824999999887, 15.12499999726882294, 0.000000000000000000 ) ) ;
#17214=CARTESIAN_POINT ( 'NONE',  ( 26.29305231718578995, 51.19999999999999574, -19.10302069950538240 ) ) ;
#17216=CARTESIAN_POINT ( 'NONE',  ( -27.16883889988624290, 17.17500000273119909, -19.73931689729374028 ) ) ;
#17219=CARTESIAN_POINT ( 'NONE',  ( -13.91746824999999532, 76.97500000273119269, 4.522059556121122093 ) ) ;
#17221=CARTESIAN_POINT ( 'NONE',  ( 20.08610463437157279, 53.80000000546237970, -27.64615127144129758 ) ) ;
#17223=ORIENTED_EDGE ( 'NONE', *, *, #21026, .T. ) ;
#17229=CARTESIAN_POINT ( 'NONE',  ( 10.37757302488624767, 11.97500000273118914, 31.93888565452638417 ) ) ;
#17232=CARTESIAN_POINT ( 'NONE',  ( 20.08610463437158344, 2.700000000000001954, 27.64615127144129403 ) ) ;
#17235=CARTESIAN_POINT ( 'NONE',  ( 33.58253175000000113, 50.12500000273117706, -4.112674001490185761E-15 ) ) ;
#17240=CARTESIAN_POINT ( 'NONE',  ( 5.779280353836490358E-15, 58.49999999999999289, 32.49999999999999289 ) ) ;
#17241=CARTESIAN_POINT ( 'NONE',  ( -23.41746825000000598, 11.72499999726882614, 7.608796670333726198 ) ) ;
#17243=VERTEX_POINT ( 'NONE', #3226 ) ;
#17249=CARTESIAN_POINT ( 'NONE',  ( -2.162160676586881955E-15, 60.87500000273116996, -35.31076352940723240 ) ) ;
#17251=CARTESIAN_POINT ( 'NONE',  ( 10.37757302488624767, 67.72500000273117848, 31.93888565452638417 ) ) ;
#17253=CARTESIAN_POINT ( 'NONE',  ( -7.570916362186210335, 12.59999999999999964, -23.30088464923126779 ) ) ;
#17254=CARTESIAN_POINT ( 'NONE',  ( -33.58253175000000113, 5.475000002731181148, 10.91162601494193929 ) ) ;
#17255=CARTESIAN_POINT ( 'NONE',  ( -27.16883889988624290, 12.92500000273116889, -19.73931689729374028 ) ) ;
#17256=CARTESIAN_POINT ( 'NONE',  ( 13.91746824999999532, 71.97500000273120691, -4.522059556121118540 ) ) ;
#17259=CARTESIAN_POINT ( 'NONE',  ( 20.08610463437158344, 22.70000000000000995, 27.64615127144129403 ) ) ;
#17261=CARTESIAN_POINT ( 'NONE',  ( 15.00000000000000000, 77.35000000546237686, -4.873795443493596835 ) ) ;
#17263=CARTESIAN_POINT ( 'NONE',  ( 33.58253175000000113, 38.22500000273119269, -10.91162601494193751 ) ) ;
#17266=CARTESIAN_POINT ( 'NONE',  ( 10.37757302488624056, 28.77500000273120051, -31.93888565452638417 ) ) ;
#17270=CARTESIAN_POINT ( 'NONE',  ( 5.147494310547428675, 78.55125428154684641, 32.50000000000000000 ) ) ;
#17272=CARTESIAN_POINT ( 'NONE',  ( -23.41746825000000243, 9.724999997268803043, 7.608796670333725309 ) ) ;
#17277=CARTESIAN_POINT ( 'NONE',  ( -10.37757302488623701, 15.52500000273118808, 31.93888565452638417 ) ) ;
#17278=CARTESIAN_POINT ( 'NONE',  ( 7.236395654485755280, 10.72499999726880837, 22.27133577429736988 ) ) ;
#17283=ORIENTED_EDGE ( 'NONE', *, *, #13886, .T. ) ;
#17287=CARTESIAN_POINT ( 'NONE',  ( -15.14183272437241889, 14.44999999453762207, -20.84094480462497856 ) ) ;
#17288=CARTESIAN_POINT ( 'NONE',  ( 1.507698388325705758E-15, 13.12499999726881228, -24.62258325217400312 ) ) ;
#17289=CARTESIAN_POINT ( 'NONE',  ( 10.37757302488624767, 21.97500000273119980, 31.93888565452638417 ) ) ;
#17291=CARTESIAN_POINT ( 'NONE',  ( 20.08610463437158344, 27.20000000546237118, 27.64615127144129403 ) ) ;
#17293=CARTESIAN_POINT ( 'NONE',  ( -32.50000000000000000, 70.10000000000000853, 10.55989012756946366 ) ) ;
#17294=CARTESIAN_POINT ( 'NONE',  ( -10.04305231718579172, 6.100000005462375086, -30.90933677959248982 ) ) ;
#17297=CARTESIAN_POINT ( 'NONE',  ( -33.58253175000000113, 37.27500000273119696, -10.91162601494193218 ) ) ;
#17301=CARTESIAN_POINT ( 'NONE',  ( -23.41746824999999887, 8.124999997268817609, -2.867812753649727150E-15 ) ) ;
#17302=CARTESIAN_POINT ( 'NONE',  ( 10.04305231718578817, 17.39999999999999858, -30.90933677959249337 ) ) ;
#17303=CARTESIAN_POINT ( 'NONE',  ( 32.50000000000000000, 9.500000005462361230, -3.980102097228898626E-15 ) ) ;
#17305=CARTESIAN_POINT ( 'NONE',  ( 10.37757302488624767, 55.72500000273117138, 31.93888565452638417 ) ) ;
#17306=AXIS2_PLACEMENT_3D ( 'NONE', #24553, #8599, #32101 ) ;
#17307=CARTESIAN_POINT ( 'NONE',  ( -20.75514604977248112, 47.67500000273118843, 28.56700777964554661 ) ) ;
#17308=CARTESIAN_POINT ( 'NONE',  ( 0.000000000000000000, 80.00000000000001421, 0.000000000000000000 ) ) ;
#17309=CARTESIAN_POINT ( 'NONE',  ( 24.50000000000000000, 9.900000000000007461, 7.960532557706212486 ) ) ;
#17310=CARTESIAN_POINT ( 'NONE',  ( 27.16883889988624290, 1.925000002731186433, 19.73931689729373673 ) ) ;
#17316=CARTESIAN_POINT ( 'NONE',  ( 3.445340210940985210E-14, 9.249999994537636994, 24.50000000000000000 ) ) ;
#17317=CARTESIAN_POINT ( 'NONE',  ( 20.08610463437158344, 41.20000000546236407, 27.64615127144129403 ) ) ;
#17320=CARTESIAN_POINT ( 'NONE',  ( -33.58253175000000113, 33.22500000273117138, 10.91162601494193929 ) ) ;
#17321=CARTESIAN_POINT ( 'NONE',  ( 33.58253175000000823, 64.27500000273118985, 10.91162601494192863 ) ) ;
#17333=CARTESIAN_POINT ( 'NONE',  ( 5.779280353836490358E-15, 56.49999999999998579, 32.49999999999999289 ) ) ;
#17334=CARTESIAN_POINT ( 'NONE',  ( 10.37757302488624767, 41.97500000273118559, 31.93888565452638417 ) ) ;
#17335=CARTESIAN_POINT ( 'NONE',  ( -2.092463501923844636E-15, 44.00000000546238965, -34.17252228774368916 ) ) ;
#17336=EDGE_CURVE ( 'NONE', #11703, #26987, #13860, .T. ) ;
#17338=CARTESIAN_POINT ( 'NONE',  ( -27.16883889988624290, 30.92500000273118488, -19.73931689729374028 ) ) ;
#17339=CARTESIAN_POINT ( 'NONE',  ( 7.570916362186207671, 13.34999999453762065, 23.30088464923126779 ) ) ;
#17340=CARTESIAN_POINT ( 'NONE',  ( 27.16883889988623935, 54.57500000273118701, -19.73931689729374384 ) ) ;
#17342=CARTESIAN_POINT ( 'NONE',  ( 32.50000000000000000, 31.10000000000000497, -10.55989012756945833 ) ) ;
#17344=CARTESIAN_POINT ( 'NONE',  ( 33.58253175000000823, 78.02500000273118985, 10.91162601494192863 ) ) ;
#17347=CARTESIAN_POINT ( 'NONE',  ( -2.162160676586882350E-15, 66.87500000273119838, -35.31076352940722529 ) ) ;
#17349=EDGE_CURVE ( 'NONE', #4016, #21770, #23921, .T. ) ;
#17351=CARTESIAN_POINT ( 'NONE',  ( 7.570916362186213000, 12.14999999453764090, -23.30088464923126423 ) ) ;
#17365=CARTESIAN_POINT ( 'NONE',  ( -10.04305231718578462, 72.90000000546237402, 30.90933677959249337 ) ) ;
#17368=LINE ( 'NONE', #30051, #11891 ) ;
#17370=CARTESIAN_POINT ( 'NONE',  ( 33.58253175000000113, 72.47500000273119269, -10.91162601494193751 ) ) ;
#17372=ORIENTED_EDGE ( 'NONE', *, *, #25226, .F. ) ;
#17374=CARTESIAN_POINT ( 'NONE',  ( -2.092463501923844636E-15, 60.00000000546238255, -34.17252228774368916 ) ) ;
#17375=VERTEX_POINT ( 'NONE', #3390 ) ;
#17376=CARTESIAN_POINT ( 'NONE',  ( -15.14183272437242067, 12.44999999453762918, -20.84094480462497856 ) ) ;
#17377=CARTESIAN_POINT ( 'NONE',  ( -27.16883889988624290, 50.92500000273120264, -19.73931689729374028 ) ) ;
#17378=CARTESIAN_POINT ( 'NONE',  ( 7.236395654485755280, 16.22499999726881370, 22.27133577429736988 ) ) ;
#17379=CARTESIAN_POINT ( 'NONE',  ( -1.778240108872766143E-15, 17.50000000000000000, -32.49999999999999289 ) ) ;
#17380=CARTESIAN_POINT ( 'NONE',  ( -20.08610463437156923, 2.800000005462385477, 27.64615127144130113 ) ) ;
#17382=CARTESIAN_POINT ( 'NONE',  ( -7.236395654485757944, 13.72499999726881015, -22.27133577429736988 ) ) ;
#17383=CARTESIAN_POINT ( 'NONE',  ( -10.04305231718578462, 52.40000000000000568, 30.90933677959249337 ) ) ;
#17385=CARTESIAN_POINT ( 'NONE',  ( -10.37757302488623701, 15.77500000273118808, 31.93888565452638417 ) ) ;
#17386=CARTESIAN_POINT ( 'NONE',  ( -15.14183272437242778, 7.300000000000001599, 20.84094480462497856 ) ) ;
#17388=CARTESIAN_POINT ( 'NONE',  ( -11.25946833292375793, 73.07500000273120122, 8.180482586598737171 ) ) ;
#17393=VERTEX_POINT ( 'NONE', #29125 ) ;
#17400=CARTESIAN_POINT ( 'NONE',  ( -10.04305231718578462, 20.40000000000000213, 30.90933677959249337 ) ) ;
#17404=EDGE_CURVE ( 'NONE', #16018, #25987, #27408, .T. ) ;
#17405=CARTESIAN_POINT ( 'NONE',  ( -13.91746824999999887, 71.37500000273119838, 0.000000000000000000 ) ) ;
#17407=CARTESIAN_POINT ( 'NONE',  ( 27.16883889988624290, 49.92500000273120264, 19.73931689729373673 ) ) ;
#17410=CARTESIAN_POINT ( 'NONE',  ( -1.778240108872766143E-15, 22.00000000546237899, -32.49999999999999289 ) ) ;
#17413=DIRECTION ( 'NONE',  ( -0.000000000000000000, -1.000000000000000000, -0.000000000000000000 ) ) ;
#17414=CARTESIAN_POINT ( 'NONE',  ( -18.94512977948576093, 9.824999997268824004, 13.76444248337722698 ) ) ;
#17416=ORIENTED_EDGE ( 'NONE', *, *, #3887, .F. ) ;
#17419=CARTESIAN_POINT ( 'NONE',  ( 7.570916362186213000, 6.399999999999988809, -23.30088464923126423 ) ) ;
#17420=ORIENTED_EDGE ( 'NONE', *, *, #17983, .T. ) ;
#17423=CARTESIAN_POINT ( 'NONE',  ( -27.16883889988623935, 67.32500000273117280, 19.73931689729374739 ) ) ;
#17425=CARTESIAN_POINT ( 'NONE',  ( 15.14183272437241889, 15.69999999999999929, 20.84094480462498211 ) ) ;
#17426=CARTESIAN_POINT ( 'NONE',  ( -27.16883889988623935, 3.575000002731199000, 19.73931689729374739 ) ) ;
#17427=CARTESIAN_POINT ( 'NONE',  ( 33.58253175000000113, 10.12500000273119838, -4.112674001490185761E-15 ) ) ;
#17428=CARTESIAN_POINT ( 'NONE',  ( 4.300734207923757602, 74.27500000273118985, -13.23629886949340673 ) ) ;
#17430=CARTESIAN_POINT ( 'NONE',  ( -9.657523855033125146E-16, 73.50000000000001421, -15.77193336357400710 ) ) ;
#17432=CARTESIAN_POINT ( 'NONE',  ( 20.08610463437157279, 19.80000000546237615, -27.64615127144129758 ) ) ;
#17435=CARTESIAN_POINT ( 'NONE',  ( -9.270509831248425314, 77.95000000546237118, -12.75976212528059861 ) ) ;
#17437=CARTESIAN_POINT ( 'NONE',  ( -33.58253175000000113, 35.22500000273119980, 10.91162601494193929 ) ) ;
#17438=DIRECTION ( 'NONE',  ( 0.000000000000000000, 0.000000000000000000, -1.000000000000000000 ) ) ;
#17440=CARTESIAN_POINT ( 'NONE',  ( -33.58253175000000113, 19.27500000273117919, -10.91162601494193041 ) ) ;
#17441=CARTESIAN_POINT ( 'NONE',  ( 3.980102097228898626E-15, 80.00000000000001421, 32.50000000000000000 ) ) ;
#17444=EDGE_CURVE ( 'NONE', #19766, #14943, #30918, .T. ) ;
#17445=CARTESIAN_POINT ( 'NONE',  ( 2.667360163309149608E-15, 79.50000000000001421, -32.50000000000000000 ) ) ;
#17447=CARTESIAN_POINT ( 'NONE',  ( 14.47279130897151944, 10.92499999726882365, -19.92008829642072598 ) ) ;
#17453=CARTESIAN_POINT ( 'NONE',  ( -2.162160676586882350E-15, 12.62500000273118772, -35.31076352940722529 ) ) ;
#17454=CARTESIAN_POINT ( 'NONE',  ( -23.41746825000000598, 10.22499999726881903, 7.608796670333726198 ) ) ;
#17459=VERTEX_POINT ( 'NONE', #33205 ) ;
#17462=CARTESIAN_POINT ( 'NONE',  ( -5.147494310547403806, 72.05125428700921475, -32.50000000000000711 ) ) ;
#17463=CARTESIAN_POINT ( 'NONE',  ( 23.41746824999999887, 5.124999997268814056, 0.000000000000000000 ) ) ;
#17464=CARTESIAN_POINT ( 'NONE',  ( 18.94512977948576093, 10.82499999726882578, -13.76444248337722875 ) ) ;
#17465=CARTESIAN_POINT ( 'NONE',  ( 6.486482029760649416E-15, 23.87500000273117706, 35.31076352940723240 ) ) ;
#17466=CARTESIAN_POINT ( 'NONE',  ( -20.08610463437157989, 22.20000000546238184, -27.64615127144129758 ) ) ;
#17467=CARTESIAN_POINT ( 'NONE',  ( 32.50000000000000000, 69.09999999999998010, -10.55989012756945833 ) ) ;
#17468=CARTESIAN_POINT ( 'NONE',  ( 5.779280353836490358E-15, 47.00000000546238255, 32.49999999999999289 ) ) ;
#17471=CARTESIAN_POINT ( 'NONE',  ( 6.486482029760649416E-15, 35.87500000273118417, 35.31076352940723240 ) ) ;
#17472=CARTESIAN_POINT ( 'NONE',  ( -26.29305231718578995, 32.70000000546238539, 19.10302069950538595 ) ) ;
#17474=CARTESIAN_POINT ( 'NONE',  ( 23.41746825000000243, 15.02499999726881086, 7.608796670333735079 ) ) ;
#17475=CARTESIAN_POINT ( 'NONE',  ( -26.29305231718579350, 15.79999999999998117, -19.10302069950537884 ) ) ;
#17476=CARTESIAN_POINT ( 'NONE',  ( -32.50000000000000000, 52.10000000000001563, 10.55989012756946366 ) ) ;
#17478=CARTESIAN_POINT ( 'NONE',  ( -33.58253175000000113, 59.02500000273120406, -10.91162601494193218 ) ) ;
#17480=CARTESIAN_POINT ( 'NONE',  ( -33.58253175000000113, 49.27500000273118985, -10.91162601494193041 ) ) ;
#17482=CARTESIAN_POINT ( 'NONE',  ( 5.779280353836490358E-15, 37.00000000546237544, 32.49999999999999289 ) ) ;
#17483=CARTESIAN_POINT ( 'NONE',  ( -32.50000000000000000, 6.000000000000005329, 0.000000000000000000 ) ) ;
#17486=CARTESIAN_POINT ( 'NONE',  ( 7.570916362186207671, 3.599999999999992095, 23.30088464923126779 ) ) ;
#17488=CARTESIAN_POINT ( 'NONE',  ( 5.779280353836490358E-15, 66.49999999999998579, 32.49999999999999289 ) ) ;
#17490=CARTESIAN_POINT ( 'NONE',  ( -26.29305231718579350, 78.30000000546239391, -19.10302069950537884 ) ) ;
#17493=CARTESIAN_POINT ( 'NONE',  ( -32.50000000000000000, 60.60000000546239107, 10.55989012756946366 ) ) ;
#17494=CARTESIAN_POINT ( 'NONE',  ( -27.16883889988624290, 34.92500000273118843, -19.73931689729374028 ) ) ;
#17499=CARTESIAN_POINT ( 'NONE',  ( -20.08610463437157989, 16.20000000546236762, -27.64615127144129758 ) ) ;
#17500=ORIENTED_EDGE ( 'NONE', *, *, #9880, .T. ) ;
#17505=CARTESIAN_POINT ( 'NONE',  ( -20.08610463437156923, 46.29999999999999716, 27.64615127144130113 ) ) ;
#17506=CARTESIAN_POINT ( 'NONE',  ( 27.16883889988623935, 38.57500000273117280, -19.73931689729374384 ) ) ;
#17507=CARTESIAN_POINT ( 'NONE',  ( -32.50000000000000000, 46.60000000546237686, 10.55989012756946366 ) ) ;
#17508=EDGE_CURVE ( 'NONE', #31882, #684, #7870, .T. ) ;
#17510=CARTESIAN_POINT ( 'NONE',  ( 10.37757302488624767, 29.72500000273120691, 31.93888565452638417 ) ) ;
#17512=CARTESIAN_POINT ( 'NONE',  ( -27.16883889988624290, 57.17500000273118133, -19.73931689729374028 ) ) ;
#17514=CARTESIAN_POINT ( 'NONE',  ( -10.04305231718578462, 34.39999999999998437, 30.90933677959249337 ) ) ;
#17516=CARTESIAN_POINT ( 'NONE',  ( 6.486482029760649416E-15, 77.62500000273121259, 35.31076352940723240 ) ) ;
#17519=CARTESIAN_POINT ( 'NONE',  ( 20.75514604977249178, 66.07500000273118701, 28.56700777964553950 ) ) ;
#17521=ORIENTED_EDGE ( 'NONE', *, *, #32906, .T. ) ;
#17522=CARTESIAN_POINT ( 'NONE',  ( -20.75514604977248823, 20.82500000273119412, -28.56700777964554305 ) ) ;
#17524=CARTESIAN_POINT ( 'NONE',  ( -15.14183272437242600, 11.04999999453761284, 20.84094480462497856 ) ) ;
#17535=CARTESIAN_POINT ( 'NONE',  ( -5.147494310547322094, 57.55125428154683931, -32.50000000000003553 ) ) ;
#17537=CARTESIAN_POINT ( 'NONE',  ( 6.277390505771533514E-15, 73.00000000546239676, 34.17252228774368916 ) ) ;
#17542=CARTESIAN_POINT ( 'NONE',  ( 33.58253175000000823, 76.27500000273118985, 10.91162601494192863 ) ) ;
#17547=CARTESIAN_POINT ( 'NONE',  ( 26.29305231718579350, 63.30000000546237260, 19.10302069950537529 ) ) ;
#17549=CARTESIAN_POINT ( 'NONE',  ( 5.779280353836490358E-15, 56.49999999999998579, 32.49999999999999289 ) ) ;
#17550=CARTESIAN_POINT ( 'NONE',  ( 10.37757302488624056, 50.52500000273118985, -31.93888565452638417 ) ) ;
#17551=CARTESIAN_POINT ( 'NONE',  ( 20.08610463437157279, 55.80000000546236549, -27.64615127144129758 ) ) ;
#17552=CARTESIAN_POINT ( 'NONE',  ( 20.08610463437157279, 7.800000005462373487, -27.64615127144129758 ) ) ;
#17553=EDGE_CURVE ( 'NONE', #15317, #24251, #14887, .T. ) ;
#17554=CARTESIAN_POINT ( 'NONE',  ( -12.13525491562421088, 77.80000000000001137, -8.816778784387096835 ) ) ;
#17555=CYLINDRICAL_SURFACE ( 'NONE', #3460, 32.50000000000000000 ) ;
#17556=CARTESIAN_POINT ( 'NONE',  ( -2.092463501923844636E-15, 51.50000000000000711, -34.17252228774368916 ) ) ;
#17558=CARTESIAN_POINT ( 'NONE',  ( 20.75514604977248467, 18.67500000273120264, -28.56700777964554305 ) ) ;
#17559=CARTESIAN_POINT ( 'NONE',  ( -32.50000000000000000, 73.90000000000001990, -10.55989012756945300 ) ) ;
#17561=CARTESIAN_POINT ( 'NONE',  ( 8.601468415847520532, 78.07500000273117280, 11.83890561707634781 ) ) ;
#17567=CARTESIAN_POINT ( 'NONE',  ( 20.08610463437157279, 71.80000000546239391, -27.64615127144129758 ) ) ;
#17572=CARTESIAN_POINT ( 'NONE',  ( -33.58253175000000113, 3.275000002731191628, -10.91162601494193041 ) ) ;
#17576=CARTESIAN_POINT ( 'NONE',  ( 10.04305231718578817, 3.400000000000014122, -30.90933677959249337 ) ) ;
#17578=CARTESIAN_POINT ( 'NONE',  ( -10.37757302488624411, 42.72500000273119269, -31.93888565452638417 ) ) ;
#17583=CARTESIAN_POINT ( 'NONE',  ( 32.50000000000000000, 42.99999999999998579, -3.980102097228898626E-15 ) ) ;
#17584=CARTESIAN_POINT ( 'NONE',  ( -18.94512977948575738, 13.42499999726881654, -13.76444248337723231 ) ) ;
#17590=CARTESIAN_POINT ( 'NONE',  ( 33.58253175000000113, 66.12500000273119838, -4.112674001490185761E-15 ) ) ;
#17592=CARTESIAN_POINT ( 'NONE',  ( -24.50000000000000000, 13.00000000000001066, -3.000384657911015469E-15 ) ) ;
#17593=CARTESIAN_POINT ( 'NONE',  ( 23.41746824999999887, 3.224999997268806151, -7.608796670333727974 ) ) ;
#17594=CARTESIAN_POINT ( 'NONE',  ( -27.16883889988623935, 9.325000002731176352, 19.73931689729374739 ) ) ;
#17595=CARTESIAN_POINT ( 'NONE',  ( -15.14183272437242067, 6.449999994537612302, -20.84094480462497856 ) ) ;
#17597=CARTESIAN_POINT ( 'NONE',  ( -4.635254915624211769, 73.59999999999999432, -14.26584774442730286 ) ) ;
#17599=CARTESIAN_POINT ( 'NONE',  ( 32.50000000000000000, 19.50000000546236834, -3.980102097228898626E-15 ) ) ;
#17600=CARTESIAN_POINT ( 'NONE',  ( -9.270509831248423538, 73.95000000546238539, -12.75976212528059861 ) ) ;
#17602=CARTESIAN_POINT ( 'NONE',  ( -12.13525491562420910, 76.45000000546237118, 8.816778784387098611 ) ) ;
#17604=CARTESIAN_POINT ( 'NONE',  ( 20.75514604977249178, 31.82500000273119056, 28.56700777964553950 ) ) ;
#17605=AXIS2_PLACEMENT_3D ( 'NONE', #5947, #23977, #29106 ) ;
#17607=CARTESIAN_POINT ( 'NONE',  ( 33.58253175000000113, 20.37500000273118062, -4.112674001490185761E-15 ) ) ;
#17609=CARTESIAN_POINT ( 'NONE',  ( -1.778240108872766143E-15, 8.000000005462370112, -32.49999999999999289 ) ) ;
#17610=CARTESIAN_POINT ( 'NONE',  ( 12.13525491562421088, 80.79999999999998295, 8.816778784387095058 ) ) ;
#17612=CARTESIAN_POINT ( 'NONE',  ( -23.41746824999999887, 9.624999997268817609, -2.867812753649727150E-15 ) ) ;
#17613=CARTESIAN_POINT ( 'NONE',  ( 6.486482029760648627E-15, 67.62500000273119838, 35.31076352940722529 ) ) ;
#17616=VECTOR ( 'NONE', #7068, 1000.000000000000000 ) ;
#17618=CARTESIAN_POINT ( 'NONE',  ( 33.58253175000000113, 12.12500000273120193, -4.112674001490185761E-15 ) ) ;
#17619=CARTESIAN_POINT ( 'NONE',  ( 23.41746825000000243, 13.02499999726881619, 7.608796670333735079 ) ) ;
#17621=VERTEX_POINT ( 'NONE', #1466 ) ;
#17624=ORIENTED_EDGE ( 'NONE', *, *, #29971, .F. ) ;
#17627=CARTESIAN_POINT ( 'NONE',  ( 7.313012447739250820E-14, 15.50000000000000178, 24.50000000000000000 ) ) ;
#17628=VECTOR ( 'NONE', #315, 1000.000000000000000 ) ;
#17630=CARTESIAN_POINT ( 'NONE',  ( 18.94512977948575738, 2.924999997268806773, 13.76444248337723408 ) ) ;
#17631=CARTESIAN_POINT ( 'NONE',  ( -23.41746825000000243, 9.524999997268810858, -7.608796670333730638 ) ) ;
#17632=CARTESIAN_POINT ( 'NONE',  ( -20.75514604977248823, 15.07500000273116747, -28.56700777964554305 ) ) ;
#17633=CARTESIAN_POINT ( 'NONE',  ( 10.04305231718578817, 21.90000000546238468, -30.90933677959249337 ) ) ;
#17634=EDGE_CURVE ( 'NONE', #20831, #7065, #18418, .T. ) ;
#17635=CARTESIAN_POINT ( 'NONE',  ( -26.29305231718578995, 68.19999999999998863, 19.10302069950538595 ) ) ;
#17639=CARTESIAN_POINT ( 'NONE',  ( -33.58253175000000113, 31.27500000273118275, -10.91162601494193218 ) ) ;
#17640=CARTESIAN_POINT ( 'NONE',  ( 11.25946833292375793, 80.17500000273119554, 8.180482586598731842 ) ) ;
#17643=CARTESIAN_POINT ( 'NONE',  ( -15.14183272437242067, 0.7000000000000070610, -20.84094480462497856 ) ) ;
#17644=CARTESIAN_POINT ( 'NONE',  ( -10.04305231718579172, 7.599999999999996092, -30.90933677959248982 ) ) ;
#17647=CARTESIAN_POINT ( 'NONE',  ( 20.75514604977248467, 56.42500000273120264, -28.56700777964554305 ) ) ;
#17649=CARTESIAN_POINT ( 'NONE',  ( 27.16883889988623935, 38.57500000273117280, -19.73931689729374384 ) ) ;
#17651=CARTESIAN_POINT ( 'NONE',  ( 15.14183272437242067, 9.700000000000013500, 20.84094480462498211 ) ) ;
#17658=LINE ( 'NONE', #25030, #17126 ) ;
#17661=CARTESIAN_POINT ( 'NONE',  ( -1.778240108872766143E-15, 35.49999999999998579, -32.49999999999999289 ) ) ;
#17662=CARTESIAN_POINT ( 'NONE',  ( 10.37757302488624767, 29.72500000273120691, 31.93888565452638417 ) ) ;
#17664=ORIENTED_EDGE ( 'NONE', *, *, #10417, .T. ) ;
#17665=EDGE_LOOP ( 'NONE', ( #18859, #23929, #1477, #2988 ) ) ;
#17668=CARTESIAN_POINT ( 'NONE',  ( -5.147494310547430452, 16.05125428700922541, -32.49999999999999289 ) ) ;
#17675=LINE ( 'NONE', #4793, #15768 ) ;
#17676=CARTESIAN_POINT ( 'NONE',  ( 27.16883889988624290, 42.17500000273119554, 19.73931689729373673 ) ) ;
#17677=CARTESIAN_POINT ( 'NONE',  ( -26.29305231718579350, 44.30000000546238681, -19.10302069950537884 ) ) ;
#17679=CARTESIAN_POINT ( 'NONE',  ( 20.75514604977249178, 19.82500000273119412, 28.56700777964553950 ) ) ;
#17680=CARTESIAN_POINT ( 'NONE',  ( 24.50000000000000000, 13.74999999453763166, 0.000000000000000000 ) ) ;
#17681=CARTESIAN_POINT ( 'NONE',  ( 10.37757302488624767, 53.97500000273119980, 31.93888565452638417 ) ) ;
#17683=ADVANCED_FACE ( 'NONE', ( #15898 ), #18135, .T. ) ;
#17685=ADVANCED_FACE ( 'NONE', ( #12973 ), #2843, .T. ) ;
#17686=CARTESIAN_POINT ( 'NONE',  ( -10.04305231718578462, 28.40000000000000924, 30.90933677959249337 ) ) ;
#17688=CARTESIAN_POINT ( 'NONE',  ( -2.162160676586881955E-15, 76.62500000273118417, -35.31076352940723240 ) ) ;
#17690=CARTESIAN_POINT ( 'NONE',  ( 5.779280353836490358E-15, 21.00000000546237544, 32.49999999999999289 ) ) ;
#17691=CARTESIAN_POINT ( 'NONE',  ( 33.58253175000000823, 60.27500000273116143, 10.91162601494192685 ) ) ;
#17694=CARTESIAN_POINT ( 'NONE',  ( -20.75514604977248112, 21.42500000273120264, 28.56700777964554661 ) ) ;
#17695=CARTESIAN_POINT ( 'NONE',  ( -7.570916362186210335, 8.349999994537615322, -23.30088464923126779 ) ) ;
#17702=EDGE_CURVE ( 'NONE', #24433, #31338, #25413, .T. ) ;
#17707=( BOUNDED_CURVE ( )  B_SPLINE_CURVE ( 2, ( #23496, #13362, #5124, #10109, #15611, #31206, #2556, #23325, #23836, #33954, #12675, #10447, #23664 ),
 .UNSPECIFIED., .F., .T. ) 
 B_SPLINE_CURVE_WITH_KNOTS ( ( 3, 2, 2, 2, 2, 2, 3 ),
 ( 0.4722222222222222099, 0.4777777777777778012, 0.4888888888888888729, 0.5000000000000000000, 0.5111111111111110716, 0.5222222222222222543, 0.5277777777777777901 ),
 .UNSPECIFIED. ) 
 CURVE ( )  GEOMETRIC_REPRESENTATION_ITEM ( )  RATIONAL_B_SPLINE_CURVE ( ( 0.9755282581475765991, 0.9755282581475765991, 1.000000000000000000, 0.9510565162951535312, 1.000000000000000000, 0.9510565162951535312, 1.000000000000000000, 0.9510565162951535312, 1.000000000000000000, 0.9510565162951535312, 1.000000000000000000, 0.9755282581475768211, 0.9755282581475768211 ) ) 
 REPRESENTATION_ITEM ( '' )  );
#17709=CARTESIAN_POINT ( 'NONE',  ( 26.29305231718578995, 63.70000000546238539, -19.10302069950538240 ) ) ;
#17710=CARTESIAN_POINT ( 'NONE',  ( -20.08610463437157989, 74.20000000546238539, -27.64615127144129758 ) ) ;
#17714=EDGE_LOOP ( 'NONE', ( #30935, #216, #6175, #21060 ) ) ;
#17715=CARTESIAN_POINT ( 'NONE',  ( -10.37757302488623701, 75.77500000273118985, 31.93888565452638417 ) ) ;
#17718=CARTESIAN_POINT ( 'NONE',  ( 20.08610463437157279, 61.80000000546237970, -27.64615127144129758 ) ) ;
#17719=ORIENTED_EDGE ( 'NONE', *, *, #17836, .F. ) ;
#17720=AXIS2_PLACEMENT_3D ( 'NONE', #5446, #18837, #20904 ) ;
#17721=CARTESIAN_POINT ( 'NONE',  ( -5.147494310547423346, 10.94874572391553436, 32.50000000000000000 ) ) ;
#17722=CARTESIAN_POINT ( 'NONE',  ( 27.16883889988623935, 46.32500000273117990, -19.73931689729374384 ) ) ;
#17723=CARTESIAN_POINT ( 'NONE',  ( 23.41746825000000243, 18.52499999726881441, 7.608796670333735079 ) ) ;
#17724=CARTESIAN_POINT ( 'NONE',  ( -20.08610463437157989, 8.200000005462390718, -27.64615127144129758 ) ) ;
#17726=CARTESIAN_POINT ( 'NONE',  ( -20.08610463437157989, 7.699999999999988631, -27.64615127144129758 ) ) ;
#17728=CARTESIAN_POINT ( 'NONE',  ( -32.50000000000000000, 54.10000000000000853, 10.55989012756946366 ) ) ;
#17730=CARTESIAN_POINT ( 'NONE',  ( -33.58253175000000113, 19.47500000273117493, 10.91162601494193929 ) ) ;
#17731=CARTESIAN_POINT ( 'NONE',  ( -26.29305231718579350, 24.30000000546236905, -19.10302069950537884 ) ) ;
#17733=CARTESIAN_POINT ( 'NONE',  ( 13.91746825000000065, 76.27500000273118985, 4.522059556121114987 ) ) ;
#17747=CARTESIAN_POINT ( 'NONE',  ( -8.601468415847515203, 73.67500000273120975, 11.83890561707634959 ) ) ;
#17749=CARTESIAN_POINT ( 'NONE',  ( 20.75514604977248467, 46.42500000273119554, -28.56700777964554305 ) ) ;
#17750=AXIS2_PLACEMENT_3D ( 'NONE', #31029, #2374, #18009 ) ;
#17752=CARTESIAN_POINT ( 'NONE',  ( 2.375766604868040144, 78.55125428154686062, 15.00000000000000178 ) ) ;
#17757=CARTESIAN_POINT ( 'NONE',  ( 33.58253175000000823, 74.27500000273117564, 10.91162601494192863 ) ) ;
#17763=CARTESIAN_POINT ( 'NONE',  ( 10.37757302488624056, 70.52500000273120406, -31.93888565452638417 ) ) ;
#17765=CARTESIAN_POINT ( 'NONE',  ( -24.50000000000000355, 10.90000000000000568, -7.960532557706207157 ) ) ;
#17766=LINE ( 'NONE', #20520, #27021 ) ;
#17767=EDGE_CURVE ( 'NONE', #28004, #24994, #20624, .T. ) ;
#17768=CARTESIAN_POINT ( 'NONE',  ( -27.16883889988624290, 10.92500000273119376, -19.73931689729374028 ) ) ;
#17771=CARTESIAN_POINT ( 'NONE',  ( -12.13525491562420910, 76.19999999999998863, 8.816778784387098611 ) ) ;
#17772=CLOSED_SHELL ( 'NONE', ( #7266, #19921, #24193, #23538, #10282, #29290, #12010, #11872, #27145, #3797, #22009, #31313, #21860, #16593, #20054, #3152, #26158, #6428, #18140, #14405, #29262, #15249, #18702, #22670, #15471, #32262, #6886, #1158, #15462, #33398, #11539, #17113, #7989, #19443, #13029, #5991, #20601, #13466, #21637, #5942, #22163, #33036, #12930, #26004, #14604, #10470, #10846, #20204, #23008, #28752, #16787, #27609, #31463, #12505, #1650, #28756, #25081, #15182, #19029, #20494, #10743, #27085, #19163, #10622, #31750, #19344, #19021, #32679, #23774, #33147, #28516, #14988, #319, #2241, #4129, #14075, #21961, #2957, #11460, #4115, #4220, #26624, #30637, #30300, #11864, #24062, #2443, #20158, #26568, #6630, #13881, #17685, #28797, #26010, #8825, #28940, #17982, #17683, #12406, #2964, #6740, #23919, #26148, #11453, #23163, #21633, #5960, #12655, #10836, #19222, #6928, #26286, #14817, #22621, #5944, #15015, #4328, #28330, #33862, #25951, #25812, #31074, #24156, #8365, #4182, #29168, #23624, #13980, #10427, #1585, #886, #31166, #3198, #20358, #11735 ) ) ;
#17775=CARTESIAN_POINT ( 'NONE',  ( 5.147494310547434893, 61.05125428700922896, 32.49999999999999289 ) ) ;
#17777=CARTESIAN_POINT ( 'NONE',  ( -4.635254915624211769, 79.85000000546239107, -14.26584774442730286 ) ) ;
#17779=CARTESIAN_POINT ( 'NONE',  ( -27.16883889988624290, 32.92500000273118843, -19.73931689729374028 ) ) ;
#17782=CARTESIAN_POINT ( 'NONE',  ( 33.58253175000000823, 24.27500000273119696, 10.91162601494192685 ) ) ;
#17783=CARTESIAN_POINT ( 'NONE',  ( -20.08610463437156923, 12.80000000546236016, 27.64615127144130113 ) ) ;
#17784=CARTESIAN_POINT ( 'NONE',  ( 33.58253175000000113, 74.22500000273119269, -10.91162601494193574 ) ) ;
#17785=CARTESIAN_POINT ( 'NONE',  ( 3.445340210940985210E-14, 7.499999999999994671, 24.50000000000000000 ) ) ;
#17787=CARTESIAN_POINT ( 'NONE',  ( -18.94512977948575738, 15.42499999726881832, -13.76444248337723231 ) ) ;
#17788=CARTESIAN_POINT ( 'NONE',  ( -20.75514604977248823, 66.82500000273118701, -28.56700777964554305 ) ) ;
#17793=CARTESIAN_POINT ( 'NONE',  ( -10.37757302488624411, 8.725000002731187365, -31.93888565452638417 ) ) ;
#17794=CARTESIAN_POINT ( 'NONE',  ( -7.236395654485757944, 13.72499999726881015, -22.27133577429736988 ) ) ;
#17798=( BOUNDED_CURVE ( )  B_SPLINE_CURVE ( 2, ( #27458, #18911, #32595, #3284, #11501, #6357, #21980, #1188, #29679, #19241, #1360, #32429, #29516 ),
 .UNSPECIFIED., .F., .T. ) 
 B_SPLINE_CURVE_WITH_KNOTS ( ( 3, 2, 2, 2, 2, 2, 3 ),
 ( 0.006410256410256410901, 0.007692307692307692735, 0.01025641025641025640, 0.01282051282051282007, 0.01538461538461538547, 0.01794871794871794740, 0.01923076923076923184 ),
 .UNSPECIFIED. ) 
 CURVE ( )  GEOMETRIC_REPRESENTATION_ITEM ( )  RATIONAL_B_SPLINE_CURVE ( ( 0.9755282581475768211, 0.9755282581475768211, 1.000000000000000000, 0.9510565162951535312, 1.000000000000000000, 0.9510565162951535312, 1.000000000000000000, 0.9510565162951535312, 1.000000000000000000, 0.9510565162951535312, 1.000000000000000000, 0.9755282581475767101, 0.9755282581475768211 ) ) 
 REPRESENTATION_ITEM ( '' )  );
#17799=ORIENTED_EDGE ( 'NONE', *, *, #13656, .F. ) ;
#17804=CARTESIAN_POINT ( 'NONE',  ( 0.000000000000000000, 82.00000000000001421, -15.00000000000000000 ) ) ;
#17805=CARTESIAN_POINT ( 'NONE',  ( 23.41746825000000243, 1.224999997268811480, -7.608796670333727974 ) ) ;
#17806=CARTESIAN_POINT ( 'NONE',  ( 1.507698388325705758E-15, 9.124999997268822938, -24.62258325217400312 ) ) ;
#17807=CARTESIAN_POINT ( 'NONE',  ( 33.58253175000000113, 14.37500000273117529, -4.112674001490185761E-15 ) ) ;
#17808=CARTESIAN_POINT ( 'NONE',  ( -32.50000000000000000, 26.50000000546237544, 0.000000000000000000 ) ) ;
#17809=CARTESIAN_POINT ( 'NONE',  ( -10.04305231718578462, 64.40000000000000568, 30.90933677959249337 ) ) ;
#17811=CARTESIAN_POINT ( 'NONE',  ( 0.000000000000000000, 80.00000000000001421, -32.50000000000000000 ) ) ;
#17813=CARTESIAN_POINT ( 'NONE',  ( 27.16883889988623935, 30.57500000273119412, -19.73931689729374384 ) ) ;
#17817=CARTESIAN_POINT ( 'NONE',  ( 7.236395654485755280, 18.72499999726881370, 22.27133577429736988 ) ) ;
#17818=CARTESIAN_POINT ( 'NONE',  ( -2.092463501923844636E-15, 5.500000000000000888, -34.17252228774368916 ) ) ;
#17820=CARTESIAN_POINT ( 'NONE',  ( -5.147494310547531704, 52.44874571845315359, 32.49999999999996447 ) ) ;
#17822=CARTESIAN_POINT ( 'NONE',  ( -10.37757302488623701, 47.52500000273118985, 31.93888565452638417 ) ) ;
#17824=CARTESIAN_POINT ( 'NONE',  ( 33.58253175000000113, 38.37500000273119838, -4.112674001490185761E-15 ) ) ;
#17825=DIRECTION ( 'NONE',  ( 0.000000000000000000, 0.000000000000000000, -1.000000000000000000 ) ) ;
#17829=CARTESIAN_POINT ( 'NONE',  ( -10.04305231718578462, 28.40000000000000924, 30.90933677959249337 ) ) ;
#17831=CARTESIAN_POINT ( 'NONE',  ( 1.555960095263670572E-15, 16.24999999453762101, -24.50000000000000000 ) ) ;
#17833=LINE ( 'NONE', #25551, #30258 ) ;
#17836=EDGE_CURVE ( 'NONE', #6801, #5893, #28918, .T. ) ;
#17837=CARTESIAN_POINT ( 'NONE',  ( -32.50000000000000000, 60.40000000546236691, -10.55989012756945300 ) ) ;
#17838=CARTESIAN_POINT ( 'NONE',  ( 27.16883889988623935, 28.32500000273119412, -19.73931689729374384 ) ) ;
#17839=AXIS2_PLACEMENT_3D ( 'NONE', #17308, #32893, #17825 ) ;
#17842=VERTEX_POINT ( 'NONE', #24287 ) ;
#17845=DIRECTION ( 'NONE',  ( 0.000000000000000000, 0.000000000000000000, 1.000000000000000000 ) ) ;
#17846=ORIENTED_EDGE ( 'NONE', *, *, #32075, .F. ) ;
#17849=ORIENTED_EDGE ( 'NONE', *, *, #14557, .T. ) ;
#17852=CARTESIAN_POINT ( 'NONE',  ( -2.165007332552593587E-13, 46.50000000000000711, 32.50000000000000000 ) ) ;
#17853=CARTESIAN_POINT ( 'NONE',  ( 20.75514604977249178, 34.07500000273117990, 28.56700777964553950 ) ) ;
#17854=CARTESIAN_POINT ( 'NONE',  ( -26.29305231718578995, 44.70000000546237118, 19.10302069950538595 ) ) ;
#17855=AXIS2_PLACEMENT_3D ( 'NONE', #17008, #11845, #27637 ) ;
#17857=CARTESIAN_POINT ( 'NONE',  ( 6.486482029760649416E-15, 25.62500000273118772, 35.31076352940723240 ) ) ;
#17858=CARTESIAN_POINT ( 'NONE',  ( 3.880418787951172011, 13.30125427608447097, 24.49999999999998579 ) ) ;
#17859=CARTESIAN_POINT ( 'NONE',  ( -2.162160676586881955E-15, 46.87500000273118417, -35.31076352940723240 ) ) ;
#17862=CARTESIAN_POINT ( 'NONE',  ( -32.50000000000000000, 30.00000000000000000, 0.000000000000000000 ) ) ;
#17864=CARTESIAN_POINT ( 'NONE',  ( 33.58253175000000113, 68.22500000273116427, -10.91162601494193751 ) ) ;
#17866=CARTESIAN_POINT ( 'NONE',  ( -24.50000000000000000, 14.89999999999999503, -7.960532557706207157 ) ) ;
#17867=CARTESIAN_POINT ( 'NONE',  ( -33.58253175000000113, 61.47500000273118559, 10.91162601494193929 ) ) ;
#17869=CARTESIAN_POINT ( 'NONE',  ( 26.29305231718579350, 72.79999999999999716, 19.10302069950537529 ) ) ;
#17870=CARTESIAN_POINT ( 'NONE',  ( -20.75514604977248112, 19.42500000273117777, 28.56700777964554661 ) ) ;
#17871=CARTESIAN_POINT ( 'NONE',  ( -24.50000000000001066, 10.84999999453761887, 7.960532557706201828 ) ) ;
#17873=CARTESIAN_POINT ( 'NONE',  ( 26.29305231718579350, 46.80000000000001137, 19.10302069950537529 ) ) ;
#17883=CARTESIAN_POINT ( 'NONE',  ( -24.50000000000000000, 2.649999994537616477, -7.960532557706207157 ) ) ;
#17886=CARTESIAN_POINT ( 'NONE',  ( -4.523095164977116484E-15, 2.624999997268825158, 24.62258325217400312 ) ) ;
#17887=CARTESIAN_POINT ( 'NONE',  ( -20.75514604977248112, 1.425000002731191984, 28.56700777964554661 ) ) ;
#17892=CARTESIAN_POINT ( 'NONE',  ( 27.16883889988623935, 72.57500000273120122, -19.73931689729374384 ) ) ;
#17895=CARTESIAN_POINT ( 'NONE',  ( -33.58253175000000113, 51.37500000273120548, 0.000000000000000000 ) ) ;
#17896=CARTESIAN_POINT ( 'NONE',  ( -20.08610463437156923, 60.80000000546239391, 27.64615127144130113 ) ) ;
#17897=ORIENTED_EDGE ( 'NONE', *, *, #21266, .F. ) ;
#17899=CARTESIAN_POINT ( 'NONE',  ( -33.58253175000000113, 45.22500000273117848, 10.91162601494193929 ) ) ;
#17900=CARTESIAN_POINT ( 'NONE',  ( -14.47279130897152122, 17.92499999726880588, 19.92008829642072243 ) ) ;
#17901=CARTESIAN_POINT ( 'NONE',  ( -10.37757302488624411, 70.97500000273119269, -31.93888565452638417 ) ) ;
#17902=CARTESIAN_POINT ( 'NONE',  ( -10.04305231718578462, 2.900000005462366470, 30.90933677959249337 ) ) ;
#17904=CYLINDRICAL_SURFACE ( 'NONE', #12777, 32.50000000000000000 ) ;
#17905=CARTESIAN_POINT ( 'NONE',  ( -20.08610463437157989, 45.69999999999998863, -27.64615127144129758 ) ) ;
#17907=CARTESIAN_POINT ( 'NONE',  ( 33.58253175000000113, 16.47500000273118204, -10.91162601494193751 ) ) ;
#17908=CARTESIAN_POINT ( 'NONE',  ( 1.555960095263670572E-15, 6.499999999999994671, -24.50000000000000000 ) ) ;
#17910=CARTESIAN_POINT ( 'NONE',  ( 13.91746824999999887, 80.37500000273118417, -1.704398294459741270E-15 ) ) ;
#17911=DIRECTION ( 'NONE',  ( -0.000000000000000000, -1.000000000000000000, -0.000000000000000000 ) ) ;
#17912=CARTESIAN_POINT ( 'NONE',  ( -10.04305231718578462, 44.39999999999999147, 30.90933677959249337 ) ) ;
#17913=( BOUNDED_CURVE ( )  B_SPLINE_CURVE ( 2, ( #18457, #26336, #2825, #13294, #23767, #234, #14300, #9298, #8972, #11545, #22522, #22358, #32805 ),
 .UNSPECIFIED., .F., .F. ) 
 B_SPLINE_CURVE_WITH_KNOTS ( ( 3, 2, 2, 2, 2, 2, 3 ),
 ( 0.9294871794871795156, 0.9307692307692307931, 0.9333333333333333481, 0.9358974358974359031, 0.9384615384615384581, 0.9410256410256410131, 0.9423076923076922906 ),
 .UNSPECIFIED. ) 
 CURVE ( )  GEOMETRIC_REPRESENTATION_ITEM ( )  RATIONAL_B_SPLINE_CURVE ( ( 0.9755282581475768211, 0.9755282581475768211, 1.000000000000000000, 0.9510565162951535312, 1.000000000000000000, 0.9510565162951535312, 1.000000000000000000, 0.9510565162951535312, 1.000000000000000000, 0.9510565162951535312, 1.000000000000000000, 0.9755282581475768211, 0.9755282581475768211 ) ) 
 REPRESENTATION_ITEM ( '' )  );
#17915=EDGE_LOOP ( 'NONE', ( #18442, #32869, #29141, #9941 ) ) ;
#17927=CARTESIAN_POINT ( 'NONE',  ( 26.29305231718578995, 3.199999999999980638, -19.10302069950538240 ) ) ;
#17929=CARTESIAN_POINT ( 'NONE',  ( -33.58253175000000113, 47.22500000273117138, 10.91162601494193929 ) ) ;
#17933=ORIENTED_EDGE ( 'NONE', *, *, #23007, .T. ) ;
#17937=CARTESIAN_POINT ( 'NONE',  ( -33.58253175000000113, 73.37500000273116996, 0.000000000000000000 ) ) ;
#17938=ORIENTED_EDGE ( 'NONE', *, *, #30695, .T. ) ;
#17942=CARTESIAN_POINT ( 'NONE',  ( -1.778240108872766143E-15, 24.00000000546237899, -32.49999999999999289 ) ) ;
#17943=CARTESIAN_POINT ( 'NONE',  ( -10.37757302488623701, 59.52500000273119696, 31.93888565452638417 ) ) ;
#17945=AXIS2_PLACEMENT_3D ( 'NONE', #11739, #27700, #9678 ) ;
#17946=CARTESIAN_POINT ( 'NONE',  ( 19.82091636218621034, 11.80000000000000426, 14.40073868116559730 ) ) ;
#17947=CARTESIAN_POINT ( 'NONE',  ( -23.41746824999999887, 4.124999997268813168, -2.867812753649727150E-15 ) ) ;
#17948=CARTESIAN_POINT ( 'NONE',  ( -33.58253175000000113, 9.125000002731198379, 0.000000000000000000 ) ) ;
#17949=CARTESIAN_POINT ( 'NONE',  ( 5.147494310547426899, 29.44874571845315714, -32.50000000000000000 ) ) ;
#17951=CARTESIAN_POINT ( 'NONE',  ( 4.635254915624212657, 76.59999999999999432, 14.26584774442730286 ) ) ;
#17952=FACE_OUTER_BOUND ( 'NONE', #705, .T. ) ;
#17953=CARTESIAN_POINT ( 'NONE',  ( 26.29305231718579350, 19.30000000546239391, 19.10302069950537529 ) ) ;
#17956=CARTESIAN_POINT ( 'NONE',  ( 8.601468415847520532, 79.57500000273120122, 11.83890561707634781 ) ) ;
#17958=CARTESIAN_POINT ( 'NONE',  ( -33.58253175000000113, 29.22500000273118914, 10.91162601494193929 ) ) ;
#17961=CARTESIAN_POINT ( 'NONE',  ( -27.16883889988624290, 21.17500000273120264, -19.73931689729374028 ) ) ;
#17963=CARTESIAN_POINT ( 'NONE',  ( 20.75514604977249178, 75.82500000273118701, 28.56700777964553950 ) ) ;
#17964=CARTESIAN_POINT ( 'NONE',  ( 5.779280353836490358E-15, 66.49999999999998579, 32.49999999999999289 ) ) ;
#17966=CARTESIAN_POINT ( 'NONE',  ( -7.236395654485757944, 15.22499999726881192, -22.27133577429736988 ) ) ;
#17967=CARTESIAN_POINT ( 'NONE',  ( -2.162160676586882350E-15, 62.62500000273117706, -35.31076352940722529 ) ) ;
#17970=CARTESIAN_POINT ( 'NONE',  ( -33.58253175000000113, 5.025000002731194293, -10.91162601494193041 ) ) ;
#17971=CARTESIAN_POINT ( 'NONE',  ( 14.47279130897151767, 2.924999997268815655, -19.92008829642072598 ) ) ;
#17973=EDGE_CURVE ( 'NONE', #969, #22307, #21215, .T. ) ;
#17974=VERTEX_POINT ( 'NONE', #11400 ) ;
#17981=CARTESIAN_POINT ( 'NONE',  ( -7.236395654485757944, 1.724999997268800156, -22.27133577429736988 ) ) ;
#17982=ADVANCED_FACE ( 'NONE', ( #16236 ), #16399, .T. ) ;
#17983=EDGE_CURVE ( 'NONE', #21829, #22725, #587, .T. ) ;
#17984=CARTESIAN_POINT ( 'NONE',  ( 18.94512977948575738, 10.42499999726881299, 13.76444248337723408 ) ) ;
#17985=CARTESIAN_POINT ( 'NONE',  ( 27.16883889988623935, 18.57500000273118346, -19.73931689729374384 ) ) ;
#17986=CARTESIAN_POINT ( 'NONE',  ( -10.04305231718578462, 16.90000000546237757, 30.90933677959249337 ) ) ;
#17987=CARTESIAN_POINT ( 'NONE',  ( -32.50000000000000000, 66.00000000000000000, 0.000000000000000000 ) ) ;
#17989=DIRECTION ( 'NONE',  ( -0.000000000000000000, 1.000000000000000000, -0.000000000000000000 ) ) ;
#17991=CARTESIAN_POINT ( 'NONE',  ( -2.162160676586881955E-15, 28.87500000273119838, -35.31076352940723240 ) ) ;
#17992=CARTESIAN_POINT ( 'NONE',  ( 5.779280353836490358E-15, 33.00000000546238965, 32.49999999999999289 ) ) ;
#17995=CARTESIAN_POINT ( 'NONE',  ( 14.47279130897151589, 16.82499999726881512, 19.92008829642072953 ) ) ;
#17996=CARTESIAN_POINT ( 'NONE',  ( -26.29305231718579350, 5.799999999999999822, -19.10302069950537884 ) ) ;
#17998=CARTESIAN_POINT ( 'NONE',  ( -15.00000000000000000, 74.10000000000000853, 4.873795443493597723 ) ) ;
#18000=CARTESIAN_POINT ( 'NONE',  ( 33.58253175000000113, 52.22500000273117848, -10.91162601494193751 ) ) ;
#18002=CARTESIAN_POINT ( 'NONE',  ( 6.486482029760648627E-15, 39.87500000273119127, 35.31076352940722529 ) ) ;
#18006=CARTESIAN_POINT ( 'NONE',  ( -2.165007332552593587E-13, 51.00000000546238255, 32.50000000000000000 ) ) ;
#18009=DIRECTION ( 'NONE',  ( 0.000000000000000000, 0.000000000000000000, 1.000000000000000000 ) ) ;
#18010=DIRECTION ( 'NONE',  ( -0.000000000000000000, -1.000000000000000000, -0.000000000000000000 ) ) ;
#18014=CARTESIAN_POINT ( 'NONE',  ( 26.29305231718579350, 10.80000000000000426, 19.10302069950537529 ) ) ;
#18015=CARTESIAN_POINT ( 'NONE',  ( -10.37757302488623701, 27.52500000273119696, 31.93888565452638417 ) ) ;
#18023=EDGE_LOOP ( 'NONE', ( #20249, #30867, #12728, #7700 ) ) ;
#18027=CARTESIAN_POINT ( 'NONE',  ( -33.58253175000000113, 33.27500000273120406, -10.91162601494193218 ) ) ;
#18028=CARTESIAN_POINT ( 'NONE',  ( -26.29305231718579350, 34.30000000546237970, -19.10302069950537884 ) ) ;
#18031=CARTESIAN_POINT ( 'NONE',  ( -27.16883889988623935, 21.32500000273118701, 19.73931689729374739 ) ) ;
#18032=CARTESIAN_POINT ( 'NONE',  ( 3.880418787951134707, 5.301254276084462980, 24.50000000000000000 ) ) ;
#18033=CARTESIAN_POINT ( 'NONE',  ( 27.16883889988623935, 46.57500000273117990, -19.73931689729374384 ) ) ;
#18035=CARTESIAN_POINT ( 'NONE',  ( 10.04305231718578817, 29.40000000000000924, -30.90933677959249337 ) ) ;
#18037=EDGE_CURVE ( 'NONE', #3193, #19899, #29420, .T. ) ;
#18038=CARTESIAN_POINT ( 'NONE',  ( -33.58253175000000113, 71.02500000273118985, -10.91162601494193218 ) ) ;
#18041=CARTESIAN_POINT ( 'NONE',  ( 27.16883889988623935, 62.57500000273119412, -19.73931689729374384 ) ) ;
#18042=FACE_OUTER_BOUND ( 'NONE', #1397, .T. ) ;
#18043=CARTESIAN_POINT ( 'NONE',  ( -20.75514604977248823, 8.825000002731190563, -28.56700777964554305 ) ) ;
#18048=CARTESIAN_POINT ( 'NONE',  ( 20.08610463437158344, 18.69999999999999574, 27.64615127144129403 ) ) ;
#18054=CARTESIAN_POINT ( 'NONE',  ( -20.08610463437157989, 76.20000000546235697, -27.64615127144129758 ) ) ;
#18059=CARTESIAN_POINT ( 'NONE',  ( -33.58253175000000113, 77.37500000273116996, 0.000000000000000000 ) ) ;
#18063=CARTESIAN_POINT ( 'NONE',  ( -33.58253175000000113, 53.27500000273117564, -10.91162601494193218 ) ) ;
#18064=CARTESIAN_POINT ( 'NONE',  ( -32.50000000000000000, 60.40000000546236691, -10.55989012756945478 ) ) ;
#18065=CARTESIAN_POINT ( 'NONE',  ( 33.58253175000000823, 44.02500000273118275, 10.91162601494192863 ) ) ;
#18067=CARTESIAN_POINT ( 'NONE',  ( -27.16883889988623935, 67.57500000273120122, 19.73931689729374739 ) ) ;
#18068=CARTESIAN_POINT ( 'NONE',  ( 32.50000000000000711, 7.400000005462386454, 10.55989012756945122 ) ) ;
#18070=CARTESIAN_POINT ( 'NONE',  ( 7.236395654485755280, 18.72499999726881370, 22.27133577429736988 ) ) ;
#18071=CARTESIAN_POINT ( 'NONE',  ( 10.04305231718578817, 45.39999999999999858, -30.90933677959249337 ) ) ;
#18072=CYLINDRICAL_SURFACE ( 'NONE', #613, 30.50000000000000000 ) ;
#18073=CARTESIAN_POINT ( 'NONE',  ( -33.58253175000000113, 9.275000002731177418, -10.91162601494193218 ) ) ;
#18074=CARTESIAN_POINT ( 'NONE',  ( -24.50000000000000711, 7.100000000000008527, 7.960532557706201828 ) ) ;
#18076=CARTESIAN_POINT ( 'NONE',  ( 8.601468415847520532, 80.07500000273118701, 11.83890561707634781 ) ) ;
#18078=CARTESIAN_POINT ( 'NONE',  ( 2.067204126564591252E-14, 4.499999999999996447, -24.50000000000000000 ) ) ;
#18081=VERTEX_POINT ( 'NONE', #11240 ) ;
#18093=DIRECTION ( 'NONE',  ( -0.000000000000000000, -1.000000000000000000, -0.000000000000000000 ) ) ;
#18094=CARTESIAN_POINT ( 'NONE',  ( -27.16883889988624290, 46.92500000273119554, -19.73931689729374028 ) ) ;
#18096=CARTESIAN_POINT ( 'NONE',  ( 2.375766604868043252, 79.44874571845313938, -14.99999999999999822 ) ) ;
#18099=CARTESIAN_POINT ( 'NONE',  ( -10.04305231718579172, 4.100000005462373309, -30.90933677959248982 ) ) ;
#18101=CARTESIAN_POINT ( 'NONE',  ( 6.486482029760649416E-15, 77.87500000273118417, 35.31076352940723240 ) ) ;
#18105=ORIENTED_EDGE ( 'NONE', *, *, #1363, .T. ) ;
#18107=CARTESIAN_POINT ( 'NONE',  ( -20.75514604977248112, 59.42500000273118843, 28.56700777964554661 ) ) ;
#18109=( BOUNDED_CURVE ( )  B_SPLINE_CURVE ( 2, ( #12263, #17949, #33190, #25313, #22913, #20523, #30792, #28398, #20699, #2137, #12956, #7466, #18114 ),
 .UNSPECIFIED., .F., .T. ) 
 B_SPLINE_CURVE_WITH_KNOTS ( ( 3, 2, 2, 2, 2, 2, 3 ),
 ( 0.6474358974358974672, 0.6487179487179487447, 0.6512820512820512997, 0.6538461538461538547, 0.6564102564102564097, 0.6589743589743589647, 0.6602564102564102422 ),
 .UNSPECIFIED. ) 
 CURVE ( )  GEOMETRIC_REPRESENTATION_ITEM ( )  RATIONAL_B_SPLINE_CURVE ( ( 0.9755282581475768211, 0.9755282581475768211, 1.000000000000000000, 0.9510565162951535312, 1.000000000000000000, 0.9510565162951535312, 1.000000000000000000, 0.9510565162951535312, 1.000000000000000000, 0.9510565162951535312, 1.000000000000000000, 0.9755282581475768211, 0.9755282581475768211 ) ) 
 REPRESENTATION_ITEM ( '' )  );
#18110=CARTESIAN_POINT ( 'NONE',  ( 15.14183272437242245, 16.30000000000001137, -20.84094480462497856 ) ) ;
#18112=CARTESIAN_POINT ( 'NONE',  ( -33.58253175000000113, 3.225000002731193138, 10.91162601494193929 ) ) ;
#18114=CARTESIAN_POINT ( 'NONE',  ( 5.779280353836490358E-15, 28.50000000000000355, 32.49999999999999289 ) ) ;
#18118=CARTESIAN_POINT ( 'NONE',  ( 32.50000000000000000, 9.000000000000007105, -3.980102097228898626E-15 ) ) ;
#18122=EDGE_CURVE ( 'NONE', #16826, #726, #21877, .T. ) ;
#18124=CARTESIAN_POINT ( 'NONE',  ( -9.657523855033125146E-16, 73.75000000546238255, -15.77193336357400710 ) ) ;
#18126=CARTESIAN_POINT ( 'NONE',  ( -20.75514604977248823, 28.82500000273116569, -28.56700777964554305 ) ) ;
#18131=CARTESIAN_POINT ( 'NONE',  ( 10.37757302488624056, 20.77500000273119340, -31.93888565452638417 ) ) ;
#18132=CARTESIAN_POINT ( 'NONE',  ( -20.08610463437157989, 63.69999999999999574, -27.64615127144129758 ) ) ;
#18134=CARTESIAN_POINT ( 'NONE',  ( 10.37757302488624767, 73.72500000273119269, 31.93888565452638417 ) ) ;
#18135=CYLINDRICAL_SURFACE ( 'NONE', #5797, 32.50000000000000000 ) ;
#18137=CARTESIAN_POINT ( 'NONE',  ( -7.236395654485757944, 17.22499999726881370, -22.27133577429736988 ) ) ;
#18138=CARTESIAN_POINT ( 'NONE',  ( 10.37757302488624767, 63.72500000273117848, 31.93888565452638417 ) ) ;
#18140=ADVANCED_FACE ( 'NONE', ( #5922 ), #19301, .F. ) ;
#18142=CARTESIAN_POINT ( 'NONE',  ( 27.16883889988623935, 8.325000002731176352, -19.73931689729374384 ) ) ;
#18143=CARTESIAN_POINT ( 'NONE',  ( 7.236395654485755280, 18.72499999726881370, 22.27133577429736988 ) ) ;
#18145=ORIENTED_EDGE ( 'NONE', *, *, #24987, .T. ) ;
#18152=CARTESIAN_POINT ( 'NONE',  ( 19.82091636218621034, 19.54999999453763238, 14.40073868116559730 ) ) ;
#18153=CARTESIAN_POINT ( 'NONE',  ( -18.94512977948576093, 17.82499999726880446, 13.76444248337722698 ) ) ;
#18154=CARTESIAN_POINT ( 'NONE',  ( -10.37757302488623701, 13.77500000273118630, 31.93888565452638417 ) ) ;
#18155=CARTESIAN_POINT ( 'NONE',  ( -32.50000000000000000, 16.60000000546238752, 10.55989012756946366 ) ) ;
#18156=CARTESIAN_POINT ( 'NONE',  ( 32.50000000000000711, 68.90000000000001990, 10.55989012756945122 ) ) ;
#18157=CARTESIAN_POINT ( 'NONE',  ( 15.00000000000000000, 77.25000000546239676, -1.836970198721029589E-15 ) ) ;
#18158=CARTESIAN_POINT ( 'NONE',  ( 1.555960095263670572E-15, 12.50000000000000355, -24.50000000000000000 ) ) ;
#18160=CARTESIAN_POINT ( 'NONE',  ( 8.601468415847516980, 80.67500000273116711, -11.83890561707634781 ) ) ;
#18163=CARTESIAN_POINT ( 'NONE',  ( 0.000000000000000000, 0.000000000000000000, 24.50000000000000000 ) ) ;
#18164=CARTESIAN_POINT ( 'NONE',  ( 7.236395654485755280, 16.72499999726881370, 22.27133577429736988 ) ) ;
#18165=CARTESIAN_POINT ( 'NONE',  ( 6.277390505771533514E-15, 8.499999999999992895, 34.17252228774368916 ) ) ;
#18166=CARTESIAN_POINT ( 'NONE',  ( -12.13525491562420910, 74.19999999999998863, 8.816778784387098611 ) ) ;
#18168=CARTESIAN_POINT ( 'NONE',  ( 33.58253175000000113, 50.12500000273117706, -4.112674001490185761E-15 ) ) ;
#18170=CARTESIAN_POINT ( 'NONE',  ( 27.16883889988624290, 38.17500000273118843, 19.73931689729373673 ) ) ;
#18171=DIRECTION ( 'NONE',  ( 0.000000000000000000, 0.000000000000000000, -1.000000000000000000 ) ) ;
#18178=CARTESIAN_POINT ( 'NONE',  ( -15.00000000000000000, 80.25000000546239676, 0.000000000000000000 ) ) ;
#18179=EDGE_CURVE ( 'NONE', #30438, #14163, #16730, .T. ) ;
#18180=CARTESIAN_POINT ( 'NONE',  ( 4.023268246324634798E-14, 10.24999999453763166, -24.50000000000000355 ) ) ;
#18183=CARTESIAN_POINT ( 'NONE',  ( 24.50000000000000000, 17.74999999453763522, 0.000000000000000000 ) ) ;
#18184=CARTESIAN_POINT ( 'NONE',  ( 20.75514604977248467, 28.42500000273118133, -28.56700777964554305 ) ) ;
#18188=ORIENTED_EDGE ( 'NONE', *, *, #33695, .F. ) ;
#18195=EDGE_CURVE ( 'NONE', #21689, #7536, #5471, .T. ) ;
#18196=CARTESIAN_POINT ( 'NONE',  ( -1.778240108872766143E-15, 45.49999999999999289, -32.49999999999999289 ) ) ;
#18197=CARTESIAN_POINT ( 'NONE',  ( 6.486482029760649416E-15, 37.87500000273117706, 35.31076352940723240 ) ) ;
#18198=CARTESIAN_POINT ( 'NONE',  ( 20.08610463437157279, 37.80000000546239391, -27.64615127144129758 ) ) ;
#18200=CARTESIAN_POINT ( 'NONE',  ( -32.50000000000000000, 47.99999999999998579, 0.000000000000000000 ) ) ;
#18201=CARTESIAN_POINT ( 'NONE',  ( 20.75514604977249178, 21.82500000273119056, 28.56700777964553950 ) ) ;
#18203=CARTESIAN_POINT ( 'NONE',  ( 27.16883889988624290, 52.17500000273117422, 19.73931689729373673 ) ) ;
#18206=CARTESIAN_POINT ( 'NONE',  ( 10.04305231718579705, 30.60000000000001563, 30.90933677959248982 ) ) ;
#18208=CARTESIAN_POINT ( 'NONE',  ( -10.37757302488624411, 70.72500000273119269, -31.93888565452638417 ) ) ;
#18211=CARTESIAN_POINT ( 'NONE',  ( -26.29305231718578995, 38.20000000000000995, 19.10302069950538595 ) ) ;
#18212=CARTESIAN_POINT ( 'NONE',  ( 33.58253175000000113, 62.37500000273119127, -4.112674001490185761E-15 ) ) ;
#18213=CARTESIAN_POINT ( 'NONE',  ( 0.000000000000000000, 80.00000000000001421, 0.000000000000000000 ) ) ;
#18214=CARTESIAN_POINT ( 'NONE',  ( 33.58253175000000113, 10.22500000273117671, -10.91162601494193751 ) ) ;
#18216=( BOUNDED_CURVE ( )  B_SPLINE_CURVE ( 2, ( #9270, #30547, #12542, #33468, #33296, #28325, #9968, #22836, #14608, #27986, #30372, #4473, #15123 ),
 .UNSPECIFIED., .F., .T. ) 
 B_SPLINE_CURVE_WITH_KNOTS ( ( 3, 2, 2, 2, 2, 2, 3 ),
 ( 0.6858974358974359031, 0.6871794871794871806, 0.6897435897435897356, 0.6923076923076922906, 0.6948717948717948456, 0.6974358974358974006, 0.6987179487179486781 ),
 .UNSPECIFIED. ) 
 CURVE ( )  GEOMETRIC_REPRESENTATION_ITEM ( )  RATIONAL_B_SPLINE_CURVE ( ( 0.9755282581475768211, 0.9755282581475768211, 1.000000000000000000, 0.9510565162951535312, 1.000000000000000000, 0.9510565162951535312, 1.000000000000000000, 0.9510565162951535312, 1.000000000000000000, 0.9510565162951535312, 1.000000000000000000, 0.9755282581475768211, 0.9755282581475768211 ) ) 
 REPRESENTATION_ITEM ( '' )  );
#18217=CARTESIAN_POINT ( 'NONE',  ( 24.50000000000000000, 1.749999994537621006, 0.000000000000000000 ) ) ;
#18218=CARTESIAN_POINT ( 'NONE',  ( 20.75514604977249178, 2.075000002731171467, 28.56700777964553950 ) ) ;
#18220=CARTESIAN_POINT ( 'NONE',  ( 32.50000000000000000, 45.60000000546236265, -10.55989012756945833 ) ) ;
#18221=CARTESIAN_POINT ( 'NONE',  ( 5.147494310547426899, 19.44874571845315003, -32.50000000000000000 ) ) ;
#18227=CARTESIAN_POINT ( 'NONE',  ( -20.08610463437156923, 54.30000000000000426, 27.64615127144130113 ) ) ;
#18228=CARTESIAN_POINT ( 'NONE',  ( 26.29305231718579350, 71.30000000546237970, 19.10302069950537529 ) ) ;
#18237=CARTESIAN_POINT ( 'NONE',  ( -10.37757302488624411, 50.97500000273119980, -31.93888565452638417 ) ) ;
#18238=CARTESIAN_POINT ( 'NONE',  ( -26.29305231718579350, 58.30000000546237260, -19.10302069950537884 ) ) ;
#18240=CARTESIAN_POINT ( 'NONE',  ( 33.58253175000000113, 42.22500000273118559, -10.91162601494193751 ) ) ;
#18241=CARTESIAN_POINT ( 'NONE',  ( 2.445080149700053643E-15, 72.50000000000001421, 15.00000000000000000 ) ) ;
#18242=CARTESIAN_POINT ( 'NONE',  ( -33.58253175000000113, 65.37500000273119838, 0.000000000000000000 ) ) ;
#18243=CARTESIAN_POINT ( 'NONE',  ( -1.778240108872766143E-15, 22.00000000546237899, -32.49999999999999289 ) ) ;
#18246=CARTESIAN_POINT ( 'NONE',  ( -10.04305231718578462, 46.39999999999999858, 30.90933677959249337 ) ) ;
#18248=CARTESIAN_POINT ( 'NONE',  ( 33.58253175000000113, 10.47500000273119802, -10.91162601494193751 ) ) ;
#18249=CARTESIAN_POINT ( 'NONE',  ( 0.000000000000000000, 80.00000000000001421, 0.000000000000000000 ) ) ;
#18251=CARTESIAN_POINT ( 'NONE',  ( -4.300734207923759378, 80.97500000273119269, -13.23629886949340495 ) ) ;
#18252=CARTESIAN_POINT ( 'NONE',  ( -2.162160676586882350E-15, 78.87500000273118417, -35.31076352940722529 ) ) ;
#18253=DIRECTION ( 'NONE',  ( -0.000000000000000000, -1.000000000000000000, -0.000000000000000000 ) ) ;
#18254=VECTOR ( 'NONE', #26959, 1000.000000000000000 ) ;
#18267=CARTESIAN_POINT ( 'NONE',  ( -20.75514604977248112, 43.42500000273117422, 28.56700777964554661 ) ) ;
#18269=CARTESIAN_POINT ( 'NONE',  ( -32.50000000000000000, 2.400000005462369579, -10.55989012756945300 ) ) ;
#18273=CARTESIAN_POINT ( 'NONE',  ( 2.445080149700053643E-15, 70.75000000546236834, 15.00000000000000000 ) ) ;
#18274=AXIS2_PLACEMENT_3D ( 'NONE', #14072, #10262, #33771 ) ;
#18276=CARTESIAN_POINT ( 'NONE',  ( -27.16883889988623935, 75.57500000273120122, 19.73931689729374739 ) ) ;
#18280=VECTOR ( 'NONE', #21491, 1000.000000000000114 ) ;
#18282=ORIENTED_EDGE ( 'NONE', *, *, #21442, .T. ) ;
#18284=CARTESIAN_POINT ( 'NONE',  ( 33.58253175000000113, 60.22500000273119980, -10.91162601494193751 ) ) ;
#18287=CARTESIAN_POINT ( 'NONE',  ( -7.236395654485763274, 2.524999997268823293, 22.27133577429736633 ) ) ;
#18288=CARTESIAN_POINT ( 'NONE',  ( -2.162160676586881955E-15, 6.625000002731173510, -35.31076352940723240 ) ) ;
#18289=CARTESIAN_POINT ( 'NONE',  ( -9.270509831248419985, 78.55000000546236549, 12.75976212528060039 ) ) ;
#18291=CARTESIAN_POINT ( 'NONE',  ( 1.836970198721029589E-15, 70.00000000000000000, 15.00000000000000000 ) ) ;
#18297=CARTESIAN_POINT ( 'NONE',  ( 11.25946833292375793, 79.67500000273119554, 8.180482586598731842 ) ) ;
#18299=CARTESIAN_POINT ( 'NONE',  ( -33.58253175000000113, 33.12500000273119127, 0.000000000000000000 ) ) ;
#18302=CARTESIAN_POINT ( 'NONE',  ( -2.162160676586882350E-15, 16.87500000273119483, -35.31076352940722529 ) ) ;
#18306=CARTESIAN_POINT ( 'NONE',  ( -27.16883889988623935, 73.32500000273117280, 19.73931689729374739 ) ) ;
#18307=CARTESIAN_POINT ( 'NONE',  ( -32.50000000000000000, 26.60000000546239107, 10.55989012756946366 ) ) ;
#18310=CARTESIAN_POINT ( 'NONE',  ( -27.16883889988624290, 64.92500000273118133, -19.73931689729374028 ) ) ;
#18314=CARTESIAN_POINT ( 'NONE',  ( -10.37757302488623701, 9.525000002731182747, 31.93888565452638417 ) ) ;
#18315=CARTESIAN_POINT ( 'NONE',  ( -14.47279130897151589, 1.324999997268808238, -19.92008829642072598 ) ) ;
#18317=ORIENTED_EDGE ( 'NONE', *, *, #17404, .F. ) ;
#18323=CARTESIAN_POINT ( 'NONE',  ( -10.37757302488623701, 77.52500000273118985, 31.93888565452638417 ) ) ;
#18325=AXIS2_PLACEMENT_3D ( 'NONE', #16183, #31444, #31273 ) ;
#18326=CARTESIAN_POINT ( 'NONE',  ( -15.14183272437242600, 1.299999999999988054, 20.84094480462497856 ) ) ;
#18327=CARTESIAN_POINT ( 'NONE',  ( 6.486482029760649416E-15, 15.87500000273120015, 35.31076352940723240 ) ) ;
#18328=CARTESIAN_POINT ( 'NONE',  ( -32.50000000000000000, 60.09999999999999432, 10.55989012756946366 ) ) ;
#18329=CARTESIAN_POINT ( 'NONE',  ( -1.778240108872766143E-15, 58.00000000546237544, -32.49999999999999289 ) ) ;
#18332=CARTESIAN_POINT ( 'NONE',  ( 8.601468415847520532, 78.07500000273117280, 11.83890561707634781 ) ) ;
#18335=CARTESIAN_POINT ( 'NONE',  ( 3.880418787951178228, 16.44874571845315359, -24.49999999999998224 ) ) ;
#18336=CARTESIAN_POINT ( 'NONE',  ( -2.092463501923844636E-15, 9.499999999999991118, -34.17252228774368916 ) ) ;
#18337=CARTESIAN_POINT ( 'NONE',  ( 26.29305231718578995, 17.70000000546237473, -19.10302069950538240 ) ) ;
#18339=CARTESIAN_POINT ( 'NONE',  ( -20.75514604977248823, 48.82500000273117280, -28.56700777964554305 ) ) ;
#18341=CARTESIAN_POINT ( 'NONE',  ( 20.75514604977248467, 38.67500000273116711, -28.56700777964554305 ) ) ;
#18342=CARTESIAN_POINT ( 'NONE',  ( -1.778240108872766143E-15, 24.00000000546237899, -32.49999999999999289 ) ) ;
#18344=DIRECTION ( 'NONE',  ( -0.8660254037844399289, -0.4999999999999977240, 0.000000000000000000 ) ) ;
#18346=CARTESIAN_POINT ( 'NONE',  ( -26.29305231718578995, 22.70000000546237828, 19.10302069950538595 ) ) ;
#18352=CARTESIAN_POINT ( 'NONE',  ( -32.50000000000000000, 40.00000000000000711, 0.000000000000000000 ) ) ;
#18355=CARTESIAN_POINT ( 'NONE',  ( 3.880418787951172011, 17.30125427608447097, 24.49999999999998579 ) ) ;
#18356=CARTESIAN_POINT ( 'NONE',  ( -33.58253175000000113, 25.22500000273119625, 10.91162601494193929 ) ) ;
#18361=VERTEX_POINT ( 'NONE', #22841 ) ;
#18365=CYLINDRICAL_SURFACE ( 'NONE', #19042, 32.50000000000000000 ) ;
#18366=CARTESIAN_POINT ( 'NONE',  ( -10.37757302488623701, 37.77500000273118275, 31.93888565452638417 ) ) ;
#18368=CARTESIAN_POINT ( 'NONE',  ( -32.50000000000000000, 40.40000000546239534, -10.55989012756945478 ) ) ;
#18369=CARTESIAN_POINT ( 'NONE',  ( -10.04305231718579172, 75.59999999999999432, -30.90933677959248982 ) ) ;
#18371=CARTESIAN_POINT ( 'NONE',  ( 10.37757302488624767, 21.72500000273119980, 31.93888565452638417 ) ) ;
#18372=CARTESIAN_POINT ( 'NONE',  ( 8.891200544363830713E-16, 81.50000000000001421, -15.00000000000000000 ) ) ;
#18373=CARTESIAN_POINT ( 'NONE',  ( -10.37757302488623701, 49.77500000273118985, 31.93888565452638417 ) ) ;
#18375=CARTESIAN_POINT ( 'NONE',  ( 26.29305231718579350, 26.79999999999999005, 19.10302069950537529 ) ) ;
#18377=CARTESIAN_POINT ( 'NONE',  ( -27.16883889988624290, 70.92500000273119554, -19.73931689729374028 ) ) ;
#18379=CARTESIAN_POINT ( 'NONE',  ( -2.162160676586882350E-15, 62.87500000273120548, -35.31076352940722529 ) ) ;
#18380=CARTESIAN_POINT ( 'NONE',  ( 5.334720326618300005E-14, 73.50000000000001421, -32.50000000000000000 ) ) ;
#18381=CARTESIAN_POINT ( 'NONE',  ( 27.16883889988624290, 9.925000002731193760, 19.73931689729373673 ) ) ;
#18384=CARTESIAN_POINT ( 'NONE',  ( 20.75514604977248467, 2.675000002731181770, -28.56700777964554305 ) ) ;
#18394=CARTESIAN_POINT ( 'NONE',  ( 10.04305231718579705, 63.10000000546239818, 30.90933677959248982 ) ) ;
#18395=CARTESIAN_POINT ( 'NONE',  ( -32.50000000000000000, 70.40000000546237402, -10.55989012756945478 ) ) ;
#18399=VERTEX_POINT ( 'NONE', #4648 ) ;
#18404=CARTESIAN_POINT ( 'NONE',  ( 5.779280353836490358E-15, 36.49999999999998579, 32.49999999999999289 ) ) ;
#18405=CARTESIAN_POINT ( 'NONE',  ( 20.75514604977248467, 56.67500000273119554, -28.56700777964554305 ) ) ;
#18406=CARTESIAN_POINT ( 'NONE',  ( -10.04305231718579172, 58.10000000546239107, -30.90933677959248982 ) ) ;
#18407=CARTESIAN_POINT ( 'NONE',  ( 0.000000000000000000, 0.000000000000000000, 0.000000000000000000 ) ) ;
#18408=CARTESIAN_POINT ( 'NONE',  ( -2.162160676586881955E-15, 40.62500000273120548, -35.31076352940723240 ) ) ;
#18410=CARTESIAN_POINT ( 'NONE',  ( 20.75514604977249178, 68.07500000273118701, 28.56700777964553950 ) ) ;
#18413=EDGE_CURVE ( 'NONE', #29502, #14163, #677, .T. ) ;
#18416=CARTESIAN_POINT ( 'NONE',  ( -26.29305231718579350, 43.80000000000000426, -19.10302069950537884 ) ) ;
#18418=( BOUNDED_CURVE ( )  B_SPLINE_CURVE ( 2, ( #19837, #7817, #20360, #7649, #31157, #18307, #30806, #5075, #28751, #13312, #2327, #2506, #28245 ),
 .UNSPECIFIED., .F., .T. ) 
 B_SPLINE_CURVE_WITH_KNOTS ( ( 3, 2, 2, 2, 2, 2, 3 ),
 ( 0.6602564102564102422, 0.6615384615384615197, 0.6641025641025640747, 0.6666666666666666297, 0.6692307692307691847, 0.6717948717948717396, 0.6730769230769231282 ),
 .UNSPECIFIED. ) 
 CURVE ( )  GEOMETRIC_REPRESENTATION_ITEM ( )  RATIONAL_B_SPLINE_CURVE ( ( 0.9755282581475768211, 0.9755282581475768211, 1.000000000000000000, 0.9510565162951535312, 1.000000000000000000, 0.9510565162951535312, 1.000000000000000000, 0.9510565162951535312, 1.000000000000000000, 0.9510565162951535312, 1.000000000000000000, 0.9755282581475757109, 0.9755282581475768211 ) ) 
 REPRESENTATION_ITEM ( '' )  );
#18419=CARTESIAN_POINT ( 'NONE',  ( 10.37757302488624056, 8.775000002731180970, -31.93888565452638417 ) ) ;
#18420=CARTESIAN_POINT ( 'NONE',  ( 3.000384657911015469E-15, 0.000000000000000000, -24.50000000000000000 ) ) ;
#18422=FACE_OUTER_BOUND ( 'NONE', #23417, .T. ) ;
#18424=DIRECTION ( 'NONE',  ( 0.000000000000000000, 0.000000000000000000, -1.000000000000000000 ) ) ;
#18427=CARTESIAN_POINT ( 'NONE',  ( 3.980102097228898626E-15, 80.00000000000001421, 32.50000000000000000 ) ) ;
#18438=CARTESIAN_POINT ( 'NONE',  ( -10.37757302488623701, 37.52500000273117564, 31.93888565452638417 ) ) ;
#18441=CARTESIAN_POINT ( 'NONE',  ( 5.779280353836490358E-15, 3.000000005462374109, 32.49999999999999289 ) ) ;
#18442=ORIENTED_EDGE ( 'NONE', *, *, #6511, .F. ) ;
#18444=CARTESIAN_POINT ( 'NONE',  ( -32.50000000000000000, 50.50000000546239676, 0.000000000000000000 ) ) ;
#18446=CARTESIAN_POINT ( 'NONE',  ( -20.75514604977248823, 75.07500000273118701, -28.56700777964554305 ) ) ;
#18452=CARTESIAN_POINT ( 'NONE',  ( 33.58253175000000823, 64.02500000273118985, 10.91162601494192863 ) ) ;
#18455=CARTESIAN_POINT ( 'NONE',  ( -14.47279130897152299, 8.424999997268816543, 19.92008829642072243 ) ) ;
#18456=CARTESIAN_POINT ( 'NONE',  ( -2.162160676586881955E-15, 2.625000002731183724, -35.31076352940723240 ) ) ;
#18457=CARTESIAN_POINT ( 'NONE',  ( -1.778240108872766143E-15, 6.000000005462371888, -32.49999999999999289 ) ) ;
#18464=CARTESIAN_POINT ( 'NONE',  ( 4.635254915624209993, 73.65000000546240244, -14.26584774442730463 ) ) ;
#18467=CARTESIAN_POINT ( 'NONE',  ( 27.16883889988623935, 22.32500000273118701, -19.73931689729374384 ) ) ;
#18469=VECTOR ( 'NONE', #33382, 1000.000000000000000 ) ;
#18471=CARTESIAN_POINT ( 'NONE',  ( 33.58253175000000113, 14.47500000273118737, -10.91162601494193574 ) ) ;
#18473=CARTESIAN_POINT ( 'NONE',  ( -33.58253175000000113, 79.02500000273118985, -10.91162601494193041 ) ) ;
#18474=CARTESIAN_POINT ( 'NONE',  ( 15.14183272437242422, 8.300000000000000711, -20.84094480462497856 ) ) ;
#18476=CARTESIAN_POINT ( 'NONE',  ( 23.41746824999999887, 18.52499999726881796, 7.608796670333735079 ) ) ;
#18477=CARTESIAN_POINT ( 'NONE',  ( 6.486482029760648627E-15, 59.62500000273118417, 35.31076352940722529 ) ) ;
#18480=ORIENTED_EDGE ( 'NONE', *, *, #741, .F. ) ;
#18482=CARTESIAN_POINT ( 'NONE',  ( -27.16883889988624290, 8.925000002731191984, -19.73931689729374028 ) ) ;
#18483=CARTESIAN_POINT ( 'NONE',  ( 23.41746824999999887, 0.6249999972688102812, 0.000000000000000000 ) ) ;
#18491=CARTESIAN_POINT ( 'NONE',  ( 10.04305231718578817, 11.90000000546237402, -30.90933677959249337 ) ) ;
#18493=CARTESIAN_POINT ( 'NONE',  ( -5.147494310547430452, 71.55125428154684641, -32.49999999999999289 ) ) ;
#18495=CARTESIAN_POINT ( 'NONE',  ( 18.94512977948575738, 16.42499999726882010, 13.76444248337723408 ) ) ;
#18496=CARTESIAN_POINT ( 'NONE',  ( 27.16883889988624290, 6.175000002731190207, 19.73931689729373673 ) ) ;
#18497=CARTESIAN_POINT ( 'NONE',  ( 6.277390505771533514E-15, 58.49999999999997868, 34.17252228774368916 ) ) ;
#18498=CARTESIAN_POINT ( 'NONE',  ( 8.601468415847520532, 77.57500000273120122, 11.83890561707634603 ) ) ;
#18499=CARTESIAN_POINT ( 'NONE',  ( 5.147494310547434893, 73.05125428700921475, 32.49999999999999289 ) ) ;
#18501=CARTESIAN_POINT ( 'NONE',  ( -13.91746824999999532, 77.47500000273120691, 4.522059556121122093 ) ) ;
#18504=CARTESIAN_POINT ( 'NONE',  ( -24.50000000000000711, 1.099999999999994316, 7.960532557706201828 ) ) ;
#18505=CARTESIAN_POINT ( 'NONE',  ( 26.29305231718579350, 4.799999999999998934, 19.10302069950537529 ) ) ;
#18506=CARTESIAN_POINT ( 'NONE',  ( 10.04305231718579705, 17.10000000546238397, 30.90933677959248982 ) ) ;
#18509=CARTESIAN_POINT ( 'NONE',  ( -27.16883889988623935, 53.32500000273118701, 19.73931689729374739 ) ) ;
#18512=CARTESIAN_POINT ( 'NONE',  ( 6.486482029760648627E-15, 31.87500000273119127, 35.31076352940722529 ) ) ;
#18513=DIRECTION ( 'NONE',  ( 0.000000000000000000, -0.000000000000000000, 1.000000000000000000 ) ) ;
#18515=CARTESIAN_POINT ( 'NONE',  ( -15.14183272437242778, 9.299999999999995381, 20.84094480462497856 ) ) ;
#18516=CARTESIAN_POINT ( 'NONE',  ( -32.50000000000000000, 22.50000000546237189, 0.000000000000000000 ) ) ;
#18519=CARTESIAN_POINT ( 'NONE',  ( 18.94512977948576093, 0.8249999972688160099, -13.76444248337722875 ) ) ;
#18520=CARTESIAN_POINT ( 'NONE',  ( -1.778240108872766143E-15, 39.50000000000000000, -32.49999999999999289 ) ) ;
#18523=CARTESIAN_POINT ( 'NONE',  ( 19.82091636218621389, 17.94999999453761319, -14.40073868116559197 ) ) ;
#18524=CARTESIAN_POINT ( 'NONE',  ( -33.58253175000000113, 23.02500000273117919, -10.91162601494193041 ) ) ;
#18526=EDGE_LOOP ( 'NONE', ( #24175, #28350, #5552, #9325 ) ) ;
#18534=CARTESIAN_POINT ( 'NONE',  ( 20.75514604977249178, 32.07500000273117990, 28.56700777964553950 ) ) ;
#18535=AXIS2_PLACEMENT_3D ( 'NONE', #28438, #30488, #25865 ) ;
#18536=CARTESIAN_POINT ( 'NONE',  ( 10.04305231718579705, 37.10000000546237686, 30.90933677959248982 ) ) ;
#18538=LINE ( 'NONE', #15961, #31852 ) ;
#18540=CARTESIAN_POINT ( 'NONE',  ( -20.75514604977248823, 47.07500000273117990, -28.56700777964554305 ) ) ;
#18542=CARTESIAN_POINT ( 'NONE',  ( -26.29305231718578995, 20.19999999999999574, 19.10302069950538595 ) ) ;
#18544=CARTESIAN_POINT ( 'NONE',  ( -20.75514604977248823, 66.82500000273118701, -28.56700777964554305 ) ) ;
#18547=CARTESIAN_POINT ( 'NONE',  ( -20.75514604977248112, 53.67500000273119554, 28.56700777964554661 ) ) ;
#18548=CARTESIAN_POINT ( 'NONE',  ( 5.147494310547453544, 73.44874571845316780, -32.49999999999999289 ) ) ;
#18549=CARTESIAN_POINT ( 'NONE',  ( -33.58253175000000113, 13.12500000273120193, 0.000000000000000000 ) ) ;
#18551=CYLINDRICAL_SURFACE ( 'NONE', #25014, 24.50000000000000000 ) ;
#18552=CARTESIAN_POINT ( 'NONE',  ( 0.000000000000000000, 80.00000000000001421, 0.000000000000000000 ) ) ;
#18555=CARTESIAN_POINT ( 'NONE',  ( 26.29305231718578995, 45.70000000546237118, -19.10302069950538240 ) ) ;
#18556=CARTESIAN_POINT ( 'NONE',  ( 32.50000000000000000, 18.99999999999998934, -3.980102097228898626E-15 ) ) ;
#18560=AXIS2_PLACEMENT_3D ( 'NONE', #9413, #19397, #9083 ) ;
#18562=CARTESIAN_POINT ( 'NONE',  ( 32.50000000000000711, 60.89999999999999147, 10.55989012756945122 ) ) ;
#18564=CARTESIAN_POINT ( 'NONE',  ( 7.236395654485760609, 5.524999997268825958, -22.27133577429736633 ) ) ;
#18565=CARTESIAN_POINT ( 'NONE',  ( -20.08610463437157989, 72.20000000546237118, -27.64615127144129758 ) ) ;
#18567=VECTOR ( 'NONE', #1288, 1000.000000000000000 ) ;
#18568=EDGE_CURVE ( 'NONE', #19359, #29552, #19106, .T. ) ;
#18575=CARTESIAN_POINT ( 'NONE',  ( 32.50000000000000000, 75.09999999999996589, -10.55989012756945833 ) ) ;
#18576=CARTESIAN_POINT ( 'NONE',  ( 33.58253175000000113, 52.47500000273117138, -10.91162601494193751 ) ) ;
#18577=CARTESIAN_POINT ( 'NONE',  ( 10.04305231718579705, 55.10000000546239107, 30.90933677959248982 ) ) ;
#18579=CARTESIAN_POINT ( 'NONE',  ( 20.75514604977248467, 44.42500000273120264, -28.56700777964554305 ) ) ;
#18580=CARTESIAN_POINT ( 'NONE',  ( -1.778240108872766143E-15, 55.49999999999999289, -32.49999999999999289 ) ) ;
#18581=CARTESIAN_POINT ( 'NONE',  ( -20.75514604977248823, 71.07500000273117280, -28.56700777964554305 ) ) ;
#18585=CARTESIAN_POINT ( 'NONE',  ( 26.29305231718578995, 37.20000000000000995, -19.10302069950538240 ) ) ;
#18587=CARTESIAN_POINT ( 'NONE',  ( 33.58253175000000823, 12.27500000273116854, 10.91162601494192863 ) ) ;
#18588=CARTESIAN_POINT ( 'NONE',  ( 15.14183272437242067, 19.44999999453763806, 20.84094480462498211 ) ) ;
#18590=DIRECTION ( 'NONE',  ( -0.000000000000000000, -1.000000000000000000, -0.000000000000000000 ) ) ;
#18591=CARTESIAN_POINT ( 'NONE',  ( -10.37757302488623701, 75.77500000273118985, 31.93888565452638417 ) ) ;
#18594=ORIENTED_EDGE ( 'NONE', *, *, #24875, .F. ) ;
#18595=CARTESIAN_POINT ( 'NONE',  ( 0.000000000000000000, 82.00000000000001421, 0.000000000000000000 ) ) ;
#18602=EDGE_CURVE ( 'NONE', #13970, #33138, #29602, .T. ) ;
#18606=CARTESIAN_POINT ( 'NONE',  ( 10.37757302488624056, 40.52500000273118275, -31.93888565452638417 ) ) ;
#18611=VERTEX_POINT ( 'NONE', #11649 ) ;
#18615=CARTESIAN_POINT ( 'NONE',  ( -20.75514604977248112, 69.67500000273119554, 28.56700777964554661 ) ) ;
#18618=EDGE_CURVE ( 'NONE', #12120, #11025, #16695, .T. ) ;
#18621=( BOUNDED_CURVE ( )  B_SPLINE_CURVE ( 2, ( #511, #2423, #10996, #7736, #13717, #20800, #31244, #18562, #8076, #21136, #26442, #31577, #23701 ),
 .UNSPECIFIED., .F., .T. ) 
 B_SPLINE_CURVE_WITH_KNOTS ( ( 3, 2, 2, 2, 2, 2, 3 ),
 ( 0.2371794871794871973, 0.2384615384615384748, 0.2410256410256410298, 0.2435897435897435848, 0.2461538461538461675, 0.2487179487179487225, 0.2500000000000000000 ),
 .UNSPECIFIED. ) 
 CURVE ( )  GEOMETRIC_REPRESENTATION_ITEM ( )  RATIONAL_B_SPLINE_CURVE ( ( 0.9755282581475768211, 0.9755282581475770431, 1.000000000000000000, 0.9510565162951535312, 1.000000000000000000, 0.9510565162951535312, 1.000000000000000000, 0.9510565162951535312, 1.000000000000000000, 0.9510565162951535312, 1.000000000000000000, 0.9755282581475768211, 0.9755282581475768211 ) ) 
 REPRESENTATION_ITEM ( '' )  );
#18623=CARTESIAN_POINT ( 'NONE',  ( 10.37757302488624767, 61.72500000273117848, 31.93888565452638417 ) ) ;
#18625=CARTESIAN_POINT ( 'NONE',  ( -24.50000000000001066, 17.10000000000001208, 7.960532557706201828 ) ) ;
#18626=CARTESIAN_POINT ( 'NONE',  ( -14.47279130897152299, 10.42499999726881121, 19.92008829642072243 ) ) ;
#18627=CARTESIAN_POINT ( 'NONE',  ( 33.58253175000000113, 4.125000002731193938, -4.112674001490185761E-15 ) ) ;
#18628=CARTESIAN_POINT ( 'NONE',  ( 27.16883889988624290, 28.17500000273118133, 19.73931689729373673 ) ) ;
#18631=CARTESIAN_POINT ( 'NONE',  ( -20.75514604977248823, 79.07500000273121543, -28.56700777964554305 ) ) ;
#18632=CARTESIAN_POINT ( 'NONE',  ( -13.91746824999999532, 80.77500000273118985, -4.522059556121115875 ) ) ;
#18633=CARTESIAN_POINT ( 'NONE',  ( 20.08610463437157279, 75.80000000546237970, -27.64615127144129758 ) ) ;
#18637=CARTESIAN_POINT ( 'NONE',  ( -13.91746824999999532, 78.77500000273116143, -4.522059556121115875 ) ) ;
#18639=CARTESIAN_POINT ( 'NONE',  ( -27.16883889988624290, 24.92500000273117777, -19.73931689729374028 ) ) ;
#18642=CARTESIAN_POINT ( 'NONE',  ( 10.37757302488624056, 16.77500000273118985, -31.93888565452638417 ) ) ;
#18644=CARTESIAN_POINT ( 'NONE',  ( -20.75514604977248823, 72.82500000273117280, -28.56700777964554305 ) ) ;
#18645=CARTESIAN_POINT ( 'NONE',  ( 5.779280353836490358E-15, 59.00000000546238255, 32.49999999999999289 ) ) ;
#18647=CARTESIAN_POINT ( 'NONE',  ( 4.635254915624209993, 79.65000000546237402, -14.26584774442730463 ) ) ;
#18648=CARTESIAN_POINT ( 'NONE',  ( 27.16883889988623935, 58.32500000273119412, -19.73931689729374384 ) ) ;
#18650=ORIENTED_EDGE ( 'NONE', *, *, #13886, .F. ) ;
#18652=CARTESIAN_POINT ( 'NONE',  ( 33.58253175000000113, 2.225000002731166937, -10.91162601494193574 ) ) ;
#18653=CARTESIAN_POINT ( 'NONE',  ( 18.94512977948575738, 2.424999997268806329, 13.76444248337723408 ) ) ;
#18655=ORIENTED_EDGE ( 'NONE', *, *, #31502, .F. ) ;
#18658=ORIENTED_EDGE ( 'NONE', *, *, #18122, .T. ) ;
#18662=CARTESIAN_POINT ( 'NONE',  ( -10.04305231718579172, 71.59999999999999432, -30.90933677959248982 ) ) ;
#18664=CARTESIAN_POINT ( 'NONE',  ( -7.570916362186210335, 2.599999999999991207, -23.30088464923126779 ) ) ;
#18665=CARTESIAN_POINT ( 'NONE',  ( -27.16883889988624290, 11.17500000273119554, -19.73931689729374028 ) ) ;
#18666=CARTESIAN_POINT ( 'NONE',  ( 10.04305231718578817, 61.40000000000001279, -30.90933677959249337 ) ) ;
#18667=CARTESIAN_POINT ( 'NONE',  ( -8.601468415847515203, 79.17500000273120975, 11.83890561707634959 ) ) ;
#18670=CARTESIAN_POINT ( 'NONE',  ( 13.91746825000000065, 78.27500000273116143, 4.522059556121114987 ) ) ;
#18674=CARTESIAN_POINT ( 'NONE',  ( -19.82091636218621389, 1.200000000000006617, 14.40073868116558842 ) ) ;
#18675=CARTESIAN_POINT ( 'NONE',  ( -26.29305231718578995, 4.199999999999981526, 19.10302069950538595 ) ) ;
#18678=CARTESIAN_POINT ( 'NONE',  ( -20.75514604977248823, 46.82500000273117990, -28.56700777964554305 ) ) ;
#18682=CARTESIAN_POINT ( 'NONE',  ( -20.75514604977248112, 37.67500000273118133, 28.56700777964554661 ) ) ;
#18683=CYLINDRICAL_SURFACE ( 'NONE', #33600, 24.50000000000000000 ) ;
#18686=CARTESIAN_POINT ( 'NONE',  ( -2.375766604868041476, 76.44874571845315359, 14.99999999999999822 ) ) ;
#18689=CARTESIAN_POINT ( 'NONE',  ( -23.41746825000000243, 7.724999997268811036, 7.608796670333725309 ) ) ;
#18690=CARTESIAN_POINT ( 'NONE',  ( -10.04305231718579172, 39.59999999999999432, -30.90933677959248982 ) ) ;
#18692=CARTESIAN_POINT ( 'NONE',  ( -10.04305231718579172, 11.59999999999999964, -30.90933677959248982 ) ) ;
#18693=CARTESIAN_POINT ( 'NONE',  ( -33.58253175000000113, 19.02500000273118630, -10.91162601494193041 ) ) ;
#18702=ADVANCED_FACE ( 'NONE', ( #16816 ), #1169, .F. ) ;
#18704=DIRECTION ( 'NONE',  ( 0.000000000000000000, 0.000000000000000000, 1.000000000000000000 ) ) ;
#18705=CARTESIAN_POINT ( 'NONE',  ( -10.37757302488624411, 28.97500000273117848, -31.93888565452638417 ) ) ;
#18706=CARTESIAN_POINT ( 'NONE',  ( -26.29305231718579350, 40.30000000546237970, -19.10302069950537884 ) ) ;
#18707=CARTESIAN_POINT ( 'NONE',  ( 32.50000000000000000, 79.10000000000000853, -10.55989012756945833 ) ) ;
#18708=CARTESIAN_POINT ( 'NONE',  ( -1.778240108872766143E-15, 34.00000000546236834, -32.49999999999999289 ) ) ;
#18710=CARTESIAN_POINT ( 'NONE',  ( -27.16883889988624290, 43.17500000273119554, -19.73931689729374028 ) ) ;
#18713=CARTESIAN_POINT ( 'NONE',  ( 10.04305231718578817, 23.40000000000000568, -30.90933677959249337 ) ) ;
#18715=CARTESIAN_POINT ( 'NONE',  ( 33.58253175000000823, 64.02500000273118985, 10.91162601494192863 ) ) ;
#18717=CARTESIAN_POINT ( 'NONE',  ( -1.778240108872766143E-15, 37.50000000000000000, -32.49999999999999289 ) ) ;
#18718=CARTESIAN_POINT ( 'NONE',  ( 20.75514604977248467, 52.67500000273116711, -28.56700777964554305 ) ) ;
#18721=CARTESIAN_POINT ( 'NONE',  ( 27.16883889988623935, 14.32500000273117990, -19.73931689729374384 ) ) ;
#18726=AXIS2_PLACEMENT_3D ( 'NONE', #14377, #24836, #1314 ) ;
#18727=CYLINDRICAL_SURFACE ( 'NONE', #31967, 32.50000000000000000 ) ;
#18733=CARTESIAN_POINT ( 'NONE',  ( -26.29305231718579350, 72.30000000546237970, -19.10302069950537884 ) ) ;
#18737=ORIENTED_EDGE ( 'NONE', *, *, #337, .F. ) ;
#18741=CARTESIAN_POINT ( 'NONE',  ( 33.58253175000000823, 48.27500000273119696, 10.91162601494192863 ) ) ;
#18742=EDGE_CURVE ( 'NONE', #30585, #29752, #17833, .T. ) ;
#18743=CARTESIAN_POINT ( 'NONE',  ( 10.04305231718579705, 59.10000000546239107, 30.90933677959248982 ) ) ;
#18745=CARTESIAN_POINT ( 'NONE',  ( 10.37757302488624767, 37.72500000273118559, 31.93888565452638417 ) ) ;
#18746=CARTESIAN_POINT ( 'NONE',  ( 26.29305231718578995, 55.19999999999999574, -19.10302069950538240 ) ) ;
#18747=CARTESIAN_POINT ( 'NONE',  ( -33.58253175000000113, 59.27500000273119696, -10.91162601494193218 ) ) ;
#18751=CARTESIAN_POINT ( 'NONE',  ( 32.50000000000000000, 42.99999999999998579, -3.980102097228898626E-15 ) ) ;
#18753=CARTESIAN_POINT ( 'NONE',  ( 33.58253175000000113, 10.37500000273117173, -4.112674001490185761E-15 ) ) ;
#18754=CARTESIAN_POINT ( 'NONE',  ( -4.223320258572819786E-15, 19.24999999453763166, 24.50000000000000000 ) ) ;
#18756=CARTESIAN_POINT ( 'NONE',  ( -27.16883889988623935, 75.57500000273120122, 19.73931689729374739 ) ) ;
#18757=DIRECTION ( 'NONE',  ( 0.000000000000000000, 0.000000000000000000, -1.000000000000000000 ) ) ;
#18760=CARTESIAN_POINT ( 'NONE',  ( 3.980102097228898626E-15, 80.00000000000001421, 32.50000000000000000 ) ) ;
#18769=DIRECTION ( 'NONE',  ( -0.000000000000000000, -1.000000000000000000, -0.000000000000000000 ) ) ;
#18770=CARTESIAN_POINT ( 'NONE',  ( 33.58253175000000113, 36.12500000273119127, -4.112674001490185761E-15 ) ) ;
#18773=CARTESIAN_POINT ( 'NONE',  ( 3.980102097228898626E-15, 80.00000000000001421, 32.50000000000000000 ) ) ;
#18774=ORIENTED_EDGE ( 'NONE', *, *, #7702, .F. ) ;
#18776=CARTESIAN_POINT ( 'NONE',  ( -1.778240108872766143E-15, 51.50000000000000711, -32.49999999999999289 ) ) ;
#18778=CARTESIAN_POINT ( 'NONE',  ( -33.58253175000000113, 71.37500000273119838, 0.000000000000000000 ) ) ;
#18779=ORIENTED_EDGE ( 'NONE', *, *, #12008, .F. ) ;
#18785=CARTESIAN_POINT ( 'NONE',  ( 20.75514604977249178, 51.82500000273120122, 28.56700777964553950 ) ) ;
#18787=CARTESIAN_POINT ( 'NONE',  ( 6.277390505771533514E-15, 17.00000000546237544, 34.17252228774368916 ) ) ;
#18788=VECTOR ( 'NONE', #24394, 1000.000000000000000 ) ;
#18790=CARTESIAN_POINT ( 'NONE',  ( 14.47279130897151944, 7.424999997268819207, -19.92008829642072598 ) ) ;
#18791=CARTESIAN_POINT ( 'NONE',  ( -27.16883889988623935, 31.57500000273119767, 19.73931689729374739 ) ) ;
#18794=CARTESIAN_POINT ( 'NONE',  ( -26.29305231718578995, 32.20000000000000284, 19.10302069950538595 ) ) ;
#18799=CARTESIAN_POINT ( 'NONE',  ( -8.601468415847518756, 72.57500000273117280, -11.83890561707634781 ) ) ;
#18801=CARTESIAN_POINT ( 'NONE',  ( -10.37757302488624411, 24.72500000273119980, -31.93888565452638417 ) ) ;
#18804=CARTESIAN_POINT ( 'NONE',  ( 33.58253175000000113, 14.37500000273117529, -4.112674001490185761E-15 ) ) ;
#18806=CARTESIAN_POINT ( 'NONE',  ( 10.37757302488624056, 70.52500000273120406, -31.93888565452638417 ) ) ;
#18808=AXIS2_PLACEMENT_3D ( 'NONE', #29832, #6334, #19551 ) ;
#18811=CARTESIAN_POINT ( 'NONE',  ( -20.75514604977248823, 56.82500000273118701, -28.56700777964554305 ) ) ;
#18814=ORIENTED_EDGE ( 'NONE', *, *, #14919, .F. ) ;
#18816=CARTESIAN_POINT ( 'NONE',  ( -20.75514604977248112, 1.425000002731191984, 28.56700777964554661 ) ) ;
#18817=CARTESIAN_POINT ( 'NONE',  ( 23.41746825000000243, 8.724999997268806595, -7.608796670333727974 ) ) ;
#18819=ORIENTED_EDGE ( 'NONE', *, *, #1891, .F. ) ;
#18822=EDGE_CURVE ( 'NONE', #4234, #9459, #7007, .T. ) ;
#18823=ORIENTED_EDGE ( 'NONE', *, *, #32006, .F. ) ;
#18825=CARTESIAN_POINT ( 'NONE',  ( 20.08610463437157279, 11.80000000546236372, -27.64615127144129758 ) ) ;
#18827=DIRECTION ( 'NONE',  ( 0.8660254037844398178, 0.4999999999999979461, -0.000000000000000000 ) ) ;
#18829=CARTESIAN_POINT ( 'NONE',  ( -4.523095164977116484E-15, 18.12499999726880517, 24.62258325217400312 ) ) ;
#18830=CARTESIAN_POINT ( 'NONE',  ( 10.37757302488624056, 6.775000002731179194, -31.93888565452638417 ) ) ;
#18831=CARTESIAN_POINT ( 'NONE',  ( -10.04305231718578462, 58.40000000000000568, 30.90933677959249337 ) ) ;
#18832=CARTESIAN_POINT ( 'NONE',  ( 32.50000000000000711, 57.40000000546237402, 10.55989012756945122 ) ) ;
#18834=CARTESIAN_POINT ( 'NONE',  ( 2.688165632520823219E-15, 75.87500000273119838, 14.63369212191046387 ) ) ;
#18836=VECTOR ( 'NONE', #10740, 1000.000000000000000 ) ;
#18837=DIRECTION ( 'NONE',  ( 0.000000000000000000, 0.000000000000000000, -1.000000000000000000 ) ) ;
#18838=CARTESIAN_POINT ( 'NONE',  ( 0.000000000000000000, 0.000000000000000000, 0.000000000000000000 ) ) ;
#18840=CARTESIAN_POINT ( 'NONE',  ( -33.58253175000000113, 43.22500000273118559, 10.91162601494193929 ) ) ;
#18843=CARTESIAN_POINT ( 'NONE',  ( -33.58253175000000113, 35.37500000273119127, 0.000000000000000000 ) ) ;
#18844=CARTESIAN_POINT ( 'NONE',  ( 20.08610463437157279, 25.29999999999998295, -27.64615127144129758 ) ) ;
#18850=CARTESIAN_POINT ( 'NONE',  ( -18.94512977948576093, 1.824999997268816898, 13.76444248337722698 ) ) ;
#18851=DIRECTION ( 'NONE',  ( 0.000000000000000000, 0.000000000000000000, -1.000000000000000000 ) ) ;
#18854=CARTESIAN_POINT ( 'NONE',  ( -10.37757302488624411, 18.72500000273119625, -31.93888565452638417 ) ) ;
#18857=ORIENTED_EDGE ( 'NONE', *, *, #33212, .T. ) ;
#18859=ORIENTED_EDGE ( 'NONE', *, *, #27617, .T. ) ;
#18863=ORIENTED_EDGE ( 'NONE', *, *, #29589, .F. ) ;
#18864=CARTESIAN_POINT ( 'NONE',  ( 0.000000000000000000, 0.000000000000000000, 0.000000000000000000 ) ) ;
#18865=CARTESIAN_POINT ( 'NONE',  ( -33.58253175000000113, 31.27500000273118275, -10.91162601494193218 ) ) ;
#18866=CARTESIAN_POINT ( 'NONE',  ( 10.04305231718579705, 29.10000000546236620, 30.90933677959248982 ) ) ;
#18867=CARTESIAN_POINT ( 'NONE',  ( 32.50000000000000000, 79.00000000000001421, -3.980102097228898626E-15 ) ) ;
#18869=CARTESIAN_POINT ( 'NONE',  ( 27.16883889988623935, 44.57500000273117990, -19.73931689729374384 ) ) ;
#18872=CARTESIAN_POINT ( 'NONE',  ( 32.50000000000000000, 20.99999999999998934, -3.980102097228898626E-15 ) ) ;
#18874=CARTESIAN_POINT ( 'NONE',  ( 33.58253175000000113, 64.12500000273119838, -4.112674001490185761E-15 ) ) ;
#18877=CARTESIAN_POINT ( 'NONE',  ( -20.75514604977248112, 55.67500000273119554, 28.56700777964554661 ) ) ;
#18880=CARTESIAN_POINT ( 'NONE',  ( -10.37757302488623701, 5.525000002731205839, 31.93888565452638417 ) ) ;
#18882=EDGE_CURVE ( 'NONE', #14306, #4197, #32897, .T. ) ;
#18884=CARTESIAN_POINT ( 'NONE',  ( -32.50000000000000000, 19.90000000000001279, -10.55989012756945300 ) ) ;
#18889=EDGE_CURVE ( 'NONE', #4296, #17375, #29171, .T. ) ;
#18894=LINE ( 'NONE', #675, #32584 ) ;
#18897=CARTESIAN_POINT ( 'NONE',  ( -26.29305231718578995, 68.70000000546238539, 19.10302069950538595 ) ) ;
#18901=ORIENTED_EDGE ( 'NONE', *, *, #33839, .F. ) ;
#18906=CARTESIAN_POINT ( 'NONE',  ( -20.75514604977248112, 45.67500000273119554, 28.56700777964554661 ) ) ;
#18907=CARTESIAN_POINT ( 'NONE',  ( 32.50000000000000711, 55.40000000546238113, 10.55989012756945122 ) ) ;
#18908=( BOUNDED_CURVE ( )  B_SPLINE_CURVE ( 2, ( #2539, #13521, #33592, #5279, #18337, #3050, #31190, #8186, #31527, #28782, #18506, #5108, #20747 ),
 .UNSPECIFIED., .F., .F. ) 
 B_SPLINE_CURVE_WITH_KNOTS ( ( 3, 2, 2, 2, 2, 2, 3 ),
 ( 0.7756410256410256610, 0.7769230769230769384, 0.7794871794871794934, 0.7820512820512820484, 0.7846153846153846034, 0.7871794871794871584, 0.7884615384615384359 ),
 .UNSPECIFIED. ) 
 CURVE ( )  GEOMETRIC_REPRESENTATION_ITEM ( )  RATIONAL_B_SPLINE_CURVE ( ( 0.9755282581475768211, 0.9755282581475768211, 1.000000000000000000, 0.9510565162951535312, 1.000000000000000000, 0.9510565162951535312, 1.000000000000000000, 0.9510565162951535312, 1.000000000000000000, 0.9510565162951535312, 1.000000000000000000, 0.9755282581475768211, 0.9755282581475768211 ) ) 
 REPRESENTATION_ITEM ( '' )  );
#18910=CARTESIAN_POINT ( 'NONE',  ( 6.486482029760649416E-15, 33.62500000273119127, 35.31076352940723240 ) ) ;
#18911=CARTESIAN_POINT ( 'NONE',  ( 5.147494310547429563, 77.94874572391552192, -32.50000000000000000 ) ) ;
#18912=CARTESIAN_POINT ( 'NONE',  ( 33.58253175000000113, 60.37500000273119127, -4.112674001490185761E-15 ) ) ;
#18916=CARTESIAN_POINT ( 'NONE',  ( 26.29305231718578995, 39.20000000000000995, -19.10302069950538240 ) ) ;
#18918=CARTESIAN_POINT ( 'NONE',  ( -2.162160676586881955E-15, 2.875000002731204596, -35.31076352940723240 ) ) ;
#18920=CARTESIAN_POINT ( 'NONE',  ( 2.688165632520823219E-15, 73.87500000273119838, 14.63369212191046387 ) ) ;
#18921=CARTESIAN_POINT ( 'NONE',  ( 20.75514604977248467, 72.67500000273118133, -28.56700777964554305 ) ) ;
#18922=DIRECTION ( 'NONE',  ( -0.000000000000000000, -1.000000000000000000, -0.000000000000000000 ) ) ;
#18924=ORIENTED_EDGE ( 'NONE', *, *, #33, .F. ) ;
#18928=EDGE_CURVE ( 'NONE', #23800, #30543, #17658, .T. ) ;
#18939=CARTESIAN_POINT ( 'NONE',  ( 33.58253175000000113, 38.22500000273119269, -10.91162601494193574 ) ) ;
#18943=ORIENTED_EDGE ( 'NONE', *, *, #17634, .F. ) ;
#18945=CARTESIAN_POINT ( 'NONE',  ( -15.00000000000000000, 70.35000000546237686, 4.873795443493597723 ) ) ;
#18947=CARTESIAN_POINT ( 'NONE',  ( 33.58253175000000113, 68.47500000273119269, -10.91162601494193751 ) ) ;
#18948=ORIENTED_EDGE ( 'NONE', *, *, #32716, .F. ) ;
#18951=ORIENTED_EDGE ( 'NONE', *, *, #12936, .F. ) ;
#18952=CARTESIAN_POINT ( 'NONE',  ( 32.50000000000000000, 65.50000000546238255, -3.980102097228898626E-15 ) ) ;
#18953=CARTESIAN_POINT ( 'NONE',  ( 33.58253175000000113, 58.12500000273118417, -4.112674001490185761E-15 ) ) ;
#18955=CARTESIAN_POINT ( 'NONE',  ( -32.50000000000000000, 20.60000000546237686, 10.55989012756946366 ) ) ;
#18957=CARTESIAN_POINT ( 'NONE',  ( -14.47279130897151767, 9.824999997268800911, -19.92008829642072598 ) ) ;
#18958=CARTESIAN_POINT ( 'NONE',  ( 33.58253175000000113, 26.47500000273118559, -10.91162601494193751 ) ) ;
#18959=VECTOR ( 'NONE', #14978, 1000.000000000000000 ) ;
#18962=CARTESIAN_POINT ( 'NONE',  ( 2.688165632520823219E-15, 79.37500000273119838, 14.63369212191046387 ) ) ;
#18963=CARTESIAN_POINT ( 'NONE',  ( -20.08610463437157989, 28.20000000546236762, -27.64615127144129758 ) ) ;
#18967=CARTESIAN_POINT ( 'NONE',  ( -13.91746824999999887, 74.87500000273116996, 0.000000000000000000 ) ) ;
#18969=CARTESIAN_POINT ( 'NONE',  ( 33.58253175000000113, 26.12500000273118417, -4.112674001490185761E-15 ) ) ;
#18972=CARTESIAN_POINT ( 'NONE',  ( -20.75514604977248112, 17.67500000273117422, 28.56700777964554661 ) ) ;
#18974=CARTESIAN_POINT ( 'NONE',  ( -33.58253175000000113, 73.02500000273118985, -10.91162601494193041 ) ) ;
#18975=CARTESIAN_POINT ( 'NONE',  ( 0.000000000000000000, 80.00000000000001421, -32.50000000000000000 ) ) ;
#18976=CARTESIAN_POINT ( 'NONE',  ( 4.300734207923761154, 75.97500000273119269, 13.23629886949340495 ) ) ;
#18978=CARTESIAN_POINT ( 'NONE',  ( -15.00000000000000000, 72.15000000546237402, -4.873795443493594171 ) ) ;
#18979=CARTESIAN_POINT ( 'NONE',  ( 33.58253175000000113, 56.22500000273117138, -10.91162601494193574 ) ) ;
#18983=CARTESIAN_POINT ( 'NONE',  ( -32.50000000000000000, 15.89999999999998970, -10.55989012756945300 ) ) ;
#18984=AXIS2_PLACEMENT_3D ( 'NONE', #27170, #29730, #26552 ) ;
#18985=CARTESIAN_POINT ( 'NONE',  ( 14.47279130897151589, 6.324999997268824892, 19.92008829642072953 ) ) ;
#18987=ORIENTED_EDGE ( 'NONE', *, *, #1457, .T. ) ;
#18989=LINE ( 'NONE', #14165, #9373 ) ;
#18992=CARTESIAN_POINT ( 'NONE',  ( 5.147494310547426899, 11.94874572391553436, -32.50000000000000000 ) ) ;
#18994=CARTESIAN_POINT ( 'NONE',  ( 27.16883889988623935, 76.32500000273118701, -19.73931689729374384 ) ) ;
#18996=CARTESIAN_POINT ( 'NONE',  ( -24.50000000000000355, 8.900000000000011013, -7.960532557706207157 ) ) ;
#18997=CARTESIAN_POINT ( 'NONE',  ( 27.16883889988624290, 10.17500000273119376, 19.73931689729373673 ) ) ;
#18998=CARTESIAN_POINT ( 'NONE',  ( 27.16883889988623935, 14.32500000273117990, -19.73931689729374384 ) ) ;
#18999=CARTESIAN_POINT ( 'NONE',  ( -4.300734207923759378, 76.47500000273119269, -13.23629886949340495 ) ) ;
#19002=CARTESIAN_POINT ( 'NONE',  ( -8.601468415847515203, 75.67500000273118133, 11.83890561707634959 ) ) ;
#19005=CARTESIAN_POINT ( 'NONE',  ( 20.08610463437157279, 71.29999999999999716, -27.64615127144129758 ) ) ;
#19007=CARTESIAN_POINT ( 'NONE',  ( 27.16883889988624290, 45.92500000273119554, 19.73931689729373673 ) ) ;
#19010=CARTESIAN_POINT ( 'NONE',  ( 33.58253175000000113, 36.47500000273119269, -10.91162601494193574 ) ) ;
#19011=( BOUNDED_CURVE ( )  B_SPLINE_CURVE ( 2, ( #9214, #27250, #16792, #9380, #29813, #19862, #32554, #30316, #6813, #27928, #17294, #9053, #14717 ),
 .UNSPECIFIED., .F., .T. ) 
 B_SPLINE_CURVE_WITH_KNOTS ( ( 3, 2, 2, 2, 2, 2, 3 ),
 ( 0.9166666666666666297, 0.9179487179487179072, 0.9205128205128204621, 0.9230769230769231282, 0.9256410256410256832, 0.9282051282051282382, 0.9294871794871795156 ),
 .UNSPECIFIED. ) 
 CURVE ( )  GEOMETRIC_REPRESENTATION_ITEM ( )  RATIONAL_B_SPLINE_CURVE ( ( 0.9755282581475768211, 0.9755282581475768211, 1.000000000000000000, 0.9510565162951535312, 1.000000000000000000, 0.9510565162951535312, 1.000000000000000000, 0.9510565162951535312, 1.000000000000000000, 0.9510565162951535312, 1.000000000000000000, 0.9755282581475768211, 0.9755282581475768211 ) ) 
 REPRESENTATION_ITEM ( '' )  );
#19016=CARTESIAN_POINT ( 'NONE',  ( 5.779280353836490358E-15, 30.49999999999999645, 32.49999999999999289 ) ) ;
#19020=CARTESIAN_POINT ( 'NONE',  ( -18.94512977948575738, 1.424999997268805441, -13.76444248337723231 ) ) ;
#19021=ADVANCED_FACE ( 'NONE', ( #25717 ), #33432, .T. ) ;
#19024=CARTESIAN_POINT ( 'NONE',  ( 27.16883889988624290, 19.92500000273117422, 19.73931689729373673 ) ) ;
#19026=EDGE_CURVE ( 'NONE', #17621, #12035, #32903, .T. ) ;
#19027=ORIENTED_EDGE ( 'NONE', *, *, #32630, .T. ) ;
#19029=ADVANCED_FACE ( 'NONE', ( #25374 ), #23140, .T. ) ;
#19030=ORIENTED_EDGE ( 'NONE', *, *, #19442, .F. ) ;
#19034=EDGE_CURVE ( 'NONE', #18081, #5219, #33606, .T. ) ;
#19035=CARTESIAN_POINT ( 'NONE',  ( 1.507698388325705758E-15, 7.124999997268799845, -24.62258325217400312 ) ) ;
#19036=CARTESIAN_POINT ( 'NONE',  ( 33.58253175000000823, 30.27500000273118630, 10.91162601494192863 ) ) ;
#19037=CARTESIAN_POINT ( 'NONE',  ( -26.29305231718578995, 28.70000000546238539, 19.10302069950538595 ) ) ;
#19038=CARTESIAN_POINT ( 'NONE',  ( 20.08610463437158344, 76.70000000000000284, 27.64615127144129403 ) ) ;
#19039=LINE ( 'NONE', #10969, #17628 ) ;
#19040=CARTESIAN_POINT ( 'NONE',  ( 5.147494310547434893, 37.05125428700922185, 32.49999999999999289 ) ) ;
#19041=CARTESIAN_POINT ( 'NONE',  ( -20.75514604977248112, 45.67500000273119554, 28.56700777964554661 ) ) ;
#19042=AXIS2_PLACEMENT_3D ( 'NONE', #2906, #13547, #33965 ) ;
#19044=CARTESIAN_POINT ( 'NONE',  ( -32.50000000000000000, 19.90000000000001279, -10.55989012756945478 ) ) ;
#19046=CARTESIAN_POINT ( 'NONE',  ( 10.37757302488624056, 62.52500000273120406, -31.93888565452638417 ) ) ;
#19047=CARTESIAN_POINT ( 'NONE',  ( -2.162160676586882350E-15, 56.87500000273117706, -35.31076352940722529 ) ) ;
#19050=CARTESIAN_POINT ( 'NONE',  ( 10.37757302488624056, 2.525000002731203619, -31.93888565452638417 ) ) ;
#19052=CARTESIAN_POINT ( 'NONE',  ( 5.779280353836490358E-15, 25.00000000546237899, 32.49999999999999289 ) ) ;
#19057=CARTESIAN_POINT ( 'NONE',  ( 7.570916362186207671, 13.60000000000000142, 23.30088464923126779 ) ) ;
#19060=DIRECTION ( 'NONE',  ( 0.000000000000000000, 1.000000000000000000, 0.000000000000000000 ) ) ;
#19063=VECTOR ( 'NONE', #15789, 1000.000000000000000 ) ;
#19067=VERTEX_POINT ( 'NONE', #2197 ) ;
#19071=CARTESIAN_POINT ( 'NONE',  ( -10.04305231718578462, 36.39999999999999147, 30.90933677959249337 ) ) ;
#19072=CARTESIAN_POINT ( 'NONE',  ( -27.16883889988623935, 47.57500000273117990, 19.73931689729374739 ) ) ;
#19073=CARTESIAN_POINT ( 'NONE',  ( 26.29305231718578995, 49.70000000546237118, -19.10302069950538240 ) ) ;
#19076=CARTESIAN_POINT ( 'NONE',  ( 10.37757302488624056, 34.52500000273117564, -31.93888565452638417 ) ) ;
#19077=DIRECTION ( 'NONE',  ( -0.000000000000000000, -1.000000000000000000, -0.000000000000000000 ) ) ;
#19078=CARTESIAN_POINT ( 'NONE',  ( 33.58253175000000113, 64.47500000273120691, -10.91162601494193751 ) ) ;
#19079=CARTESIAN_POINT ( 'NONE',  ( 6.277390505771533514E-15, 42.50000000000000000, 34.17252228774368916 ) ) ;
#19081=CARTESIAN_POINT ( 'NONE',  ( 33.58253175000000113, 4.375000002731193938, -4.112674001490185761E-15 ) ) ;
#19082=DIRECTION ( 'NONE',  ( 0.000000000000000000, 0.000000000000000000, -1.000000000000000000 ) ) ;
#19083=CARTESIAN_POINT ( 'NONE',  ( 11.25946833292375793, 74.57500000273120122, -8.180482586598735395 ) ) ;
#19084=CARTESIAN_POINT ( 'NONE',  ( -33.58253175000000113, 73.37500000273116996, 0.000000000000000000 ) ) ;
#19085=CARTESIAN_POINT ( 'NONE',  ( 24.50000000000000000, 3.649999994537613812, 7.960532557706212486 ) ) ;
#19086=APPLICATION_CONTEXT ( 'automotive_design' ) ;
#19090=AXIS2_PLACEMENT_3D ( 'NONE', #11220, #32140, #4670 ) ;
#19100=CARTESIAN_POINT ( 'NONE',  ( 3.980102097228898626E-15, 80.00000000000001421, 32.50000000000000000 ) ) ;
#19103=CARTESIAN_POINT ( 'NONE',  ( 10.04305231718579705, 13.10000000546238041, 30.90933677959248982 ) ) ;
#19104=ORIENTED_EDGE ( 'NONE', *, *, #31881, .T. ) ;
#19106=( BOUNDED_CURVE ( )  B_SPLINE_CURVE ( 2, ( #6164, #3930, #29660, #671, #21630, #27271, #21960, #8738, #19223, #19389, #27438, #32076, #16317 ),
 .UNSPECIFIED., .F., .T. ) 
 B_SPLINE_CURVE_WITH_KNOTS ( ( 3, 2, 2, 2, 2, 2, 3 ),
 ( 0.9807692307692307265, 0.9820512820512820040, 0.9846153846153846700, 0.9871794871794872250, 0.9897435897435897800, 0.9923076923076923350, 0.9935897435897436125 ),
 .UNSPECIFIED. ) 
 CURVE ( )  GEOMETRIC_REPRESENTATION_ITEM ( )  RATIONAL_B_SPLINE_CURVE ( ( 0.9755282581475768211, 0.9755282581475768211, 1.000000000000000000, 0.9510565162951535312, 1.000000000000000000, 0.9510565162951535312, 1.000000000000000000, 0.9510565162951535312, 1.000000000000000000, 0.9510565162951535312, 1.000000000000000000, 0.9755282581475768211, 0.9755282581475768211 ) ) 
 REPRESENTATION_ITEM ( '' )  );
#19107=CARTESIAN_POINT ( 'NONE',  ( -32.50000000000000000, 50.60000000546236265, 10.55989012756946366 ) ) ;
#19109=CARTESIAN_POINT ( 'NONE',  ( -10.37757302488624411, 66.97500000273117848, -31.93888565452638417 ) ) ;
#19110=ORIENTED_EDGE ( 'NONE', *, *, #31228, .T. ) ;
#19114=ORIENTED_EDGE ( 'NONE', *, *, #26149, .F. ) ;
#19115=CARTESIAN_POINT ( 'NONE',  ( -26.29305231718579350, 48.30000000546236549, -19.10302069950537884 ) ) ;
#19116=CARTESIAN_POINT ( 'NONE',  ( -10.37757302488623701, 57.52500000273119696, 31.93888565452638417 ) ) ;
#19118=EDGE_CURVE ( 'NONE', #12293, #23252, #5967, .T. ) ;
#19119=CARTESIAN_POINT ( 'NONE',  ( 6.277390505771533514E-15, 19.00000000546236834, 34.17252228774368916 ) ) ;
#19121=CARTESIAN_POINT ( 'NONE',  ( 23.41746824999999887, 11.22499999726881548, -7.608796670333727974 ) ) ;
#19122=CARTESIAN_POINT ( 'NONE',  ( -2.162160676586881955E-15, 20.87500000273119127, -35.31076352940723240 ) ) ;
#19125=CARTESIAN_POINT ( 'NONE',  ( 0.000000000000000000, 0.000000000000000000, 26.50000000000000355 ) ) ;
#19130=CARTESIAN_POINT ( 'NONE',  ( 8.601468415847516980, 74.17500000273119554, -11.83890561707634781 ) ) ;
#19132=CARTESIAN_POINT ( 'NONE',  ( -10.37757302488624411, 22.72500000273119980, -31.93888565452638417 ) ) ;
#19136=CARTESIAN_POINT ( 'NONE',  ( -27.16883889988624290, 9.175000002731191984, -19.73931689729374028 ) ) ;
#19138=CARTESIAN_POINT ( 'NONE',  ( 33.58253175000000823, 72.02500000273118985, 10.91162601494192685 ) ) ;
#19141=CARTESIAN_POINT ( 'NONE',  ( 4.300734207923761154, 77.97500000273119269, 13.23629886949340495 ) ) ;
#19143=CARTESIAN_POINT ( 'NONE',  ( 10.37757302488624056, 60.52500000273119696, -31.93888565452638417 ) ) ;
#19145=( BOUNDED_CURVE ( )  B_SPLINE_CURVE ( 2, ( #18380, #18548, #5324, #15804, #20620, #5493, #33641, #4983, #17869, #154, #10138, #26260, #2748 ),
 .UNSPECIFIED., .F., .F. ) 
 B_SPLINE_CURVE_WITH_KNOTS ( ( 3, 2, 2, 2, 2, 2, 3 ),
 ( 0.08333333333333334259, 0.08461538461538462008, 0.08717948717948717507, 0.08974358974358974395, 0.09230769230769231282, 0.09487179487179486781, 0.09615384615384615918 ),
 .UNSPECIFIED. ) 
 CURVE ( )  GEOMETRIC_REPRESENTATION_ITEM ( )  RATIONAL_B_SPLINE_CURVE ( ( 0.9755282581475767101, 0.9755282581475768211, 1.000000000000000000, 0.9510565162951535312, 1.000000000000000000, 0.9510565162951535312, 1.000000000000000000, 0.9510565162951535312, 1.000000000000000000, 0.9510565162951535312, 1.000000000000000000, 0.9755282581475765991, 0.9755282581475767101 ) ) 
 REPRESENTATION_ITEM ( '' )  );
#19146=ORIENTED_EDGE ( 'NONE', *, *, #5812, .F. ) ;
#19148=CARTESIAN_POINT ( 'NONE',  ( 27.16883889988624290, 1.925000002731186433, 19.73931689729373673 ) ) ;
#19149=CARTESIAN_POINT ( 'NONE',  ( 23.41746825000000243, 4.724999997268818142, -7.608796670333727974 ) ) ;
#19153=CARTESIAN_POINT ( 'NONE',  ( -4.934616302121927505E-14, 69.00000000546236834, 32.50000000000000000 ) ) ;
#19154=ORIENTED_EDGE ( 'NONE', *, *, #19026, .T. ) ;
#19156=CARTESIAN_POINT ( 'NONE',  ( 26.29305231718578995, 11.70000000546239605, -19.10302069950538240 ) ) ;
#19158=CARTESIAN_POINT ( 'NONE',  ( -20.75514604977248823, 74.82500000273115859, -28.56700777964554305 ) ) ;
#19160=CARTESIAN_POINT ( 'NONE',  ( 1.577395562988744260E-15, 4.500000000000003553, -25.76082449383753925 ) ) ;
#19161=EDGE_CURVE ( 'NONE', #29590, #30543, #33107, .T. ) ;
#19162=CARTESIAN_POINT ( 'NONE',  ( -2.162160676586881955E-15, 6.875000002731195714, -35.31076352940723240 ) ) ;
#19163=ADVANCED_FACE ( 'NONE', ( #31203 ), #26569, .T. ) ;
#19164=CARTESIAN_POINT ( 'NONE',  ( 33.58253175000000823, 18.02500000273118630, 10.91162601494192863 ) ) ;
#19165=CARTESIAN_POINT ( 'NONE',  ( -8.960552108402744065E-16, 76.37500000273116996, -14.63369212191046209 ) ) ;
#19168=CARTESIAN_POINT ( 'NONE',  ( -9.657523855033125146E-16, 81.50000000000002842, -15.77193336357400710 ) ) ;
#19171=CARTESIAN_POINT ( 'NONE',  ( 26.29305231718578995, 71.19999999999998863, -19.10302069950538240 ) ) ;
#19173=CARTESIAN_POINT ( 'NONE',  ( 33.58253175000000823, 42.02500000273118985, 10.91162601494192863 ) ) ;
#19176=CARTESIAN_POINT ( 'NONE',  ( -10.37757302488623701, 25.77500000273119696, 31.93888565452638417 ) ) ;
#19182=CARTESIAN_POINT ( 'NONE',  ( -4.523095164977117273E-15, 4.124999997268806951, 24.62258325217400312 ) ) ;
#19186=CARTESIAN_POINT ( 'NONE',  ( -33.58253175000000113, 21.02500000273118275, -10.91162601494193041 ) ) ;
#19187=CARTESIAN_POINT ( 'NONE',  ( 23.41746825000000243, 3.024999997268812635, 7.608796670333735079 ) ) ;
#19191=ORIENTED_EDGE ( 'NONE', *, *, #31468, .F. ) ;
#19194=CARTESIAN_POINT ( 'NONE',  ( 32.50000000000000000, 39.00000000000000711, -3.980102097228898626E-15 ) ) ;
#19195=CARTESIAN_POINT ( 'NONE',  ( -14.47279130897152122, 3.924999997268813434, 19.92008829642072243 ) ) ;
#19196=CARTESIAN_POINT ( 'NONE',  ( -33.58253175000000113, 27.37500000273118772, 0.000000000000000000 ) ) ;
#19197=CARTESIAN_POINT ( 'NONE',  ( -20.08610463437157989, 28.20000000546236762, -27.64615127144129758 ) ) ;
#19198=CARTESIAN_POINT ( 'NONE',  ( 10.04305231718579705, 74.59999999999999432, 30.90933677959248982 ) ) ;
#19200=DIRECTION ( 'NONE',  ( 0.000000000000000000, 0.000000000000000000, -1.000000000000000000 ) ) ;
#19202=CARTESIAN_POINT ( 'NONE',  ( -33.58253175000000113, 41.27500000273117564, -10.91162601494193218 ) ) ;
#19204=( BOUNDED_CURVE ( )  B_SPLINE_CURVE ( 2, ( #24967, #1449, #6775, #29943, #12092, #29769, #9338 ),
 .UNSPECIFIED., .F., .T. ) 
 B_SPLINE_CURVE_WITH_KNOTS ( ( 3, 2, 2, 3 ),
 ( 0.9935897435897436125, 0.9948717948717948900, 0.9974358974358974450, 1.000000000000000000 ),
 .UNSPECIFIED. ) 
 CURVE ( )  GEOMETRIC_REPRESENTATION_ITEM ( )  RATIONAL_B_SPLINE_CURVE ( ( 0.9755282581475768211, 0.9755282581475768211, 1.000000000000000000, 0.9510565162951535312, 1.000000000000000000, 0.9510565162951535312, 1.000000000000000000 ) ) 
 REPRESENTATION_ITEM ( '' )  );
#19205=CARTESIAN_POINT ( 'NONE',  ( 23.41746825000000243, 7.224999997268826135, -7.608796670333727974 ) ) ;
#19206=CARTESIAN_POINT ( 'NONE',  ( -20.08610463437156923, 18.30000000000000782, 27.64615127144130113 ) ) ;
#19209=( BOUNDED_CURVE ( )  B_SPLINE_CURVE ( 2, ( #4377, #10047, #30971, #17432, #7470, #31145, #17599, #30796, #17953, #4209, #20177, #4891, #1790 ),
 .UNSPECIFIED., .F., .F. ) 
 B_SPLINE_CURVE_WITH_KNOTS ( ( 3, 2, 2, 2, 2, 2, 3 ),
 ( 0.7500000000000000000, 0.7512820512820512775, 0.7538461538461538325, 0.7564102564102563875, 0.7589743589743589425, 0.7615384615384614975, 0.7628205128205127750 ),
 .UNSPECIFIED. ) 
 CURVE ( )  GEOMETRIC_REPRESENTATION_ITEM ( )  RATIONAL_B_SPLINE_CURVE ( ( 0.9755282581475768211, 0.9755282581475768211, 1.000000000000000000, 0.9510565162951535312, 1.000000000000000000, 0.9510565162951535312, 1.000000000000000000, 0.9510565162951535312, 1.000000000000000000, 0.9510565162951535312, 1.000000000000000000, 0.9755282581475768211, 0.9755282581475768211 ) ) 
 REPRESENTATION_ITEM ( '' )  );
#19210=CARTESIAN_POINT ( 'NONE',  ( -10.37757302488623701, 65.52500000273120406, 31.93888565452638417 ) ) ;
#19211=CARTESIAN_POINT ( 'NONE',  ( -27.16883889988623935, 53.57500000273118701, 19.73931689729374739 ) ) ;
#19215=CARTESIAN_POINT ( 'NONE',  ( 6.486482029760649416E-15, 3.625000002731181059, 35.31076352940723240 ) ) ;
#19217=CARTESIAN_POINT ( 'NONE',  ( 0.000000000000000000, 80.00000000000001421, 0.000000000000000000 ) ) ;
#19218=DIRECTION ( 'NONE',  ( 0.000000000000000000, 0.000000000000000000, -1.000000000000000000 ) ) ;
#19221=DIRECTION ( 'NONE',  ( 0.8660254037844410391, -0.4999999999999958367, -0.000000000000000000 ) ) ;
#19222=ADVANCED_FACE ( 'NONE', ( #3065 ), #5462, .T. ) ;
#19223=CARTESIAN_POINT ( 'NONE',  ( 26.29305231718579350, 1.300000005462376151, 19.10302069950537529 ) ) ;
#19236=CARTESIAN_POINT ( 'NONE',  ( 5.779280353836490358E-15, 47.00000000546238255, 32.49999999999999289 ) ) ;
#19237=CARTESIAN_POINT ( 'NONE',  ( 33.58253175000000823, 50.27500000273118985, 10.91162601494192863 ) ) ;
#19238=CARTESIAN_POINT ( 'NONE',  ( -32.50000000000000000, 48.60000000546236976, 10.55989012756946366 ) ) ;
#19240=CARTESIAN_POINT ( 'NONE',  ( 20.75514604977248467, 38.42500000273118133, -28.56700777964554305 ) ) ;
#19241=CARTESIAN_POINT ( 'NONE',  ( 20.08610463437158344, 77.20000000546238539, 27.64615127144129403 ) ) ;
#19242=CARTESIAN_POINT ( 'NONE',  ( 27.16883889988624290, 64.17500000273118133, 19.73931689729373673 ) ) ;
#19243=CARTESIAN_POINT ( 'NONE',  ( 20.08610463437158344, 38.70000000000000284, 27.64615127144129403 ) ) ;
#19245=CARTESIAN_POINT ( 'NONE',  ( 20.75514604977248467, 6.675000002731201754, -28.56700777964554305 ) ) ;
#19248=CARTESIAN_POINT ( 'NONE',  ( -33.58253175000000113, 75.37500000273116996, 0.000000000000000000 ) ) ;
#19252=CARTESIAN_POINT ( 'NONE',  ( -7.570916362186210335, 2.349999994537638415, -23.30088464923126779 ) ) ;
#19254=CARTESIAN_POINT ( 'NONE',  ( 15.00000000000000000, 75.00000000000001421, -1.836970198721029589E-15 ) ) ;
#19262=VECTOR ( 'NONE', #25249, 1000.000000000000000 ) ;
#19266=CARTESIAN_POINT ( 'NONE',  ( 32.50000000000000711, 58.90000000000000568, 10.55989012756945122 ) ) ;
#19267=EDGE_LOOP ( 'NONE', ( #11951, #11866, #26744, #2306 ) ) ;
#19272=CARTESIAN_POINT ( 'NONE',  ( -27.16883889988623935, 71.57500000273120122, 19.73931689729374739 ) ) ;
#19277=CARTESIAN_POINT ( 'NONE',  ( 26.29305231718579350, 65.30000000546237970, 19.10302069950537529 ) ) ;
#19278=CARTESIAN_POINT ( 'NONE',  ( 20.75514604977249178, 53.82500000273119412, 28.56700777964553950 ) ) ;
#19280=CARTESIAN_POINT ( 'NONE',  ( -20.08610463437156923, 10.80000000546236549, 27.64615127144130113 ) ) ;
#19281=CARTESIAN_POINT ( 'NONE',  ( 24.50000000000000000, 15.74999999453763344, 0.000000000000000000 ) ) ;
#19282=CARTESIAN_POINT ( 'NONE',  ( 23.41746824999999887, 17.22499999726879594, -7.608796670333727974 ) ) ;
#19283=CARTESIAN_POINT ( 'NONE',  ( 10.37757302488624056, 24.77500000273119696, -31.93888565452638417 ) ) ;
#19284=CARTESIAN_POINT ( 'NONE',  ( -26.29305231718578995, 24.70000000546238184, 19.10302069950538595 ) ) ;
#19286=CARTESIAN_POINT ( 'NONE',  ( -11.25946833292375793, 74.67500000273119554, -8.180482586598733619 ) ) ;
#19287=CARTESIAN_POINT ( 'NONE',  ( 20.08610463437158344, 64.70000000000001705, 27.64615127144129403 ) ) ;
#19288=CARTESIAN_POINT ( 'NONE',  ( 4.445600272181915325E-13, 15.49999999999999822, -32.50000000000000000 ) ) ;
#19290=ORIENTED_EDGE ( 'NONE', *, *, #17767, .T. ) ;
#19292=CARTESIAN_POINT ( 'NONE',  ( 11.25946833292375793, 75.67500000273119554, 8.180482586598731842 ) ) ;
#19294=CARTESIAN_POINT ( 'NONE',  ( -2.162160676586881955E-15, 18.62500000273117351, -35.31076352940723240 ) ) ;
#19298=CARTESIAN_POINT ( 'NONE',  ( 20.75514604977248467, 6.675000002731200865, -28.56700777964554305 ) ) ;
#19301=CYLINDRICAL_SURFACE ( 'NONE', #20419, 24.50000000000000000 ) ;
#19303=( BOUNDED_CURVE ( )  B_SPLINE_CURVE ( 2, ( #18217, #13216, #2415, #28996, #16148, #21298, #31568 ),
 .UNSPECIFIED., .F., .F. ) 
 B_SPLINE_CURVE_WITH_KNOTS ( ( 3, 2, 2, 3 ),
 ( 0.000000000000000000, 0.01111111111111111154, 0.02222222222222222307, 0.02777777777777777624 ),
 .UNSPECIFIED. ) 
 CURVE ( )  GEOMETRIC_REPRESENTATION_ITEM ( )  RATIONAL_B_SPLINE_CURVE ( ( 1.000000000000000000, 0.9510565162951535312, 1.000000000000000000, 0.9510565162951535312, 1.000000000000000000, 0.9755282581475768211, 0.9755282581475768211 ) ) 
 REPRESENTATION_ITEM ( '' )  );
#19304=CARTESIAN_POINT ( 'NONE',  ( -8.601468415847518756, 75.07500000273118701, -11.83890561707634603 ) ) ;
#19307=CARTESIAN_POINT ( 'NONE',  ( -2.162160676586882350E-15, 48.62500000273118417, -35.31076352940722529 ) ) ;
#19308=EDGE_CURVE ( 'NONE', #30741, #29542, #3758, .T. ) ;
#19313=CARTESIAN_POINT ( 'NONE',  ( -18.94512977948575738, 7.424999997268811214, -13.76444248337723231 ) ) ;
#19315=ORIENTED_EDGE ( 'NONE', *, *, #9555, .T. ) ;
#19320=CARTESIAN_POINT ( 'NONE',  ( 10.37757302488624767, 61.97500000273120691, 31.93888565452638417 ) ) ;
#19321=CARTESIAN_POINT ( 'NONE',  ( 26.29305231718578995, 69.70000000546238539, -19.10302069950538240 ) ) ;
#19322=CARTESIAN_POINT ( 'NONE',  ( -2.162160676586881955E-15, 72.62500000273118417, -35.31076352940723240 ) ) ;
#19324=CARTESIAN_POINT ( 'NONE',  ( -7.570916362186210335, 6.599999999999994316, -23.30088464923126779 ) ) ;
#19325=DIRECTION ( 'NONE',  ( -0.000000000000000000, -1.000000000000000000, -0.000000000000000000 ) ) ;
#19326=CARTESIAN_POINT ( 'NONE',  ( -20.75514604977248112, 19.42500000273117777, 28.56700777964554661 ) ) ;
#19327=CARTESIAN_POINT ( 'NONE',  ( 2.688165632520823219E-15, 71.37500000273119838, 14.63369212191046209 ) ) ;
#19329=CARTESIAN_POINT ( 'NONE',  ( 9.270509831248425314, 80.69999999999998863, 12.75976212528059683 ) ) ;
#19334=CARTESIAN_POINT ( 'NONE',  ( -27.16883889988623935, 43.32500000273120833, 19.73931689729374739 ) ) ;
#19338=CARTESIAN_POINT ( 'NONE',  ( 27.16883889988624290, 30.17500000273118488, 19.73931689729373673 ) ) ;
#19339=DIRECTION ( 'NONE',  ( 0.8660254037844410391, 0.4999999999999958367, 0.000000000000000000 ) ) ;
#19344=ADVANCED_FACE ( 'NONE', ( #20921 ), #7527, .T. ) ;
#19345=CARTESIAN_POINT ( 'NONE',  ( -10.04305231718578462, 44.90000000546237402, 30.90933677959249337 ) ) ;
#19348=CARTESIAN_POINT ( 'NONE',  ( -7.236395654485763274, 4.024999997268824181, 22.27133577429736633 ) ) ;
#19350=CARTESIAN_POINT ( 'NONE',  ( -32.50000000000000000, 52.40000000546238823, -10.55989012756945300 ) ) ;
#19352=CARTESIAN_POINT ( 'NONE',  ( -15.00000000000000000, 76.35000000546234844, 4.873795443493597723 ) ) ;
#19353=CARTESIAN_POINT ( 'NONE',  ( -33.58253175000000113, 21.12500000273118062, 0.000000000000000000 ) ) ;
#19354=CARTESIAN_POINT ( 'NONE',  ( 23.41746824999999887, 3.124999997268812280, 0.000000000000000000 ) ) ;
#19359=VERTEX_POINT ( 'NONE', #7861 ) ;
#19363=CARTESIAN_POINT ( 'NONE',  ( -26.29305231718578995, 10.19999999999998685, 19.10302069950538595 ) ) ;
#19364=CARTESIAN_POINT ( 'NONE',  ( -7.570916362186210335, 14.34999999453762065, -23.30088464923126779 ) ) ;
#19366=CARTESIAN_POINT ( 'NONE',  ( 23.41746825000000243, 6.724999997268811924, -7.608796670333727974 ) ) ;
#19367=CARTESIAN_POINT ( 'NONE',  ( -27.16883889988623935, 29.57500000273119412, 19.73931689729374739 ) ) ;
#19368=CARTESIAN_POINT ( 'NONE',  ( 26.29305231718578995, 33.70000000546238539, -19.10302069950538240 ) ) ;
#19369=CARTESIAN_POINT ( 'NONE',  ( 20.08610463437157279, 71.29999999999999716, -27.64615127144129758 ) ) ;
#19370=CARTESIAN_POINT ( 'NONE',  ( -14.45873412499999944, 70.56250000409680467, 0.000000000000000000 ) ) ;
#19372=CARTESIAN_POINT ( 'NONE',  ( -33.58253175000000113, 41.37500000273119838, 0.000000000000000000 ) ) ;
#19373=CARTESIAN_POINT ( 'NONE',  ( 14.47279130897151589, 8.824999997268804464, 19.92008829642072953 ) ) ;
#19374=CARTESIAN_POINT ( 'NONE',  ( -32.50000000000000000, 12.09999999999999787, 10.55989012756946366 ) ) ;
#19377=CARTESIAN_POINT ( 'NONE',  ( -33.58253175000000113, 61.22500000273118559, 10.91162601494193929 ) ) ;
#19378=CARTESIAN_POINT ( 'NONE',  ( -33.58253175000000113, 47.37500000273120548, 0.000000000000000000 ) ) ;
#19381=CARTESIAN_POINT ( 'NONE',  ( 33.58253175000000113, 4.125000002731193938, -4.112674001490185761E-15 ) ) ;
#19383=DIRECTION ( 'NONE',  ( -0.000000000000000000, -1.000000000000000000, -0.000000000000000000 ) ) ;
#19387=CARTESIAN_POINT ( 'NONE',  ( 5.779280353836490358E-15, 21.00000000546237544, 32.49999999999999289 ) ) ;
#19388=VECTOR ( 'NONE', #5293, 1000.000000000000000 ) ;
#19389=CARTESIAN_POINT ( 'NONE',  ( 20.08610463437158344, 1.200000005462378283, 27.64615127144129403 ) ) ;
#19393=( NAMED_UNIT ( * ) PLANE_ANGLE_UNIT ( ) SI_UNIT ( $, .RADIAN. ) );
#19397=DIRECTION ( 'NONE',  ( -0.000000000000000000, -1.000000000000000000, -0.000000000000000000 ) ) ;
#19398=ORIENTED_EDGE ( 'NONE', *, *, #3894, .F. ) ;
#19403=CARTESIAN_POINT ( 'NONE',  ( -26.29305231718579350, 46.30000000546238681, -19.10302069950537884 ) ) ;
#19404=CARTESIAN_POINT ( 'NONE',  ( 27.16883889988624290, 48.17500000273117422, 19.73931689729373673 ) ) ;
#19405=CARTESIAN_POINT ( 'NONE',  ( -20.08610463437157989, 50.20000000546237118, -27.64615127144129758 ) ) ;
#19407=CARTESIAN_POINT ( 'NONE',  ( 20.75514604977249178, 33.82500000273117990, 28.56700777964553950 ) ) ;
#19409=CARTESIAN_POINT ( 'NONE',  ( 33.58253175000000113, 64.37500000273119838, -4.112674001490185761E-15 ) ) ;
#19411=CARTESIAN_POINT ( 'NONE',  ( 20.08610463437157279, 35.29999999999999716, -27.64615127144129758 ) ) ;
#19413=CARTESIAN_POINT ( 'NONE',  ( -33.58253175000000113, 5.475000002731181148, 10.91162601494193929 ) ) ;
#19414=CARTESIAN_POINT ( 'NONE',  ( 20.08610463437157279, 13.29999999999998650, -27.64615127144129758 ) ) ;
#19416=CARTESIAN_POINT ( 'NONE',  ( -10.37757302488624411, 64.97500000273120691, -31.93888565452638417 ) ) ;
#19419=EDGE_LOOP ( 'NONE', ( #12814, #1735, #22487, #31251 ) ) ;
#19420=CARTESIAN_POINT ( 'NONE',  ( -4.732186688966233175E-15, 7.249999994537616566, 25.76082449383753925 ) ) ;
#19433=CARTESIAN_POINT ( 'NONE',  ( -20.08610463437156923, 58.29999999999999716, 27.64615127144130113 ) ) ;
#19435=CARTESIAN_POINT ( 'NONE',  ( 5.147494310547434893, 58.55125428154682510, 32.49999999999999289 ) ) ;
#19436=EDGE_LOOP ( 'NONE', ( #3070, #29310, #19643, #597 ) ) ;
#19440=ORIENTED_EDGE ( 'NONE', *, *, #31799, .T. ) ;
#19442=EDGE_CURVE ( 'NONE', #3647, #22014, #23715, .T. ) ;
#19443=ADVANCED_FACE ( 'NONE', ( #21591 ), #3230, .T. ) ;
#19447=CARTESIAN_POINT ( 'NONE',  ( -10.37757302488623701, 53.52500000273118985, 31.93888565452638417 ) ) ;
#19449=CARTESIAN_POINT ( 'NONE',  ( 32.50000000000000000, 9.600000005462375086, -10.55989012756945833 ) ) ;
#19451=CARTESIAN_POINT ( 'NONE',  ( 18.94512977948576093, 17.32499999726880446, -13.76444248337722875 ) ) ;
#19453=CARTESIAN_POINT ( 'NONE',  ( 10.04305231718579705, 56.59999999999998010, 30.90933677959248982 ) ) ;
#19454=CARTESIAN_POINT ( 'NONE',  ( -33.58253175000000113, 21.27500000273117209, -10.91162601494193218 ) ) ;
#19456=CARTESIAN_POINT ( 'NONE',  ( 11.25946833292375793, 73.67500000273119554, 8.180482586598731842 ) ) ;
#19457=CARTESIAN_POINT ( 'NONE',  ( 3.880418787951172011, 15.55125428154684819, 24.49999999999998579 ) ) ;
#19458=CARTESIAN_POINT ( 'NONE',  ( 5.779280353836490358E-15, 29.00000000546237544, 32.49999999999999289 ) ) ;
#19462=CARTESIAN_POINT ( 'NONE',  ( -4.300734207923755825, 71.27500000273117564, 13.23629886949340673 ) ) ;
#19464=CARTESIAN_POINT ( 'NONE',  ( 33.58253175000000113, 20.12500000273118062, -4.112674001490185761E-15 ) ) ;
#19468=CARTESIAN_POINT ( 'NONE',  ( 33.58253175000000823, 12.27500000273116854, 10.91162601494192685 ) ) ;
#19471=CARTESIAN_POINT ( 'NONE',  ( 13.91746824999999887, 76.37500000273116996, -1.704398294459741270E-15 ) ) ;
#19473=DIRECTION ( 'NONE',  ( 0.000000000000000000, 1.000000000000000000, 0.000000000000000000 ) ) ;
#19474=CARTESIAN_POINT ( 'NONE',  ( 20.75514604977249178, 49.82500000273117990, 28.56700777964553950 ) ) ;
#19477=ORIENTED_EDGE ( 'NONE', *, *, #22577, .F. ) ;
#19479=DIRECTION ( 'NONE',  ( 0.000000000000000000, 0.000000000000000000, -1.000000000000000000 ) ) ;
#19480=CARTESIAN_POINT ( 'NONE',  ( -18.94512977948575738, 5.424999997268809437, -13.76444248337723231 ) ) ;
#19484=CARTESIAN_POINT ( 'NONE',  ( 19.82091636218621389, 6.200000000000010836, -14.40073868116559197 ) ) ;
#19487=CARTESIAN_POINT ( 'NONE',  ( 33.58253175000000823, 60.27500000273116143, 10.91162601494192863 ) ) ;
#19489=CARTESIAN_POINT ( 'NONE',  ( -27.16883889988623935, 73.32500000273117280, 19.73931689729374739 ) ) ;
#19491=CARTESIAN_POINT ( 'NONE',  ( 19.82091636218621389, 6.200000000000010836, -14.40073868116559197 ) ) ;
#19492=CARTESIAN_POINT ( 'NONE',  ( 33.58253175000000113, 2.375000002731192161, -4.112674001490185761E-15 ) ) ;
#19494=CARTESIAN_POINT ( 'NONE',  ( -10.37757302488623701, 19.52500000273118985, 31.93888565452638417 ) ) ;
#19497=CARTESIAN_POINT ( 'NONE',  ( 4.635254915624209993, 79.39999999999999147, -14.26584774442730463 ) ) ;
#19499=DIRECTION ( 'NONE',  ( -0.000000000000000000, -1.000000000000000000, -0.000000000000000000 ) ) ;
#19501=CARTESIAN_POINT ( 'NONE',  ( 5.147494310547434893, 49.05125428700922185, 32.49999999999999289 ) ) ;
#19504=CARTESIAN_POINT ( 'NONE',  ( -20.75514604977248112, 39.42500000273118843, 28.56700777964554661 ) ) ;
#19507=CARTESIAN_POINT ( 'NONE',  ( -10.37757302488624411, 28.97500000273117848, -31.93888565452638417 ) ) ;
#19510=CARTESIAN_POINT ( 'NONE',  ( 2.375766604868043697, 80.55125428154684641, 15.00000000000000178 ) ) ;
#19512=CARTESIAN_POINT ( 'NONE',  ( 14.47279130897151767, 12.32499999726880802, 19.92008829642072953 ) ) ;
#19517=CARTESIAN_POINT ( 'NONE',  ( 27.16883889988624290, 15.92500000273117067, 19.73931689729373673 ) ) ;
#19518=CARTESIAN_POINT ( 'NONE',  ( 18.94512977948575738, 4.924999997268808549, 13.76444248337723408 ) ) ;
#19520=ORIENTED_EDGE ( 'NONE', *, *, #30596, .F. ) ;
#19523=ORIENTED_EDGE ( 'NONE', *, *, #1457, .F. ) ;
#19527=CARTESIAN_POINT ( 'NONE',  ( 1.577395562988744260E-15, 18.24999999453762101, -25.76082449383753925 ) ) ;
#19528=CARTESIAN_POINT ( 'NONE',  ( 23.41746825000000243, 2.524999997268798868, 7.608796670333735079 ) ) ;
#19529=CARTESIAN_POINT ( 'NONE',  ( -20.75514604977248112, 19.67500000273119909, 28.56700777964554661 ) ) ;
#19530=CARTESIAN_POINT ( 'NONE',  ( -20.08610463437157989, 32.20000000546238539, -27.64615127144129758 ) ) ;
#19531=EDGE_CURVE ( 'NONE', #29552, #8544, #21428, .T. ) ;
#19532=CARTESIAN_POINT ( 'NONE',  ( -10.04305231718578462, 74.40000000000001990, 30.90933677959249337 ) ) ;
#19534=CARTESIAN_POINT ( 'NONE',  ( 26.29305231718579350, 37.30000000546237970, 19.10302069950537529 ) ) ;
#19536=CARTESIAN_POINT ( 'NONE',  ( -33.58253175000000113, 35.27500000273120406, -10.91162601494193218 ) ) ;
#19540=CARTESIAN_POINT ( 'NONE',  ( 23.41746825000000243, 9.024999997268826846, 7.608796670333735079 ) ) ;
#19541=CARTESIAN_POINT ( 'NONE',  ( -20.08610463437157989, 11.70000000000000995, -27.64615127144129758 ) ) ;
#19544=CARTESIAN_POINT ( 'NONE',  ( 6.486482029760649416E-15, 55.62500000273119838, 35.31076352940723240 ) ) ;
#19545=CARTESIAN_POINT ( 'NONE',  ( -2.162160676586882350E-15, 44.87500000273119127, -35.31076352940722529 ) ) ;
#19547=CARTESIAN_POINT ( 'NONE',  ( 32.50000000000000000, 67.50000000546238255, -3.980102097228898626E-15 ) ) ;
#19548=CARTESIAN_POINT ( 'NONE',  ( -20.75514604977248112, 7.425000002731177773, 28.56700777964554661 ) ) ;
#19551=DIRECTION ( 'NONE',  ( 0.000000000000000000, 0.000000000000000000, -1.000000000000000000 ) ) ;
#19555=CARTESIAN_POINT ( 'NONE',  ( 5.779280353836490358E-15, 48.50000000000000000, 32.49999999999999289 ) ) ;
#19556=CARTESIAN_POINT ( 'NONE',  ( 15.14183272437242422, 14.29999999999998472, -20.84094480462497856 ) ) ;
#19560=CARTESIAN_POINT ( 'NONE',  ( -33.58253175000000113, 33.12500000273119127, 0.000000000000000000 ) ) ;
#19563=VECTOR ( 'NONE', #26383, 1000.000000000000000 ) ;
#19569=VECTOR ( 'NONE', #10031, 1000.000000000000000 ) ;
#19571=CARTESIAN_POINT ( 'NONE',  ( 26.29305231718579350, 56.80000000000001847, 19.10302069950537529 ) ) ;
#19572=CARTESIAN_POINT ( 'NONE',  ( 27.16883889988623935, 42.57500000273117990, -19.73931689729374384 ) ) ;
#19573=CARTESIAN_POINT ( 'NONE',  ( -32.50000000000000000, 48.40000000546237402, -10.55989012756945478 ) ) ;
#19575=CARTESIAN_POINT ( 'NONE',  ( 33.58253175000000113, 30.22500000273118559, -10.91162601494193751 ) ) ;
#19577=CARTESIAN_POINT ( 'NONE',  ( -33.58253175000000113, 55.27500000273120406, -10.91162601494193218 ) ) ;
#19579=CARTESIAN_POINT ( 'NONE',  ( -10.04305231718578462, 32.39999999999998437, 30.90933677959249337 ) ) ;
#19581=CARTESIAN_POINT ( 'NONE',  ( 20.75514604977249178, 2.075000002731171467, 28.56700777964553950 ) ) ;
#19582=CARTESIAN_POINT ( 'NONE',  ( 5.779280353836490358E-15, 12.49999999999999112, 32.49999999999999289 ) ) ;
#19584=CARTESIAN_POINT ( 'NONE',  ( -27.16883889988623935, 67.57500000273120122, 19.73931689729374739 ) ) ;
#19585=CARTESIAN_POINT ( 'NONE',  ( 15.14183272437242067, 3.449999994537619852, 20.84094480462498211 ) ) ;
#19586=ORIENTED_EDGE ( 'NONE', *, *, #5804, .F. ) ;
#19587=CARTESIAN_POINT ( 'NONE',  ( 7.570916362186213000, 4.149999994537633796, -23.30088464923126423 ) ) ;
#19597=EDGE_CURVE ( 'NONE', #1732, #31503, #32016, .T. ) ;
#19598=FACE_OUTER_BOUND ( 'NONE', #28050, .T. ) ;
#19601=CARTESIAN_POINT ( 'NONE',  ( -24.50000000000000000, 16.89999999999998792, -7.960532557706207157 ) ) ;
#19602=ORIENTED_EDGE ( 'NONE', *, *, #22567, .T. ) ;
#19606=EDGE_LOOP ( 'NONE', ( #22812, #26325 ) ) ;
#19610=CARTESIAN_POINT ( 'NONE',  ( 26.29305231718579350, 26.79999999999999005, 19.10302069950537529 ) ) ;
#19611=CARTESIAN_POINT ( 'NONE',  ( -20.75514604977248823, 46.82500000273117990, -28.56700777964554305 ) ) ;
#19613=CARTESIAN_POINT ( 'NONE',  ( -20.08610463437157989, 14.20000000546237295, -27.64615127144129758 ) ) ;
#19615=CARTESIAN_POINT ( 'NONE',  ( -23.41746824999999887, 14.02499999726881263, -7.608796670333730638 ) ) ;
#19617=CARTESIAN_POINT ( 'NONE',  ( -10.04305231718579172, 53.60000000000000853, -30.90933677959248982 ) ) ;
#19618=CARTESIAN_POINT ( 'NONE',  ( -33.58253175000000113, 23.37500000273118417, 0.000000000000000000 ) ) ;
#19620=CARTESIAN_POINT ( 'NONE',  ( -8.960552108402742093E-16, 74.37500000273118417, -14.63369212191046387 ) ) ;
#19622=CARTESIAN_POINT ( 'NONE',  ( -32.50000000000000000, 28.60000000546238397, 10.55989012756946366 ) ) ;
#19623=EDGE_CURVE ( 'NONE', #28042, #601, #5965, .T. ) ;
#19627=CARTESIAN_POINT ( 'NONE',  ( -11.25946833292375793, 71.07500000273120122, 8.180482586598737171 ) ) ;
#19632=CARTESIAN_POINT ( 'NONE',  ( -2.162160676586882350E-15, 10.87500000273118417, -35.31076352940722529 ) ) ;
#19637=CARTESIAN_POINT ( 'NONE',  ( 13.91746825000000065, 78.27500000273117564, 4.522059556121115875 ) ) ;
#19640=CARTESIAN_POINT ( 'NONE',  ( 27.16883889988623935, 54.32500000273118701, -19.73931689729374384 ) ) ;
#19643=ORIENTED_EDGE ( 'NONE', *, *, #21344, .F. ) ;
#19645=CARTESIAN_POINT ( 'NONE',  ( -1.778240108872766143E-15, 43.50000000000000000, -32.49999999999999289 ) ) ;
#19646=CARTESIAN_POINT ( 'NONE',  ( 14.47279130897151589, 10.32499999726881335, 19.92008829642072953 ) ) ;
#19650=CARTESIAN_POINT ( 'NONE',  ( 15.14183272437242422, 6.300000000000004263, -20.84094480462497856 ) ) ;
#19653=CARTESIAN_POINT ( 'NONE',  ( -10.37757302488623701, 57.77500000273119696, 31.93888565452638417 ) ) ;
#19654=CARTESIAN_POINT ( 'NONE',  ( 32.50000000000000711, 69.40000000546237402, 10.55989012756945122 ) ) ;
#19655=CARTESIAN_POINT ( 'NONE',  ( -27.16883889988624290, 76.92500000273119554, -19.73931689729374028 ) ) ;
#19657=CARTESIAN_POINT ( 'NONE',  ( -24.50000000000000000, 3.000000000000002665, -3.000384657911015469E-15 ) ) ;
#19658=CYLINDRICAL_SURFACE ( 'NONE', #13877, 32.50000000000000000 ) ;
#19659=CARTESIAN_POINT ( 'NONE',  ( 27.16883889988624290, 15.92500000273117067, 19.73931689729373673 ) ) ;
#19660=CARTESIAN_POINT ( 'NONE',  ( -4.300734207923759378, 74.47500000273119269, -13.23629886949340495 ) ) ;
#19662=CARTESIAN_POINT ( 'NONE',  ( -4.300734207923755825, 71.77500000273117564, 13.23629886949340673 ) ) ;
#19664=CARTESIAN_POINT ( 'NONE',  ( 3.445340210940985210E-14, 9.249999994537636994, 24.50000000000000000 ) ) ;
#19666=CARTESIAN_POINT ( 'NONE',  ( 9.270509831248423538, 75.55000000546239391, -12.75976212528059861 ) ) ;
#19668=CARTESIAN_POINT ( 'NONE',  ( 6.486482029760649416E-15, 35.62500000273119127, 35.31076352940723240 ) ) ;
#19671=CARTESIAN_POINT ( 'NONE',  ( 20.75514604977249178, 28.07500000273119412, 28.56700777964553950 ) ) ;
#19674=CARTESIAN_POINT ( 'NONE',  ( -10.04305231718579172, 17.60000000000000497, -30.90933677959248982 ) ) ;
#19677=CARTESIAN_POINT ( 'NONE',  ( 18.94512977948575738, 12.42499999726881477, 13.76444248337723408 ) ) ;
#19682=CARTESIAN_POINT ( 'NONE',  ( 33.58253175000000113, 14.12500000273120193, -4.112674001490185761E-15 ) ) ;
#19683=CARTESIAN_POINT ( 'NONE',  ( 23.41746825000000243, 5.224999997268802154, -7.608796670333727974 ) ) ;
#19688=VERTEX_POINT ( 'NONE', #32535 ) ;
#19692=CARTESIAN_POINT ( 'NONE',  ( 7.570916362186207671, 15.34999999453762243, 23.30088464923126779 ) ) ;
#19693=CARTESIAN_POINT ( 'NONE',  ( -4.523095164977116484E-15, 6.124999997268802510, 24.62258325217400312 ) ) ;
#19694=CARTESIAN_POINT ( 'NONE',  ( -33.58253175000000113, 21.47500000273119980, 10.91162601494193929 ) ) ;
#19695=CARTESIAN_POINT ( 'NONE',  ( 6.277390505771533514E-15, 25.00000000546238255, 34.17252228774368916 ) ) ;
#19697=CARTESIAN_POINT ( 'NONE',  ( -20.08610463437156923, 74.30000000000001137, 27.64615127144130113 ) ) ;
#19698=CARTESIAN_POINT ( 'NONE',  ( 3.980102097228898626E-15, 80.00000000000001421, 32.50000000000000000 ) ) ;
#19701=CARTESIAN_POINT ( 'NONE',  ( 33.58253175000000823, 36.27500000273119696, 10.91162601494192863 ) ) ;
#19704=CARTESIAN_POINT ( 'NONE',  ( 7.236395654485755280, 12.72499999726881015, 22.27133577429736988 ) ) ;
#19705=CARTESIAN_POINT ( 'NONE',  ( -32.50000000000000000, 17.89999999999998437, -10.55989012756945478 ) ) ;
#19706=CARTESIAN_POINT ( 'NONE',  ( -1.778240108872766143E-15, 51.50000000000000711, -32.49999999999999289 ) ) ;
#19708=CARTESIAN_POINT ( 'NONE',  ( -10.37757302488624411, 56.72500000273117138, -31.93888565452638417 ) ) ;
#19709=CARTESIAN_POINT ( 'NONE',  ( 20.75514604977249178, 50.07500000273120122, 28.56700777964553950 ) ) ;
#19711=DIRECTION ( 'NONE',  ( 0.000000000000000000, 0.000000000000000000, 1.000000000000000000 ) ) ;
#19712=CARTESIAN_POINT ( 'NONE',  ( -10.04305231718579172, 5.599999999999994316, -30.90933677959248982 ) ) ;
#19719=CARTESIAN_POINT ( 'NONE',  ( 20.08610463437157279, 41.80000000546237260, -27.64615127144129758 ) ) ;
#19723=CARTESIAN_POINT ( 'NONE',  ( 32.50000000000000000, 35.00000000000000000, -3.980102097228898626E-15 ) ) ;
#19724=CARTESIAN_POINT ( 'NONE',  ( -33.58253175000000113, 35.22500000273120691, 10.91162601494193929 ) ) ;
#19727=ORIENTED_EDGE ( 'NONE', *, *, #21954, .F. ) ;
#19731=DIRECTION ( 'NONE',  ( -0.000000000000000000, 1.000000000000000000, -0.000000000000000000 ) ) ;
#19732=ORIENTED_EDGE ( 'NONE', *, *, #20285, .F. ) ;
#19736=DIRECTION ( 'NONE',  ( -0.000000000000000000, -1.000000000000000000, -0.000000000000000000 ) ) ;
#19737=CARTESIAN_POINT ( 'NONE',  ( -33.58253175000000113, 41.37500000273119838, 0.000000000000000000 ) ) ;
#19738=CARTESIAN_POINT ( 'NONE',  ( -20.08610463437156923, 46.80000000546235839, 27.64615127144130113 ) ) ;
#19740=CARTESIAN_POINT ( 'NONE',  ( -33.58253175000000113, 27.22500000273119269, 10.91162601494193929 ) ) ;
#19741=CARTESIAN_POINT ( 'NONE',  ( 32.50000000000000000, 31.60000000546237686, -10.55989012756945833 ) ) ;
#19742=CARTESIAN_POINT ( 'NONE',  ( -33.58253175000000113, 53.47500000273117848, 10.91162601494193929 ) ) ;
#19744=CARTESIAN_POINT ( 'NONE',  ( 20.08610463437158344, 36.70000000000000995, 27.64615127144129403 ) ) ;
#19746=CARTESIAN_POINT ( 'NONE',  ( -33.58253175000000113, 73.12500000273119838, 0.000000000000000000 ) ) ;
#19747=CARTESIAN_POINT ( 'NONE',  ( 26.29305231718578995, 13.19999999999998863, -19.10302069950538240 ) ) ;
#19749=CARTESIAN_POINT ( 'NONE',  ( -10.37757302488623701, 63.77500000273117564, 31.93888565452638417 ) ) ;
#19752=CARTESIAN_POINT ( 'NONE',  ( 19.82091636218621389, 5.949999994537630066, -14.40073868116559197 ) ) ;
#19765=CARTESIAN_POINT ( 'NONE',  ( -19.82091636218621389, 4.949999994537629178, 14.40073868116558842 ) ) ;
#19766=VERTEX_POINT ( 'NONE', #30638 ) ;
#19773=CARTESIAN_POINT ( 'NONE',  ( 5.779280353836490358E-15, 26.50000000000000711, 32.49999999999999289 ) ) ;
#19775=CARTESIAN_POINT ( 'NONE',  ( 20.75514604977249178, 47.82500000273117990, 28.56700777964553950 ) ) ;
#19777=CARTESIAN_POINT ( 'NONE',  ( 10.04305231718579705, 13.10000000546238041, 30.90933677959248982 ) ) ;
#19778=CARTESIAN_POINT ( 'NONE',  ( -9.270509831248423538, 77.70000000000001705, -12.75976212528059861 ) ) ;
#19779=CARTESIAN_POINT ( 'NONE',  ( -23.41746825000000243, 16.22499999726880304, 7.608796670333725309 ) ) ;
#19780=CARTESIAN_POINT ( 'NONE',  ( 20.08610463437157279, 55.29999999999999716, -27.64615127144129758 ) ) ;
#19781=CARTESIAN_POINT ( 'NONE',  ( 33.58253175000000113, 14.47500000273118737, -10.91162601494193751 ) ) ;
#19784=CARTESIAN_POINT ( 'NONE',  ( 2.688165632520823219E-15, 73.37500000273118417, 14.63369212191046387 ) ) ;
#19785=DIRECTION ( 'NONE',  ( 0.000000000000000000, 0.000000000000000000, 1.000000000000000000 ) ) ;
#19788=ORIENTED_EDGE ( 'NONE', *, *, #29081, .T. ) ;
#19790=CARTESIAN_POINT ( 'NONE',  ( 13.91746824999999887, 71.87500000273119838, -1.704398294459741270E-15 ) ) ;
#19796=CARTESIAN_POINT ( 'NONE',  ( 33.58253175000000113, 8.375000002731169957, -4.112674001490185761E-15 ) ) ;
#19799=CARTESIAN_POINT ( 'NONE',  ( 4.300734207923757602, 72.77500000273118985, -13.23629886949340673 ) ) ;
#19802=AXIS2_PLACEMENT_3D ( 'NONE', #7105, #25305, #30092 ) ;
#19803=CARTESIAN_POINT ( 'NONE',  ( 6.001560367445586717E-15, 3.249999994537631665, 24.50000000000000000 ) ) ;
#19804=CARTESIAN_POINT ( 'NONE',  ( -33.58253175000000113, 49.12500000273117706, 0.000000000000000000 ) ) ;
#19808=CARTESIAN_POINT ( 'NONE',  ( 5.779280353836490358E-15, 2.500000000000005329, 32.49999999999999289 ) ) ;
#19809=CARTESIAN_POINT ( 'NONE',  ( 23.41746825000000243, 10.52499999726880731, 7.608796670333735079 ) ) ;
#19813=CARTESIAN_POINT ( 'NONE',  ( -32.50000000000000000, 34.50000000546238255, 0.000000000000000000 ) ) ;
#19814=ORIENTED_EDGE ( 'NONE', *, *, #18037, .T. ) ;
#19816=CARTESIAN_POINT ( 'NONE',  ( 20.75514604977248467, 62.67500000273117422, -28.56700777964554305 ) ) ;
#19817=CARTESIAN_POINT ( 'NONE',  ( -20.08610463437156923, 36.80000000546239391, 27.64615127144130113 ) ) ;
#19818=CARTESIAN_POINT ( 'NONE',  ( 33.58253175000000823, 68.02500000273117564, 10.91162601494192863 ) ) ;
#19820=CARTESIAN_POINT ( 'NONE',  ( -4.732186688966233175E-15, 11.49999999999998579, 25.76082449383753925 ) ) ;
#19821=CARTESIAN_POINT ( 'NONE',  ( 10.37757302488624056, 4.775000002731177418, -31.93888565452638417 ) ) ;
#19822=CARTESIAN_POINT ( 'NONE',  ( -10.37757302488623701, 7.525000002731207616, 31.93888565452638417 ) ) ;
#19825=CARTESIAN_POINT ( 'NONE',  ( 2.897257156509938333E-15, 78.49999999999998579, 15.77193336357400710 ) ) ;
#19829=CARTESIAN_POINT ( 'NONE',  ( -9.657523855033125146E-16, 79.75000000546236834, -15.77193336357400710 ) ) ;
#19831=CARTESIAN_POINT ( 'NONE',  ( 27.16883889988623935, 40.32500000273120122, -19.73931689729374384 ) ) ;
#19834=CARTESIAN_POINT ( 'NONE',  ( -20.75514604977248823, 31.07500000273118701, -28.56700777964554305 ) ) ;
#19836=CARTESIAN_POINT ( 'NONE',  ( 0.000000000000000000, 70.00000000000000000, 0.000000000000000000 ) ) ;
#19837=CARTESIAN_POINT ( 'NONE',  ( 5.779280353836490358E-15, 27.00000000546237544, 32.49999999999999289 ) ) ;
#19839=CARTESIAN_POINT ( 'NONE',  ( 7.236395654485760609, 9.024999997268800200, -22.27133577429736633 ) ) ;
#19845=CARTESIAN_POINT ( 'NONE',  ( -27.16883889988624290, 12.92500000273116889, -19.73931689729374028 ) ) ;
#19846=CARTESIAN_POINT ( 'NONE',  ( 18.94512977948575738, 14.92499999726881654, 13.76444248337723408 ) ) ;
#19848=ORIENTED_EDGE ( 'NONE', *, *, #8117, .T. ) ;
#19851=VERTEX_POINT ( 'NONE', #23916 ) ;
#19855=CARTESIAN_POINT ( 'NONE',  ( -24.50000000000001066, 14.84999999453764019, 7.960532557706201828 ) ) ;
#19857=CARTESIAN_POINT ( 'NONE',  ( 14.47279130897151767, 8.924999997268800556, -19.92008829642072598 ) ) ;
#19858=CARTESIAN_POINT ( 'NONE',  ( -27.16883889988624290, 25.17500000273117777, -19.73931689729374028 ) ) ;
#19859=CARTESIAN_POINT ( 'NONE',  ( -10.04305231718579172, 24.10000000546236265, -30.90933677959248982 ) ) ;
#19860=AXIS2_PLACEMENT_3D ( 'NONE', #27775, #11817, #32738 ) ;
#19861=CARTESIAN_POINT ( 'NONE',  ( -26.29305231718578995, 70.19999999999998863, 19.10302069950538595 ) ) ;
#19862=CARTESIAN_POINT ( 'NONE',  ( -32.50000000000000000, 6.600000005462382191, 10.55989012756946366 ) ) ;
#19865=CARTESIAN_POINT ( 'NONE',  ( -27.16883889988624290, 35.17500000273118843, -19.73931689729374028 ) ) ;
#19869=CIRCLE ( 'NONE', #27535, 15.00000000000000000 ) ;
#19870=CARTESIAN_POINT ( 'NONE',  ( 23.41746824999999887, 13.12499999726882116, 0.000000000000000000 ) ) ;
#19871=CARTESIAN_POINT ( 'NONE',  ( -26.29305231718579350, 13.79999999999997939, -19.10302069950537884 ) ) ;
#19874=CARTESIAN_POINT ( 'NONE',  ( -20.75514604977248823, 56.82500000273117990, -28.56700777964554305 ) ) ;
#19875=CARTESIAN_POINT ( 'NONE',  ( 27.16883889988623935, 48.57500000273118701, -19.73931689729374384 ) ) ;
#19876=CARTESIAN_POINT ( 'NONE',  ( 26.29305231718579350, 44.80000000000000426, 19.10302069950537529 ) ) ;
#19877=CARTESIAN_POINT ( 'NONE',  ( 20.08610463437158344, 67.20000000546235697, 27.64615127144129403 ) ) ;
#19878=CARTESIAN_POINT ( 'NONE',  ( -10.04305231718578462, 6.400000000000016342, 30.90933677959249337 ) ) ;
#19885=CARTESIAN_POINT ( 'NONE',  ( 0.000000000000000000, 80.00000000000001421, -32.50000000000000000 ) ) ;
#19888=CARTESIAN_POINT ( 'NONE',  ( -20.08610463437157989, 60.20000000546237828, -27.64615127144129758 ) ) ;
#19890=CARTESIAN_POINT ( 'NONE',  ( -27.16883889988623935, 29.32500000273119412, 19.73931689729374739 ) ) ;
#19891=CARTESIAN_POINT ( 'NONE',  ( -2.162160676586881955E-15, 64.87500000273119838, -35.31076352940723240 ) ) ;
#19893=ORIENTED_EDGE ( 'NONE', *, *, #8508, .T. ) ;
#19894=AXIS2_PLACEMENT_3D ( 'NONE', #12789, #33725, #7469 ) ;
#19897=( BOUNDED_CURVE ( )  B_SPLINE_CURVE ( 2, ( #15577, #23631, #21398, #10757, #10587, #7834, #13508, #5092, #8008, #3035, #21064, #29270, #31678 ),
 .UNSPECIFIED., .F., .T. ) 
 B_SPLINE_CURVE_WITH_KNOTS ( ( 3, 2, 2, 2, 2, 2, 3 ),
 ( 0.6474358974358974672, 0.6487179487179487447, 0.6512820512820512997, 0.6538461538461538547, 0.6564102564102564097, 0.6589743589743589647, 0.6602564102564102422 ),
 .UNSPECIFIED. ) 
 CURVE ( )  GEOMETRIC_REPRESENTATION_ITEM ( )  RATIONAL_B_SPLINE_CURVE ( ( 0.9755282581475768211, 0.9755282581475768211, 1.000000000000000000, 0.9510565162951535312, 1.000000000000000000, 0.9510565162951535312, 1.000000000000000000, 0.9510565162951535312, 1.000000000000000000, 0.9510565162951535312, 1.000000000000000000, 0.9755282581475768211, 0.9755282581475768211 ) ) 
 REPRESENTATION_ITEM ( '' )  );
#19899=VERTEX_POINT ( 'NONE', #30047 ) ;
#19904=CARTESIAN_POINT ( 'NONE',  ( -32.50000000000000000, 64.50000000546238255, 0.000000000000000000 ) ) ;
#19905=CARTESIAN_POINT ( 'NONE',  ( -27.16883889988624290, 41.17500000273119554, -19.73931689729374028 ) ) ;
#19906=CARTESIAN_POINT ( 'NONE',  ( -20.08610463437156923, 42.80000000546236549, 27.64615127144130113 ) ) ;
#19908=CARTESIAN_POINT ( 'NONE',  ( 10.37757302488624056, 32.52500000273117564, -31.93888565452638417 ) ) ;
#19909=CARTESIAN_POINT ( 'NONE',  ( -10.04305231718578462, 24.40000000000000568, 30.90933677959249337 ) ) ;
#19910=CARTESIAN_POINT ( 'NONE',  ( -10.37757302488624411, 54.97500000273119980, -31.93888565452638417 ) ) ;
#19913=CARTESIAN_POINT ( 'NONE',  ( -26.29305231718579350, 31.79999999999999361, -19.10302069950537884 ) ) ;
#19915=EDGE_CURVE ( 'NONE', #5805, #28550, #41, .T. ) ;
#19916=CARTESIAN_POINT ( 'NONE',  ( -20.75514604977248823, 78.82500000273120122, -28.56700777964554305 ) ) ;
#19917=DIRECTION ( 'NONE',  ( 0.000000000000000000, 0.000000000000000000, 1.000000000000000000 ) ) ;
#19919=CARTESIAN_POINT ( 'NONE',  ( -10.37757302488624411, 68.97500000273117848, -31.93888565452638417 ) ) ;
#19921=ADVANCED_FACE ( 'NONE', ( #24737 ), #6716, .F. ) ;
#19923=ORIENTED_EDGE ( 'NONE', *, *, #755, .T. ) ;
#19924=CARTESIAN_POINT ( 'NONE',  ( -19.82091636218621034, 12.54999999453762527, -14.40073868116559552 ) ) ;
#19926=LINE ( 'NONE', #4300, #11858 ) ;
#19936=CARTESIAN_POINT ( 'NONE',  ( -10.04305231718579172, 74.10000000546237686, -30.90933677959248982 ) ) ;
#19940=VERTEX_POINT ( 'NONE', #6883 ) ;
#19946=CARTESIAN_POINT ( 'NONE',  ( -32.50000000000000000, 62.40000000546235981, -10.55989012756945478 ) ) ;
#19947=VERTEX_POINT ( 'NONE', #14618 ) ;
#19948=CARTESIAN_POINT ( 'NONE',  ( -32.50000000000000000, 74.50000000546236834, 0.000000000000000000 ) ) ;
#19949=CARTESIAN_POINT ( 'NONE',  ( 20.75514604977249178, 45.82500000273118701, 28.56700777964553950 ) ) ;
#19950=CARTESIAN_POINT ( 'NONE',  ( 5.147494310547434893, 55.05125428700924317, 32.49999999999999289 ) ) ;
#19951=CARTESIAN_POINT ( 'NONE',  ( -1.778240108872766143E-15, 47.49999999999999289, -32.49999999999999289 ) ) ;
#19952=CARTESIAN_POINT ( 'NONE',  ( 10.04305231718578817, 9.900000005462372243, -30.90933677959249337 ) ) ;
#19954=CARTESIAN_POINT ( 'NONE',  ( 7.236395654485755280, 14.72499999726881192, 22.27133577429736988 ) ) ;
#19955=CARTESIAN_POINT ( 'NONE',  ( 32.50000000000000000, 53.09999999999998721, -10.55989012756945833 ) ) ;
#19958=CARTESIAN_POINT ( 'NONE',  ( 10.37757302488624056, 18.77500000273118985, -31.93888565452638417 ) ) ;
#19959=CARTESIAN_POINT ( 'NONE',  ( -32.50000000000000000, 74.00000000000001421, 0.000000000000000000 ) ) ;
#19961=CARTESIAN_POINT ( 'NONE',  ( 4.300734207923761154, 75.47500000273119269, 13.23629886949340495 ) ) ;
#19962=CYLINDRICAL_SURFACE ( 'NONE', #14045, 24.50000000000000000 ) ;
#19963=CARTESIAN_POINT ( 'NONE',  ( -32.50000000000000000, 43.90000000000001279, -10.55989012756945300 ) ) ;
#19964=EDGE_CURVE ( 'NONE', #22660, #3077, #30557, .T. ) ;
#19966=ORIENTED_EDGE ( 'NONE', *, *, #19034, .T. ) ;
#19968=LINE ( 'NONE', #30414, #11789 ) ;
#19973=CYLINDRICAL_SURFACE ( 'NONE', #22078, 32.50000000000000000 ) ;
#19977=CARTESIAN_POINT ( 'NONE',  ( 5.147494310547426899, 69.44874571845315359, -32.50000000000000000 ) ) ;
#19979=CARTESIAN_POINT ( 'NONE',  ( -33.58253175000000113, 53.02500000273118985, -10.91162601494193041 ) ) ;
#19982=ORIENTED_EDGE ( 'NONE', *, *, #27320, .T. ) ;
#19984=CARTESIAN_POINT ( 'NONE',  ( 5.779280353836490358E-15, 16.50000000000000000, 32.49999999999999289 ) ) ;
#19985=CARTESIAN_POINT ( 'NONE',  ( 1.507698388325705758E-15, 11.12499999726881761, -24.62258325217400312 ) ) ;
#19989=CARTESIAN_POINT ( 'NONE',  ( -10.04305231718579172, 34.10000000546236976, -30.90933677959248982 ) ) ;
#19994=CARTESIAN_POINT ( 'NONE',  ( -10.37757302488623701, 67.52500000273120406, 31.93888565452638417 ) ) ;
#19996=CARTESIAN_POINT ( 'NONE',  ( -7.570916362186215665, 11.39999999999999325, 23.30088464923126423 ) ) ;
#19997=CARTESIAN_POINT ( 'NONE',  ( -10.37757302488623701, 5.775000002731179194, 31.93888565452638417 ) ) ;
#19998=CARTESIAN_POINT ( 'NONE',  ( -10.37757302488624411, 12.72500000273119092, -31.93888565452638417 ) ) ;
#19999=( BOUNDED_CURVE ( )  B_SPLINE_CURVE ( 2, ( #18580, #24057, #26290, #13244, #18746, #10843, #28855, #7589, #7924, #2779, #525, #21152, #359 ),
 .UNSPECIFIED., .F., .T. ) 
 B_SPLINE_CURVE_WITH_KNOTS ( ( 3, 2, 2, 2, 2, 2, 3 ),
 ( 0.3141025641025640969, 0.3153846153846153744, 0.3179487179487179294, 0.3205128205128205399, 0.3230769230769230949, 0.3256410256410256499, 0.3269230769230769273 ),
 .UNSPECIFIED. ) 
 CURVE ( )  GEOMETRIC_REPRESENTATION_ITEM ( )  RATIONAL_B_SPLINE_CURVE ( ( 0.9755282581475768211, 0.9755282581475768211, 1.000000000000000000, 0.9510565162951535312, 1.000000000000000000, 0.9510565162951535312, 1.000000000000000000, 0.9510565162951535312, 1.000000000000000000, 0.9510565162951535312, 1.000000000000000000, 0.9755282581475768211, 0.9755282581475768211 ) ) 
 REPRESENTATION_ITEM ( '' )  );
#20000=CARTESIAN_POINT ( 'NONE',  ( -13.91746824999999532, 70.97500000273117848, 4.522059556121122093 ) ) ;
#20002=CARTESIAN_POINT ( 'NONE',  ( -12.13525491562420910, 72.19999999999998863, 8.816778784387098611 ) ) ;
#20005=CARTESIAN_POINT ( 'NONE',  ( 32.50000000000000000, 61.60000000546236265, -10.55989012756945833 ) ) ;
#20007=CARTESIAN_POINT ( 'NONE',  ( 2.897257156509938333E-15, 74.75000000546235412, 15.77193336357400710 ) ) ;
#20009=CARTESIAN_POINT ( 'NONE',  ( -33.58253175000000113, 37.02500000273117564, -10.91162601494193218 ) ) ;
#20012=CARTESIAN_POINT ( 'NONE',  ( 10.37757302488624056, 24.77500000273119696, -31.93888565452638417 ) ) ;
#20014=CARTESIAN_POINT ( 'NONE',  ( -5.147494310547430452, 8.051254287009218302, -32.49999999999999289 ) ) ;
#20016=CARTESIAN_POINT ( 'NONE',  ( 10.04305231718578817, 33.39999999999998437, -30.90933677959249337 ) ) ;
#20018=CARTESIAN_POINT ( 'NONE',  ( -14.47279130897151767, 9.324999997268816898, -19.92008829642072598 ) ) ;
#20023=CARTESIAN_POINT ( 'NONE',  ( -2.162160676586882350E-15, 10.62500000273119483, -35.31076352940722529 ) ) ;
#20024=CARTESIAN_POINT ( 'NONE',  ( 23.41746825000000243, 13.22499999726881192, -7.608796670333727974 ) ) ;
#20026=ORIENTED_EDGE ( 'NONE', *, *, #7791, .T. ) ;
#20033=CARTESIAN_POINT ( 'NONE',  ( -7.570916362186215665, 15.14999999453761603, 23.30088464923126423 ) ) ;
#20034=CARTESIAN_POINT ( 'NONE',  ( 7.236395654485755280, 10.22499999726880837, 22.27133577429736988 ) ) ;
#20035=CARTESIAN_POINT ( 'NONE',  ( 6.486482029760649416E-15, 21.87500000273118062, 35.31076352940723240 ) ) ;
#20037=CARTESIAN_POINT ( 'NONE',  ( 10.04305231718579705, 25.10000000546236265, 30.90933677959248982 ) ) ;
#20038=CARTESIAN_POINT ( 'NONE',  ( 26.29305231718579350, 66.79999999999999716, 19.10302069950537529 ) ) ;
#20039=CARTESIAN_POINT ( 'NONE',  ( 10.04305231718579705, 47.10000000546238397, 30.90933677959248982 ) ) ;
#20042=CARTESIAN_POINT ( 'NONE',  ( 6.486482029760649416E-15, 37.87500000273117706, 35.31076352940723240 ) ) ;
#20043=CYLINDRICAL_SURFACE ( 'NONE', #5394, 32.50000000000000000 ) ;
#20046=CARTESIAN_POINT ( 'NONE',  ( -23.41746825000000598, 14.22499999726880660, 7.608796670333726198 ) ) ;
#20047=CARTESIAN_POINT ( 'NONE',  ( 32.50000000000000000, 17.10000000000001208, -10.55989012756945833 ) ) ;
#20049=CARTESIAN_POINT ( 'NONE',  ( -10.37757302488623701, 57.52500000273119696, 31.93888565452638417 ) ) ;
#20052=CARTESIAN_POINT ( 'NONE',  ( 10.37757302488624767, 49.97500000273119269, 31.93888565452638417 ) ) ;
#20053=CARTESIAN_POINT ( 'NONE',  ( 5.779280353836490358E-15, 44.49999999999999289, 32.49999999999999289 ) ) ;
#20054=ADVANCED_FACE ( 'NONE', ( #22006 ), #1212, .F. ) ;
#20067=CARTESIAN_POINT ( 'NONE',  ( -26.29305231718578995, 60.70000000546238539, 19.10302069950538595 ) ) ;
#20068=CARTESIAN_POINT ( 'NONE',  ( -20.75514604977248112, 35.42500000273119554, 28.56700777964554661 ) ) ;
#20069=CARTESIAN_POINT ( 'NONE',  ( 20.75514604977249178, 66.07500000273118701, 28.56700777964553950 ) ) ;
#20071=ORIENTED_EDGE ( 'NONE', *, *, #17349, .F. ) ;
#20075=CARTESIAN_POINT ( 'NONE',  ( -26.29305231718578995, 16.70000000546237473, 19.10302069950538595 ) ) ;
#20079=VECTOR ( 'NONE', #12404, 1000.000000000000000 ) ;
#20082=CARTESIAN_POINT ( 'NONE',  ( -32.50000000000000000, 45.99999999999998579, 0.000000000000000000 ) ) ;
#20083=CARTESIAN_POINT ( 'NONE',  ( -20.75514604977248823, 43.07500000273118701, -28.56700777964554305 ) ) ;
#20084=CARTESIAN_POINT ( 'NONE',  ( 6.277390505771533514E-15, 47.00000000546238965, 34.17252228774368916 ) ) ;
#20086=CARTESIAN_POINT ( 'NONE',  ( 33.58253175000000113, 26.22500000273119625, -10.91162601494193751 ) ) ;
#20088=CARTESIAN_POINT ( 'NONE',  ( 27.16883889988623935, 58.57500000273119412, -19.73931689729374384 ) ) ;
#20090=CARTESIAN_POINT ( 'NONE',  ( 32.50000000000000711, 30.89999999999998437, 10.55989012756945122 ) ) ;
#20092=CARTESIAN_POINT ( 'NONE',  ( 6.486482029760649416E-15, 75.62500000273121259, 35.31076352940723240 ) ) ;
#20094=CARTESIAN_POINT ( 'NONE',  ( -32.50000000000000000, 20.60000000546237686, 10.55989012756946366 ) ) ;
#20095=CARTESIAN_POINT ( 'NONE',  ( 27.16883889988623935, 66.57500000273120122, -19.73931689729374384 ) ) ;
#20098=CARTESIAN_POINT ( 'NONE',  ( 33.58253175000000113, 16.22500000273118914, -10.91162601494193751 ) ) ;
#20099=CARTESIAN_POINT ( 'NONE',  ( 1.577395562988744260E-15, 8.249999994537613901, -25.76082449383753925 ) ) ;
#20101=CARTESIAN_POINT ( 'NONE',  ( 3.445340210940985210E-14, 7.249999994537621895, 24.50000000000000000 ) ) ;
#20106=CIRCLE ( 'NONE', #8048, 32.50000000000000000 ) ;
#20110=( BOUNDED_CURVE ( )  B_SPLINE_CURVE ( 2, ( #11095, #18992, #18491, #18825, #19156, #440, #29436, #2694, #28934, #603, #268, #13154, #3204 ),
 .UNSPECIFIED., .F., .T. ) 
 B_SPLINE_CURVE_WITH_KNOTS ( ( 3, 2, 2, 2, 2, 2, 3 ),
 ( 0.8525641025641025328, 0.8538461538461538103, 0.8564102564102563653, 0.8589743589743589203, 0.8615384615384615863, 0.8641025641025641413, 0.8653846153846154188 ),
 .UNSPECIFIED. ) 
 CURVE ( )  GEOMETRIC_REPRESENTATION_ITEM ( )  RATIONAL_B_SPLINE_CURVE ( ( 0.9755282581475768211, 0.9755282581475768211, 1.000000000000000000, 0.9510565162951535312, 1.000000000000000000, 0.9510565162951535312, 1.000000000000000000, 0.9510565162951535312, 1.000000000000000000, 0.9510565162951535312, 1.000000000000000000, 0.9755282581475768211, 0.9755282581475768211 ) ) 
 REPRESENTATION_ITEM ( '' )  );
#20112=DIRECTION ( 'NONE',  ( -0.000000000000000000, -1.000000000000000000, -0.000000000000000000 ) ) ;
#20113=CARTESIAN_POINT ( 'NONE',  ( 26.29305231718578995, 75.70000000546239960, -19.10302069950538240 ) ) ;
#20115=EDGE_CURVE ( 'NONE', #23284, #19851, #27996, .T. ) ;
#20119=CARTESIAN_POINT ( 'NONE',  ( -20.75514604977248823, 77.07500000273117280, -28.56700777964554305 ) ) ;
#20123=CARTESIAN_POINT ( 'NONE',  ( -10.04305231718578462, 64.90000000546235981, 30.90933677959249337 ) ) ;
#20125=CARTESIAN_POINT ( 'NONE',  ( -32.50000000000000000, 74.60000000546234844, 10.55989012756946366 ) ) ;
#20126=CARTESIAN_POINT ( 'NONE',  ( -33.58253175000000113, 51.12500000273117706, 0.000000000000000000 ) ) ;
#20127=CARTESIAN_POINT ( 'NONE',  ( 9.270509831248421762, 73.55000000546237970, -12.75976212528059861 ) ) ;
#20128=CARTESIAN_POINT ( 'NONE',  ( 26.29305231718579350, 5.300000005462379704, 19.10302069950537529 ) ) ;
#20129=CARTESIAN_POINT ( 'NONE',  ( -20.08610463437156923, 8.300000000000000711, 27.64615127144130113 ) ) ;
#20131=CARTESIAN_POINT ( 'NONE',  ( -32.50000000000000000, 52.10000000000001563, 10.55989012756946366 ) ) ;
#20132=CARTESIAN_POINT ( 'NONE',  ( -32.50000000000000000, 14.09999999999999076, 10.55989012756946366 ) ) ;
#20133=CARTESIAN_POINT ( 'NONE',  ( -20.75514604977248823, 19.07500000273118701, -28.56700777964554305 ) ) ;
#20136=CARTESIAN_POINT ( 'NONE',  ( 8.601468415847516980, 76.67500000273116711, -11.83890561707634781 ) ) ;
#20138=CARTESIAN_POINT ( 'NONE',  ( 26.29305231718578995, 53.70000000546237828, -19.10302069950538240 ) ) ;
#20143=CARTESIAN_POINT ( 'NONE',  ( -13.91746824999999887, 70.87500000273119838, 0.000000000000000000 ) ) ;
#20148=DIRECTION ( 'NONE',  ( -0.000000000000000000, -1.000000000000000000, -0.000000000000000000 ) ) ;
#20152=CARTESIAN_POINT ( 'NONE',  ( 5.779280353836490358E-15, 68.49999999999998579, 32.49999999999999289 ) ) ;
#20154=CARTESIAN_POINT ( 'NONE',  ( -33.58253175000000113, 47.12500000273117706, 0.000000000000000000 ) ) ;
#20156=CARTESIAN_POINT ( 'NONE',  ( 32.50000000000000000, 21.50000000546237189, -3.980102097228898626E-15 ) ) ;
#20158=ADVANCED_FACE ( 'NONE', ( #1045 ), #11525, .T. ) ;
#20160=CARTESIAN_POINT ( 'NONE',  ( 26.29305231718578995, 43.20000000000001705, -19.10302069950538240 ) ) ;
#20161=CARTESIAN_POINT ( 'NONE',  ( -14.47279130897151589, 13.32499999726880624, -19.92008829642072598 ) ) ;
#20166=CARTESIAN_POINT ( 'NONE',  ( -13.91746824999999887, 81.12500000273121259, 0.000000000000000000 ) ) ;
#20167=ORIENTED_EDGE ( 'NONE', *, *, #32298, .F. ) ;
#20168=CARTESIAN_POINT ( 'NONE',  ( -1.778240108872766143E-15, 36.00000000546238255, -32.49999999999999289 ) ) ;
#20169=CARTESIAN_POINT ( 'NONE',  ( -10.37757302488623701, 69.52500000273120406, 31.93888565452638417 ) ) ;
#20171=CARTESIAN_POINT ( 'NONE',  ( 15.14183272437242245, 10.29999999999999361, -20.84094480462497856 ) ) ;
#20172=CARTESIAN_POINT ( 'NONE',  ( 7.236395654485760609, 1.524999997268822183, -22.27133577429736633 ) ) ;
#20173=CARTESIAN_POINT ( 'NONE',  ( -33.58253175000000113, 13.22500000273119802, 10.91162601494193929 ) ) ;
#20175=CARTESIAN_POINT ( 'NONE',  ( 9.270509831248425314, 74.70000000000000284, 12.75976212528059683 ) ) ;
#20177=CARTESIAN_POINT ( 'NONE',  ( 10.04305231718579705, 19.10000000546238752, 30.90933677959248982 ) ) ;
#20178=CARTESIAN_POINT ( 'NONE',  ( -4.635254915624208216, 74.65000000546240244, 14.26584774442730463 ) ) ;
#20180=CARTESIAN_POINT ( 'NONE',  ( -15.00000000000000000, 74.35000000546237686, 4.873795443493597723 ) ) ;
#20182=CARTESIAN_POINT ( 'NONE',  ( 6.486482029760649416E-15, 39.62500000273117706, 35.31076352940723240 ) ) ;
#20185=CARTESIAN_POINT ( 'NONE',  ( -10.37757302488623701, 21.77500000273119340, 31.93888565452638417 ) ) ;
#20186=CARTESIAN_POINT ( 'NONE',  ( 20.08610463437157279, 41.30000000000000426, -27.64615127144129758 ) ) ;
#20190=CARTESIAN_POINT ( 'NONE',  ( 26.29305231718578995, 33.20000000000000995, -19.10302069950538240 ) ) ;
#20192=CARTESIAN_POINT ( 'NONE',  ( -14.47279130897152299, 9.924999997268827201, 19.92008829642072243 ) ) ;
#20193=CARTESIAN_POINT ( 'NONE',  ( -27.16883889988623935, 65.32500000273117280, 19.73931689729374739 ) ) ;
#20197=CARTESIAN_POINT ( 'NONE',  ( -33.58253175000000113, 15.02500000273119873, -10.91162601494193041 ) ) ;
#20198=CARTESIAN_POINT ( 'NONE',  ( 7.236395654485760609, 11.52499999726880375, -22.27133577429736633 ) ) ;
#20204=ADVANCED_FACE ( 'NONE', ( #15653 ), #23024, .T. ) ;
#20206=VERTEX_POINT ( 'NONE', #25598 ) ;
#20210=CYLINDRICAL_SURFACE ( 'NONE', #11271, 15.00000000000000000 ) ;
#20211=CARTESIAN_POINT ( 'NONE',  ( 7.236395654485755280, 6.724999997268804819, 22.27133577429736988 ) ) ;
#20212=CARTESIAN_POINT ( 'NONE',  ( -4.523095164977116484E-15, 10.12499999726881938, 24.62258325217400312 ) ) ;
#20213=CARTESIAN_POINT ( 'NONE',  ( -10.37757302488624411, 18.97500000273119625, -31.93888565452638417 ) ) ;
#20214=CARTESIAN_POINT ( 'NONE',  ( -32.50000000000000000, 24.50000000546237544, 0.000000000000000000 ) ) ;
#20215=CARTESIAN_POINT ( 'NONE',  ( -32.50000000000000000, 68.09999999999995168, 10.55989012756946366 ) ) ;
#20216=CARTESIAN_POINT ( 'NONE',  ( 7.570916362186213000, 12.14999999453764090, -23.30088464923126423 ) ) ;
#20219=CARTESIAN_POINT ( 'NONE',  ( -10.37757302488624411, 30.97500000273117848, -31.93888565452638417 ) ) ;
#20220=DIRECTION ( 'NONE',  ( -0.000000000000000000, -1.000000000000000000, -0.000000000000000000 ) ) ;
#20223=CARTESIAN_POINT ( 'NONE',  ( 3.778760231354629433E-15, 0.5000000000000067724, -24.50000000000000355 ) ) ;
#20224=CARTESIAN_POINT ( 'NONE',  ( 32.50000000000000000, 9.000000000000007105, -3.980102097228898626E-15 ) ) ;
#20225=CARTESIAN_POINT ( 'NONE',  ( -4.405589869732278832E-13, 9.000000005462366559, 32.50000000000000000 ) ) ;
#20227=CARTESIAN_POINT ( 'NONE',  ( 33.58253175000000823, 58.02500000273117564, 10.91162601494192863 ) ) ;
#20229=CARTESIAN_POINT ( 'NONE',  ( -33.58253175000000113, 39.27500000273118275, -10.91162601494193041 ) ) ;
#20232=CARTESIAN_POINT ( 'NONE',  ( -20.08610463437156923, 6.300000000000004263, 27.64615127144130113 ) ) ;
#20235=CARTESIAN_POINT ( 'NONE',  ( -20.08610463437156923, 28.30000000000000782, 27.64615127144130113 ) ) ;
#20237=CARTESIAN_POINT ( 'NONE',  ( 20.08610463437158344, 66.69999999999998863, 27.64615127144129403 ) ) ;
#20239=CARTESIAN_POINT ( 'NONE',  ( 0.000000000000000000, 80.00000000000001421, 0.000000000000000000 ) ) ;
#20242=CARTESIAN_POINT ( 'NONE',  ( 33.58253175000000823, 30.02500000273118985, 10.91162601494192685 ) ) ;
#20243=CARTESIAN_POINT ( 'NONE',  ( 33.58253175000000113, 64.37500000273119838, -4.112674001490185761E-15 ) ) ;
#20245=ORIENTED_EDGE ( 'NONE', *, *, #20115, .F. ) ;
#20249=ORIENTED_EDGE ( 'NONE', *, *, #4371, .F. ) ;
#20254=LINE ( 'NONE', #30697, #32726 ) ;
#20255=CARTESIAN_POINT ( 'NONE',  ( -27.16883889988624290, 39.17500000273118843, -19.73931689729374028 ) ) ;
#20256=CARTESIAN_POINT ( 'NONE',  ( -2.092463501923844636E-15, 46.00000000546238965, -34.17252228774368916 ) ) ;
#20258=CARTESIAN_POINT ( 'NONE',  ( 27.16883889988623935, 26.32500000273119056, -19.73931689729374384 ) ) ;
#20260=CARTESIAN_POINT ( 'NONE',  ( 20.75514604977249178, 56.07500000273117990, 28.56700777964553950 ) ) ;
#20262=CARTESIAN_POINT ( 'NONE',  ( -32.50000000000000000, 30.10000000000000853, 10.55989012756946366 ) ) ;
#20264=CARTESIAN_POINT ( 'NONE',  ( -20.75514604977248823, 76.82500000273120122, -28.56700777964554305 ) ) ;
#20266=CARTESIAN_POINT ( 'NONE',  ( 33.58253175000000823, 62.27500000273118985, 10.91162601494192685 ) ) ;
#20269=CARTESIAN_POINT ( 'NONE',  ( -27.16883889988623935, 19.32500000273118701, 19.73931689729374739 ) ) ;
#20270=CARTESIAN_POINT ( 'NONE',  ( -15.14183272437242600, 13.04999999453763770, 20.84094480462497856 ) ) ;
#20277=CARTESIAN_POINT ( 'NONE',  ( 5.779280353836490358E-15, 3.000000005462374109, 32.49999999999999289 ) ) ;
#20283=CARTESIAN_POINT ( 'NONE',  ( -10.04305231718579172, 76.10000000546237686, -30.90933677959248982 ) ) ;
#20285=EDGE_CURVE ( 'NONE', #15702, #14454, #14284, .T. ) ;
#20289=CARTESIAN_POINT ( 'NONE',  ( 33.58253175000000823, 74.27500000273117564, 10.91162601494192863 ) ) ;
#20292=CARTESIAN_POINT ( 'NONE',  ( 32.50000000000000000, 65.60000000546237686, -10.55989012756945833 ) ) ;
#20295=CARTESIAN_POINT ( 'NONE',  ( 6.486482029760649416E-15, 49.62500000273117706, 35.31076352940723240 ) ) ;
#20296=CARTESIAN_POINT ( 'NONE',  ( 18.94512977948575738, 16.42499999726882010, 13.76444248337723408 ) ) ;
#20297=CARTESIAN_POINT ( 'NONE',  ( -26.29305231718578995, 4.700000005462390718, 19.10302069950538595 ) ) ;
#20298=CARTESIAN_POINT ( 'NONE',  ( 0.000000000000000000, 0.000000000000000000, -32.50000000000000000 ) ) ;
#20300=CARTESIAN_POINT ( 'NONE',  ( -20.08610463437156923, 52.30000000000001137, 27.64615127144130113 ) ) ;
#20301=CARTESIAN_POINT ( 'NONE',  ( -10.04305231718579172, 13.60000000000000142, -30.90933677959248982 ) ) ;
#20302=CARTESIAN_POINT ( 'NONE',  ( -33.58253175000000113, 15.37500000273117706, 0.000000000000000000 ) ) ;
#20304=CARTESIAN_POINT ( 'NONE',  ( -4.300734207923755825, 77.77500000273118985, 13.23629886949340673 ) ) ;
#20305=CARTESIAN_POINT ( 'NONE',  ( 12.13525491562420910, 75.45000000546237118, -8.816778784387098611 ) ) ;
#20306=CARTESIAN_POINT ( 'NONE',  ( -20.08610463437157989, 43.69999999999998863, -27.64615127144129758 ) ) ;
#20309=ORIENTED_EDGE ( 'NONE', *, *, #10417, .F. ) ;
#20313=( BOUNDED_CURVE ( )  B_SPLINE_CURVE ( 2, ( #19458, #29563, #8476, #27344, #16717, #19622, #24928, #27171, #22362, #18963, #29407, #3334, #13805 ),
 .UNSPECIFIED., .F., .T. ) 
 B_SPLINE_CURVE_WITH_KNOTS ( ( 3, 2, 2, 2, 2, 2, 3 ),
 ( 0.6346153846153845812, 0.6358974358974358587, 0.6384615384615384137, 0.6410256410256410797, 0.6435897435897436347, 0.6461538461538461897, 0.6474358974358974672 ),
 .UNSPECIFIED. ) 
 CURVE ( )  GEOMETRIC_REPRESENTATION_ITEM ( )  RATIONAL_B_SPLINE_CURVE ( ( 0.9755282581475768211, 0.9755282581475768211, 1.000000000000000000, 0.9510565162951535312, 1.000000000000000000, 0.9510565162951535312, 1.000000000000000000, 0.9510565162951535312, 1.000000000000000000, 0.9510565162951535312, 1.000000000000000000, 0.9755282581475768211, 0.9755282581475768211 ) ) 
 REPRESENTATION_ITEM ( '' )  );
#20318=CARTESIAN_POINT ( 'NONE',  ( -27.16883889988624290, 5.175000002731189319, -19.73931689729374028 ) ) ;
#20322=CARTESIAN_POINT ( 'NONE',  ( 20.08610463437157279, 3.299999999999982947, -27.64615127144129758 ) ) ;
#20324=CARTESIAN_POINT ( 'NONE',  ( 27.16883889988623935, 42.32500000273120833, -19.73931689729374384 ) ) ;
#20331=CARTESIAN_POINT ( 'NONE',  ( 20.75514604977248467, 78.67500000273116711, -28.56700777964554305 ) ) ;
#20335=VERTEX_POINT ( 'NONE', #33655 ) ;
#20336=CARTESIAN_POINT ( 'NONE',  ( 0.000000000000000000, 0.000000000000000000, 0.000000000000000000 ) ) ;
#20337=CARTESIAN_POINT ( 'NONE',  ( 10.37757302488624767, 65.72500000273117848, 31.93888565452638417 ) ) ;
#20339=CARTESIAN_POINT ( 'NONE',  ( -4.732186688966233175E-15, 13.50000000000001066, 25.76082449383753925 ) ) ;
#20340=CARTESIAN_POINT ( 'NONE',  ( -23.41746825000000243, 4.224999997268803931, 7.608796670333725309 ) ) ;
#20341=CARTESIAN_POINT ( 'NONE',  ( -10.37757302488624411, 10.72500000273118914, -31.93888565452638417 ) ) ;
#20344=CARTESIAN_POINT ( 'NONE',  ( -4.635254915624208216, 74.40000000000001990, 14.26584774442730463 ) ) ;
#20347=CARTESIAN_POINT ( 'NONE',  ( 32.50000000000000711, 61.40000000546236691, 10.55989012756945122 ) ) ;
#20349=CARTESIAN_POINT ( 'NONE',  ( 15.00000000000000000, 79.35000000546239107, -4.873795443493596835 ) ) ;
#20351=EDGE_CURVE ( 'NONE', #20335, #33960, #6156, .T. ) ;
#20352=CARTESIAN_POINT ( 'NONE',  ( -33.58253175000000113, 31.12500000273119127, 0.000000000000000000 ) ) ;
#20357=CARTESIAN_POINT ( 'NONE',  ( -33.58253175000000113, 23.47500000273119269, 10.91162601494193929 ) ) ;
#20358=ADVANCED_FACE ( 'NONE', ( #33828 ), #10788, .F. ) ;
#20359=CARTESIAN_POINT ( 'NONE',  ( 33.58253175000000113, 78.22500000273117848, -10.91162601494193574 ) ) ;
#20360=CARTESIAN_POINT ( 'NONE',  ( -10.04305231718578462, 26.90000000546238823, 30.90933677959249337 ) ) ;
#20362=CARTESIAN_POINT ( 'NONE',  ( 23.41746824999999887, 18.62499999726882649, 0.000000000000000000 ) ) ;
#20363=CARTESIAN_POINT ( 'NONE',  ( -10.37757302488623701, 67.52500000273120406, 31.93888565452638417 ) ) ;
#20367=CARTESIAN_POINT ( 'NONE',  ( 33.58253175000000823, 4.025000002731196957, 10.91162601494192685 ) ) ;
#20368=CARTESIAN_POINT ( 'NONE',  ( 23.41746824999999887, 13.12499999726882116, 0.000000000000000000 ) ) ;
#20370=ORIENTED_EDGE ( 'NONE', *, *, #25524, .T. ) ;
#20373=ORIENTED_EDGE ( 'NONE', *, *, #12596, .T. ) ;
#20377=DIRECTION ( 'NONE',  ( -0.000000000000000000, -1.000000000000000000, -0.000000000000000000 ) ) ;
#20378=CARTESIAN_POINT ( 'NONE',  ( -14.47279130897151589, 3.824999997268816454, -19.92008829642072598 ) ) ;
#20379=CARTESIAN_POINT ( 'NONE',  ( 14.47279130897151589, 14.32499999726880624, 19.92008829642072953 ) ) ;
#20380=CARTESIAN_POINT ( 'NONE',  ( -10.37757302488624411, 16.97500000273119269, -31.93888565452638417 ) ) ;
#20381=CARTESIAN_POINT ( 'NONE',  ( 10.04305231718578817, 23.90000000546238468, -30.90933677959249337 ) ) ;
#20382=CARTESIAN_POINT ( 'NONE',  ( -32.50000000000000000, 67.89999999999996305, -10.55989012756945478 ) ) ;
#20386=CARTESIAN_POINT ( 'NONE',  ( 20.75514604977248467, 32.67500000273118843, -28.56700777964554305 ) ) ;
#20387=CARTESIAN_POINT ( 'NONE',  ( -2.165007332552593587E-13, 45.00000000546237544, 32.50000000000000000 ) ) ;
#20390=CARTESIAN_POINT ( 'NONE',  ( -18.94512977948575738, 13.92499999726881654, -13.76444248337723231 ) ) ;
#20391=CARTESIAN_POINT ( 'NONE',  ( 20.08610463437158344, 10.70000000000001172, 27.64615127144129403 ) ) ;
#20393=EDGE_CURVE ( 'NONE', #17459, #32333, #28353, .T. ) ;
#20395=CARTESIAN_POINT ( 'NONE',  ( -2.162160676586881955E-15, 50.62500000273118417, -35.31076352940723240 ) ) ;
#20397=CARTESIAN_POINT ( 'NONE',  ( -27.16883889988624290, 39.17500000273118843, -19.73931689729374028 ) ) ;
#20401=CARTESIAN_POINT ( 'NONE',  ( -10.04305231718579172, 27.60000000000001208, -30.90933677959248982 ) ) ;
#20403=DIRECTION ( 'NONE',  ( 0.000000000000000000, -1.000000000000000000, 0.000000000000000000 ) ) ;
#20408=( BOUNDED_CURVE ( )  B_SPLINE_CURVE ( 2, ( #20101, #12711, #6873, #28157, #4643, #25064, #22490, #30203, #25586, #6704, #12193, #32941, #9440 ),
 .UNSPECIFIED., .F., .F. ) 
 B_SPLINE_CURVE_WITH_KNOTS ( ( 3, 2, 2, 2, 2, 2, 3 ),
 ( 0.3055555555555555802, 0.3111111111111111160, 0.3222222222222222432, 0.3333333333333333148, 0.3444444444444444420, 0.3555555555555555691, 0.3611111111111111049 ),
 .UNSPECIFIED. ) 
 CURVE ( )  GEOMETRIC_REPRESENTATION_ITEM ( )  RATIONAL_B_SPLINE_CURVE ( ( 0.9755282581475767101, 0.9755282581475768211, 1.000000000000000000, 0.9510565162951535312, 1.000000000000000000, 0.9510565162951535312, 1.000000000000000000, 0.9510565162951535312, 1.000000000000000000, 0.9510565162951535312, 1.000000000000000000, 0.9755282581475768211, 0.9755282581475768211 ) ) 
 REPRESENTATION_ITEM ( '' )  );
#20409=CARTESIAN_POINT ( 'NONE',  ( 5.779280353836490358E-15, 61.00000000546238255, 32.49999999999999289 ) ) ;
#20410=CARTESIAN_POINT ( 'NONE',  ( -20.75514604977248112, 25.42500000273119198, 28.56700777964554661 ) ) ;
#20415=CARTESIAN_POINT ( 'NONE',  ( -10.04305231718579172, 16.10000000546238397, -30.90933677959248982 ) ) ;
#20416=ORIENTED_EDGE ( 'NONE', *, *, #10557, .T. ) ;
#20419=AXIS2_PLACEMENT_3D ( 'NONE', #8655, #26852, #29577 ) ;
#20424=CARTESIAN_POINT ( 'NONE',  ( 10.37757302488624767, 37.97500000273118559, 31.93888565452638417 ) ) ;
#20425=CARTESIAN_POINT ( 'NONE',  ( 6.277390505771533514E-15, 41.00000000546236123, 34.17252228774368916 ) ) ;
#20427=CARTESIAN_POINT ( 'NONE',  ( 33.58253175000000113, 24.12500000273118417, -4.112674001490185761E-15 ) ) ;
#20428=CARTESIAN_POINT ( 'NONE',  ( 26.29305231718578995, 31.70000000546238539, -19.10302069950538240 ) ) ;
#20429=CARTESIAN_POINT ( 'NONE',  ( 10.37757302488624056, 46.77500000273118985, -31.93888565452638417 ) ) ;
#20432=CARTESIAN_POINT ( 'NONE',  ( -32.50000000000000000, 25.99999999999999645, 0.000000000000000000 ) ) ;
#20434=CARTESIAN_POINT ( 'NONE',  ( 6.486482029760649416E-15, 73.62500000273118417, 35.31076352940723240 ) ) ;
#20436=CARTESIAN_POINT ( 'NONE',  ( -7.570916362186215665, 15.39999999999999680, 23.30088464923126423 ) ) ;
#20437=CARTESIAN_POINT ( 'NONE',  ( 33.58253175000000113, 58.37500000273118417, -4.112674001490185761E-15 ) ) ;
#20439=CARTESIAN_POINT ( 'NONE',  ( -5.147494310547423346, 40.94874572391552903, 32.50000000000000000 ) ) ;
#20440=CARTESIAN_POINT ( 'NONE',  ( -10.37757302488624411, 20.72500000273119625, -31.93888565452638417 ) ) ;
#20441=CARTESIAN_POINT ( 'NONE',  ( -15.14183272437241889, 8.449999994537634507, -20.84094480462497856 ) ) ;
#20443=LINE ( 'NONE', #1715, #5307 ) ;
#20444=VECTOR ( 'NONE', #9751, 1000.000000000000000 ) ;
#20453=CARTESIAN_POINT ( 'NONE',  ( 5.147494310547434893, 62.55125428154684641, 32.49999999999999289 ) ) ;
#20455=CARTESIAN_POINT ( 'NONE',  ( -18.94512977948576093, 2.324999997268817342, 13.76444248337722698 ) ) ;
#20456=CARTESIAN_POINT ( 'NONE',  ( -26.29305231718578995, 72.70000000546239960, 19.10302069950538595 ) ) ;
#20461=CARTESIAN_POINT ( 'NONE',  ( 20.75514604977248467, 76.67500000273116711, -28.56700777964554305 ) ) ;
#20464=CARTESIAN_POINT ( 'NONE',  ( -33.58253175000000113, 57.37500000273118417, 0.000000000000000000 ) ) ;
#20465=CARTESIAN_POINT ( 'NONE',  ( 6.277390505771533514E-15, 61.00000000546237544, 34.17252228774368916 ) ) ;
#20468=CARTESIAN_POINT ( 'NONE',  ( 27.16883889988623935, 44.32500000273117990, -19.73931689729374384 ) ) ;
#20469=CARTESIAN_POINT ( 'NONE',  ( -23.41746824999999887, 15.62499999726882294, -2.867812753649727150E-15 ) ) ;
#20470=CARTESIAN_POINT ( 'NONE',  ( -27.16883889988624290, 67.17500000273119554, -19.73931689729374028 ) ) ;
#20471=CARTESIAN_POINT ( 'NONE',  ( 32.50000000000000000, 3.600000005462360431, -10.55989012756945833 ) ) ;
#20474=CARTESIAN_POINT ( 'NONE',  ( 23.41746824999999887, 19.02499999726880375, 7.608796670333735079 ) ) ;
#20475=CARTESIAN_POINT ( 'NONE',  ( 10.04305231718578817, 49.39999999999999858, -30.90933677959249337 ) ) ;
#20476=CARTESIAN_POINT ( 'NONE',  ( 0.000000000000000000, 80.00000000000001421, 0.000000000000000000 ) ) ;
#20477=CARTESIAN_POINT ( 'NONE',  ( 33.58253175000000113, 18.47500000273117848, -10.91162601494193751 ) ) ;
#20478=CARTESIAN_POINT ( 'NONE',  ( 5.334720326618300005E-14, 73.50000000000001421, -32.50000000000000000 ) ) ;
#20480=CARTESIAN_POINT ( 'NONE',  ( 8.601468415847516980, 80.67500000273116711, -11.83890561707634781 ) ) ;
#20481=CARTESIAN_POINT ( 'NONE',  ( 27.16883889988623935, 78.57500000273121543, -19.73931689729374384 ) ) ;
#20482=CARTESIAN_POINT ( 'NONE',  ( 5.147494310547434893, 53.05125428700922185, 32.49999999999999289 ) ) ;
#20494=ADVANCED_FACE ( 'NONE', ( #4157 ), #4839, .T. ) ;
#20497=CARTESIAN_POINT ( 'NONE',  ( -13.91746824999999887, 73.37500000273119838, 0.000000000000000000 ) ) ;
#20499=CARTESIAN_POINT ( 'NONE',  ( 33.58253175000000113, 46.22500000273119980, -10.91162601494193574 ) ) ;
#20502=EDGE_CURVE ( 'NONE', #16901, #22348, #11868, .T. ) ;
#20503=EDGE_CURVE ( 'NONE', #26581, #10540, #4866, .T. ) ;
#20505=VERTEX_POINT ( 'NONE', #23718 ) ;
#20507=CARTESIAN_POINT ( 'NONE',  ( 2.489536152421872915E-14, 75.50000000000000000, -32.49999999999999289 ) ) ;
#20509=CARTESIAN_POINT ( 'NONE',  ( 20.75514604977249178, 74.07500000273120122, 28.56700777964553950 ) ) ;
#20516=CARTESIAN_POINT ( 'NONE',  ( 33.58253175000000823, 60.02500000273116854, 10.91162601494192863 ) ) ;
#20519=CARTESIAN_POINT ( 'NONE',  ( -19.82091636218621389, 13.19999999999998863, 14.40073868116558842 ) ) ;
#20520=CARTESIAN_POINT ( 'NONE',  ( 3.980102097228898626E-15, 80.00000000000001421, 32.50000000000000000 ) ) ;
#20521=CARTESIAN_POINT ( 'NONE',  ( -27.16883889988624290, 8.925000002731191984, -19.73931689729374028 ) ) ;
#20523=CARTESIAN_POINT ( 'NONE',  ( 32.50000000000000000, 29.10000000000001208, -10.55989012756945833 ) ) ;
#20525=CARTESIAN_POINT ( 'NONE',  ( 2.897257156509938333E-15, 72.50000000000001421, 15.77193336357400710 ) ) ;
#20526=VECTOR ( 'NONE', #32894, 1000.000000000000000 ) ;
#20531=CARTESIAN_POINT ( 'NONE',  ( 2.897257156509938333E-15, 70.75000000546236834, 15.77193336357400710 ) ) ;
#20533=CARTESIAN_POINT ( 'NONE',  ( 27.16883889988624290, 29.92500000273118488, 19.73931689729373673 ) ) ;
#20536=CARTESIAN_POINT ( 'NONE',  ( 27.16883889988624290, 22.17500000273120264, 19.73931689729373673 ) ) ;
#20537=CARTESIAN_POINT ( 'NONE',  ( -12.13525491562420910, 80.19999999999998863, 8.816778784387098611 ) ) ;
#20538=CARTESIAN_POINT ( 'NONE',  ( 33.58253175000000113, 76.22500000273119269, -10.91162601494193574 ) ) ;
#20539=CARTESIAN_POINT ( 'NONE',  ( -10.04305231718579172, 65.59999999999999432, -30.90933677959248982 ) ) ;
#20541=CARTESIAN_POINT ( 'NONE',  ( -4.523095164977117273E-15, 16.12499999726880517, 24.62258325217400312 ) ) ;
#20542=CARTESIAN_POINT ( 'NONE',  ( 33.58253175000000823, 64.02500000273118985, 10.91162601494192685 ) ) ;
#20545=CARTESIAN_POINT ( 'NONE',  ( -2.162160676586882350E-15, 6.625000002731173510, -35.31076352940722529 ) ) ;
#20546=CARTESIAN_POINT ( 'NONE',  ( -23.41746825000000598, 14.22499999726880660, 7.608796670333726198 ) ) ;
#20550=EDGE_CURVE ( 'NONE', #7704, #15702, #19999, .T. ) ;
#20556=CARTESIAN_POINT ( 'NONE',  ( 7.236395654485760609, 1.524999997268822183, -22.27133577429736633 ) ) ;
#20557=CARTESIAN_POINT ( 'NONE',  ( 23.41746824999999887, 14.62499999726882294, 0.000000000000000000 ) ) ;
#20559=CARTESIAN_POINT ( 'NONE',  ( -33.58253175000000113, 15.27500000273118985, -10.91162601494193218 ) ) ;
#20560=CARTESIAN_POINT ( 'NONE',  ( -26.29305231718578995, 16.70000000546237473, 19.10302069950538595 ) ) ;
#20561=CARTESIAN_POINT ( 'NONE',  ( 10.04305231718579705, 64.59999999999999432, 30.90933677959248982 ) ) ;
#20562=CARTESIAN_POINT ( 'NONE',  ( 24.50000000000000000, 11.84999999453761710, -7.960532557706203605 ) ) ;
#20563=DIRECTION ( 'NONE',  ( 0.000000000000000000, 0.000000000000000000, 1.000000000000000000 ) ) ;
#20565=CARTESIAN_POINT ( 'NONE',  ( -33.58253175000000113, 31.47500000273117493, 10.91162601494193929 ) ) ;
#20566=CARTESIAN_POINT ( 'NONE',  ( -1.778240108872766143E-15, 44.00000000546238255, -32.49999999999999289 ) ) ;
#20569=CARTESIAN_POINT ( 'NONE',  ( -14.47279130897152122, 14.42499999726880056, 19.92008829642072243 ) ) ;
#20570=CARTESIAN_POINT ( 'NONE',  ( 32.50000000000000000, 7.000000000000006217, -3.980102097228898626E-15 ) ) ;
#20571=VECTOR ( 'NONE', #29005, 1000.000000000000000 ) ;
#20572=CARTESIAN_POINT ( 'NONE',  ( 5.779280353836490358E-15, 74.50000000000001421, 32.49999999999999289 ) ) ;
#20574=CARTESIAN_POINT ( 'NONE',  ( 20.75514604977248467, 50.42500000273118843, -28.56700777964554305 ) ) ;
#20576=CARTESIAN_POINT ( 'NONE',  ( 6.486482029760648627E-15, 41.87500000273119127, 35.31076352940722529 ) ) ;
#20579=CARTESIAN_POINT ( 'NONE',  ( -26.29305231718579350, 61.79999999999999716, -19.10302069950537884 ) ) ;
#20583=CARTESIAN_POINT ( 'NONE',  ( 32.50000000000000711, 6.900000000000014566, 10.55989012756945122 ) ) ;
#20585=CARTESIAN_POINT ( 'NONE',  ( 24.50000000000000000, 9.749999994537628112, 0.000000000000000000 ) ) ;
#20588=CARTESIAN_POINT ( 'NONE',  ( -32.50000000000000000, 11.90000000000000213, -10.55989012756945300 ) ) ;
#20589=CARTESIAN_POINT ( 'NONE',  ( 20.75514604977248467, 24.42500000273119198, -28.56700777964554305 ) ) ;
#20590=AXIS2_PLACEMENT_3D ( 'NONE', #22203, #22530, #17052 ) ;
#20592=ORIENTED_EDGE ( 'NONE', *, *, #22716, .F. ) ;
#20596=ORIENTED_EDGE ( 'NONE', *, *, #31314, .T. ) ;
#20601=ADVANCED_FACE ( 'NONE', ( #25946 ), #31593, .T. ) ;
#20603=DIRECTION ( 'NONE',  ( -0.000000000000000000, -1.000000000000000000, -0.000000000000000000 ) ) ;
#20604=CARTESIAN_POINT ( 'NONE',  ( 33.58253175000000113, 34.47500000273119980, -10.91162601494193751 ) ) ;
#20605=CARTESIAN_POINT ( 'NONE',  ( -32.50000000000000000, 34.60000000546236976, 10.55989012756946366 ) ) ;
#20606=CIRCLE ( 'NONE', #3081, 26.50000000000000355 ) ;
#20609=CARTESIAN_POINT ( 'NONE',  ( 6.486482029760649416E-15, 21.62500000273119483, 35.31076352940723240 ) ) ;
#20611=CARTESIAN_POINT ( 'NONE',  ( 33.58253175000000113, 48.37500000273120548, -4.112674001490185761E-15 ) ) ;
#20614=CARTESIAN_POINT ( 'NONE',  ( -32.50000000000000000, 29.89999999999998437, -10.55989012756945478 ) ) ;
#20616=CARTESIAN_POINT ( 'NONE',  ( 10.37757302488624767, 67.72500000273117848, 31.93888565452638417 ) ) ;
#20618=CARTESIAN_POINT ( 'NONE',  ( -19.82091636218621389, 15.19999999999999218, 14.40073868116558842 ) ) ;
#20619=CARTESIAN_POINT ( 'NONE',  ( 27.16883889988623935, 58.57500000273119412, -19.73931689729374384 ) ) ;
#20620=CARTESIAN_POINT ( 'NONE',  ( 26.29305231718578995, 73.19999999999998863, -19.10302069950538240 ) ) ;
#20621=CARTESIAN_POINT ( 'NONE',  ( 10.37757302488624767, 9.725000002731187365, 31.93888565452638417 ) ) ;
#20622=CARTESIAN_POINT ( 'NONE',  ( -24.50000000000001066, 8.849999994537624204, 7.960532557706201828 ) ) ;
#20624=( BOUNDED_CURVE ( )  B_SPLINE_CURVE ( 2, ( #17785, #82, #7988, #5418, #13140, #23613, #28413, #10569, #2152, #18474, #30984, #15209, #23096 ),
 .UNSPECIFIED., .F., .T. ) 
 B_SPLINE_CURVE_WITH_KNOTS ( ( 3, 2, 2, 2, 2, 2, 3 ),
 ( 0.4166666666666666852, 0.4222222222222222210, 0.4333333333333333481, 0.4444444444444444198, 0.4555555555555555469, 0.4666666666666666741, 0.4722222222222222099 ),
 .UNSPECIFIED. ) 
 CURVE ( )  GEOMETRIC_REPRESENTATION_ITEM ( )  RATIONAL_B_SPLINE_CURVE ( ( 0.9755282581475767101, 0.9755282581475768211, 1.000000000000000000, 0.9510565162951535312, 1.000000000000000000, 0.9510565162951535312, 1.000000000000000000, 0.9510565162951535312, 1.000000000000000000, 0.9510565162951535312, 1.000000000000000000, 0.9755282581475768211, 0.9755282581475765991 ) ) 
 REPRESENTATION_ITEM ( '' )  );
#20627=DIRECTION ( 'NONE',  ( -0.000000000000000000, -1.000000000000000000, -0.000000000000000000 ) ) ;
#20628=CARTESIAN_POINT ( 'NONE',  ( 0.000000000000000000, 0.000000000000000000, 0.000000000000000000 ) ) ;
#20632=CARTESIAN_POINT ( 'NONE',  ( -8.891200544363830713E-16, 79.50000000000000000, -15.00000000000000000 ) ) ;
#20635=CARTESIAN_POINT ( 'NONE',  ( 32.50000000000000000, 63.60000000546238397, -10.55989012756945833 ) ) ;
#20636=CARTESIAN_POINT ( 'NONE',  ( -2.092463501923844636E-15, 76.00000000546235412, -34.17252228774368916 ) ) ;
#20640=ORIENTED_EDGE ( 'NONE', *, *, #28233, .T. ) ;
#20641=CARTESIAN_POINT ( 'NONE',  ( -2.162160676586881955E-15, 72.87500000273115575, -35.31076352940723240 ) ) ;
#20646=CARTESIAN_POINT ( 'NONE',  ( 10.37757302488624767, 53.97500000273119980, 31.93888565452638417 ) ) ;
#20647=EDGE_CURVE ( 'NONE', #2121, #22307, #9671, .T. ) ;
#20648=CARTESIAN_POINT ( 'NONE',  ( -20.08610463437156923, 64.80000000546237970, 27.64615127144130113 ) ) ;
#20650=CARTESIAN_POINT ( 'NONE',  ( -20.08610463437157989, 10.20000000546238539, -27.64615127144129758 ) ) ;
#20651=CARTESIAN_POINT ( 'NONE',  ( 27.16883889988623935, 42.32500000273120833, -19.73931689729374384 ) ) ;
#20652=DIRECTION ( 'NONE',  ( -0.000000000000000000, -1.000000000000000000, -0.000000000000000000 ) ) ;
#20653=CARTESIAN_POINT ( 'NONE',  ( -33.58253175000000113, 69.47500000273116427, 10.91162601494193929 ) ) ;
#20654=CARTESIAN_POINT ( 'NONE',  ( -20.08610463437157989, 6.200000005462364960, -27.64615127144129758 ) ) ;
#20657=CARTESIAN_POINT ( 'NONE',  ( 20.08610463437158344, 44.69999999999998153, 27.64615127144129403 ) ) ;
#20658=DIRECTION ( 'NONE',  ( -0.000000000000000000, -1.000000000000000000, -0.000000000000000000 ) ) ;
#20659=CARTESIAN_POINT ( 'NONE',  ( -27.16883889988623935, 9.575000002731204773, 19.73931689729374739 ) ) ;
#20660=CARTESIAN_POINT ( 'NONE',  ( -1.778240108872766143E-15, 6.000000005462371888, -32.49999999999999289 ) ) ;
#20662=CARTESIAN_POINT ( 'NONE',  ( -8.601468415847518756, 79.07500000273121543, -11.83890561707634781 ) ) ;
#20663=CARTESIAN_POINT ( 'NONE',  ( -33.58253175000000113, 79.37500000273118417, 0.000000000000000000 ) ) ;
#20664=CYLINDRICAL_SURFACE ( 'NONE', #11181, 15.00000000000000000 ) ;
#20681=CARTESIAN_POINT ( 'NONE',  ( -20.75514604977248823, 46.82500000273117990, -28.56700777964554305 ) ) ;
#20688=CARTESIAN_POINT ( 'NONE',  ( 6.486482029760649416E-15, 75.87500000273119838, 35.31076352940723240 ) ) ;
#20694=CARTESIAN_POINT ( 'NONE',  ( 33.58253175000000113, 64.22500000273117848, -10.91162601494193751 ) ) ;
#20696=CARTESIAN_POINT ( 'NONE',  ( 24.50000000000000355, 15.89999999999999147, 7.960532557706212486 ) ) ;
#20697=CARTESIAN_POINT ( 'NONE',  ( 23.41746824999999887, 5.024999997268808194, 7.608796670333735079 ) ) ;
#20698=CARTESIAN_POINT ( 'NONE',  ( -20.75514604977248823, 6.825000002731195892, -28.56700777964554305 ) ) ;
#20699=CARTESIAN_POINT ( 'NONE',  ( 26.29305231718579350, 28.79999999999999361, 19.10302069950537529 ) ) ;
#20701=CARTESIAN_POINT ( 'NONE',  ( -9.270509831248423538, 79.95000000546235697, -12.75976212528059861 ) ) ;
#20707=CARTESIAN_POINT ( 'NONE',  ( -15.00000000000000000, 72.25000000546238255, 0.000000000000000000 ) ) ;
#20709=CARTESIAN_POINT ( 'NONE',  ( -20.75514604977248112, 29.42500000273118133, 28.56700777964554661 ) ) ;
#20712=CARTESIAN_POINT ( 'NONE',  ( -33.58253175000000113, 23.37500000273118417, 0.000000000000000000 ) ) ;
#20713=CARTESIAN_POINT ( 'NONE',  ( -5.147494310547430452, 63.55125428154684641, -32.49999999999999289 ) ) ;
#20715=CARTESIAN_POINT ( 'NONE',  ( -33.58253175000000113, 77.02500000273120406, -10.91162601494193041 ) ) ;
#20716=CARTESIAN_POINT ( 'NONE',  ( -26.29305231718579350, 65.79999999999999716, -19.10302069950537884 ) ) ;
#20718=CARTESIAN_POINT ( 'NONE',  ( 18.94512977948576093, 14.82499999726882933, -13.76444248337722875 ) ) ;
#20719=CARTESIAN_POINT ( 'NONE',  ( -27.16883889988624290, 66.92500000273119554, -19.73931689729374028 ) ) ;
#20722=CARTESIAN_POINT ( 'NONE',  ( 27.16883889988623935, 6.325000002731173687, -19.73931689729374384 ) ) ;
#20723=CARTESIAN_POINT ( 'NONE',  ( 1.507698388325705758E-15, 17.62499999726881938, -24.62258325217400312 ) ) ;
#20725=( BOUNDED_CURVE ( )  B_SPLINE_CURVE ( 2, ( #24217, #26453, #27797, #14419, #6523, #24706, #32590, #22472, #21811, #1013, #16995, #11834, #32757 ),
 .UNSPECIFIED., .F., .F. ) 
 B_SPLINE_CURVE_WITH_KNOTS ( ( 3, 2, 2, 2, 2, 2, 3 ),
 ( 0.7500000000000000000, 0.7512820512820512775, 0.7538461538461538325, 0.7564102564102563875, 0.7589743589743589425, 0.7615384615384614975, 0.7628205128205127750 ),
 .UNSPECIFIED. ) 
 CURVE ( )  GEOMETRIC_REPRESENTATION_ITEM ( )  RATIONAL_B_SPLINE_CURVE ( ( 0.9755282581475768211, 0.9755282581475768211, 1.000000000000000000, 0.9510565162951535312, 1.000000000000000000, 0.9510565162951535312, 1.000000000000000000, 0.9510565162951535312, 1.000000000000000000, 0.9510565162951535312, 1.000000000000000000, 0.9755282581475768211, 0.9755282581475768211 ) ) 
 REPRESENTATION_ITEM ( '' )  );
#20728=ORIENTED_EDGE ( 'NONE', *, *, #21220, .F. ) ;
#20732=CARTESIAN_POINT ( 'NONE',  ( 33.58253175000000113, 78.12500000273119838, -4.112674001490185761E-15 ) ) ;
#20733=CARTESIAN_POINT ( 'NONE',  ( -7.236395654485763274, 4.524999997268825069, 22.27133577429736633 ) ) ;
#20734=CARTESIAN_POINT ( 'NONE',  ( 7.236395654485760609, 17.02499999726880731, -22.27133577429736633 ) ) ;
#20735=CARTESIAN_POINT ( 'NONE',  ( 6.486482029760649416E-15, 13.87500000273117529, 35.31076352940723240 ) ) ;
#20736=CARTESIAN_POINT ( 'NONE',  ( 10.04305231718578817, 17.90000000546238113, -30.90933677959249337 ) ) ;
#20737=CARTESIAN_POINT ( 'NONE',  ( -26.29305231718578995, 66.19999999999997442, 19.10302069950538595 ) ) ;
#20738=CARTESIAN_POINT ( 'NONE',  ( 7.890940483122900408E-14, 12.24999999453763166, -24.50000000000000000 ) ) ;
#20741=CARTESIAN_POINT ( 'NONE',  ( -32.50000000000000000, 32.60000000546237686, 10.55989012756946366 ) ) ;
#20743=PRODUCT_CONTEXT ( 'NONE', #25441, 'mechanical' ) ;
#20744=CYLINDRICAL_SURFACE ( 'NONE', #33238, 32.50000000000000000 ) ;
#20745=CARTESIAN_POINT ( 'NONE',  ( -18.94512977948576093, 14.32499999726882756, 13.76444248337722698 ) ) ;
#20746=CARTESIAN_POINT ( 'NONE',  ( -32.50000000000000000, 6.099999999999981881, 10.55989012756946366 ) ) ;
#20747=CARTESIAN_POINT ( 'NONE',  ( 5.779280353836490358E-15, 17.00000000546237899, 32.49999999999999289 ) ) ;
#20749=CARTESIAN_POINT ( 'NONE',  ( 33.58253175000000113, 50.22500000273118559, -10.91162601494193751 ) ) ;
#20751=CARTESIAN_POINT ( 'NONE',  ( -33.58253175000000113, 41.37500000273119838, 0.000000000000000000 ) ) ;
#20753=CARTESIAN_POINT ( 'NONE',  ( 32.50000000000000711, 15.40000000546236514, 10.55989012756945122 ) ) ;
#20754=CARTESIAN_POINT ( 'NONE',  ( -1.778240108872766143E-15, 31.49999999999998579, -32.49999999999999289 ) ) ;
#20755=CARTESIAN_POINT ( 'NONE',  ( -26.29305231718578995, 28.20000000000000284, 19.10302069950538595 ) ) ;
#20762=CARTESIAN_POINT ( 'NONE',  ( 7.570916362186213000, 18.14999999453761959, -23.30088464923126423 ) ) ;
#20763=CARTESIAN_POINT ( 'NONE',  ( -33.58253175000000113, 29.02500000273119340, -10.91162601494193041 ) ) ;
#20768=ORIENTED_EDGE ( 'NONE', *, *, #14495, .F. ) ;
#20773=CARTESIAN_POINT ( 'NONE',  ( 6.486482029760649416E-15, 33.87500000273118417, 35.31076352940723240 ) ) ;
#20774=CARTESIAN_POINT ( 'NONE',  ( -20.08610463437156923, 38.80000000546237260, 27.64615127144130113 ) ) ;
#20776=CARTESIAN_POINT ( 'NONE',  ( -26.29305231718579350, 47.80000000000001137, -19.10302069950537884 ) ) ;
#20777=CARTESIAN_POINT ( 'NONE',  ( 33.58253175000000113, 22.22500000273117493, -10.91162601494193751 ) ) ;
#20778=CARTESIAN_POINT ( 'NONE',  ( -9.270509831248423538, 81.70000000000000284, -12.75976212528059861 ) ) ;
#20779=CARTESIAN_POINT ( 'NONE',  ( -27.16883889988624290, 49.17500000273117422, -19.73931689729374028 ) ) ;
#20782=CARTESIAN_POINT ( 'NONE',  ( -26.29305231718579350, 29.79999999999999361, -19.10302069950537884 ) ) ;
#20784=CARTESIAN_POINT ( 'NONE',  ( -2.162160676586881955E-15, 72.62500000273118417, -35.31076352940723240 ) ) ;
#20785=CARTESIAN_POINT ( 'NONE',  ( 2.489536152421872915E-14, 77.50000000000001421, -32.49999999999999289 ) ) ;
#20786=CARTESIAN_POINT ( 'NONE',  ( -3.880418787951104953, 15.44874571845315359, 24.50000000000000711 ) ) ;
#20787=CARTESIAN_POINT ( 'NONE',  ( 6.486482029760648627E-15, 57.87500000273117706, 35.31076352940722529 ) ) ;
#20789=CARTESIAN_POINT ( 'NONE',  ( -20.75514604977248823, 10.82500000273118701, -28.56700777964554305 ) ) ;
#20795=EDGE_CURVE ( 'NONE', #4197, #32174, #17798, .T. ) ;
#20800=CARTESIAN_POINT ( 'NONE',  ( 32.50000000000000000, 61.09999999999998721, -10.55989012756945833 ) ) ;
#20803=CARTESIAN_POINT ( 'NONE',  ( -32.50000000000000000, 66.40000000546238823, -10.55989012756945478 ) ) ;
#20808=CARTESIAN_POINT ( 'NONE',  ( -33.58253175000000113, 77.27500000273117564, -10.91162601494193218 ) ) ;
#20812=CARTESIAN_POINT ( 'NONE',  ( -33.58253175000000113, 55.37500000273118417, 0.000000000000000000 ) ) ;
#20813=CARTESIAN_POINT ( 'NONE',  ( -10.04305231718578462, 58.90000000546238823, 30.90933677959249337 ) ) ;
#20815=CARTESIAN_POINT ( 'NONE',  ( -20.75514604977248823, 42.82500000273119412, -28.56700777964554305 ) ) ;
#20817=CARTESIAN_POINT ( 'NONE',  ( -33.58253175000000113, 71.27500000273118985, -10.91162601494193218 ) ) ;
#20821=CARTESIAN_POINT ( 'NONE',  ( -10.04305231718579172, 45.60000000000000142, -30.90933677959248982 ) ) ;
#20824=CARTESIAN_POINT ( 'NONE',  ( 20.75514604977248467, 10.67500000273119021, -28.56700777964554305 ) ) ;
#20827=CARTESIAN_POINT ( 'NONE',  ( -13.91746824999999532, 81.27500000273120406, -4.522059556121115875 ) ) ;
#20828=DIRECTION ( 'NONE',  ( 0.000000000000000000, -1.000000000000000000, 0.000000000000000000 ) ) ;
#20829=FACE_OUTER_BOUND ( 'NONE', #6434, .T. ) ;
#20831=VERTEX_POINT ( 'NONE', #8757 ) ;
#20842=CARTESIAN_POINT ( 'NONE',  ( -27.16883889988623935, 45.32500000273117990, 19.73931689729374739 ) ) ;
#20849=CARTESIAN_POINT ( 'NONE',  ( 27.16883889988623935, 78.57500000273121543, -19.73931689729374384 ) ) ;
#20854=CARTESIAN_POINT ( 'NONE',  ( -5.147494310547423346, 14.94874572391553080, 32.50000000000000000 ) ) ;
#20855=CARTESIAN_POINT ( 'NONE',  ( 33.58253175000000823, 62.02500000273116143, 10.91162601494192863 ) ) ;
#20858=CARTESIAN_POINT ( 'NONE',  ( -23.41746824999999887, 2.024999997268815299, -7.608796670333730638 ) ) ;
#20859=CARTESIAN_POINT ( 'NONE',  ( 27.16883889988623935, 2.325000002731170134, -19.73931689729374384 ) ) ;
#20862=DIRECTION ( 'NONE',  ( -0.000000000000000000, -1.000000000000000000, -0.000000000000000000 ) ) ;
#20863=CARTESIAN_POINT ( 'NONE',  ( 1.836970198721029589E-15, 82.00000000000001421, 15.00000000000000000 ) ) ;
#20868=CARTESIAN_POINT ( 'NONE',  ( 13.91746824999999887, 79.87500000273118417, -1.704398294459741270E-15 ) ) ;
#20870=CARTESIAN_POINT ( 'NONE',  ( 20.75514604977249178, 33.82500000273117990, 28.56700777964553950 ) ) ;
#20874=CARTESIAN_POINT ( 'NONE',  ( 33.58253175000000823, 18.27500000273118275, 10.91162601494192685 ) ) ;
#20875=CARTESIAN_POINT ( 'NONE',  ( -2.375766604868044585, 80.44874571845313938, 14.99999999999999822 ) ) ;
#20877=CARTESIAN_POINT ( 'NONE',  ( -20.75514604977248112, 73.42500000273118133, 28.56700777964554661 ) ) ;
#20878=CARTESIAN_POINT ( 'NONE',  ( -20.08610463437156923, 66.29999999999999716, 27.64615127144130113 ) ) ;
#20880=CARTESIAN_POINT ( 'NONE',  ( -7.236395654485763274, 18.02499999726880731, 22.27133577429736633 ) ) ;
#20881=CARTESIAN_POINT ( 'NONE',  ( -10.37757302488623701, 65.52500000273120406, 31.93888565452638417 ) ) ;
#20884=CARTESIAN_POINT ( 'NONE',  ( 20.75514604977249178, 7.825000002731194115, 28.56700777964553950 ) ) ;
#20885=CARTESIAN_POINT ( 'NONE',  ( -23.41746825000000243, 1.524999997268801755, -7.608796670333730638 ) ) ;
#20887=VERTEX_POINT ( 'NONE', #26792 ) ;
#20891=CARTESIAN_POINT ( 'NONE',  ( 3.980102097228898626E-15, 80.00000000000001421, 32.50000000000000000 ) ) ;
#20893=CARTESIAN_POINT ( 'NONE',  ( -20.08610463437156923, 72.30000000000001137, 27.64615127144130113 ) ) ;
#20894=CARTESIAN_POINT ( 'NONE',  ( 23.41746825000000243, 3.224999997268806151, -7.608796670333727974 ) ) ;
#20895=CARTESIAN_POINT ( 'NONE',  ( -7.236395654485763274, 16.02499999726880731, 22.27133577429736633 ) ) ;
#20896=CARTESIAN_POINT ( 'NONE',  ( -20.75514604977248112, 17.67500000273117422, 28.56700777964554661 ) ) ;
#20897=CARTESIAN_POINT ( 'NONE',  ( -20.08610463437156923, 58.29999999999999716, 27.64615127144130113 ) ) ;
#20898=CARTESIAN_POINT ( 'NONE',  ( 3.880418787951178228, 12.19874571299079236, -24.49999999999998224 ) ) ;
#20899=CARTESIAN_POINT ( 'NONE',  ( 5.147494310547440222, 73.94874572391552192, -32.50000000000000000 ) ) ;
#20902=CARTESIAN_POINT ( 'NONE',  ( -13.91746824999999887, 73.37500000273119838, 0.000000000000000000 ) ) ;
#20904=DIRECTION ( 'NONE',  ( -1.000000000000000000, 0.000000000000000000, -0.000000000000000000 ) ) ;
#20905=CARTESIAN_POINT ( 'NONE',  ( 20.08610463437158344, 6.699999999999991296, 27.64615127144129403 ) ) ;
#20906=CARTESIAN_POINT ( 'NONE',  ( -8.891200544363830713E-16, 73.50000000000001421, -15.00000000000000000 ) ) ;
#20908=CARTESIAN_POINT ( 'NONE',  ( 10.37757302488624767, 51.72500000273119980, 31.93888565452638417 ) ) ;
#20910=CARTESIAN_POINT ( 'NONE',  ( -20.75514604977248823, 39.07500000273119412, -28.56700777964554305 ) ) ;
#20911=CARTESIAN_POINT ( 'NONE',  ( 20.08610463437158344, 24.70000000000000284, 27.64615127144129403 ) ) ;
#20912=CARTESIAN_POINT ( 'NONE',  ( 0.000000000000000000, 82.00000000000001421, 0.000000000000000000 ) ) ;
#20913=CARTESIAN_POINT ( 'NONE',  ( -32.50000000000000000, 62.00000000000000000, 0.000000000000000000 ) ) ;
#20915=CARTESIAN_POINT ( 'NONE',  ( -4.223320258572819786E-15, 5.249999994537622783, 24.50000000000000000 ) ) ;
#20918=CARTESIAN_POINT ( 'NONE',  ( -5.147494310547430452, 62.05125428700922896, -32.49999999999999289 ) ) ;
#20919=PLANE ( 'NONE',  #31434 ) ;
#20920=EDGE_CURVE ( 'NONE', #31503, #18399, #6528, .T. ) ;
#20921=FACE_OUTER_BOUND ( 'NONE', #6764, .T. ) ;
#20924=CARTESIAN_POINT ( 'NONE',  ( -4.405589869732278832E-13, 10.49999999999998934, 32.50000000000000000 ) ) ;
#20925=CARTESIAN_POINT ( 'NONE',  ( 33.58253175000000823, 28.02500000273119340, 10.91162601494192685 ) ) ;
#20933=ORIENTED_EDGE ( 'NONE', *, *, #30695, .F. ) ;
#20937=CARTESIAN_POINT ( 'NONE',  ( 18.94512977948576093, 0.8249999972688160099, -13.76444248337722875 ) ) ;
#20938=CARTESIAN_POINT ( 'NONE',  ( -10.37757302488624411, 32.97500000273117848, -31.93888565452638417 ) ) ;
#20939=CARTESIAN_POINT ( 'NONE',  ( -32.50000000000000000, 36.60000000546239818, 10.55989012756946366 ) ) ;
#20942=CARTESIAN_POINT ( 'NONE',  ( 20.75514604977248467, 22.42500000273119909, -28.56700777964554305 ) ) ;
#20943=CARTESIAN_POINT ( 'NONE',  ( 7.570916362186213000, 6.149999994537635573, -23.30088464923126423 ) ) ;
#20944=CARTESIAN_POINT ( 'NONE',  ( -20.75514604977248112, 51.67500000273117422, 28.56700777964554661 ) ) ;
#20947=CARTESIAN_POINT ( 'NONE',  ( 10.04305231718579705, 26.60000000000001208, 30.90933677959248982 ) ) ;
#20949=CARTESIAN_POINT ( 'NONE',  ( 27.16883889988623935, 72.32500000273117280, -19.73931689729374384 ) ) ;
#20951=CARTESIAN_POINT ( 'NONE',  ( -32.50000000000000000, 76.40000000546235981, -10.55989012756945300 ) ) ;
#20952=CARTESIAN_POINT ( 'NONE',  ( -10.37757302488624411, 58.97500000273120691, -31.93888565452638417 ) ) ;
#20953=CARTESIAN_POINT ( 'NONE',  ( 20.08610463437158344, 7.200000005462392494, 27.64615127144129403 ) ) ;
#20954=CARTESIAN_POINT ( 'NONE',  ( -27.16883889988624290, 10.92500000273119376, -19.73931689729374028 ) ) ;
#20957=CARTESIAN_POINT ( 'NONE',  ( -33.58253175000000113, 1.475000002731190474, 10.91162601494193929 ) ) ;
#20959=CARTESIAN_POINT ( 'NONE',  ( 24.50000000000000000, 18.87499999726882649, 0.000000000000000000 ) ) ;
#20960=CARTESIAN_POINT ( 'NONE',  ( -1.778240108872766143E-15, 19.50000000000000000, -32.49999999999999289 ) ) ;
#20966=CARTESIAN_POINT ( 'NONE',  ( 18.94512977948576093, 1.324999997268816454, -13.76444248337722875 ) ) ;
#20967=CARTESIAN_POINT ( 'NONE',  ( -32.50000000000000000, 68.50000000546238255, 0.000000000000000000 ) ) ;
#20977=CARTESIAN_POINT ( 'NONE',  ( 33.58253175000000113, 56.47500000273116427, -10.91162601494193751 ) ) ;
#20978=CARTESIAN_POINT ( 'NONE',  ( 32.50000000000000711, 57.40000000546237402, 10.55989012756945122 ) ) ;
#20979=EDGE_CURVE ( 'NONE', #2384, #32915, #11179, .T. ) ;
#20981=CARTESIAN_POINT ( 'NONE',  ( -33.58253175000000113, 45.12500000273117706, 0.000000000000000000 ) ) ;
#20983=CARTESIAN_POINT ( 'NONE',  ( 10.37757302488624767, 69.97500000273119269, 31.93888565452638417 ) ) ;
#20987=CARTESIAN_POINT ( 'NONE',  ( -32.50000000000000000, 43.99999999999998579, 0.000000000000000000 ) ) ;
#20989=CARTESIAN_POINT ( 'NONE',  ( 10.37757302488624056, 10.77500000273118275, -31.93888565452638417 ) ) ;
#20993=CARTESIAN_POINT ( 'NONE',  ( -8.601468415847518756, 73.07500000273115859, -11.83890561707634781 ) ) ;
#20997=ORIENTED_EDGE ( 'NONE', *, *, #7791, .F. ) ;
#21008=CARTESIAN_POINT ( 'NONE',  ( -27.16883889988623935, 37.32500000273120122, 19.73931689729374739 ) ) ;
#21014=AXIS2_PLACEMENT_3D ( 'NONE', #16858, #27146, #29383 ) ;
#21016=CARTESIAN_POINT ( 'NONE',  ( 33.58253175000000823, 76.27500000273118985, 10.91162601494192863 ) ) ;
#21017=ORIENTED_EDGE ( 'NONE', *, *, #28242, .T. ) ;
#21019=VECTOR ( 'NONE', #12261, 1000.000000000000000 ) ;
#21022=ORIENTED_EDGE ( 'NONE', *, *, #8739, .F. ) ;
#21024=CARTESIAN_POINT ( 'NONE',  ( -2.162160676586881955E-15, 58.62500000273118417, -35.31076352940723240 ) ) ;
#21026=EDGE_CURVE ( 'NONE', #21853, #3936, #9457, .T. ) ;
#21027=CARTESIAN_POINT ( 'NONE',  ( 15.14183272437241889, 17.69999999999999218, 20.84094480462498211 ) ) ;
#21028=CARTESIAN_POINT ( 'NONE',  ( -23.41746824999999887, 12.02499999726881974, -7.608796670333730638 ) ) ;
#21029=CARTESIAN_POINT ( 'NONE',  ( 27.16883889988624290, 5.925000002731190207, 19.73931689729373673 ) ) ;
#21030=CARTESIAN_POINT ( 'NONE',  ( -12.13525491562420910, 78.45000000546237118, 8.816778784387098611 ) ) ;
#21032=CARTESIAN_POINT ( 'NONE',  ( -12.13525491562421088, 80.05000000546236549, -8.816778784387096835 ) ) ;
#21034=CARTESIAN_POINT ( 'NONE',  ( 10.04305231718579705, 75.10000000546237686, 30.90933677959248982 ) ) ;
#21038=CARTESIAN_POINT ( 'NONE',  ( -15.00000000000000000, 70.25000000546238255, 0.000000000000000000 ) ) ;
#21040=CARTESIAN_POINT ( 'NONE',  ( 27.16883889988624290, 33.92500000273118843, 19.73931689729373673 ) ) ;
#21043=CARTESIAN_POINT ( 'NONE',  ( -27.16883889988624290, 15.17500000273119909, -19.73931689729374028 ) ) ;
#21047=CARTESIAN_POINT ( 'NONE',  ( 27.16883889988623935, 74.32500000273117280, -19.73931689729374384 ) ) ;
#21048=DIRECTION ( 'NONE',  ( 0.000000000000000000, 0.000000000000000000, -1.000000000000000000 ) ) ;
#21050=CARTESIAN_POINT ( 'NONE',  ( -23.41746824999999887, 15.52499999726882507, -7.608796670333730638 ) ) ;
#21051=CARTESIAN_POINT ( 'NONE',  ( 27.16883889988623935, 56.32500000273118701, -19.73931689729374384 ) ) ;
#21055=CARTESIAN_POINT ( 'NONE',  ( -20.75514604977248112, 5.425000002731181326, 28.56700777964554661 ) ) ;
#21056=CARTESIAN_POINT ( 'NONE',  ( -7.236395654485763274, 18.52499999726881086, 22.27133577429736633 ) ) ;
#21060=ORIENTED_EDGE ( 'NONE', *, *, #4613, .F. ) ;
#21062=CARTESIAN_POINT ( 'NONE',  ( 20.08610463437157279, 5.300000000000006040, -27.64615127144129758 ) ) ;
#21064=CARTESIAN_POINT ( 'NONE',  ( 10.04305231718579705, 27.10000000546236620, 30.90933677959248982 ) ) ;
#21065=AXIS2_PLACEMENT_3D ( 'NONE', #24850, #19711, #30157 ) ;
#21067=CARTESIAN_POINT ( 'NONE',  ( 7.236395654485755280, 16.22499999726881370, 22.27133577429736988 ) ) ;
#21068=CARTESIAN_POINT ( 'NONE',  ( 33.58253175000000113, 12.47500000273119447, -10.91162601494193751 ) ) ;
#21069=CARTESIAN_POINT ( 'NONE',  ( 6.277390505771533514E-15, 60.49999999999997868, 34.17252228774368916 ) ) ;
#21070=CARTESIAN_POINT ( 'NONE',  ( 4.300734207923761154, 79.47500000273119269, 13.23629886949340495 ) ) ;
#21071=LINE ( 'NONE', #17811, #8821 ) ;
#21073=CARTESIAN_POINT ( 'NONE',  ( -8.601468415847518756, 75.07500000273118701, -11.83890561707634781 ) ) ;
#21076=DIRECTION ( 'NONE',  ( -0.000000000000000000, -1.000000000000000000, -0.000000000000000000 ) ) ;
#21077=CARTESIAN_POINT ( 'NONE',  ( -24.50000000000000711, 13.09999999999999432, 7.960532557706201828 ) ) ;
#21078=CARTESIAN_POINT ( 'NONE',  ( -32.50000000000000000, 3.899999999999992806, -10.55989012756945478 ) ) ;
#21079=CARTESIAN_POINT ( 'NONE',  ( 5.779280353836490358E-15, 41.00000000546237544, 32.49999999999999289 ) ) ;
#21081=CARTESIAN_POINT ( 'NONE',  ( -27.16883889988624290, 50.92500000273120264, -19.73931689729374028 ) ) ;
#21084=CARTESIAN_POINT ( 'NONE',  ( 33.58253175000000113, 32.47500000273117138, -10.91162601494193574 ) ) ;
#21085=CARTESIAN_POINT ( 'NONE',  ( 5.147494310547426899, 25.44874571845316069, -32.50000000000000000 ) ) ;
#21087=CARTESIAN_POINT ( 'NONE',  ( -24.50000000000000000, 8.900000000000011013, -7.960532557706207157 ) ) ;
#21093=CARTESIAN_POINT ( 'NONE',  ( 23.41746824999999887, 0.6249999972688102812, 0.000000000000000000 ) ) ;
#21094=CARTESIAN_POINT ( 'NONE',  ( 7.570916362186207671, 11.59999999999999964, 23.30088464923126779 ) ) ;
#21097=CARTESIAN_POINT ( 'NONE',  ( 24.50000000000000000, 17.84999999453762953, -7.960532557706203605 ) ) ;
#21098=CARTESIAN_POINT ( 'NONE',  ( -33.58253175000000113, 23.12500000273118417, 0.000000000000000000 ) ) ;
#21106=CARTESIAN_POINT ( 'NONE',  ( 23.95873412499999944, 18.31249999863440792, 0.000000000000000000 ) ) ;
#21107=CARTESIAN_POINT ( 'NONE',  ( -10.37757302488623701, 33.77500000273120406, 31.93888565452638417 ) ) ;
#21108=AXIS2_PLACEMENT_3D ( 'NONE', #14073, #11823, #31911 ) ;
#21109=CARTESIAN_POINT ( 'NONE',  ( -10.04305231718578462, 38.90000000546237402, 30.90933677959249337 ) ) ;
#21110=CARTESIAN_POINT ( 'NONE',  ( -20.08610463437156923, 78.29999999999999716, 27.64615127144130113 ) ) ;
#21111=CARTESIAN_POINT ( 'NONE',  ( 5.779280353836490358E-15, 48.50000000000000000, 32.49999999999999289 ) ) ;
#21112=CARTESIAN_POINT ( 'NONE',  ( -15.00000000000000000, 82.00000000000001421, 0.000000000000000000 ) ) ;
#21113=CARTESIAN_POINT ( 'NONE',  ( 6.486482029760649416E-15, 47.87500000273117706, 35.31076352940723240 ) ) ;
#21114=EDGE_CURVE ( 'NONE', #25643, #11416, #13187, .T. ) ;
#21116=CARTESIAN_POINT ( 'NONE',  ( -20.08610463437156923, 24.29999999999999005, 27.64615127144130113 ) ) ;
#21118=CARTESIAN_POINT ( 'NONE',  ( -33.58253175000000113, 67.12500000273119838, 0.000000000000000000 ) ) ;
#21120=CARTESIAN_POINT ( 'NONE',  ( 33.58253175000000113, 54.47500000273117138, -10.91162601494193574 ) ) ;
#21121=EDGE_CURVE ( 'NONE', #32300, #10964, #30186, .T. ) ;
#21123=CARTESIAN_POINT ( 'NONE',  ( -27.16883889988623935, 13.32500000273117990, 19.73931689729374739 ) ) ;
#21136=CARTESIAN_POINT ( 'NONE',  ( 20.08610463437158344, 60.70000000000000284, 27.64615127144129403 ) ) ;
#21138=CARTESIAN_POINT ( 'NONE',  ( -7.236395654485763274, 4.524999997268825069, 22.27133577429736633 ) ) ;
#21139=CARTESIAN_POINT ( 'NONE',  ( 6.277390505771533514E-15, 69.00000000546239676, 34.17252228774368916 ) ) ;
#21143=VERTEX_POINT ( 'NONE', #28142 ) ;
#21147=CARTESIAN_POINT ( 'NONE',  ( 10.04305231718578817, 75.39999999999999147, -30.90933677959249337 ) ) ;
#21148=CARTESIAN_POINT ( 'NONE',  ( 10.37757302488624056, 52.77500000273118985, -31.93888565452638417 ) ) ;
#21149=CARTESIAN_POINT ( 'NONE',  ( 26.29305231718578995, 57.70000000546238539, -19.10302069950538240 ) ) ;
#21151=CARTESIAN_POINT ( 'NONE',  ( -20.75514604977248112, 39.42500000273118843, 28.56700777964554661 ) ) ;
#21152=CARTESIAN_POINT ( 'NONE',  ( 5.147494310547434893, 54.55125428154682510, 32.49999999999999289 ) ) ;
#21153=CARTESIAN_POINT ( 'NONE',  ( -10.37757302488624411, 68.97500000273117848, -31.93888565452638417 ) ) ;
#21154=CARTESIAN_POINT ( 'NONE',  ( 3.980102097228898626E-15, 80.00000000000001421, 32.50000000000000000 ) ) ;
#21158=CARTESIAN_POINT ( 'NONE',  ( -20.08610463437156923, 44.30000000000000426, 27.64615127144130113 ) ) ;
#21160=CARTESIAN_POINT ( 'NONE',  ( -20.75514604977248112, 13.67500000273118133, 28.56700777964554661 ) ) ;
#21161=DIRECTION ( 'NONE',  ( -0.000000000000000000, 1.000000000000000000, -0.000000000000000000 ) ) ;
#21163=CARTESIAN_POINT ( 'NONE',  ( -8.960552108402742093E-16, 72.87500000273115575, -14.63369212191046387 ) ) ;
#21164=CARTESIAN_POINT ( 'NONE',  ( -27.16883889988623935, 77.57500000273121543, 19.73931689729374739 ) ) ;
#21165=CARTESIAN_POINT ( 'NONE',  ( 3.000384657911015469E-15, 0.000000000000000000, -24.50000000000000000 ) ) ;
#21167=ORIENTED_EDGE ( 'NONE', *, *, #17444, .T. ) ;
#21168=DIRECTION ( 'NONE',  ( 0.000000000000000000, 0.000000000000000000, -1.000000000000000000 ) ) ;
#21179=CARTESIAN_POINT ( 'NONE',  ( -27.16883889988623935, 39.32500000273120122, 19.73931689729374739 ) ) ;
#21183=ORIENTED_EDGE ( 'NONE', *, *, #12008, .T. ) ;
#21187=CARTESIAN_POINT ( 'NONE',  ( 20.75514604977248467, 70.67500000273118133, -28.56700777964554305 ) ) ;
#21191=ORIENTED_EDGE ( 'NONE', *, *, #31502, .T. ) ;
#21193=CARTESIAN_POINT ( 'NONE',  ( -20.75514604977248112, 61.42500000273118133, 28.56700777964554661 ) ) ;
#21195=CARTESIAN_POINT ( 'NONE',  ( -10.04305231718578462, 66.90000000546237402, 30.90933677959249337 ) ) ;
#21196=CARTESIAN_POINT ( 'NONE',  ( 14.47279130897151944, 9.424999997268814766, -19.92008829642072598 ) ) ;
#21197=CARTESIAN_POINT ( 'NONE',  ( -10.37757302488623701, 5.525000002731205839, 31.93888565452638417 ) ) ;
#21198=CARTESIAN_POINT ( 'NONE',  ( 10.37757302488624767, 31.97500000273117848, 31.93888565452638417 ) ) ;
#21201=DIRECTION ( 'NONE',  ( -0.000000000000000000, 1.000000000000000000, -0.000000000000000000 ) ) ;
#21206=CARTESIAN_POINT ( 'NONE',  ( -13.91746824999999532, 78.97500000273117848, 4.522059556121122093 ) ) ;
#21208=CARTESIAN_POINT ( 'NONE',  ( -20.75514604977248112, 25.42500000273119198, 28.56700777964554661 ) ) ;
#21211=CARTESIAN_POINT ( 'NONE',  ( 27.16883889988624290, 16.17500000273119909, 19.73931689729373673 ) ) ;
#21214=CARTESIAN_POINT ( 'NONE',  ( 20.75514604977248467, 68.42500000273120975, -28.56700777964554305 ) ) ;
#21215=LINE ( 'NONE', #8818, #32168 ) ;
#21218=LINE ( 'NONE', #5925, #18836 ) ;
#21219=CARTESIAN_POINT ( 'NONE',  ( -27.16883889988623935, 59.32500000273119412, 19.73931689729374739 ) ) ;
#21220=EDGE_CURVE ( 'NONE', #27572, #13970, #27211, .T. ) ;
#21223=ORIENTED_EDGE ( 'NONE', *, *, #846, .F. ) ;
#21225=CARTESIAN_POINT ( 'NONE',  ( -14.47279130897152122, 1.924999997268818541, 19.92008829642072243 ) ) ;
#21227=ORIENTED_EDGE ( 'NONE', *, *, #32716, .T. ) ;
#21235=CARTESIAN_POINT ( 'NONE',  ( -32.50000000000000000, 80.00000000000001421, 0.000000000000000000 ) ) ;
#21237=CARTESIAN_POINT ( 'NONE',  ( 23.41746825000000243, 18.52499999726881441, 7.608796670333735079 ) ) ;
#21238=CARTESIAN_POINT ( 'NONE',  ( 33.58253175000000113, 10.37500000273117173, -4.112674001490185761E-15 ) ) ;
#21239=CARTESIAN_POINT ( 'NONE',  ( -32.50000000000000000, 59.89999999999999858, -10.55989012756945478 ) ) ;
#21240=CARTESIAN_POINT ( 'NONE',  ( -13.91746824999999532, 76.77500000273117564, -4.522059556121115875 ) ) ;
#21241=CARTESIAN_POINT ( 'NONE',  ( 5.779280353836490358E-15, 73.00000000546236834, 32.49999999999999289 ) ) ;
#21243=CARTESIAN_POINT ( 'NONE',  ( 4.300734207923757602, 74.77500000273118985, -13.23629886949340673 ) ) ;
#21246=CARTESIAN_POINT ( 'NONE',  ( 0.000000000000000000, 80.00000000000001421, 0.000000000000000000 ) ) ;
#21247=CARTESIAN_POINT ( 'NONE',  ( 5.147494310547380714, 64.55125428154683220, 32.50000000000002132 ) ) ;
#21248=CARTESIAN_POINT ( 'NONE',  ( 6.277390505771533514E-15, 4.500000000000003553, 34.17252228774368916 ) ) ;
#21249=CARTESIAN_POINT ( 'NONE',  ( -4.635254915624211769, 73.59999999999999432, -14.26584774442730286 ) ) ;
#21251=CARTESIAN_POINT ( 'NONE',  ( 10.37757302488624767, 41.72500000273118559, 31.93888565452638417 ) ) ;
#21254=CARTESIAN_POINT ( 'NONE',  ( 6.486482029760648627E-15, 35.87500000273117706, 35.31076352940722529 ) ) ;
#21261=CARTESIAN_POINT ( 'NONE',  ( -23.41746824999999887, 7.524999997268816188, -7.608796670333730638 ) ) ;
#21262=CARTESIAN_POINT ( 'NONE',  ( -32.50000000000000000, 40.09999999999998721, 10.55989012756946366 ) ) ;
#21266=EDGE_CURVE ( 'NONE', #33755, #15317, #24997, .T. ) ;
#21267=CARTESIAN_POINT ( 'NONE',  ( -32.50000000000000000, 12.09999999999999609, 10.55989012756946366 ) ) ;
#21268=CARTESIAN_POINT ( 'NONE',  ( 20.75514604977248467, 22.42500000273119909, -28.56700777964554305 ) ) ;
#21272=VERTEX_POINT ( 'NONE', #15451 ) ;
#21276=EDGE_CURVE ( 'NONE', #17032, #23750, #28511, .T. ) ;
#21277=ORIENTED_EDGE ( 'NONE', *, *, #28647, .F. ) ;
#21279=CARTESIAN_POINT ( 'NONE',  ( 33.58253175000000823, 26.27500000273119340, 10.91162601494192863 ) ) ;
#21281=CARTESIAN_POINT ( 'NONE',  ( -2.092463501923844636E-15, 38.00000000546237544, -34.17252228774368916 ) ) ;
#21282=CARTESIAN_POINT ( 'NONE',  ( -26.29305231718578995, 76.19999999999998863, 19.10302069950538595 ) ) ;
#21283=CARTESIAN_POINT ( 'NONE',  ( 5.147494310547327423, 52.55125428154685352, 32.50000000000003553 ) ) ;
#21284=CARTESIAN_POINT ( 'NONE',  ( -4.223320258572819786E-15, 5.249999994537622783, 24.50000000000000000 ) ) ;
#21285=CARTESIAN_POINT ( 'NONE',  ( -27.16883889988623935, 43.57500000273117990, 19.73931689729374739 ) ) ;
#21288=CARTESIAN_POINT ( 'NONE',  ( 32.50000000000000000, 21.10000000000000142, -10.55989012756945833 ) ) ;
#21290=CARTESIAN_POINT ( 'NONE',  ( -27.16883889988624290, 64.92500000273118133, -19.73931689729374028 ) ) ;
#21293=CARTESIAN_POINT ( 'NONE',  ( -27.16883889988623935, 55.57500000273118701, 19.73931689729374739 ) ) ;
#21296=CARTESIAN_POINT ( 'NONE',  ( 33.58253175000000113, 14.22500000273119625, -10.91162601494193751 ) ) ;
#21298=CARTESIAN_POINT ( 'NONE',  ( 3.880418787951141812, 2.198745712990784806, -24.50000000000000000 ) ) ;
#21301=CARTESIAN_POINT ( 'NONE',  ( -32.50000000000000000, 18.40000000546238823, -10.55989012756945300 ) ) ;
#21308=CARTESIAN_POINT ( 'NONE',  ( -10.04305231718578462, 66.90000000546237402, 30.90933677959249337 ) ) ;
#21312=ORIENTED_EDGE ( 'NONE', *, *, #15884, .T. ) ;
#21316=CARTESIAN_POINT ( 'NONE',  ( -27.16883889988623935, 51.57500000273118701, 19.73931689729374739 ) ) ;
#21317=CARTESIAN_POINT ( 'NONE',  ( 26.29305231718579350, 57.30000000546237260, 19.10302069950537529 ) ) ;
#21320=CARTESIAN_POINT ( 'NONE',  ( 33.58253175000000113, 38.22500000273119269, -10.91162601494193751 ) ) ;
#21321=CARTESIAN_POINT ( 'NONE',  ( 12.13525491562421088, 73.05000000546237970, 8.816778784387095058 ) ) ;
#21322=CARTESIAN_POINT ( 'NONE',  ( -20.75514604977248823, 61.07500000273119412, -28.56700777964554305 ) ) ;
#21325=CARTESIAN_POINT ( 'NONE',  ( 32.50000000000000000, 41.00000000000000711, -3.980102097228898626E-15 ) ) ;
#21327=CARTESIAN_POINT ( 'NONE',  ( -27.16883889988624290, 11.17500000273119554, -19.73931689729374028 ) ) ;
#21331=CARTESIAN_POINT ( 'NONE',  ( -2.162160676586882350E-15, 74.87500000273116996, -35.31076352940722529 ) ) ;
#21332=DIRECTION ( 'NONE',  ( 0.000000000000000000, 0.000000000000000000, 1.000000000000000000 ) ) ;
#21334=VERTEX_POINT ( 'NONE', #13202 ) ;
#21335=CARTESIAN_POINT ( 'NONE',  ( 1.555960095263670572E-15, 14.24999999453762278, -24.50000000000000000 ) ) ;
#21344=EDGE_CURVE ( 'NONE', #12209, #8211, #7261, .T. ) ;
#21346=CARTESIAN_POINT ( 'NONE',  ( -10.37757302488624411, 36.72500000273118559, -31.93888565452638417 ) ) ;
#21349=CARTESIAN_POINT ( 'NONE',  ( -20.08610463437156923, 2.800000005462385921, 27.64615127144130113 ) ) ;
#21350=ORIENTED_EDGE ( 'NONE', *, *, #10080, .T. ) ;
#21354=CARTESIAN_POINT ( 'NONE',  ( 33.58253175000000113, 66.37500000273119838, -4.112674001490185761E-15 ) ) ;
#21355=ORIENTED_EDGE ( 'NONE', *, *, #11443, .F. ) ;
#21358=ORIENTED_EDGE ( 'NONE', *, *, #757, .F. ) ;
#21360=CARTESIAN_POINT ( 'NONE',  ( 33.58253175000000113, 52.12500000273118417, -4.112674001490185761E-15 ) ) ;
#21362=CARTESIAN_POINT ( 'NONE',  ( 20.08610463437158344, 21.20000000546238894, 27.64615127144129403 ) ) ;
#21364=CARTESIAN_POINT ( 'NONE',  ( 1.507698388325705758E-15, 7.624999997268813168, -24.62258325217400312 ) ) ;
#21365=CARTESIAN_POINT ( 'NONE',  ( 33.58253175000000113, 30.37500000273119127, -4.112674001490185761E-15 ) ) ;
#21368=CARTESIAN_POINT ( 'NONE',  ( -4.934616302121927505E-14, 72.50000000000001421, 32.50000000000000000 ) ) ;
#21369=CARTESIAN_POINT ( 'NONE',  ( 32.50000000000000000, 9.100000000000003197, -10.55989012756945833 ) ) ;
#21373=CARTESIAN_POINT ( 'NONE',  ( -13.91746824999999887, 72.87500000273119838, 0.000000000000000000 ) ) ;
#21375=CARTESIAN_POINT ( 'NONE',  ( -27.16883889988623935, 27.32500000273119412, 19.73931689729374739 ) ) ;
#21378=CARTESIAN_POINT ( 'NONE',  ( 27.16883889988623935, 16.57500000273118346, -19.73931689729374384 ) ) ;
#21380=CARTESIAN_POINT ( 'NONE',  ( -27.16883889988624290, 70.92500000273119554, -19.73931689729374028 ) ) ;
#21381=DIRECTION ( 'NONE',  ( -0.000000000000000000, -1.000000000000000000, -0.000000000000000000 ) ) ;
#21383=CARTESIAN_POINT ( 'NONE',  ( 2.375766604868043697, 78.80125428700924317, 15.00000000000000178 ) ) ;
#21384=CARTESIAN_POINT ( 'NONE',  ( 33.58253175000000113, 58.22500000273117138, -10.91162601494193574 ) ) ;
#21388=CARTESIAN_POINT ( 'NONE',  ( 20.75514604977249178, 1.825000002731179460, 28.56700777964553950 ) ) ;
#21389=CARTESIAN_POINT ( 'NONE',  ( -4.523095164977116484E-15, 4.124999997268806951, 24.62258325217400312 ) ) ;
#21391=VERTEX_POINT ( 'NONE', #10634 ) ;
#21397=CARTESIAN_POINT ( 'NONE',  ( -4.223320258572819786E-15, 19.24999999453763166, 24.50000000000000000 ) ) ;
#21398=CARTESIAN_POINT ( 'NONE',  ( 10.04305231718578817, 27.90000000546238823, -30.90933677959249337 ) ) ;
#21400=CARTESIAN_POINT ( 'NONE',  ( -24.50000000000001066, 1.099999999999994094, 7.960532557706201828 ) ) ;
#21401=CARTESIAN_POINT ( 'NONE',  ( -2.162160676586881955E-15, 8.875000002731189497, -35.31076352940723240 ) ) ;
#21403=CARTESIAN_POINT ( 'NONE',  ( 20.08610463437158344, 58.70000000000000995, 27.64615127144129403 ) ) ;
#21404=CARTESIAN_POINT ( 'NONE',  ( 11.25946833292375793, 77.67500000273119554, 8.180482586598731842 ) ) ;
#21405=CARTESIAN_POINT ( 'NONE',  ( 5.779280353836490358E-15, 55.00000000546238965, 32.49999999999999289 ) ) ;
#21407=CARTESIAN_POINT ( 'NONE',  ( 11.25946833292375793, 76.17500000273119554, 8.180482586598731842 ) ) ;
#21410=LINE ( 'NONE', #5616, #19563 ) ;
#21411=CARTESIAN_POINT ( 'NONE',  ( 6.001560367445586717E-15, 1.500000000000005995, 24.50000000000000000 ) ) ;
#21412=CARTESIAN_POINT ( 'NONE',  ( 32.50000000000000000, 5.000000000000004441, -3.980102097228898626E-15 ) ) ;
#21413=CARTESIAN_POINT ( 'NONE',  ( 20.08610463437158344, 49.20000000546237118, 27.64615127144129403 ) ) ;
#21415=CARTESIAN_POINT ( 'NONE',  ( 33.58253175000000113, 42.22500000273118559, -10.91162601494193751 ) ) ;
#21418=CARTESIAN_POINT ( 'NONE',  ( -33.58253175000000113, 37.37500000273119838, 0.000000000000000000 ) ) ;
#21420=CARTESIAN_POINT ( 'NONE',  ( -4.223320258572821363E-15, 80.50000000000000000, 15.00000000000000355 ) ) ;
#21422=LINE ( 'NONE', #21757, #1520 ) ;
#21423=CARTESIAN_POINT ( 'NONE',  ( 5.147494310547426899, 31.44874571845313582, -32.50000000000000000 ) ) ;
#21424=( BOUNDED_CURVE ( )  B_SPLINE_CURVE ( 2, ( #27034, #939, #14001, #21894, #19321, #14841, #9170, #19654, #22554, #16912, #27540, #1779, #9687 ),
 .UNSPECIFIED., .F., .T. ) 
 B_SPLINE_CURVE_WITH_KNOTS ( ( 3, 2, 2, 2, 2, 2, 3 ),
 ( 0.1089743589743589758, 0.1102564102564102533, 0.1128205128205128221, 0.1153846153846153910, 0.1179487179487179460, 0.1205128205128205149, 0.1217948717948718063 ),
 .UNSPECIFIED. ) 
 CURVE ( )  GEOMETRIC_REPRESENTATION_ITEM ( )  RATIONAL_B_SPLINE_CURVE ( ( 0.9755282581475768211, 0.9755282581475768211, 1.000000000000000000, 0.9510565162951535312, 1.000000000000000000, 0.9510565162951535312, 1.000000000000000000, 0.9510565162951535312, 1.000000000000000000, 0.9510565162951535312, 1.000000000000000000, 0.9755282581475765991, 0.9755282581475767101 ) ) 
 REPRESENTATION_ITEM ( '' )  );
#21427=CARTESIAN_POINT ( 'NONE',  ( 7.236395654485755280, 6.224999997268803931, 22.27133577429736988 ) ) ;
#21428=LINE ( 'NONE', #29962, #2251 ) ;
#21430=CARTESIAN_POINT ( 'NONE',  ( 10.37757302488624056, 20.52500000273119340, -31.93888565452638417 ) ) ;
#21432=VERTEX_POINT ( 'NONE', #15629 ) ;
#21434=ORIENTED_EDGE ( 'NONE', *, *, #32828, .F. ) ;
#21440=CARTESIAN_POINT ( 'NONE',  ( -33.58253175000000113, 25.47500000273118914, 10.91162601494193929 ) ) ;
#21441=CARTESIAN_POINT ( 'NONE',  ( -32.50000000000000000, 32.50000000546238255, 0.000000000000000000 ) ) ;
#21442=EDGE_CURVE ( 'NONE', #17842, #2121, #22592, .T. ) ;
#21443=CARTESIAN_POINT ( 'NONE',  ( -10.04305231718578462, 78.39999999999999147, 30.90933677959249337 ) ) ;
#21445=CARTESIAN_POINT ( 'NONE',  ( 5.779280353836490358E-15, 37.00000000546237544, 32.49999999999999289 ) ) ;
#21446=CARTESIAN_POINT ( 'NONE',  ( 20.75514604977249178, 42.07500000273117990, 28.56700777964553950 ) ) ;
#21448=CARTESIAN_POINT ( 'NONE',  ( -32.50000000000000000, 21.99999999999999289, 0.000000000000000000 ) ) ;
#21450=CARTESIAN_POINT ( 'NONE',  ( -33.58253175000000113, 61.02500000273118985, -10.91162601494193218 ) ) ;
#21451=CARTESIAN_POINT ( 'NONE',  ( -5.147494310547430452, 78.44874571845313938, 32.50000000000000000 ) ) ;
#21452=CARTESIAN_POINT ( 'NONE',  ( -8.446640517145639571E-15, 77.00000000546236834, 32.49999999999999289 ) ) ;
#21453=CARTESIAN_POINT ( 'NONE',  ( 33.58253175000000113, 56.47500000273116427, -10.91162601494193574 ) ) ;
#21455=CARTESIAN_POINT ( 'NONE',  ( 32.50000000000000711, 39.40000000546236691, 10.55989012756945122 ) ) ;
#21456=CARTESIAN_POINT ( 'NONE',  ( -33.58253175000000113, 5.125000002731194826, 0.000000000000000000 ) ) ;
#21458=CYLINDRICAL_SURFACE ( 'NONE', #22842, 32.50000000000000000 ) ;
#21464=CARTESIAN_POINT ( 'NONE',  ( -5.147494310547430452, 58.05125428700922185, -32.49999999999999289 ) ) ;
#21468=CARTESIAN_POINT ( 'NONE',  ( 32.50000000000000711, 48.89999999999999858, 10.55989012756945122 ) ) ;
#21470=CARTESIAN_POINT ( 'NONE',  ( -10.04305231718579172, 70.10000000546237686, -30.90933677959248982 ) ) ;
#21472=CARTESIAN_POINT ( 'NONE',  ( 0.000000000000000000, 80.00000000000001421, 0.000000000000000000 ) ) ;
#21473=ORIENTED_EDGE ( 'NONE', *, *, #18195, .T. ) ;
#21478=CARTESIAN_POINT ( 'NONE',  ( 33.58253175000000113, 46.47500000273118559, -10.91162601494193751 ) ) ;
#21479=CARTESIAN_POINT ( 'NONE',  ( -2.092463501923844636E-15, 56.00000000546236123, -34.17252228774368916 ) ) ;
#21481=CARTESIAN_POINT ( 'NONE',  ( 20.75514604977249178, 35.82500000273117990, 28.56700777964553950 ) ) ;
#21482=DIRECTION ( 'NONE',  ( 0.000000000000000000, 0.000000000000000000, -1.000000000000000000 ) ) ;
#21483=CARTESIAN_POINT ( 'NONE',  ( -33.58253175000000113, 63.37500000273119127, 0.000000000000000000 ) ) ;
#21484=CARTESIAN_POINT ( 'NONE',  ( 20.08610463437158344, 1.200000005462378283, 27.64615127144129403 ) ) ;
#21487=CARTESIAN_POINT ( 'NONE',  ( 10.04305231718578817, 43.39999999999999147, -30.90933677959249337 ) ) ;
#21489=CARTESIAN_POINT ( 'NONE',  ( -20.75514604977248112, 7.675000002731199089, 28.56700777964554661 ) ) ;
#21491=DIRECTION ( 'NONE',  ( 0.8660254037844402619, -0.4999999999999970579, 0.000000000000000000 ) ) ;
#21492=CARTESIAN_POINT ( 'NONE',  ( 10.37757302488624056, 70.77500000273117564, -31.93888565452638417 ) ) ;
#21495=ORIENTED_EDGE ( 'NONE', *, *, #10557, .F. ) ;
#21506=CARTESIAN_POINT ( 'NONE',  ( 20.75514604977249178, 35.82500000273117990, 28.56700777964553950 ) ) ;
#21513=CARTESIAN_POINT ( 'NONE',  ( 26.29305231718578995, 51.19999999999999574, -19.10302069950538240 ) ) ;
#21515=CARTESIAN_POINT ( 'NONE',  ( -27.16883889988624290, 69.17500000273119554, -19.73931689729374028 ) ) ;
#21516=ORIENTED_EDGE ( 'NONE', *, *, #18122, .F. ) ;
#21519=ORIENTED_EDGE ( 'NONE', *, *, #11270, .T. ) ;
#21521=CARTESIAN_POINT ( 'NONE',  ( -32.50000000000000000, 48.50000000546239676, 0.000000000000000000 ) ) ;
#21522=CARTESIAN_POINT ( 'NONE',  ( 20.75514604977248467, 52.42500000273118133, -28.56700777964554305 ) ) ;
#21524=CARTESIAN_POINT ( 'NONE',  ( 26.29305231718579350, 17.30000000546239036, 19.10302069950537529 ) ) ;
#21526=CARTESIAN_POINT ( 'NONE',  ( -14.47279130897151767, 7.824999997268806240, -19.92008829642072598 ) ) ;
#21527=CARTESIAN_POINT ( 'NONE',  ( -2.162160676586881955E-15, 26.87500000273116996, -35.31076352940723240 ) ) ;
#21530=CARTESIAN_POINT ( 'NONE',  ( 11.25946833292375793, 80.07500000273121543, -8.180482586598735395 ) ) ;
#21531=EDGE_CURVE ( 'NONE', #1522, #3647, #15395, .T. ) ;
#21533=ORIENTED_EDGE ( 'NONE', *, *, #3570, .T. ) ;
#21535=CARTESIAN_POINT ( 'NONE',  ( 4.300734207923761154, 75.47500000273119269, 13.23629886949340495 ) ) ;
#21537=CARTESIAN_POINT ( 'NONE',  ( -20.75514604977248823, 24.82500000273117635, -28.56700777964554305 ) ) ;
#21540=CARTESIAN_POINT ( 'NONE',  ( -20.75514604977248823, 15.07500000273116747, -28.56700777964554305 ) ) ;
#21543=CARTESIAN_POINT ( 'NONE',  ( -20.75514604977248112, 71.42500000273119554, 28.56700777964554661 ) ) ;
#21544=EDGE_CURVE ( 'NONE', #16826, #774, #445, .T. ) ;
#21545=DIRECTION ( 'NONE',  ( -0.000000000000000000, 1.000000000000000000, -0.000000000000000000 ) ) ;
#21546=CARTESIAN_POINT ( 'NONE',  ( -13.91746824999999887, 81.37500000273118417, 0.000000000000000000 ) ) ;
#21549=CARTESIAN_POINT ( 'NONE',  ( -4.635254915624211769, 71.85000000546237686, -14.26584774442730286 ) ) ;
#21550=CARTESIAN_POINT ( 'NONE',  ( -33.58253175000000113, 55.12500000273118417, 0.000000000000000000 ) ) ;
#21553=( BOUNDED_SURFACE ( )  B_SPLINE_SURFACE ( 1, 2, ( 
 ( #4758, #30660, #30838, #25181, #2010, #12652, #33768, #18160, #28602, #6989, #15065, #5101, #17640, #15235, #27932, #7330, #4416, #28101, #2179, #23122, #7843, #26380, #26210, #15924, #24146, #13000, #2704, #3044, #13164, #2871, #13516, #18670, #23979, #18332, #13340, #31350, #32020, #5613, #450, #18501, #31522, #28945, #21574, #616, #10424, #10932, #29446, #29109, #10596, #23813, #15587, #278, #21407, #11105, #8516, #18834, #33933, #19002, #105, #5274, #10766, #31686, #8180, #21073, #23641, #16097, #21243, #31853, #29280, #5781, #26548, #8345, #26038, #16261, #26718, #3214, #13682, #2532, #23471, #8016, #20902, #28777, #15756, #5443, #16755, #24472, #32515, #6108, #16921, #1107, #22238, #3376, #6449, #16588, #32190, #1451, #19662, #947, #17089, #1277, #30105 ),
 ( #22400, #6611, #11427, #786, #24969, #19168, #27381, #29771, #3705, #21902, #11930, #27548, #9340, #19329, #8684, #26880, #3870, #29606, #9015, #14343, #32848, #24800, #27044, #11757, #32683, #9178, #19497, #6279, #24634, #3538, #14177, #32354, #22071, #14510, #4035, #19825, #5949, #8848, #29945, #16428, #11592, #13846, #24312, #11268, #14010, #21744, #27214, #27891, #30449, #22915, #6947, #30277, #7287, #15370, #17951, #28230, #12094, #9695, #17771, #25825, #14679, #10046, #27719, #1970, #2315, #22741, #4716, #30619, #9520, #33544, #23261, #4546, #6777, #20175, #15196, #4375, #20344, #23083, #15021, #12788, #33724, #25660, #7115, #22564, #17597, #17430, #28059, #4889, #4207, #14849, #2139, #25315, #25491, #12614, #33371, #20525, #33015, #12445, #20002, #10222, #30794 ) ),
 .UNSPECIFIED., .F., .F., .F. ) 
 B_SPLINE_SURFACE_WITH_KNOTS ( ( 2, 2 ),
 ( 3, 2, 2, 2, 2, 2, 2, 2, 2, 2, 2, 2, 2, 2, 2, 2, 2, 2, 2, 2, 2, 2, 2, 2, 2, 2, 2, 2, 2, 2, 2, 2, 2, 2, 2, 2, 2, 2, 2, 2, 2, 2, 2, 2, 2, 2, 2, 2, 2, 2, 3 ),
 ( 0.000000000000000000, 1.000000000000000000 ),
 ( 0.000000000000000000, 0.02000000000000000042, 0.04000000000000000083, 0.05999999999999999778, 0.08000000000000000167, 0.1000000000000000056, 0.1199999999999999956, 0.1400000000000000133, 0.1600000000000000033, 0.1799999999999999933, 0.2000000000000000111, 0.2200000000000000011, 0.2399999999999999911, 0.2600000000000000089, 0.2800000000000000266, 0.2999999999999999889, 0.3200000000000000067, 0.3400000000000000244, 0.3599999999999999867, 0.3800000000000000044, 0.4000000000000000222, 0.4199999999999999845, 0.4400000000000000022, 0.4600000000000000200, 0.4799999999999999822, 0.5000000000000000000, 0.5200000000000000178, 0.5400000000000000355, 0.5600000000000000533, 0.5799999999999999600, 0.5999999999999999778, 0.6199999999999999956, 0.6400000000000000133, 0.6600000000000000311, 0.6800000000000000488, 0.6999999999999999556, 0.7199999999999999734, 0.7399999999999999911, 0.7600000000000000089, 0.7800000000000000266, 0.8000000000000000444, 0.8199999999999999512, 0.8399999999999999689, 0.8599999999999999867, 0.8800000000000000044, 0.9000000000000000222, 0.9200000000000000400, 0.9399999999999999467, 0.9599999999999999645, 0.9799999999999999822, 1.000000000000000000 ),
 .UNSPECIFIED. ) 
 GEOMETRIC_REPRESENTATION_ITEM ( )  RATIONAL_B_SPLINE_SURFACE ( (
 ( 1.000000000000000000, 0.9510565162951535312, 1.000000000000000000, 0.9510565162951535312, 1.000000000000000000, 0.9510565162951535312, 1.000000000000000000, 0.9510565162951535312, 1.000000000000000000, 0.9510565162951535312, 1.000000000000000000, 0.9510565162951535312, 1.000000000000000000, 0.9510565162951535312, 1.000000000000000000, 0.9510565162951535312, 1.000000000000000000, 0.9510565162951535312, 1.000000000000000000, 0.9510565162951535312, 1.000000000000000000, 0.9510565162951535312, 1.000000000000000000, 0.9510565162951535312, 1.000000000000000000, 0.9510565162951535312, 1.000000000000000000, 0.9510565162951535312, 1.000000000000000000, 0.9510565162951535312, 1.000000000000000000, 0.9510565162951535312, 1.000000000000000000, 0.9510565162951535312, 1.000000000000000000, 0.9510565162951535312, 1.000000000000000000, 0.9510565162951535312, 1.000000000000000000, 0.9510565162951535312, 1.000000000000000000, 0.9510565162951535312, 1.000000000000000000, 0.9510565162951535312, 1.000000000000000000, 0.9510565162951535312, 1.000000000000000000, 0.9510565162951535312, 1.000000000000000000, 0.9510565162951535312, 1.000000000000000000, 0.9510565162951535312, 1.000000000000000000, 0.9510565162951535312, 1.000000000000000000, 0.9510565162951535312, 1.000000000000000000, 0.9510565162951535312, 1.000000000000000000, 0.9510565162951535312, 1.000000000000000000, 0.9510565162951535312, 1.000000000000000000, 0.9510565162951535312, 1.000000000000000000, 0.9510565162951535312, 1.000000000000000000, 0.9510565162951535312, 1.000000000000000000, 0.9510565162951535312, 1.000000000000000000, 0.9510565162951535312, 1.000000000000000000, 0.9510565162951535312, 1.000000000000000000, 0.9510565162951535312, 1.000000000000000000, 0.9510565162951535312, 1.000000000000000000, 0.9510565162951535312, 1.000000000000000000, 0.9510565162951535312, 1.000000000000000000, 0.9510565162951535312, 1.000000000000000000, 0.9510565162951535312, 1.000000000000000000, 0.9510565162951535312, 1.000000000000000000, 0.9510565162951535312, 1.000000000000000000, 0.9510565162951535312, 1.000000000000000000, 0.9510565162951535312, 1.000000000000000000, 0.9510565162951535312, 1.000000000000000000, 0.9510565162951535312, 1.000000000000000000, 0.9510565162951535312, 1.000000000000000000),
 ( 1.000000000000000000, 0.9510565162951535312, 1.000000000000000000, 0.9510565162951535312, 1.000000000000000000, 0.9510565162951535312, 1.000000000000000000, 0.9510565162951535312, 1.000000000000000000, 0.9510565162951535312, 1.000000000000000000, 0.9510565162951535312, 1.000000000000000000, 0.9510565162951535312, 1.000000000000000000, 0.9510565162951535312, 1.000000000000000000, 0.9510565162951535312, 1.000000000000000000, 0.9510565162951535312, 1.000000000000000000, 0.9510565162951535312, 1.000000000000000000, 0.9510565162951535312, 1.000000000000000000, 0.9510565162951535312, 1.000000000000000000, 0.9510565162951535312, 1.000000000000000000, 0.9510565162951535312, 1.000000000000000000, 0.9510565162951535312, 1.000000000000000000, 0.9510565162951535312, 1.000000000000000000, 0.9510565162951535312, 1.000000000000000000, 0.9510565162951535312, 1.000000000000000000, 0.9510565162951535312, 1.000000000000000000, 0.9510565162951535312, 1.000000000000000000, 0.9510565162951535312, 1.000000000000000000, 0.9510565162951535312, 1.000000000000000000, 0.9510565162951535312, 1.000000000000000000, 0.9510565162951535312, 1.000000000000000000, 0.9510565162951535312, 1.000000000000000000, 0.9510565162951535312, 1.000000000000000000, 0.9510565162951535312, 1.000000000000000000, 0.9510565162951535312, 1.000000000000000000, 0.9510565162951535312, 1.000000000000000000, 0.9510565162951535312, 1.000000000000000000, 0.9510565162951535312, 1.000000000000000000, 0.9510565162951535312, 1.000000000000000000, 0.9510565162951535312, 1.000000000000000000, 0.9510565162951535312, 1.000000000000000000, 0.9510565162951535312, 1.000000000000000000, 0.9510565162951535312, 1.000000000000000000, 0.9510565162951535312, 1.000000000000000000, 0.9510565162951535312, 1.000000000000000000, 0.9510565162951535312, 1.000000000000000000, 0.9510565162951535312, 1.000000000000000000, 0.9510565162951535312, 1.000000000000000000, 0.9510565162951535312, 1.000000000000000000, 0.9510565162951535312, 1.000000000000000000, 0.9510565162951535312, 1.000000000000000000, 0.9510565162951535312, 1.000000000000000000, 0.9510565162951535312, 1.000000000000000000, 0.9510565162951535312, 1.000000000000000000, 0.9510565162951535312, 1.000000000000000000, 0.9510565162951535312, 1.000000000000000000) ) ) 
 REPRESENTATION_ITEM ( '' )  SURFACE ( )  );
#21557=CARTESIAN_POINT ( 'NONE',  ( 14.47279130897151589, 4.324999997268801799, 19.92008829642072953 ) ) ;
#21562=ORIENTED_EDGE ( 'NONE', *, *, #18568, .T. ) ;
#21566=CARTESIAN_POINT ( 'NONE',  ( -33.58253175000000113, 73.12500000273119838, 0.000000000000000000 ) ) ;
#21568=CARTESIAN_POINT ( 'NONE',  ( 1.577395562988744260E-15, 8.499999999999992895, -25.76082449383753925 ) ) ;
#21569=CARTESIAN_POINT ( 'NONE',  ( -33.58253175000000113, 11.47500000273119625, 10.91162601494193929 ) ) ;
#21570=CARTESIAN_POINT ( 'NONE',  ( 10.37757302488624767, 17.72500000273119625, 31.93888565452638417 ) ) ;
#21571=CARTESIAN_POINT ( 'NONE',  ( -13.91746824999999887, 76.87500000273116996, 0.000000000000000000 ) ) ;
#21572=CARTESIAN_POINT ( 'NONE',  ( -15.00000000000000000, 72.00000000000001421, 0.000000000000000000 ) ) ;
#21574=CARTESIAN_POINT ( 'NONE',  ( -11.25946833292375793, 77.17500000273119554, -8.180482586598733619 ) ) ;
#21580=CARTESIAN_POINT ( 'NONE',  ( 10.37757302488624767, 45.72500000273119269, 31.93888565452638417 ) ) ;
#21583=CARTESIAN_POINT ( 'NONE',  ( 10.37757302488624767, 33.97500000273117848, 31.93888565452638417 ) ) ;
#21587=CARTESIAN_POINT ( 'NONE',  ( -32.50000000000000000, 44.50000000546238965, 0.000000000000000000 ) ) ;
#21590=CARTESIAN_POINT ( 'NONE',  ( -18.94512977948576093, 3.824999997268818674, 13.76444248337722698 ) ) ;
#21591=FACE_OUTER_BOUND ( 'NONE', #26151, .T. ) ;
#21593=EDGE_CURVE ( 'NONE', #24499, #11893, #29479, .T. ) ;
#21594=CARTESIAN_POINT ( 'NONE',  ( -4.635254915624208216, 76.65000000546237402, 14.26584774442730463 ) ) ;
#21595=CARTESIAN_POINT ( 'NONE',  ( 33.58253175000000113, 20.12500000273118062, -4.112674001490185761E-15 ) ) ;
#21599=ORIENTED_EDGE ( 'NONE', *, *, #14693, .F. ) ;
#21601=ORIENTED_EDGE ( 'NONE', *, *, #27904, .T. ) ;
#21606=CARTESIAN_POINT ( 'NONE',  ( 23.41746825000000243, 0.7249999972688272454, -7.608796670333727974 ) ) ;
#21607=CARTESIAN_POINT ( 'NONE',  ( 27.16883889988624290, 28.17500000273118133, 19.73931689729373673 ) ) ;
#21608=CARTESIAN_POINT ( 'NONE',  ( -10.04305231718578462, 32.90000000546239534, 30.90933677959249337 ) ) ;
#21609=CARTESIAN_POINT ( 'NONE',  ( 20.08610463437157279, 77.30000000000001137, -27.64615127144129758 ) ) ;
#21610=DIRECTION ( 'NONE',  ( 0.000000000000000000, 0.000000000000000000, 1.000000000000000000 ) ) ;
#21611=CARTESIAN_POINT ( 'NONE',  ( -24.50000000000000000, 11.00000000000001066, -3.000384657911015469E-15 ) ) ;
#21612=CARTESIAN_POINT ( 'NONE',  ( -20.75514604977248823, 45.07500000273117990, -28.56700777964554305 ) ) ;
#21613=( BOUNDED_CURVE ( )  B_SPLINE_CURVE ( 2, ( #31141, #7113, #28562, #17595, #15542, #12786, #15019, #10382, #25658, #33722, #1968, #28057, #12443 ),
 .UNSPECIFIED., .F., .T. ) 
 B_SPLINE_CURVE_WITH_KNOTS ( ( 3, 2, 2, 2, 2, 2, 3 ),
 ( 0.2499999999999999722, 0.2555555555555555358, 0.2666666666666666630, 0.2777777777777777901, 0.2888888888888888618, 0.2999999999999999889, 0.3055555555555555802 ),
 .UNSPECIFIED. ) 
 CURVE ( )  GEOMETRIC_REPRESENTATION_ITEM ( )  RATIONAL_B_SPLINE_CURVE ( ( 0.9755282581475768211, 0.9755282581475768211, 1.000000000000000000, 0.9510565162951535312, 1.000000000000000000, 0.9510565162951535312, 1.000000000000000000, 0.9510565162951535312, 1.000000000000000000, 0.9510565162951535312, 1.000000000000000000, 0.9755282581475765991, 0.9755282581475767101 ) ) 
 REPRESENTATION_ITEM ( '' )  );
#21615=CARTESIAN_POINT ( 'NONE',  ( 10.04305231718579705, 20.60000000000000853, 30.90933677959248982 ) ) ;
#21617=( BOUNDED_CURVE ( )  B_SPLINE_CURVE ( 2, ( #10565, #23783, #7814, #250, #33736, #15894, #2326, #2678, #12970, #18132, #79, #20713, #23444 ),
 .UNSPECIFIED., .F., .F. ) 
 B_SPLINE_CURVE_WITH_KNOTS ( ( 3, 2, 2, 2, 2, 2, 3 ),
 ( 0.1987179487179487336, 0.2000000000000000111, 0.2025641025641025661, 0.2051282051282051211, 0.2076923076923077038, 0.2102564102564102588, 0.2115384615384615363 ),
 .UNSPECIFIED. ) 
 CURVE ( )  GEOMETRIC_REPRESENTATION_ITEM ( )  RATIONAL_B_SPLINE_CURVE ( ( 0.9755282581475768211, 0.9755282581475770431, 1.000000000000000000, 0.9510565162951535312, 1.000000000000000000, 0.9510565162951535312, 1.000000000000000000, 0.9510565162951535312, 1.000000000000000000, 0.9510565162951535312, 1.000000000000000000, 0.9755282581475768211, 0.9755282581475768211 ) ) 
 REPRESENTATION_ITEM ( '' )  );
#21618=CARTESIAN_POINT ( 'NONE',  ( -2.162160676586881955E-15, 60.62500000273117706, -35.31076352940723240 ) ) ;
#21620=CARTESIAN_POINT ( 'NONE',  ( 33.58253175000000823, 54.27500000273118985, 10.91162601494192685 ) ) ;
#21623=CARTESIAN_POINT ( 'NONE',  ( -20.75514604977248112, 5.425000002731182214, 28.56700777964554661 ) ) ;
#21629=CARTESIAN_POINT ( 'NONE',  ( 5.779280353836490358E-15, 59.00000000546238255, 32.49999999999999289 ) ) ;
#21630=CARTESIAN_POINT ( 'NONE',  ( 26.29305231718578995, 1.700000005462387609, -19.10302069950538240 ) ) ;
#21633=ADVANCED_FACE ( 'NONE', ( #24350 ), #3411, .T. ) ;
#21635=DIRECTION ( 'NONE',  ( -0.000000000000000000, -1.000000000000000000, -0.000000000000000000 ) ) ;
#21637=ADVANCED_FACE ( 'NONE', ( #29639 ), #6142, .T. ) ;
#21641=ORIENTED_EDGE ( 'NONE', *, *, #24810, .F. ) ;
#21645=CARTESIAN_POINT ( 'NONE',  ( 0.000000000000000000, 82.00000000000001421, -15.00000000000000000 ) ) ;
#21646=CARTESIAN_POINT ( 'NONE',  ( 20.75514604977248467, 46.67500000273118133, -28.56700777964554305 ) ) ;
#21647=CARTESIAN_POINT ( 'NONE',  ( -26.29305231718579350, 50.30000000546236549, -19.10302069950537884 ) ) ;
#21649=CARTESIAN_POINT ( 'NONE',  ( -27.16883889988623935, 35.32500000273120122, 19.73931689729374739 ) ) ;
#21650=CARTESIAN_POINT ( 'NONE',  ( 3.980102097228898626E-15, 80.00000000000001421, 32.50000000000000000 ) ) ;
#21651=CARTESIAN_POINT ( 'NONE',  ( -20.75514604977248823, 63.07500000273119412, -28.56700777964554305 ) ) ;
#21652=FILL_AREA_STYLE_COLOUR ( '', #6871 ) ;
#21653=CARTESIAN_POINT ( 'NONE',  ( 26.29305231718579350, 40.80000000000000426, 19.10302069950537529 ) ) ;
#21655=CARTESIAN_POINT ( 'NONE',  ( 33.58253175000000823, 2.275000002731194293, 10.91162601494192863 ) ) ;
#21656=FACE_OUTER_BOUND ( 'NONE', #13872, .T. ) ;
#21657=CARTESIAN_POINT ( 'NONE',  ( -11.25946833292375793, 75.57500000273120122, 8.180482586598737171 ) ) ;
#21658=CARTESIAN_POINT ( 'NONE',  ( 6.486482029760648627E-15, 73.87500000273119838, 35.31076352940722529 ) ) ;
#21659=CYLINDRICAL_SURFACE ( 'NONE', #25898, 32.50000000000000000 ) ;
#21674=CARTESIAN_POINT ( 'NONE',  ( -33.58253175000000113, 39.02500000273119696, -10.91162601494193041 ) ) ;
#21677=EDGE_CURVE ( 'NONE', #6411, #19947, #3084, .T. ) ;
#21678=CARTESIAN_POINT ( 'NONE',  ( 26.29305231718579350, 13.30000000546238681, 19.10302069950537529 ) ) ;
#21680=ORIENTED_EDGE ( 'NONE', *, *, #14450, .T. ) ;
#21682=FACE_OUTER_BOUND ( 'NONE', #32669, .T. ) ;
#21684=CARTESIAN_POINT ( 'NONE',  ( -10.37757302488624411, 68.97500000273117848, -31.93888565452638417 ) ) ;
#21688=ORIENTED_EDGE ( 'NONE', *, *, #33358, .T. ) ;
#21689=VERTEX_POINT ( 'NONE', #6986 ) ;
#21691=CARTESIAN_POINT ( 'NONE',  ( -20.75514604977248823, 56.82500000273117990, -28.56700777964554305 ) ) ;
#21693=CARTESIAN_POINT ( 'NONE',  ( 10.04305231718579705, 21.10000000546238752, 30.90933677959248982 ) ) ;
#21695=CARTESIAN_POINT ( 'NONE',  ( -23.41746824999999887, 6.124999997268814944, -2.867812753649727150E-15 ) ) ;
#21697=CARTESIAN_POINT ( 'NONE',  ( 10.37757302488624767, 21.97500000273119980, 31.93888565452638417 ) ) ;
#21698=AXIS2_PLACEMENT_3D ( 'NONE', #18249, #31769, #23391 ) ;
#21701=CARTESIAN_POINT ( 'NONE',  ( -8.960552108402742093E-16, 78.37500000273116996, -14.63369212191046387 ) ) ;
#21706=CARTESIAN_POINT ( 'NONE',  ( 2.688165632520823219E-15, 75.37500000273118417, 14.63369212191046387 ) ) ;
#21708=CARTESIAN_POINT ( 'NONE',  ( -20.75514604977248823, 22.82500000273118701, -28.56700777964554305 ) ) ;
#21712=CARTESIAN_POINT ( 'NONE',  ( -2.162160676586882350E-15, 8.875000002731189497, -35.31076352940722529 ) ) ;
#21714=CARTESIAN_POINT ( 'NONE',  ( 33.58253175000000113, 72.22500000273119269, -10.91162601494193574 ) ) ;
#21718=CARTESIAN_POINT ( 'NONE',  ( -13.91746824999999532, 75.47500000273116427, 4.522059556121122093 ) ) ;
#21720=CARTESIAN_POINT ( 'NONE',  ( -9.270509831248423538, 71.95000000546238539, -12.75976212528059861 ) ) ;
#21721=CARTESIAN_POINT ( 'NONE',  ( 33.58253175000000823, 60.02500000273116854, 10.91162601494192685 ) ) ;
#21726=VECTOR ( 'NONE', #13765, 1000.000000000000000 ) ;
#21727=CARTESIAN_POINT ( 'NONE',  ( -23.41746825000000243, 3.524999997268826402, -7.608796670333730638 ) ) ;
#21732=ORIENTED_EDGE ( 'NONE', *, *, #223, .F. ) ;
#21736=CARTESIAN_POINT ( 'NONE',  ( -2.162160676586881955E-15, 74.62500000273116996, -35.31076352940723240 ) ) ;
#21738=CARTESIAN_POINT ( 'NONE',  ( -19.82091636218621034, 6.800000000000000711, -14.40073868116559552 ) ) ;
#21739=CARTESIAN_POINT ( 'NONE',  ( -33.58253175000000113, 11.27500000273117031, -10.91162601494193218 ) ) ;
#21740=CARTESIAN_POINT ( 'NONE',  ( -20.75514604977248823, 18.82500000273119767, -28.56700777964554305 ) ) ;
#21741=CARTESIAN_POINT ( 'NONE',  ( 11.25946833292375793, 76.07500000273120122, -8.180482586598735395 ) ) ;
#21744=CARTESIAN_POINT ( 'NONE',  ( -9.657523855033125146E-16, 77.50000000000000000, -15.77193336357400710 ) ) ;
#21747=CARTESIAN_POINT ( 'NONE',  ( -15.14183272437242778, 9.049999994537618164, 20.84094480462497856 ) ) ;
#21750=CARTESIAN_POINT ( 'NONE',  ( 27.16883889988623935, 46.32500000273117990, -19.73931689729374384 ) ) ;
#21753=CARTESIAN_POINT ( 'NONE',  ( 10.37757302488624767, 31.97500000273117848, 31.93888565452638417 ) ) ;
#21755=CARTESIAN_POINT ( 'NONE',  ( 7.570916362186207671, 17.60000000000000497, 23.30088464923126779 ) ) ;
#21757=CARTESIAN_POINT ( 'NONE',  ( 0.000000000000000000, 82.00000000000001421, -15.00000000000000000 ) ) ;
#21762=CARTESIAN_POINT ( 'NONE',  ( 23.41746824999999887, 4.724999997268818142, -7.608796670333727974 ) ) ;
#21763=VECTOR ( 'NONE', #29390, 1000.000000000000000 ) ;
#21764=CARTESIAN_POINT ( 'NONE',  ( -10.04305231718578462, 52.90000000546238113, 30.90933677959249337 ) ) ;
#21766=DIRECTION ( 'NONE',  ( -0.000000000000000000, -1.000000000000000000, -0.000000000000000000 ) ) ;
#21767=CARTESIAN_POINT ( 'NONE',  ( -33.58253175000000113, 21.22500000273117848, 10.91162601494193929 ) ) ;
#21768=CARTESIAN_POINT ( 'NONE',  ( 14.47279130897151589, 8.824999997268804464, 19.92008829642072953 ) ) ;
#21770=VERTEX_POINT ( 'NONE', #1490 ) ;
#21775=CARTESIAN_POINT ( 'NONE',  ( -4.405589869732278832E-13, 10.49999999999998934, 32.50000000000000000 ) ) ;
#21776=CARTESIAN_POINT ( 'NONE',  ( -18.94512977948576093, 7.824999997268822227, 13.76444248337722698 ) ) ;
#21777=CARTESIAN_POINT ( 'NONE',  ( -27.16883889988624290, 31.17500000273118488, -19.73931689729374028 ) ) ;
#21778=CARTESIAN_POINT ( 'NONE',  ( -2.092463501923844636E-15, 30.00000000546236478, -34.17252228774368916 ) ) ;
#21779=CARTESIAN_POINT ( 'NONE',  ( -32.50000000000000000, 75.89999999999996305, -10.55989012756945478 ) ) ;
#21780=CARTESIAN_POINT ( 'NONE',  ( 26.29305231718578995, 53.19999999999999574, -19.10302069950538240 ) ) ;
#21782=CARTESIAN_POINT ( 'NONE',  ( 6.486482029760649416E-15, 45.87500000273117706, 35.31076352940723240 ) ) ;
#21784=CARTESIAN_POINT ( 'NONE',  ( 26.29305231718578995, 19.19999999999999574, -19.10302069950538240 ) ) ;
#21786=CARTESIAN_POINT ( 'NONE',  ( 27.16883889988623935, 66.32500000273117280, -19.73931689729374384 ) ) ;
#21787=CARTESIAN_POINT ( 'NONE',  ( 33.58253175000000113, 54.37500000273118417, -4.112674001490185761E-15 ) ) ;
#21790=CARTESIAN_POINT ( 'NONE',  ( 10.37757302488624056, 6.525000002731207616, -31.93888565452638417 ) ) ;
#21796=CARTESIAN_POINT ( 'NONE',  ( -20.08610463437156923, 30.80000000546237615, 27.64615127144130113 ) ) ;
#21805=PLANE ( 'NONE',  #14643 ) ;
#21811=CARTESIAN_POINT ( 'NONE',  ( 26.29305231718579350, 20.79999999999998650, 19.10302069950537529 ) ) ;
#21812=CARTESIAN_POINT ( 'NONE',  ( -20.75514604977248112, 47.67500000273118843, 28.56700777964554661 ) ) ;
#21813=CARTESIAN_POINT ( 'NONE',  ( -32.50000000000000000, 50.60000000546236265, 10.55989012756946366 ) ) ;
#21815=CARTESIAN_POINT ( 'NONE',  ( 6.486482029760649416E-15, 35.62500000273119127, 35.31076352940723240 ) ) ;
#21817=CARTESIAN_POINT ( 'NONE',  ( -33.58253175000000113, 63.27500000273118985, -10.91162601494193218 ) ) ;
#21818=DIRECTION ( 'NONE',  ( 1.000000000000000000, 0.000000000000000000, 0.000000000000000000 ) ) ;
#21819=CARTESIAN_POINT ( 'NONE',  ( -26.29305231718579350, 39.80000000000000426, -19.10302069950537884 ) ) ;
#21822=CARTESIAN_POINT ( 'NONE',  ( -33.58253175000000113, 3.375000002731193049, 0.000000000000000000 ) ) ;
#21824=CYLINDRICAL_SURFACE ( 'NONE', #11679, 24.50000000000000000 ) ;
#21825=CARTESIAN_POINT ( 'NONE',  ( -10.37757302488623701, 73.77500000273118985, 31.93888565452638417 ) ) ;
#21826=CARTESIAN_POINT ( 'NONE',  ( 7.890940483122900408E-14, 18.24999999453761745, -24.50000000000000000 ) ) ;
#21829=VERTEX_POINT ( 'NONE', #12827 ) ;
#21830=CARTESIAN_POINT ( 'NONE',  ( -15.14183272437242600, 5.049999994537627934, 20.84094480462497856 ) ) ;
#21831=VECTOR ( 'NONE', #18344, 1000.000000000000114 ) ;
#21844=CARTESIAN_POINT ( 'NONE',  ( -19.82091636218621034, 4.549999994537618164, -14.40073868116559552 ) ) ;
#21849=CARTESIAN_POINT ( 'NONE',  ( -20.75514604977248823, 67.07500000273118701, -28.56700777964554305 ) ) ;
#21850=VERTEX_POINT ( 'NONE', #4927 ) ;
#21853=VERTEX_POINT ( 'NONE', #23119 ) ;
#21854=CARTESIAN_POINT ( 'NONE',  ( 0.000000000000000000, 70.00000000000000000, 0.000000000000000000 ) ) ;
#21855=CARTESIAN_POINT ( 'NONE',  ( 27.16883889988623935, 56.32500000273118701, -19.73931689729374384 ) ) ;
#21857=CARTESIAN_POINT ( 'NONE',  ( -26.29305231718579350, 10.30000000546238326, -19.10302069950537884 ) ) ;
#21858=CARTESIAN_POINT ( 'NONE',  ( 1.093617666956751375E-13, 66.00000000546238255, -32.50000000000000711 ) ) ;
#21859=CARTESIAN_POINT ( 'NONE',  ( 14.47279130897151944, 15.42499999726883075, -19.92008829642072598 ) ) ;
#21860=ADVANCED_FACE ( 'NONE', ( #15754 ), #15407, .F. ) ;
#21861=CARTESIAN_POINT ( 'NONE',  ( -33.58253175000000113, 25.37500000273118417, 0.000000000000000000 ) ) ;
#21862=CARTESIAN_POINT ( 'NONE',  ( -20.08610463437156923, 24.80000000546235839, 27.64615127144130113 ) ) ;
#21864=CARTESIAN_POINT ( 'NONE',  ( 4.300734207923761154, 79.47500000273119269, 13.23629886949340495 ) ) ;
#21866=ORIENTED_EDGE ( 'NONE', *, *, #15625, .T. ) ;
#21868=CARTESIAN_POINT ( 'NONE',  ( 2.688165632520823219E-15, 73.37500000273118417, 14.63369212191046387 ) ) ;
#21870=CARTESIAN_POINT ( 'NONE',  ( 10.37757302488624767, 19.72500000273119625, 31.93888565452638417 ) ) ;
#21874=CARTESIAN_POINT ( 'NONE',  ( -27.16883889988623935, 9.575000002731204773, 19.73931689729374739 ) ) ;
#21877=LINE ( 'NONE', #18975, #30808 ) ;
#21878=CARTESIAN_POINT ( 'NONE',  ( 11.25946833292375793, 78.17500000273119554, 8.180482586598731842 ) ) ;
#21881=CARTESIAN_POINT ( 'NONE',  ( -10.37757302488624411, 48.72500000273119269, -31.93888565452638417 ) ) ;
#21885=CARTESIAN_POINT ( 'NONE',  ( -10.37757302488624411, 2.725000002731181592, -31.93888565452638417 ) ) ;
#21886=CARTESIAN_POINT ( 'NONE',  ( 23.41746825000000243, 6.524999997268818852, 7.608796670333735079 ) ) ;
#21891=EDGE_LOOP ( 'NONE', ( #30602, #17283, #22346, #33042 ) ) ;
#21893=CARTESIAN_POINT ( 'NONE',  ( 33.58253175000000113, 62.47500000273118559, -10.91162601494193751 ) ) ;
#21894=CARTESIAN_POINT ( 'NONE',  ( 20.08610463437157279, 69.80000000546239391, -27.64615127144129758 ) ) ;
#21895=CARTESIAN_POINT ( 'NONE',  ( -33.58253175000000113, 77.02500000273118985, -10.91162601494193218 ) ) ;
#21897=CARTESIAN_POINT ( 'NONE',  ( 24.50000000000000000, 4.000000000000003553, 0.000000000000000000 ) ) ;
#21898=CARTESIAN_POINT ( 'NONE',  ( 33.58253175000000113, 6.375000002731168181, -4.112674001490185761E-15 ) ) ;
#21899=CARTESIAN_POINT ( 'NONE',  ( -33.58253175000000113, 15.02500000273120051, -10.91162601494193218 ) ) ;
#21900=CARTESIAN_POINT ( 'NONE',  ( -8.601468415847518756, 74.57500000273117280, -11.83890561707634603 ) ) ;
#21902=CARTESIAN_POINT ( 'NONE',  ( 15.00000000000000000, 81.09999999999999432, -4.873795443493596835 ) ) ;
#21906=CARTESIAN_POINT ( 'NONE',  ( 10.04305231718579705, 70.59999999999999432, 30.90933677959248982 ) ) ;
#21908=( BOUNDED_CURVE ( )  B_SPLINE_CURVE ( 2, ( #16716, #22030, #23475, #13519, #15928, #454, #13344, #32474, #23816, #19287, #33937, #21247, #10770 ),
 .UNSPECIFIED., .F., .F. ) 
 B_SPLINE_CURVE_WITH_KNOTS ( ( 3, 2, 2, 2, 2, 2, 3 ),
 ( 0.1858974358974359031, 0.1871794871794871806, 0.1897435897435897356, 0.1923076923076923184, 0.1948717948717948734, 0.1974358974358974284, 0.1987179487179487336 ),
 .UNSPECIFIED. ) 
 CURVE ( )  GEOMETRIC_REPRESENTATION_ITEM ( )  RATIONAL_B_SPLINE_CURVE ( ( 0.9755282581475768211, 0.9755282581475768211, 1.000000000000000000, 0.9510565162951535312, 1.000000000000000000, 0.9510565162951535312, 1.000000000000000000, 0.9510565162951535312, 1.000000000000000000, 0.9510565162951535312, 1.000000000000000000, 0.9755282581475764880, 0.9755282581475768211 ) ) 
 REPRESENTATION_ITEM ( '' )  );
#21909=CARTESIAN_POINT ( 'NONE',  ( -10.37757302488624411, 46.72500000273119269, -31.93888565452638417 ) ) ;
#21912=CARTESIAN_POINT ( 'NONE',  ( 20.75514604977248467, 28.67500000273117422, -28.56700777964554305 ) ) ;
#21919=CARTESIAN_POINT ( 'NONE',  ( -23.41746824999999887, 1.624999997268811169, -2.867812753649727150E-15 ) ) ;
#21923=CARTESIAN_POINT ( 'NONE',  ( -2.162160676586882350E-15, 16.62500000273120548, -35.31076352940722529 ) ) ;
#21924=CARTESIAN_POINT ( 'NONE',  ( 7.236395654485755280, 2.724999997268801266, 22.27133577429736988 ) ) ;
#21929=VERTEX_POINT ( 'NONE', #28775 ) ;
#21933=CARTESIAN_POINT ( 'NONE',  ( 15.14183272437242245, 18.04999999453762172, -20.84094480462497856 ) ) ;
#21935=CARTESIAN_POINT ( 'NONE',  ( 23.41746824999999887, 8.624999997268817609, 0.000000000000000000 ) ) ;
#21936=CARTESIAN_POINT ( 'NONE',  ( -33.58253175000000113, 29.37500000273118772, 0.000000000000000000 ) ) ;
#21937=CARTESIAN_POINT ( 'NONE',  ( -2.092463501923844636E-15, 28.00000000546237544, -34.17252228774368916 ) ) ;
#21938=CARTESIAN_POINT ( 'NONE',  ( -2.092463501923844636E-15, 75.50000000000001421, -34.17252228774368916 ) ) ;
#21940=DIRECTION ( 'NONE',  ( -0.000000000000000000, -1.000000000000000000, -0.000000000000000000 ) ) ;
#21942=CARTESIAN_POINT ( 'NONE',  ( 27.16883889988623935, 40.57500000273117280, -19.73931689729374384 ) ) ;
#21943=CARTESIAN_POINT ( 'NONE',  ( 7.236395654485760609, 7.524999997268800200, -22.27133577429736633 ) ) ;
#21944=CARTESIAN_POINT ( 'NONE',  ( -20.08610463437157989, 13.70000000000000462, -27.64615127144129758 ) ) ;
#21947=CARTESIAN_POINT ( 'NONE',  ( -27.16883889988624290, 62.92500000273118843, -19.73931689729374028 ) ) ;
#21948=CARTESIAN_POINT ( 'NONE',  ( -20.75514604977248112, 45.67500000273118843, 28.56700777964554661 ) ) ;
#21950=EDGE_CURVE ( 'NONE', #29891, #27031, #10582, .T. ) ;
#21951=CARTESIAN_POINT ( 'NONE',  ( 5.147494310547434893, 39.05125428700922185, 32.49999999999999289 ) ) ;
#21952=CARTESIAN_POINT ( 'NONE',  ( 27.16883889988624290, 7.925000002731191984, 19.73931689729373673 ) ) ;
#21954=EDGE_CURVE ( 'NONE', #33710, #5395, #7672, .T. ) ;
#21956=CARTESIAN_POINT ( 'NONE',  ( -26.29305231718578995, 20.19999999999999574, 19.10302069950538595 ) ) ;
#21960=CARTESIAN_POINT ( 'NONE',  ( 32.50000000000000000, 1.500000005462381880, -3.980102097228898626E-15 ) ) ;
#21961=ADVANCED_FACE ( 'NONE', ( #31008 ), #2353, .T. ) ;
#21975=CARTESIAN_POINT ( 'NONE',  ( -32.50000000000000000, 46.40000000546237402, -10.55989012756945300 ) ) ;
#21976=CARTESIAN_POINT ( 'NONE',  ( -10.37757302488624411, 44.97500000273119269, -31.93888565452638417 ) ) ;
#21977=CARTESIAN_POINT ( 'NONE',  ( -20.08610463437156923, 52.80000000546237260, 27.64615127144130113 ) ) ;
#21979=CARTESIAN_POINT ( 'NONE',  ( -27.16883889988623935, 33.32500000273120122, 19.73931689729374739 ) ) ;
#21980=CARTESIAN_POINT ( 'NONE',  ( 32.50000000000000000, 77.50000000546236834, -3.980102097228898626E-15 ) ) ;
#21981=CARTESIAN_POINT ( 'NONE',  ( -33.58253175000000113, 61.47500000273117848, 10.91162601494193929 ) ) ;
#21982=( NAMED_UNIT ( * ) PLANE_ANGLE_UNIT ( ) SI_UNIT ( $, .RADIAN. ) );
#21984=CARTESIAN_POINT ( 'NONE',  ( 32.50000000000000000, 43.10000000000000853, -10.55989012756945833 ) ) ;
#21986=CARTESIAN_POINT ( 'NONE',  ( 10.37757302488624767, 5.975000002731184701, 31.93888565452638417 ) ) ;
#21989=CARTESIAN_POINT ( 'NONE',  ( 20.75514604977249178, 74.07500000273120122, 28.56700777964553950 ) ) ;
#21990=CARTESIAN_POINT ( 'NONE',  ( 3.880418787951139592, 3.301254276084478523, 24.50000000000000000 ) ) ;
#21993=CARTESIAN_POINT ( 'NONE',  ( -15.14183272437241889, 4.449999994537617631, -20.84094480462497856 ) ) ;
#22006=FACE_OUTER_BOUND ( 'NONE', #3693, .T. ) ;
#22007=CARTESIAN_POINT ( 'NONE',  ( 26.29305231718578995, 59.20000000000000284, -19.10302069950538240 ) ) ;
#22008=ORIENTED_EDGE ( 'NONE', *, *, #14197, .F. ) ;
#22009=ADVANCED_FACE ( 'NONE', ( #4755 ), #2869, .F. ) ;
#22012=AXIS2_PLACEMENT_3D ( 'NONE', #27755, #22602, #4243 ) ;
#22014=VERTEX_POINT ( 'NONE', #18158 ) ;
#22017=ORIENTED_EDGE ( 'NONE', *, *, #17336, .T. ) ;
#22019=CARTESIAN_POINT ( 'NONE',  ( 32.50000000000000711, 26.89999999999999503, 10.55989012756945122 ) ) ;
#22020=CARTESIAN_POINT ( 'NONE',  ( -20.75514604977248112, 55.42500000273119554, 28.56700777964554661 ) ) ;
#22022=CARTESIAN_POINT ( 'NONE',  ( 10.04305231718578817, 13.90000000546237580, -30.90933677959249337 ) ) ;
#22023=CARTESIAN_POINT ( 'NONE',  ( 24.50000000000000000, 15.64999999453761248, 7.960532557706212486 ) ) ;
#22024=CARTESIAN_POINT ( 'NONE',  ( -7.236395654485757944, 17.72499999726881370, -22.27133577429736988 ) ) ;
#22025=CARTESIAN_POINT ( 'NONE',  ( -26.29305231718579350, 59.79999999999999005, -19.10302069950537884 ) ) ;
#22026=CARTESIAN_POINT ( 'NONE',  ( 27.16883889988623935, 22.57500000273118701, -19.73931689729374384 ) ) ;
#22027=DIRECTION ( 'NONE',  ( -0.000000000000000000, -1.000000000000000000, -0.000000000000000000 ) ) ;
#22029=CARTESIAN_POINT ( 'NONE',  ( -8.601468415847518756, 76.57500000273115859, -11.83890561707634781 ) ) ;
#22030=CARTESIAN_POINT ( 'NONE',  ( 5.147494310547426899, 65.44874571845315359, -32.50000000000000000 ) ) ;
#22031=CARTESIAN_POINT ( 'NONE',  ( 10.04305231718579705, 14.60000000000000142, 30.90933677959248982 ) ) ;
#22033=ORIENTED_EDGE ( 'NONE', *, *, #20351, .T. ) ;
#22035=CARTESIAN_POINT ( 'NONE',  ( -11.25946833292375793, 74.67500000273119554, -8.180482586598733619 ) ) ;
#22037=CARTESIAN_POINT ( 'NONE',  ( 33.58253175000000823, 20.02500000273118275, 10.91162601494192863 ) ) ;
#22041=CARTESIAN_POINT ( 'NONE',  ( 10.37757302488624767, 5.975000002731184701, 31.93888565452638417 ) ) ;
#22045=CARTESIAN_POINT ( 'NONE',  ( -4.300734207923755825, 79.77500000273118985, 13.23629886949340673 ) ) ;
#22048=CARTESIAN_POINT ( 'NONE',  ( -10.37757302488623701, 51.52500000273118985, 31.93888565452638417 ) ) ;
#22050=EDGE_CURVE ( 'NONE', #12770, #31338, #21071, .T. ) ;
#22051=EDGE_LOOP ( 'NONE', ( #33221, #14668, #16372, #7188 ) ) ;
#22053=CARTESIAN_POINT ( 'NONE',  ( 32.50000000000000000, 17.00000000000001421, -3.980102097228898626E-15 ) ) ;
#22054=CARTESIAN_POINT ( 'NONE',  ( 23.41746825000000243, 4.524999997268823293, 7.608796670333735079 ) ) ;
#22056=EDGE_CURVE ( 'NONE', #18611, #27962, #3954, .T. ) ;
#22057=ORIENTED_EDGE ( 'NONE', *, *, #25091, .T. ) ;
#22059=CARTESIAN_POINT ( 'NONE',  ( 24.50000000000000000, 6.100000000000011191, -7.960532557706203605 ) ) ;
#22060=ORIENTED_EDGE ( 'NONE', *, *, #6408, .F. ) ;
#22062=CARTESIAN_POINT ( 'NONE',  ( 6.486482029760649416E-15, 59.87500000273117706, 35.31076352940723240 ) ) ;
#22063=CARTESIAN_POINT ( 'NONE',  ( -15.14183272437242067, 2.700000000000001954, -20.84094480462497856 ) ) ;
#22064=CARTESIAN_POINT ( 'NONE',  ( 33.58253175000000113, 72.22500000273119269, -10.91162601494193751 ) ) ;
#22066=CARTESIAN_POINT ( 'NONE',  ( -15.14183272437242600, 7.300000000000001599, 20.84094480462497856 ) ) ;
#22067=CARTESIAN_POINT ( 'NONE',  ( 10.37757302488624767, 3.975000002731182924, 31.93888565452638417 ) ) ;
#22068=CARTESIAN_POINT ( 'NONE',  ( -10.37757302488623701, 15.52500000273118808, 31.93888565452638417 ) ) ;
#22069=CARTESIAN_POINT ( 'NONE',  ( 13.91746825000000065, 73.77500000273120406, 4.522059556121115875 ) ) ;
#22071=CARTESIAN_POINT ( 'NONE',  ( 12.13525491562421088, 78.80000000000001137, 8.816778784387095058 ) ) ;
#22073=CARTESIAN_POINT ( 'NONE',  ( -7.570916362186210335, 8.349999994537615322, -23.30088464923126779 ) ) ;
#22075=CARTESIAN_POINT ( 'NONE',  ( 10.04305231718578817, 49.90000000546238113, -30.90933677959249337 ) ) ;
#22077=CARTESIAN_POINT ( 'NONE',  ( 20.75514604977248467, 34.42500000273117422, -28.56700777964554305 ) ) ;
#22078=AXIS2_PLACEMENT_3D ( 'NONE', #18552, #20148, #30419 ) ;
#22081=CARTESIAN_POINT ( 'NONE',  ( -33.58253175000000113, 25.27500000273119696, -10.91162601494193041 ) ) ;
#22089=CARTESIAN_POINT ( 'NONE',  ( -23.41746824999999887, 13.62499999726882116, -2.867812753649727150E-15 ) ) ;
#22091=CARTESIAN_POINT ( 'NONE',  ( 7.570916362186213000, 12.39999999999999503, -23.30088464923126423 ) ) ;
#22093=CARTESIAN_POINT ( 'NONE',  ( -2.165007332552593587E-13, 46.50000000000000711, 32.50000000000000000 ) ) ;
#22094=CARTESIAN_POINT ( 'NONE',  ( -33.58253175000000113, 11.02500000273117919, -10.91162601494193041 ) ) ;
#22095=CARTESIAN_POINT ( 'NONE',  ( 23.41746825000000243, 7.224999997268826135, -7.608796670333727974 ) ) ;
#22097=EDGE_LOOP ( 'NONE', ( #30643, #5637, #33535, #15266 ) ) ;
#22100=ORIENTED_EDGE ( 'NONE', *, *, #841, .T. ) ;
#22104=CARTESIAN_POINT ( 'NONE',  ( 15.14183272437242245, 16.04999999453762882, -20.84094480462497856 ) ) ;
#22105=CARTESIAN_POINT ( 'NONE',  ( -7.236395654485757944, 3.224999997268801266, -22.27133577429736988 ) ) ;
#22106=CARTESIAN_POINT ( 'NONE',  ( 6.486482029760649416E-15, 19.87500000273119483, 35.31076352940723240 ) ) ;
#22107=CARTESIAN_POINT ( 'NONE',  ( -2.092463501923844636E-15, 32.00000000546236834, -34.17252228774368916 ) ) ;
#22108=SHAPE_REPRESENTATION ( 'primary mounting nut', ( #1376 ), #16210 ) ;
#22109=CARTESIAN_POINT ( 'NONE',  ( 32.50000000000000711, 70.90000000000000568, 10.55989012756945122 ) ) ;
#22110=CARTESIAN_POINT ( 'NONE',  ( 20.08610463437158344, 33.20000000546238539, 27.64615127144129403 ) ) ;
#22111=CARTESIAN_POINT ( 'NONE',  ( -32.50000000000000000, 1.250000002731177506, 0.000000000000000000 ) ) ;
#22113=CARTESIAN_POINT ( 'NONE',  ( -10.37757302488623701, 33.77500000273120406, 31.93888565452638417 ) ) ;
#22116=CARTESIAN_POINT ( 'NONE',  ( -23.41746825000000243, 10.02499999726882507, -7.608796670333730638 ) ) ;
#22117=CARTESIAN_POINT ( 'NONE',  ( -10.04305231718579172, 13.60000000000000142, -30.90933677959248982 ) ) ;
#22121=CARTESIAN_POINT ( 'NONE',  ( 33.58253175000000823, 54.02500000273118275, 10.91162601494192863 ) ) ;
#22122=CARTESIAN_POINT ( 'NONE',  ( -33.58253175000000113, 47.47500000273119269, 10.91162601494193929 ) ) ;
#22124=CARTESIAN_POINT ( 'NONE',  ( 19.82091636218621034, 9.800000000000002487, 14.40073868116559730 ) ) ;
#22125=CARTESIAN_POINT ( 'NONE',  ( -20.75514604977248823, 4.825000002731171023, -28.56700777964554305 ) ) ;
#22130=CARTESIAN_POINT ( 'NONE',  ( 5.779280353836490358E-15, 20.49999999999999645, 32.49999999999999289 ) ) ;
#22132=VECTOR ( 'NONE', #31329, 1000.000000000000000 ) ;
#22133=CARTESIAN_POINT ( 'NONE',  ( 0.000000000000000000, 82.00000000000001421, 0.000000000000000000 ) ) ;
#22136=SURFACE_SIDE_STYLE ('',( #11652 ) ) ;
#22141=ORIENTED_EDGE ( 'NONE', *, *, #2535, .T. ) ;
#22146=CARTESIAN_POINT ( 'NONE',  ( -26.29305231718578995, 64.70000000546238539, 19.10302069950538595 ) ) ;
#22147=CARTESIAN_POINT ( 'NONE',  ( 10.37757302488624056, 40.77500000273118275, -31.93888565452638417 ) ) ;
#22148=CARTESIAN_POINT ( 'NONE',  ( -32.50000000000000000, 50.40000000546237402, -10.55989012756945478 ) ) ;
#22150=CARTESIAN_POINT ( 'NONE',  ( 27.16883889988623935, 30.32500000273119412, -19.73931689729374384 ) ) ;
#22153=CARTESIAN_POINT ( 'NONE',  ( 20.75514604977248467, 56.67500000273119554, -28.56700777964554305 ) ) ;
#22154=EDGE_CURVE ( 'NONE', #29542, #1522, #13514, .T. ) ;
#22156=CARTESIAN_POINT ( 'NONE',  ( -26.29305231718579350, 33.79999999999999716, -19.10302069950537884 ) ) ;
#22158=CARTESIAN_POINT ( 'NONE',  ( 33.58253175000000113, 4.475000002731183812, -10.91162601494193751 ) ) ;
#22159=CARTESIAN_POINT ( 'NONE',  ( 1.555960095263670572E-15, 14.50000000000000178, -24.50000000000000000 ) ) ;
#22161=CARTESIAN_POINT ( 'NONE',  ( -20.75514604977248112, 69.67500000273119554, 28.56700777964554661 ) ) ;
#22162=CARTESIAN_POINT ( 'NONE',  ( -3.880418787951127602, 4.551254281546843750, -24.50000000000000000 ) ) ;
#22163=ADVANCED_FACE ( 'NONE', ( #16095 ), #24310, .T. ) ;
#22164=ORIENTED_EDGE ( 'NONE', *, *, #11443, .T. ) ;
#22165=CARTESIAN_POINT ( 'NONE',  ( 19.82091636218621034, 5.549999994537619052, 14.40073868116559730 ) ) ;
#22167=CARTESIAN_POINT ( 'NONE',  ( 0.000000000000000000, 80.00000000000001421, -32.50000000000000000 ) ) ;
#22179=ORIENTED_EDGE ( 'NONE', *, *, #5047, .F. ) ;
#22181=CARTESIAN_POINT ( 'NONE',  ( -10.04305231718579172, 75.59999999999999432, -30.90933677959248982 ) ) ;
#22183=ORIENTED_EDGE ( 'NONE', *, *, #30303, .F. ) ;
#22185=VERTEX_POINT ( 'NONE', #1407 ) ;
#22186=ORIENTED_EDGE ( 'NONE', *, *, #16781, .T. ) ;
#22187=CARTESIAN_POINT ( 'NONE',  ( -26.29305231718578995, 56.20000000000000284, 19.10302069950538595 ) ) ;
#22188=CARTESIAN_POINT ( 'NONE',  ( 27.16883889988624290, 49.92500000273120264, 19.73931689729373673 ) ) ;
#22190=CARTESIAN_POINT ( 'NONE',  ( -26.29305231718578995, 14.70000000546237118, 19.10302069950538595 ) ) ;
#22192=CARTESIAN_POINT ( 'NONE',  ( -14.47279130897152299, 18.42499999726882010, 19.92008829642072243 ) ) ;
#22193=VECTOR ( 'NONE', #16117, 1000.000000000000114 ) ;
#22194=CARTESIAN_POINT ( 'NONE',  ( 32.50000000000000711, 52.89999999999999147, 10.55989012756945122 ) ) ;
#22195=CARTESIAN_POINT ( 'NONE',  ( 6.486482029760649416E-15, 25.87500000273117351, 35.31076352940723240 ) ) ;
#22197=CARTESIAN_POINT ( 'NONE',  ( -13.91746824999999887, 74.87500000273116996, 0.000000000000000000 ) ) ;
#22199=CARTESIAN_POINT ( 'NONE',  ( 32.50000000000000000, 15.09999999999998899, -10.55989012756945833 ) ) ;
#22201=VERTEX_POINT ( 'NONE', #16426 ) ;
#22203=CARTESIAN_POINT ( 'NONE',  ( 0.000000000000000000, 80.00000000000001421, 0.000000000000000000 ) ) ;
#22208=CARTESIAN_POINT ( 'NONE',  ( 33.58253175000000113, 8.475000002731173154, -10.91162601494193574 ) ) ;
#22212=CARTESIAN_POINT ( 'NONE',  ( 4.300734207923761154, 79.97500000273119269, 13.23629886949340495 ) ) ;
#22215=CARTESIAN_POINT ( 'NONE',  ( -10.37757302488624411, 50.72500000273119980, -31.93888565452638417 ) ) ;
#22217=VERTEX_POINT ( 'NONE', #16259 ) ;
#22219=CARTESIAN_POINT ( 'NONE',  ( 5.147494310547426899, 43.44874571845313938, -32.50000000000000000 ) ) ;
#22220=CARTESIAN_POINT ( 'NONE',  ( 7.236395654485755280, 14.22499999726881192, 22.27133577429736988 ) ) ;
#22224=CARTESIAN_POINT ( 'NONE',  ( -5.147494310547430452, 34.05125428700920764, -32.49999999999999289 ) ) ;
#22227=CARTESIAN_POINT ( 'NONE',  ( 10.37757302488624767, 59.97500000273120691, 31.93888565452638417 ) ) ;
#22229=CARTESIAN_POINT ( 'NONE',  ( -26.29305231718578995, 36.70000000546236407, 19.10302069950538595 ) ) ;
#22230=CARTESIAN_POINT ( 'NONE',  ( 27.16883889988624290, 71.92500000273119554, 19.73931689729373673 ) ) ;
#22233=CARTESIAN_POINT ( 'NONE',  ( 15.14183272437241889, 7.699999999999988631, 20.84094480462498211 ) ) ;
#22234=CARTESIAN_POINT ( 'NONE',  ( 27.16883889988624290, 4.175000002731188431, 19.73931689729373673 ) ) ;
#22235=CARTESIAN_POINT ( 'NONE',  ( 33.58253175000000113, 14.22500000273119625, -10.91162601494193751 ) ) ;
#22236=CARTESIAN_POINT ( 'NONE',  ( 4.300734207923761154, 73.47500000273119269, 13.23629886949340495 ) ) ;
#22238=CARTESIAN_POINT ( 'NONE',  ( 13.91746824999999887, 72.37500000273119838, -1.704398294459741270E-15 ) ) ;
#22242=CARTESIAN_POINT ( 'NONE',  ( -12.13525491562421088, 80.05000000546236549, -8.816778784387096835 ) ) ;
#22245=CARTESIAN_POINT ( 'NONE',  ( 33.58253175000000113, 36.22500000273119980, -10.91162601494193751 ) ) ;
#22248=CARTESIAN_POINT ( 'NONE',  ( 10.37757302488624767, 29.97500000273117848, 31.93888565452638417 ) ) ;
#22249=CARTESIAN_POINT ( 'NONE',  ( 5.779280353836490358E-15, 8.500000000000000000, 32.49999999999999289 ) ) ;
#22253=CARTESIAN_POINT ( 'NONE',  ( 15.00000000000000000, 81.09999999999999432, -4.873795443493596835 ) ) ;
#22255=CARTESIAN_POINT ( 'NONE',  ( -4.523095164977117273E-15, 12.12499999726881583, 24.62258325217400312 ) ) ;
#22260=CARTESIAN_POINT ( 'NONE',  ( -33.58253175000000113, 13.02500000273117564, -10.91162601494193041 ) ) ;
#22261=CARTESIAN_POINT ( 'NONE',  ( -14.47279130897151589, 3.824999997268816454, -19.92008829642072598 ) ) ;
#22266=ORIENTED_EDGE ( 'NONE', *, *, #17135, .F. ) ;
#22270=CARTESIAN_POINT ( 'NONE',  ( -4.732186688966233175E-15, 17.24999999453762101, 25.76082449383753925 ) ) ;
#22271=CARTESIAN_POINT ( 'NONE',  ( 7.236395654485755280, 6.224999997268803931, 22.27133577429736988 ) ) ;
#22272=CARTESIAN_POINT ( 'NONE',  ( -20.75514604977248823, 23.07500000273117635, -28.56700777964554305 ) ) ;
#22273=CARTESIAN_POINT ( 'NONE',  ( 20.08610463437158344, 25.20000000546237473, 27.64615127144129403 ) ) ;
#22274=CARTESIAN_POINT ( 'NONE',  ( 32.50000000000000000, 75.00000000000001421, -3.980102097228898626E-15 ) ) ;
#22278=CARTESIAN_POINT ( 'NONE',  ( -33.58253175000000113, 33.37500000273119127, 0.000000000000000000 ) ) ;
#22282=CARTESIAN_POINT ( 'NONE',  ( 18.94512977948575738, 8.924999997268812990, 13.76444248337723408 ) ) ;
#22283=CARTESIAN_POINT ( 'NONE',  ( 20.08610463437157279, 15.29999999999998472, -27.64615127144129758 ) ) ;
#22286=CARTESIAN_POINT ( 'NONE',  ( 20.75514604977248467, 58.42500000273119554, -28.56700777964554305 ) ) ;
#22287=CARTESIAN_POINT ( 'NONE',  ( 33.58253175000000823, 50.27500000273118985, 10.91162601494192685 ) ) ;
#22289=CARTESIAN_POINT ( 'NONE',  ( 3.980102097228898626E-15, 80.00000000000001421, 32.50000000000000000 ) ) ;
#22290=CARTESIAN_POINT ( 'NONE',  ( 27.16883889988623935, 2.325000002731170134, -19.73931689729374384 ) ) ;
#22293=CARTESIAN_POINT ( 'NONE',  ( -1.778240108872766143E-15, 41.49999999999999289, -32.49999999999999289 ) ) ;
#22295=DIRECTION ( 'NONE',  ( -0.000000000000000000, -1.000000000000000000, -0.000000000000000000 ) ) ;
#22300=CARTESIAN_POINT ( 'NONE',  ( 26.29305231718579350, 34.79999999999999716, 19.10302069950537529 ) ) ;
#22301=CARTESIAN_POINT ( 'NONE',  ( 20.75514604977248467, 30.42500000273117777, -28.56700777964554305 ) ) ;
#22304=AXIS2_PLACEMENT_3D ( 'NONE', #107, #26551, #31855 ) ;
#22307=VERTEX_POINT ( 'NONE', #21572 ) ;
#22310=VECTOR ( 'NONE', #16527, 1000.000000000000000 ) ;
#22312=FACE_OUTER_BOUND ( 'NONE', #4829, .T. ) ;
#22313=CARTESIAN_POINT ( 'NONE',  ( 33.58253175000000823, 44.27500000273120406, 10.91162601494192863 ) ) ;
#22314=CARTESIAN_POINT ( 'NONE',  ( -10.04305231718579172, 50.10000000546238397, -30.90933677959248982 ) ) ;
#22316=CARTESIAN_POINT ( 'NONE',  ( 33.58253175000000113, 32.22500000273117848, -10.91162601494193751 ) ) ;
#22318=CARTESIAN_POINT ( 'NONE',  ( 33.58253175000000823, 58.27500000273116854, 10.91162601494192863 ) ) ;
#22319=SHAPE_REPRESENTATION_RELATIONSHIP ( 'NONE' , 'NONE' ,  #22108, #11923 ) ;
#22321=CARTESIAN_POINT ( 'NONE',  ( -20.08610463437157989, 31.69999999999998508, -27.64615127144129758 ) ) ;
#22323=CARTESIAN_POINT ( 'NONE',  ( 27.16883889988623935, 74.32500000273117280, -19.73931689729374384 ) ) ;
#22326=CARTESIAN_POINT ( 'NONE',  ( 6.486482029760648627E-15, 69.87500000273121259, 35.31076352940722529 ) ) ;
#22328=CARTESIAN_POINT ( 'NONE',  ( 5.779280353836490358E-15, 41.00000000546237544, 32.49999999999999289 ) ) ;
#22329=CARTESIAN_POINT ( 'NONE',  ( -7.570916362186215665, 3.149999994537633352, 23.30088464923126423 ) ) ;
#22341=CARTESIAN_POINT ( 'NONE',  ( 2.205017735002230837E-13, 57.49999999999999289, -32.50000000000000000 ) ) ;
#22346=ORIENTED_EDGE ( 'NONE', *, *, #14925, .F. ) ;
#22348=VERTEX_POINT ( 'NONE', #21405 ) ;
#22349=CARTESIAN_POINT ( 'NONE',  ( -20.08610463437156923, 74.80000000546236549, 27.64615127144130113 ) ) ;
#22350=CARTESIAN_POINT ( 'NONE',  ( 27.16883889988623935, 50.32500000273118701, -19.73931689729374384 ) ) ;
#22352=CARTESIAN_POINT ( 'NONE',  ( 20.08610463437158344, 13.20000000546237651, 27.64615127144129403 ) ) ;
#22353=CARTESIAN_POINT ( 'NONE',  ( -2.375766604868048137, 78.44874571845313938, 14.99999999999999822 ) ) ;
#22354=CARTESIAN_POINT ( 'NONE',  ( -23.41746824999999887, 16.12499999726882294, -2.867812753649727150E-15 ) ) ;
#22355=CARTESIAN_POINT ( 'NONE',  ( -20.08610463437157989, 51.70000000000000284, -27.64615127144129758 ) ) ;
#22356=DIRECTION ( 'NONE',  ( 0.000000000000000000, 1.000000000000000000, 0.000000000000000000 ) ) ;
#22357=CARTESIAN_POINT ( 'NONE',  ( 33.58253175000000113, 20.37500000273118062, -4.112674001490185761E-15 ) ) ;
#22358=CARTESIAN_POINT ( 'NONE',  ( 5.147494310547434893, 5.051254287009220079, 32.49999999999999289 ) ) ;
#22360=CARTESIAN_POINT ( 'NONE',  ( 8.601468415847516980, 72.17500000273118133, -11.83890561707634781 ) ) ;
#22361=CARTESIAN_POINT ( 'NONE',  ( 9.270509831248421762, 75.55000000546237970, -12.75976212528059861 ) ) ;
#22362=CARTESIAN_POINT ( 'NONE',  ( -26.29305231718579350, 28.30000000546237260, -19.10302069950537884 ) ) ;
#22364=ORIENTED_EDGE ( 'NONE', *, *, #15625, .F. ) ;
#22372=CARTESIAN_POINT ( 'NONE',  ( 27.16883889988623935, 8.575000002731202997, -19.73931689729374384 ) ) ;
#22375=CARTESIAN_POINT ( 'NONE',  ( 8.601468415847520532, 76.07500000273118701, 11.83890561707634603 ) ) ;
#22377=CARTESIAN_POINT ( 'NONE',  ( 32.50000000000000711, 62.89999999999998437, 10.55989012756945122 ) ) ;
#22378=CARTESIAN_POINT ( 'NONE',  ( -20.75514604977248112, 49.42500000273118843, 28.56700777964554661 ) ) ;
#22382=CARTESIAN_POINT ( 'NONE',  ( 0.000000000000000000, 80.00000000000001421, 0.000000000000000000 ) ) ;
#22383=CARTESIAN_POINT ( 'NONE',  ( -18.94512977948575738, 11.42499999726881477, -13.76444248337723231 ) ) ;
#22388=ORIENTED_EDGE ( 'NONE', *, *, #16499, .F. ) ;
#22390=CARTESIAN_POINT ( 'NONE',  ( 6.486482029760649416E-15, 57.87500000273117706, 35.31076352940723240 ) ) ;
#22392=CARTESIAN_POINT ( 'NONE',  ( -33.58253175000000113, 67.12500000273119838, 0.000000000000000000 ) ) ;
#22394=CARTESIAN_POINT ( 'NONE',  ( -24.50000000000001066, 15.09999999999998899, 7.960532557706201828 ) ) ;
#22395=CARTESIAN_POINT ( 'NONE',  ( -27.16883889988624290, 5.175000002731189319, -19.73931689729374028 ) ) ;
#22396=CARTESIAN_POINT ( 'NONE',  ( -33.58253175000000113, 13.02500000273117564, -10.91162601494193218 ) ) ;
#22398=CARTESIAN_POINT ( 'NONE',  ( -11.25946833292375793, 72.67500000273119554, -8.180482586598733619 ) ) ;
#22400=CARTESIAN_POINT ( 'NONE',  ( -15.00000000000000000, 82.00000000000001421, 0.000000000000000000 ) ) ;
#22403=CARTESIAN_POINT ( 'NONE',  ( -15.00000000000000000, 78.35000000546239107, 4.873795443493597723 ) ) ;
#22405=CARTESIAN_POINT ( 'NONE',  ( 27.16883889988623935, 36.32500000273120122, -19.73931689729374384 ) ) ;
#22408=CARTESIAN_POINT ( 'NONE',  ( 33.58253175000000823, 28.27500000273118985, 10.91162601494192685 ) ) ;
#22409=CARTESIAN_POINT ( 'NONE',  ( -26.29305231718578995, 12.70000000546239782, 19.10302069950538595 ) ) ;
#22413=CARTESIAN_POINT ( 'NONE',  ( -7.236395654485763274, 10.02499999726880198, 22.27133577429736633 ) ) ;
#22417=CARTESIAN_POINT ( 'NONE',  ( 20.75514604977248467, 14.42500000273118843, -28.56700777964554305 ) ) ;
#22418=CARTESIAN_POINT ( 'NONE',  ( 7.236395654485755280, 14.72499999726881192, 22.27133577429736988 ) ) ;
#22420=EDGE_LOOP ( 'NONE', ( #2848, #9142, #17846, #18924 ) ) ;
#22423=EDGE_CURVE ( 'NONE', #28216, #771, #31850, .T. ) ;
#22424=EDGE_LOOP ( 'NONE', ( #6263, #19893, #27916 ) ) ;
#22427=FACE_OUTER_BOUND ( 'NONE', #11570, .T. ) ;
#22428=CARTESIAN_POINT ( 'NONE',  ( -7.570916362186215665, 13.14999999453761426, 23.30088464923126423 ) ) ;
#22430=CARTESIAN_POINT ( 'NONE',  ( 18.94512977948576093, 6.824999997268821339, -13.76444248337722875 ) ) ;
#22431=CARTESIAN_POINT ( 'NONE',  ( -2.162160676586881955E-15, 24.87500000273117351, -35.31076352940723240 ) ) ;
#22432=CARTESIAN_POINT ( 'NONE',  ( -10.04305231718578462, 26.90000000546238823, 30.90933677959249337 ) ) ;
#22433=CARTESIAN_POINT ( 'NONE',  ( -20.08610463437157989, 73.70000000000000284, -27.64615127144129758 ) ) ;
#22434=FACE_OUTER_BOUND ( 'NONE', #10158, .T. ) ;
#22437=CARTESIAN_POINT ( 'NONE',  ( 27.16883889988624290, 34.17500000273118843, 19.73931689729373673 ) ) ;
#22441=CARTESIAN_POINT ( 'NONE',  ( -7.236395654485757944, 9.724999997268806595, -22.27133577429736988 ) ) ;
#22442=CARTESIAN_POINT ( 'NONE',  ( 20.08610463437157279, 13.29999999999998650, -27.64615127144129758 ) ) ;
#22444=CARTESIAN_POINT ( 'NONE',  ( 20.75514604977249178, 55.82500000273119412, 28.56700777964553950 ) ) ;
#22445=CARTESIAN_POINT ( 'NONE',  ( 27.16883889988623935, 46.57500000273117990, -19.73931689729374384 ) ) ;
#22446=CARTESIAN_POINT ( 'NONE',  ( 5.147494310547426899, 45.44874571845313938, -32.50000000000000000 ) ) ;
#22447=CARTESIAN_POINT ( 'NONE',  ( 5.147494310547434893, 67.05125428700921475, 32.49999999999999289 ) ) ;
#22448=CARTESIAN_POINT ( 'NONE',  ( -26.29305231718579350, 49.80000000000001137, -19.10302069950537884 ) ) ;
#22451=CARTESIAN_POINT ( 'NONE',  ( 7.570916362186213000, 4.399999999999987033, -23.30088464923126423 ) ) ;
#22454=DIRECTION ( 'NONE',  ( -0.000000000000000000, 1.000000000000000000, -0.000000000000000000 ) ) ;
#22458=CARTESIAN_POINT ( 'NONE',  ( -20.75514604977248823, 34.82500000273118701, -28.56700777964554305 ) ) ;
#22465=ORIENTED_EDGE ( 'NONE', *, *, #22567, .F. ) ;
#22470=EDGE_CURVE ( 'NONE', #26665, #20887, #29444, .T. ) ;
#22472=CARTESIAN_POINT ( 'NONE',  ( 32.50000000000000711, 20.90000000000000924, 10.55989012756945122 ) ) ;
#22473=CARTESIAN_POINT ( 'NONE',  ( 33.58253175000000113, 40.47500000273118559, -10.91162601494193751 ) ) ;
#22474=CARTESIAN_POINT ( 'NONE',  ( -26.29305231718579350, 46.30000000546238681, -19.10302069950537884 ) ) ;
#22476=CARTESIAN_POINT ( 'NONE',  ( 20.75514604977249178, 31.82500000273119056, 28.56700777964553950 ) ) ;
#22477=CARTESIAN_POINT ( 'NONE',  ( 19.82091636218621034, 13.54999999453762527, 14.40073868116559730 ) ) ;
#22478=CARTESIAN_POINT ( 'NONE',  ( 10.37757302488624767, 57.97500000273119980, 31.93888565452638417 ) ) ;
#22480=CARTESIAN_POINT ( 'NONE',  ( -26.29305231718578995, 32.20000000000000284, 19.10302069950538595 ) ) ;
#22482=CARTESIAN_POINT ( 'NONE',  ( 33.58253175000000113, 76.22500000273119269, -10.91162601494193751 ) ) ;
#22485=CARTESIAN_POINT ( 'NONE',  ( 20.75514604977249178, 68.07500000273118701, 28.56700777964553950 ) ) ;
#22487=ORIENTED_EDGE ( 'NONE', *, *, #21593, .T. ) ;
#22488=CARTESIAN_POINT ( 'NONE',  ( -7.570916362186215665, 5.149999994537635573, 23.30088464923126423 ) ) ;
#22490=CARTESIAN_POINT ( 'NONE',  ( 24.50000000000000000, 7.749999994537626336, 0.000000000000000000 ) ) ;
#22494=( BOUNDED_CURVE ( )  B_SPLINE_CURVE ( 2, ( #24851, #9746, #19878, #20232, #30672, #32735, #17483, #27945, #9228, #30331, #19712, #30158, #33946 ),
 .UNSPECIFIED., .F., .T. ) 
 B_SPLINE_CURVE_WITH_KNOTS ( ( 3, 2, 2, 2, 2, 2, 3 ),
 ( 0.9423076923076922906, 0.9435897435897435681, 0.9461538461538461231, 0.9487179487179486781, 0.9512820512820512331, 0.9538461538461538991, 0.9551282051282051766 ),
 .UNSPECIFIED. ) 
 CURVE ( )  GEOMETRIC_REPRESENTATION_ITEM ( )  RATIONAL_B_SPLINE_CURVE ( ( 0.9755282581475768211, 0.9755282581475768211, 1.000000000000000000, 0.9510565162951535312, 1.000000000000000000, 0.9510565162951535312, 1.000000000000000000, 0.9510565162951535312, 1.000000000000000000, 0.9510565162951535312, 1.000000000000000000, 0.9755282581475768211, 0.9755282581475768211 ) ) 
 REPRESENTATION_ITEM ( '' )  );
#22504=CARTESIAN_POINT ( 'NONE',  ( -26.29305231718579350, 75.80000000000001137, -19.10302069950537884 ) ) ;
#22509=CARTESIAN_POINT ( 'NONE',  ( -10.04305231718579172, 60.10000000546239818, -30.90933677959248982 ) ) ;
#22513=CARTESIAN_POINT ( 'NONE',  ( -20.75514604977248112, 47.42500000273118843, 28.56700777964554661 ) ) ;
#22514=CARTESIAN_POINT ( 'NONE',  ( 10.04305231718578817, 55.90000000546238823, -30.90933677959249337 ) ) ;
#22516=CARTESIAN_POINT ( 'NONE',  ( -20.08610463437157989, 10.20000000546238539, -27.64615127144129758 ) ) ;
#22517=DIRECTION ( 'NONE',  ( -0.000000000000000000, 1.000000000000000000, -0.000000000000000000 ) ) ;
#22518=CARTESIAN_POINT ( 'NONE',  ( 18.94512977948575738, 14.92499999726881654, 13.76444248337723408 ) ) ;
#22519=CARTESIAN_POINT ( 'NONE',  ( -20.08610463437157989, 55.69999999999998863, -27.64615127144129758 ) ) ;
#22521=CARTESIAN_POINT ( 'NONE',  ( -27.16883889988623935, 17.57500000273118346, 19.73931689729374739 ) ) ;
#22522=CARTESIAN_POINT ( 'NONE',  ( 10.04305231718579705, 5.100000005462374197, 30.90933677959248982 ) ) ;
#22524=CARTESIAN_POINT ( 'NONE',  ( -4.300734207923755825, 77.27500000273118985, 13.23629886949340673 ) ) ;
#22526=CARTESIAN_POINT ( 'NONE',  ( 20.08610463437158344, 53.20000000546237118, 27.64615127144129403 ) ) ;
#22530=DIRECTION ( 'NONE',  ( -0.000000000000000000, -1.000000000000000000, -0.000000000000000000 ) ) ;
#22536=CARTESIAN_POINT ( 'NONE',  ( 5.779280353836490358E-15, 20.49999999999999645, 32.49999999999999289 ) ) ;
#22539=CARTESIAN_POINT ( 'NONE',  ( 13.91746825000000065, 72.27500000273118985, 4.522059556121115875 ) ) ;
#22541=CARTESIAN_POINT ( 'NONE',  ( -33.58253175000000113, 53.12500000273118417, 0.000000000000000000 ) ) ;
#22544=ORIENTED_EDGE ( 'NONE', *, *, #26245, .T. ) ;
#22546=CARTESIAN_POINT ( 'NONE',  ( 23.41746825000000243, 10.72499999726880127, -7.608796670333727974 ) ) ;
#22550=CARTESIAN_POINT ( 'NONE',  ( 15.14183272437242067, 5.699999999999993960, 20.84094480462498211 ) ) ;
#22553=CARTESIAN_POINT ( 'NONE',  ( 33.58253175000000113, 58.47500000273118559, -10.91162601494193751 ) ) ;
#22554=CARTESIAN_POINT ( 'NONE',  ( 26.29305231718579350, 69.30000000546237970, 19.10302069950537529 ) ) ;
#22555=CARTESIAN_POINT ( 'NONE',  ( -33.58253175000000113, 69.22500000273117848, 10.91162601494193929 ) ) ;
#22557=EDGE_CURVE ( 'NONE', #25888, #27023, #28547, .T. ) ;
#22558=CARTESIAN_POINT ( 'NONE',  ( 7.570916362186207671, 15.60000000000000320, 23.30088464923126779 ) ) ;
#22559=CARTESIAN_POINT ( 'NONE',  ( 33.58253175000000113, 2.475000002731187809, -10.91162601494193751 ) ) ;
#22560=CARTESIAN_POINT ( 'NONE',  ( 10.37757302488624056, 8.525000002731180970, -31.93888565452638417 ) ) ;
#22561=CARTESIAN_POINT ( 'NONE',  ( -13.91746824999999887, 74.87500000273116996, 0.000000000000000000 ) ) ;
#22564=CARTESIAN_POINT ( 'NONE',  ( -9.270509831248425314, 73.70000000000000284, -12.75976212528059861 ) ) ;
#22567=EDGE_CURVE ( 'NONE', #20505, #29467, #32803, .T. ) ;
#22568=CARTESIAN_POINT ( 'NONE',  ( 10.04305231718578817, 23.40000000000000568, -30.90933677959249337 ) ) ;
#22570=CARTESIAN_POINT ( 'NONE',  ( -15.00000000000000000, 78.25000000546239676, 0.000000000000000000 ) ) ;
#22572=CARTESIAN_POINT ( 'NONE',  ( 10.37757302488624056, 38.52500000273118275, -31.93888565452638417 ) ) ;
#22575=CARTESIAN_POINT ( 'NONE',  ( 10.37757302488624767, 25.97500000273117493, 31.93888565452638417 ) ) ;
#22576=CARTESIAN_POINT ( 'NONE',  ( 32.50000000000000711, 40.89999999999998437, 10.55989012756945122 ) ) ;
#22577=EDGE_CURVE ( 'NONE', #5051, #601, #1537, .T. ) ;
#22578=DIRECTION ( 'NONE',  ( -0.000000000000000000, 1.000000000000000000, -0.000000000000000000 ) ) ;
#22579=CARTESIAN_POINT ( 'NONE',  ( -4.405589869732278832E-13, 32.49999999999997868, 32.50000000000000000 ) ) ;
#22581=CARTESIAN_POINT ( 'NONE',  ( 14.47279130897151767, 10.32499999726881335, 19.92008829642072953 ) ) ;
#22586=CARTESIAN_POINT ( 'NONE',  ( -20.75514604977248112, 11.42500000273116711, 28.56700777964554661 ) ) ;
#22587=CARTESIAN_POINT ( 'NONE',  ( 23.41746824999999887, 15.12499999726882294, 0.000000000000000000 ) ) ;
#22589=ORIENTED_EDGE ( 'NONE', *, *, #25382, .F. ) ;
#22592=( BOUNDED_CURVE ( )  B_SPLINE_CURVE ( 2, ( #27251, #29317, #32390, #13715, #16960, #3576, #16296, #822, #8885, #14048, #653, #13884, #13553 ),
 .UNSPECIFIED., .F., .T. ) 
 B_SPLINE_CURVE_WITH_KNOTS ( ( 3, 2, 2, 2, 2, 2, 3 ),
 ( 0.8499999999999999778, 0.8599999999999999867, 0.8800000000000000044, 0.9000000000000000222, 0.9200000000000000400, 0.9399999999999999467, 0.9499999999999999556 ),
 .UNSPECIFIED. ) 
 CURVE ( )  GEOMETRIC_REPRESENTATION_ITEM ( )  RATIONAL_B_SPLINE_CURVE ( ( 0.9755282581475768211, 0.9755282581475768211, 1.000000000000000000, 0.9510565162951535312, 1.000000000000000000, 0.9510565162951535312, 1.000000000000000000, 0.9510565162951535312, 1.000000000000000000, 0.9510565162951535312, 1.000000000000000000, 0.9755282581475768211, 0.9755282581475768211 ) ) 
 REPRESENTATION_ITEM ( '' )  );
#22597=CARTESIAN_POINT ( 'NONE',  ( -15.14183272437241889, 16.44999999453761319, -20.84094480462497856 ) ) ;
#22598=CARTESIAN_POINT ( 'NONE',  ( 23.41746824999999887, 12.62499999726882116, 0.000000000000000000 ) ) ;
#22599=CARTESIAN_POINT ( 'NONE',  ( -10.37757302488624411, 24.97500000273117493, -31.93888565452638417 ) ) ;
#22600=CARTESIAN_POINT ( 'NONE',  ( 32.50000000000000711, 27.40000000546239534, 10.55989012756945122 ) ) ;
#22601=CARTESIAN_POINT ( 'NONE',  ( -2.092463501923844636E-15, 67.50000000000000000, -34.17252228774368916 ) ) ;
#22602=DIRECTION ( 'NONE',  ( -0.000000000000000000, -1.000000000000000000, -0.000000000000000000 ) ) ;
#22605=CARTESIAN_POINT ( 'NONE',  ( 20.75514604977248467, 38.67500000273117422, -28.56700777964554305 ) ) ;
#22606=CARTESIAN_POINT ( 'NONE',  ( -5.147494310547423346, 32.94874572391555034, 32.50000000000000000 ) ) ;
#22611=CARTESIAN_POINT ( 'NONE',  ( 32.50000000000000711, 16.89999999999998437, 10.55989012756945122 ) ) ;
#22612=CARTESIAN_POINT ( 'NONE',  ( -32.50000000000000000, 51.99999999999999289, 0.000000000000000000 ) ) ;
#22614=CARTESIAN_POINT ( 'NONE',  ( 10.37757302488624767, 59.72500000273117848, 31.93888565452638417 ) ) ;
#22616=CARTESIAN_POINT ( 'NONE',  ( -27.16883889988623935, 47.57500000273117990, 19.73931689729374739 ) ) ;
#22617=CARTESIAN_POINT ( 'NONE',  ( 10.04305231718579705, 44.60000000000000142, 30.90933677959248982 ) ) ;
#22618=CARTESIAN_POINT ( 'NONE',  ( 24.50000000000000000, 10.10000000000000142, -7.960532557706203605 ) ) ;
#22619=CARTESIAN_POINT ( 'NONE',  ( -5.147494310547423346, 50.44874571845315359, 32.50000000000000000 ) ) ;
#22621=ADVANCED_FACE ( 'NONE', ( #12744 ), #18072, .F. ) ;
#22623=CARTESIAN_POINT ( 'NONE',  ( 3.880418787951150694, 4.448745718453149145, -24.49999999999999645 ) ) ;
#22627=CARTESIAN_POINT ( 'NONE',  ( 5.779280353836490358E-15, 41.00000000546237544, 32.49999999999999289 ) ) ;
#22630=CARTESIAN_POINT ( 'NONE',  ( 20.08610463437157279, 35.29999999999999716, -27.64615127144129758 ) ) ;
#22632=CARTESIAN_POINT ( 'NONE',  ( -33.58253175000000113, 35.02500000273117564, -10.91162601494193041 ) ) ;
#22633=CARTESIAN_POINT ( 'NONE',  ( 20.75514604977249178, 64.07500000273120122, 28.56700777964553950 ) ) ;
#22635=ORIENTED_EDGE ( 'NONE', *, *, #29784, .T. ) ;
#22640=EDGE_LOOP ( 'NONE', ( #21223, #8459, #26868, #721 ) ) ;
#22645=CARTESIAN_POINT ( 'NONE',  ( -33.58253175000000113, 39.47500000273117848, 10.91162601494193929 ) ) ;
#22646=CARTESIAN_POINT ( 'NONE',  ( 20.08610463437157279, 41.80000000546237260, -27.64615127144129758 ) ) ;
#22648=CARTESIAN_POINT ( 'NONE',  ( -33.58253175000000113, 29.22500000273118914, 10.91162601494193929 ) ) ;
#22649=CARTESIAN_POINT ( 'NONE',  ( 3.880418787951140036, 14.19874571299077637, -24.49999999999999645 ) ) ;
#22650=CARTESIAN_POINT ( 'NONE',  ( -27.16883889988624290, 53.17500000273117422, -19.73931689729374028 ) ) ;
#22652=CARTESIAN_POINT ( 'NONE',  ( 32.50000000000000711, 34.89999999999999858, 10.55989012756945122 ) ) ;
#22654=CARTESIAN_POINT ( 'NONE',  ( 10.37757302488624767, 75.72500000273119269, 31.93888565452638417 ) ) ;
#22655=CARTESIAN_POINT ( 'NONE',  ( 0.000000000000000000, 80.00000000000001421, -32.50000000000000000 ) ) ;
#22657=CARTESIAN_POINT ( 'NONE',  ( -10.37757302488623701, 69.77500000273117564, 31.93888565452638417 ) ) ;
#22660=VERTEX_POINT ( 'NONE', #9824 ) ;
#22661=CARTESIAN_POINT ( 'NONE',  ( 33.58253175000000113, 18.12500000273117706, -4.112674001490185761E-15 ) ) ;
#22662=CARTESIAN_POINT ( 'NONE',  ( -24.50000000000000000, 12.74999999453763166, -3.000384657911015469E-15 ) ) ;
#22664=EDGE_CURVE ( 'NONE', #9328, #24994, #2447, .T. ) ;
#22665=CARTESIAN_POINT ( 'NONE',  ( 5.147494310547327423, 46.55125428154685352, 32.50000000000003553 ) ) ;
#22670=ADVANCED_FACE ( 'NONE', ( #14805 ), #23217, .F. ) ;
#22676=CARTESIAN_POINT ( 'NONE',  ( 20.08610463437157279, 77.80000000546237970, -27.64615127144129758 ) ) ;
#22680=ORIENTED_EDGE ( 'NONE', *, *, #14537, .T. ) ;
#22681=CARTESIAN_POINT ( 'NONE',  ( -33.58253175000000113, 73.47500000273117848, 10.91162601494193929 ) ) ;
#22687=CARTESIAN_POINT ( 'NONE',  ( 32.50000000000000000, 65.50000000546238255, -3.980102097228898626E-15 ) ) ;
#22689=CARTESIAN_POINT ( 'NONE',  ( 10.04305231718579705, 26.60000000000001208, 30.90933677959248982 ) ) ;
#22690=CARTESIAN_POINT ( 'NONE',  ( -33.58253175000000113, 47.12500000273117706, 0.000000000000000000 ) ) ;
#22691=CARTESIAN_POINT ( 'NONE',  ( 2.375766604868043252, 73.69874572391555034, -14.99999999999999822 ) ) ;
#22692=CARTESIAN_POINT ( 'NONE',  ( 6.277390505771533514E-15, 3.000000005462379882, 34.17252228774368916 ) ) ;
#22693=CARTESIAN_POINT ( 'NONE',  ( -15.00000000000000000, 78.10000000000002274, 4.873795443493597723 ) ) ;
#22695=CARTESIAN_POINT ( 'NONE',  ( -32.50000000000000000, 51.89999999999998437, -10.55989012756945478 ) ) ;
#22696=CARTESIAN_POINT ( 'NONE',  ( 0.000000000000000000, 80.00000000000001421, -32.50000000000000000 ) ) ;
#22697=CARTESIAN_POINT ( 'NONE',  ( 10.37757302488624767, 15.97500000273119269, 31.93888565452638417 ) ) ;
#22698=CARTESIAN_POINT ( 'NONE',  ( -7.570916362186210335, 6.599999999999994316, -23.30088464923126779 ) ) ;
#22700=CARTESIAN_POINT ( 'NONE',  ( 4.300734207923761154, 71.47500000273119269, 13.23629886949340495 ) ) ;
#22714=CARTESIAN_POINT ( 'NONE',  ( -10.37757302488623701, 1.775000002731175197, 31.93888565452638417 ) ) ;
#22716=EDGE_CURVE ( 'NONE', #9595, #29888, #23042, .T. ) ;
#22720=CARTESIAN_POINT ( 'NONE',  ( 26.29305231718578995, 69.19999999999998863, -19.10302069950538240 ) ) ;
#22722=CARTESIAN_POINT ( 'NONE',  ( -2.162160676586882350E-15, 46.62500000273119127, -35.31076352940722529 ) ) ;
#22724=CARTESIAN_POINT ( 'NONE',  ( 5.147494310547426899, 21.94874572391553968, -32.50000000000000000 ) ) ;
#22725=VERTEX_POINT ( 'NONE', #15153 ) ;
#22727=FACE_OUTER_BOUND ( 'NONE', #2991, .T. ) ;
#22728=CARTESIAN_POINT ( 'NONE',  ( 18.94512977948576093, 12.82499999726882578, -13.76444248337722875 ) ) ;
#22730=ORIENTED_EDGE ( 'NONE', *, *, #2433, .T. ) ;
#22734=CARTESIAN_POINT ( 'NONE',  ( -5.147494310547430452, 36.05125428700922185, -32.49999999999999289 ) ) ;
#22735=CARTESIAN_POINT ( 'NONE',  ( -2.162160676586881955E-15, 70.62500000273118417, -35.31076352940723240 ) ) ;
#22737=CARTESIAN_POINT ( 'NONE',  ( -7.570916362186210335, 10.59999999999999787, -23.30088464923126779 ) ) ;
#22738=CARTESIAN_POINT ( 'NONE',  ( 7.313012447739250820E-14, 17.24999999453762456, 24.50000000000000000 ) ) ;
#22739=CARTESIAN_POINT ( 'NONE',  ( -20.75514604977248112, 11.42500000273116711, 28.56700777964554661 ) ) ;
#22741=CARTESIAN_POINT ( 'NONE',  ( -9.657523855033125146E-16, 75.50000000000001421, -15.77193336357400710 ) ) ;
#22746=CARTESIAN_POINT ( 'NONE',  ( -9.270509831248421762, 74.55000000546239391, 12.75976212528060039 ) ) ;
#22748=CARTESIAN_POINT ( 'NONE',  ( 27.16883889988624290, 35.92500000273118843, 19.73931689729373673 ) ) ;
#22751=CARTESIAN_POINT ( 'NONE',  ( 20.75514604977248467, 20.67500000273119554, -28.56700777964554305 ) ) ;
#22752=CARTESIAN_POINT ( 'NONE',  ( -7.570916362186210335, 16.34999999453762243, -23.30088464923126779 ) ) ;
#22753=CARTESIAN_POINT ( 'NONE',  ( -26.29305231718578995, 8.700000005462394270, 19.10302069950538595 ) ) ;
#22755=CARTESIAN_POINT ( 'NONE',  ( 10.04305231718579705, 78.60000000000000853, 30.90933677959248982 ) ) ;
#22757=CARTESIAN_POINT ( 'NONE',  ( 23.41746824999999887, 12.52499999726880375, 7.608796670333735079 ) ) ;
#22762=CARTESIAN_POINT ( 'NONE',  ( 6.486482029760648627E-15, 11.62500000273118950, 35.31076352940722529 ) ) ;
#22763=CARTESIAN_POINT ( 'NONE',  ( -14.47279130897152122, 10.42499999726881299, 19.92008829642072243 ) ) ;
#22765=EDGE_LOOP ( 'NONE', ( #28022, #10451, #14538, #15003 ) ) ;
#22768=EDGE_LOOP ( 'NONE', ( #8978, #29469, #12517, #12390 ) ) ;
#22772=CARTESIAN_POINT ( 'NONE',  ( -20.08610463437157989, 72.20000000546237118, -27.64615127144129758 ) ) ;
#22773=CARTESIAN_POINT ( 'NONE',  ( 18.94512977948576093, 5.324999997268820451, -13.76444248337722875 ) ) ;
#22775=CARTESIAN_POINT ( 'NONE',  ( -14.47279130897152122, 9.924999997268825425, 19.92008829642072243 ) ) ;
#22776=CARTESIAN_POINT ( 'NONE',  ( -27.16883889988624290, 19.17500000273120264, -19.73931689729374028 ) ) ;
#22777=CARTESIAN_POINT ( 'NONE',  ( 26.29305231718578995, 25.70000000546238184, -19.10302069950538240 ) ) ;
#22778=CARTESIAN_POINT ( 'NONE',  ( 6.277390505771533514E-15, 64.50000000000000000, 34.17252228774368916 ) ) ;
#22782=CARTESIAN_POINT ( 'NONE',  ( -10.37757302488624411, 34.97500000273118559, -31.93888565452638417 ) ) ;
#22783=CARTESIAN_POINT ( 'NONE',  ( 20.08610463437157279, 43.80000000546236549, -27.64615127144129758 ) ) ;
#22786=CARTESIAN_POINT ( 'NONE',  ( 18.94512977948575738, 16.92499999726882010, 13.76444248337723408 ) ) ;
#22787=CARTESIAN_POINT ( 'NONE',  ( 20.08610463437158344, 8.699999999999986855, 27.64615127144129403 ) ) ;
#22788=CARTESIAN_POINT ( 'NONE',  ( 20.08610463437157279, 9.800000005462367270, -27.64615127144129758 ) ) ;
#22790=CARTESIAN_POINT ( 'NONE',  ( 27.16883889988623935, 54.32500000273118701, -19.73931689729374384 ) ) ;
#22792=CARTESIAN_POINT ( 'NONE',  ( 33.58253175000000113, 40.47500000273117848, -10.91162601494193574 ) ) ;
#22794=DIRECTION ( 'NONE',  ( -0.000000000000000000, -1.000000000000000000, -0.000000000000000000 ) ) ;
#22800=CARTESIAN_POINT ( 'NONE',  ( 10.04305231718578817, 67.40000000000001990, -30.90933677959249337 ) ) ;
#22802=CARTESIAN_POINT ( 'NONE',  ( 0.000000000000000000, 70.00000000000000000, 0.000000000000000000 ) ) ;
#22806=CARTESIAN_POINT ( 'NONE',  ( 33.58253175000000113, 30.22500000273118559, -10.91162601494193574 ) ) ;
#22812=ORIENTED_EDGE ( 'NONE', *, *, #18413, .T. ) ;
#22818=CARTESIAN_POINT ( 'NONE',  ( -27.16883889988623935, 41.57500000273117990, 19.73931689729374739 ) ) ;
#22819=CARTESIAN_POINT ( 'NONE',  ( -10.04305231718579172, 42.10000000546237686, -30.90933677959248982 ) ) ;
#22821=CARTESIAN_POINT ( 'NONE',  ( -2.162160676586881955E-15, 26.62500000273118417, -35.31076352940723240 ) ) ;
#22823=CARTESIAN_POINT ( 'NONE',  ( 6.486482029760649416E-15, 53.87500000273118417, 35.31076352940723240 ) ) ;
#22825=CARTESIAN_POINT ( 'NONE',  ( -32.50000000000000000, 35.90000000000000568, -10.55989012756945478 ) ) ;
#22827=CARTESIAN_POINT ( 'NONE',  ( -20.75514604977248112, 77.42500000273119554, 28.56700777964554661 ) ) ;
#22830=CARTESIAN_POINT ( 'NONE',  ( -20.75514604977248823, 65.07500000273118701, -28.56700777964554305 ) ) ;
#22833=CARTESIAN_POINT ( 'NONE',  ( 6.486482029760649416E-15, 15.62500000273117884, 35.31076352940723240 ) ) ;
#22834=CARTESIAN_POINT ( 'NONE',  ( 24.50000000000000355, 7.849999994537626868, -7.960532557706203605 ) ) ;
#22836=CARTESIAN_POINT ( 'NONE',  ( -32.50000000000000000, 25.89999999999999147, -10.55989012756945300 ) ) ;
#22841=CARTESIAN_POINT ( 'NONE',  ( -4.934616302121927505E-14, 69.00000000546238255, 32.50000000000000000 ) ) ;
#22842=AXIS2_PLACEMENT_3D ( 'NONE', #19217, #19383, #27433 ) ;
#22844=( BOUNDED_CURVE ( )  B_SPLINE_CURVE ( 2, ( #65, #10551, #21032, #20701, #31482, #31308, #8142 ),
 .UNSPECIFIED., .F., .T. ) 
 B_SPLINE_CURVE_WITH_KNOTS ( ( 3, 2, 2, 3 ),
 ( 0.000000000000000000, 0.02000000000000000042, 0.04000000000000000083, 0.05000000000000000971 ),
 .UNSPECIFIED. ) 
 CURVE ( )  GEOMETRIC_REPRESENTATION_ITEM ( )  RATIONAL_B_SPLINE_CURVE ( ( 1.000000000000000000, 0.9510565162951535312, 1.000000000000000000, 0.9510565162951535312, 1.000000000000000000, 0.9755282581475768211, 0.9755282581475768211 ) ) 
 REPRESENTATION_ITEM ( '' )  );
#22848=CARTESIAN_POINT ( 'NONE',  ( -7.236395654485757944, 1.724999997268800156, -22.27133577429736988 ) ) ;
#22850=CARTESIAN_POINT ( 'NONE',  ( 20.08610463437158344, 75.20000000546241381, 27.64615127144129403 ) ) ;
#22855=CARTESIAN_POINT ( 'NONE',  ( 10.37757302488624056, 72.77500000273118985, -31.93888565452638417 ) ) ;
#22858=CARTESIAN_POINT ( 'NONE',  ( -26.29305231718579350, 64.30000000546237970, -19.10302069950537884 ) ) ;
#22859=EDGE_CURVE ( 'NONE', #19899, #23926, #28315, .T. ) ;
#22861=CARTESIAN_POINT ( 'NONE',  ( -26.29305231718579350, 10.30000000546238326, -19.10302069950537884 ) ) ;
#22862=CARTESIAN_POINT ( 'NONE',  ( -20.75514604977248112, 49.42500000273118133, 28.56700777964554661 ) ) ;
#22863=CARTESIAN_POINT ( 'NONE',  ( -18.94512977948575738, 15.42499999726881832, -13.76444248337723231 ) ) ;
#22865=CARTESIAN_POINT ( 'NONE',  ( -2.092463501923844636E-15, 6.000000005462371888, -34.17252228774368916 ) ) ;
#22866=CARTESIAN_POINT ( 'NONE',  ( -5.147494310547423346, 8.448745718453160691, 32.50000000000000000 ) ) ;
#22868=CARTESIAN_POINT ( 'NONE',  ( 32.50000000000000000, 54.99999999999999289, -3.980102097228898626E-15 ) ) ;
#22870=CARTESIAN_POINT ( 'NONE',  ( 10.37757302488624767, 19.97500000273119625, 31.93888565452638417 ) ) ;
#22871=CARTESIAN_POINT ( 'NONE',  ( -19.82091636218621389, 7.200000000000011724, 14.40073868116558842 ) ) ;
#22873=CARTESIAN_POINT ( 'NONE',  ( -4.300734207923759378, 76.97500000273119269, -13.23629886949340495 ) ) ;
#22875=CARTESIAN_POINT ( 'NONE',  ( 10.04305231718579705, 53.10000000546239107, 30.90933677959248982 ) ) ;
#22880=CARTESIAN_POINT ( 'NONE',  ( 2.067204126564591252E-14, 6.249999994537622783, -24.50000000000000000 ) ) ;
#22886=CARTESIAN_POINT ( 'NONE',  ( -20.75514604977248823, 5.075000002731193227, -28.56700777964554305 ) ) ;
#22890=CARTESIAN_POINT ( 'NONE',  ( -11.25946833292375793, 73.17500000273119554, -8.180482586598733619 ) ) ;
#22892=CARTESIAN_POINT ( 'NONE',  ( 20.75514604977248467, 44.42500000273120264, -28.56700777964554305 ) ) ;
#22895=ORIENTED_EDGE ( 'NONE', *, *, #6221, .T. ) ;
#22897=CARTESIAN_POINT ( 'NONE',  ( 32.50000000000000000, 43.10000000000000853, -10.55989012756945833 ) ) ;
#22899=CARTESIAN_POINT ( 'NONE',  ( -20.75514604977248112, 77.67500000273119554, 28.56700777964554661 ) ) ;
#22900=ORIENTED_EDGE ( 'NONE', *, *, #24875, .T. ) ;
#22903=VECTOR ( 'NONE', #22517, 1000.000000000000000 ) ;
#22905=ORIENTED_EDGE ( 'NONE', *, *, #20393, .F. ) ;
#22906=DIRECTION ( 'NONE',  ( 0.000000000000000000, 0.000000000000000000, -1.000000000000000000 ) ) ;
#22907=CARTESIAN_POINT ( 'NONE',  ( -10.37757302488623701, 65.52500000273120406, 31.93888565452638417 ) ) ;
#22910=CARTESIAN_POINT ( 'NONE',  ( -15.14183272437242600, 13.29999999999998650, 20.84094480462497856 ) ) ;
#22911=CARTESIAN_POINT ( 'NONE',  ( -4.523095164977117273E-15, 2.624999997268825602, 24.62258325217400312 ) ) ;
#22912=CARTESIAN_POINT ( 'NONE',  ( 10.37757302488624056, 12.52500000273118452, -31.93888565452638417 ) ) ;
#22913=CARTESIAN_POINT ( 'NONE',  ( 26.29305231718578995, 29.20000000000000284, -19.10302069950538240 ) ) ;
#22915=CARTESIAN_POINT ( 'NONE',  ( 15.00000000000000000, 77.09999999999998010, -4.873795443493596835 ) ) ;
#22918=CARTESIAN_POINT ( 'NONE',  ( -15.00000000000000000, 74.25000000546239676, 0.000000000000000000 ) ) ;
#22920=CARTESIAN_POINT ( 'NONE',  ( 15.00000000000000000, 79.25000000546239676, -1.836970198721029589E-15 ) ) ;
#22922=CARTESIAN_POINT ( 'NONE',  ( -27.16883889988624290, 30.92500000273118488, -19.73931689729374028 ) ) ;
#22925=CARTESIAN_POINT ( 'NONE',  ( 10.37757302488624056, 18.77500000273118985, -31.93888565452638417 ) ) ;
#22926=CARTESIAN_POINT ( 'NONE',  ( 33.58253175000000113, 74.12500000273119838, -4.112674001490185761E-15 ) ) ;
#22927=AXIS2_PLACEMENT_3D ( 'NONE', #19836, #22578, #17102 ) ;
#22928=CARTESIAN_POINT ( 'NONE',  ( 15.00000000000000355, 80.89999999999997726, 4.873795443493592394 ) ) ;
#22930=CARTESIAN_POINT ( 'NONE',  ( 0.000000000000000000, 80.00000000000001421, 0.000000000000000000 ) ) ;
#22931=CARTESIAN_POINT ( 'NONE',  ( 6.486482029760648627E-15, 63.62500000273117706, 35.31076352940722529 ) ) ;
#22935=CARTESIAN_POINT ( 'NONE',  ( 33.58253175000000113, 4.225000002731190918, -10.91162601494193574 ) ) ;
#22936=CARTESIAN_POINT ( 'NONE',  ( -7.236395654485763274, 10.52499999726880198, 22.27133577429736633 ) ) ;
#22941=ORIENTED_EDGE ( 'NONE', *, *, #8724, .T. ) ;
#22946=CARTESIAN_POINT ( 'NONE',  ( 1.507698388325705758E-15, 3.624999997268822938, -24.62258325217400312 ) ) ;
#22947=CARTESIAN_POINT ( 'NONE',  ( -7.236395654485757944, 13.22499999726881015, -22.27133577429736988 ) ) ;
#22948=CARTESIAN_POINT ( 'NONE',  ( 20.75514604977248467, 18.67500000273120264, -28.56700777964554305 ) ) ;
#22949=CARTESIAN_POINT ( 'NONE',  ( 32.50000000000000000, 23.50000000546237544, -3.980102097228898626E-15 ) ) ;
#22950=CARTESIAN_POINT ( 'NONE',  ( 26.29305231718578995, 67.19999999999998863, -19.10302069950538240 ) ) ;
#22951=CARTESIAN_POINT ( 'NONE',  ( 2.375766604868043252, 77.69874572391552192, -14.99999999999999822 ) ) ;
#22954=CARTESIAN_POINT ( 'NONE',  ( -10.37757302488624411, 26.97500000273117493, -31.93888565452638417 ) ) ;
#22955=CARTESIAN_POINT ( 'NONE',  ( 32.50000000000000000, 43.50000000546238965, -3.980102097228898626E-15 ) ) ;
#22958=CARTESIAN_POINT ( 'NONE',  ( 14.47279130897151767, 17.42499999726882365, -19.92008829642072598 ) ) ;
#22959=CARTESIAN_POINT ( 'NONE',  ( -20.08610463437157989, 7.699999999999988631, -27.64615127144129758 ) ) ;
#22962=CARTESIAN_POINT ( 'NONE',  ( 20.75514604977249178, 47.82500000273117990, 28.56700777964553950 ) ) ;
#22964=CARTESIAN_POINT ( 'NONE',  ( -33.58253175000000113, 43.27500000273117564, -10.91162601494193041 ) ) ;
#22965=CYLINDRICAL_SURFACE ( 'NONE', #17839, 32.50000000000000000 ) ;
#22966=CARTESIAN_POINT ( 'NONE',  ( -14.45873412499999944, 81.68750000136559208, 0.000000000000000000 ) ) ;
#22967=LINE ( 'NONE', #9923, #23477 ) ;
#22969=CARTESIAN_POINT ( 'NONE',  ( 4.445600272181915325E-13, 27.50000000000000355, -32.50000000000000000 ) ) ;
#22971=CARTESIAN_POINT ( 'NONE',  ( -20.08610463437157989, 62.20000000546237118, -27.64615127144129758 ) ) ;
#22973=DIRECTION ( 'NONE',  ( 0.000000000000000000, -1.000000000000000000, 0.000000000000000000 ) ) ;
#22976=CARTESIAN_POINT ( 'NONE',  ( 9.270509831248421762, 71.55000000546239391, -12.75976212528059861 ) ) ;
#22977=CARTESIAN_POINT ( 'NONE',  ( 20.75514604977248467, 34.42500000273116711, -28.56700777964554305 ) ) ;
#22978=CARTESIAN_POINT ( 'NONE',  ( 27.16883889988623935, 64.57500000273120122, -19.73931689729374384 ) ) ;
#22983=CARTESIAN_POINT ( 'NONE',  ( -32.50000000000000000, 16.40000000546239178, -10.55989012756945300 ) ) ;
#22987=ORIENTED_EDGE ( 'NONE', *, *, #22423, .T. ) ;
#22991=CARTESIAN_POINT ( 'NONE',  ( -20.75514604977248112, 31.67500000273119909, 28.56700777964554661 ) ) ;
#22992=CARTESIAN_POINT ( 'NONE',  ( -32.50000000000000000, 44.50000000546238965, 0.000000000000000000 ) ) ;
#22994=CARTESIAN_POINT ( 'NONE',  ( -10.37757302488623701, 25.52500000273119696, 31.93888565452638417 ) ) ;
#22995=CARTESIAN_POINT ( 'NONE',  ( -1.778240108872766143E-15, 32.00000000546237544, -32.49999999999999289 ) ) ;
#22996=CARTESIAN_POINT ( 'NONE',  ( 10.37757302488624056, 48.77500000273118985, -31.93888565452638417 ) ) ;
#22998=EDGE_CURVE ( 'NONE', #7660, #18399, #1333, .T. ) ;
#23000=CARTESIAN_POINT ( 'NONE',  ( -20.08610463437157989, 25.70000000000000284, -27.64615127144129758 ) ) ;
#23002=CARTESIAN_POINT ( 'NONE',  ( -2.162160676586881955E-15, 74.62500000273116996, -35.31076352940723240 ) ) ;
#23003=CARTESIAN_POINT ( 'NONE',  ( -5.147494310547430452, 70.05125428700921475, -32.49999999999999289 ) ) ;
#23004=CARTESIAN_POINT ( 'NONE',  ( -15.14183272437242778, 15.30000000000001137, 20.84094480462497856 ) ) ;
#23005=CARTESIAN_POINT ( 'NONE',  ( -10.37757302488623701, 59.77500000273119696, 31.93888565452638417 ) ) ;
#23007=EDGE_CURVE ( 'NONE', #22660, #1605, #27006, .T. ) ;
#23008=ADVANCED_FACE ( 'NONE', ( #25537 ), #2016, .T. ) ;
#23010=CARTESIAN_POINT ( 'NONE',  ( 27.16883889988624290, 17.92500000273117422, 19.73931689729373673 ) ) ;
#23011=CARTESIAN_POINT ( 'NONE',  ( 1.577395562988744260E-15, 10.24999999453763877, -25.76082449383753925 ) ) ;
#23013=( BOUNDED_CURVE ( )  B_SPLINE_CURVE ( 2, ( #26056, #30675, #17829, #20235, #20755, #13016, #4943, #5290, #10440, #15079, #20401, #15772, #22969 ),
 .UNSPECIFIED., .F., .T. ) 
 B_SPLINE_CURVE_WITH_KNOTS ( ( 3, 2, 2, 2, 2, 2, 3 ),
 ( 0.6602564102564102422, 0.6615384615384615197, 0.6641025641025640747, 0.6666666666666666297, 0.6692307692307691847, 0.6717948717948717396, 0.6730769230769231282 ),
 .UNSPECIFIED. ) 
 CURVE ( )  GEOMETRIC_REPRESENTATION_ITEM ( )  RATIONAL_B_SPLINE_CURVE ( ( 0.9755282581475768211, 0.9755282581475768211, 1.000000000000000000, 0.9510565162951535312, 1.000000000000000000, 0.9510565162951535312, 1.000000000000000000, 0.9510565162951535312, 1.000000000000000000, 0.9510565162951535312, 1.000000000000000000, 0.9755282581475757109, 0.9755282581475768211 ) ) 
 REPRESENTATION_ITEM ( '' )  );
#23024=CYLINDRICAL_SURFACE ( 'NONE', #24185, 32.50000000000000000 ) ;
#23025=CARTESIAN_POINT ( 'NONE',  ( -27.16883889988623935, 1.325000002731169246, 19.73931689729374739 ) ) ;
#23026=DIRECTION ( 'NONE',  ( -0.000000000000000000, 1.000000000000000000, -0.000000000000000000 ) ) ;
#23029=VERTEX_POINT ( 'NONE', #20572 ) ;
#23030=CARTESIAN_POINT ( 'NONE',  ( 27.16883889988623935, 74.57500000273120122, -19.73931689729374384 ) ) ;
#23033=CARTESIAN_POINT ( 'NONE',  ( 26.29305231718579350, 61.30000000546237260, 19.10302069950537529 ) ) ;
#23035=CARTESIAN_POINT ( 'NONE',  ( -32.50000000000000000, 10.50000000546236123, 0.000000000000000000 ) ) ;
#23036=CARTESIAN_POINT ( 'NONE',  ( 6.486482029760649416E-15, 39.62500000273117706, 35.31076352940723240 ) ) ;
#23037=CARTESIAN_POINT ( 'NONE',  ( 0.000000000000000000, 80.00000000000001421, 0.000000000000000000 ) ) ;
#23038=CARTESIAN_POINT ( 'NONE',  ( 20.08610463437158344, 5.200000005462368513, 27.64615127144129403 ) ) ;
#23039=CARTESIAN_POINT ( 'NONE',  ( -1.778240108872766143E-15, 7.500000000000001776, -32.49999999999999289 ) ) ;
#23041=CARTESIAN_POINT ( 'NONE',  ( 32.50000000000000000, 49.09999999999999432, -10.55989012756945833 ) ) ;
#23042=LINE ( 'NONE', #22696, #13785 ) ;
#23043=CARTESIAN_POINT ( 'NONE',  ( 33.58253175000000823, 18.27500000273118275, 10.91162601494192863 ) ) ;
#23044=CARTESIAN_POINT ( 'NONE',  ( -24.50000000000000000, 7.000000000000006217, -3.000384657911015469E-15 ) ) ;
#23046=CARTESIAN_POINT ( 'NONE',  ( 4.300734207923757602, 78.77500000273118985, -13.23629886949340673 ) ) ;
#23047=CARTESIAN_POINT ( 'NONE',  ( 0.000000000000000000, 80.00000000000001421, 0.000000000000000000 ) ) ;
#23049=ORIENTED_EDGE ( 'NONE', *, *, #17973, .T. ) ;
#23061=CARTESIAN_POINT ( 'NONE',  ( 4.300734207923761154, 73.97500000273119269, 13.23629886949340495 ) ) ;
#23063=CARTESIAN_POINT ( 'NONE',  ( 33.58253175000000113, 48.12500000273117706, -4.112674001490185761E-15 ) ) ;
#23068=CARTESIAN_POINT ( 'NONE',  ( -32.50000000000000000, 4.600000005462387520, 10.55989012756946366 ) ) ;
#23070=CARTESIAN_POINT ( 'NONE',  ( 20.75514604977249178, 78.07500000273117280, 28.56700777964553950 ) ) ;
#23075=CARTESIAN_POINT ( 'NONE',  ( 20.08610463437158344, 29.20000000546237118, 27.64615127144129403 ) ) ;
#23076=CARTESIAN_POINT ( 'NONE',  ( 10.37757302488624056, 68.52500000273120406, -31.93888565452638417 ) ) ;
#23078=CARTESIAN_POINT ( 'NONE',  ( 1.577395562988744260E-15, 14.50000000000000888, -25.76082449383753925 ) ) ;
#23080=CARTESIAN_POINT ( 'NONE',  ( -27.16883889988623935, 11.32500000273117813, 19.73931689729374739 ) ) ;
#23083=CARTESIAN_POINT ( 'NONE',  ( -9.270509831248421762, 74.30000000000001137, 12.75976212528060039 ) ) ;
#23086=CARTESIAN_POINT ( 'NONE',  ( -9.657523855033125146E-16, 71.75000000546239676, -15.77193336357400710 ) ) ;
#23088=CARTESIAN_POINT ( 'NONE',  ( 33.58253175000000113, 28.12500000273118772, -4.112674001490185761E-15 ) ) ;
#23092=CARTESIAN_POINT ( 'NONE',  ( -27.16883889988623935, 19.57500000273118701, 19.73931689729374739 ) ) ;
#23093=CARTESIAN_POINT ( 'NONE',  ( -24.50000000000000000, 16.74999999453763522, -3.000384657911015469E-15 ) ) ;
#23094=CARTESIAN_POINT ( 'NONE',  ( 33.58253175000000823, 78.02500000273118985, 10.91162601494192685 ) ) ;
#23095=EDGE_CURVE ( 'NONE', #33570, #26901, #18908, .T. ) ;
#23096=CARTESIAN_POINT ( 'NONE',  ( 4.023268246324634798E-14, 8.499999999999992895, -24.50000000000000355 ) ) ;
#23098=CARTESIAN_POINT ( 'NONE',  ( -1.778240108872766143E-15, 52.00000000546237544, -32.49999999999999289 ) ) ;
#23099=CARTESIAN_POINT ( 'NONE',  ( -2.162160676586882350E-15, 64.62500000273121259, -35.31076352940722529 ) ) ;
#23103=CARTESIAN_POINT ( 'NONE',  ( -33.58253175000000113, 9.225000002731178483, 10.91162601494193929 ) ) ;
#23104=CARTESIAN_POINT ( 'NONE',  ( 18.94512977948575738, 12.92499999726881654, 13.76444248337723408 ) ) ;
#23114=CARTESIAN_POINT ( 'NONE',  ( 24.50000000000000355, 19.64999999453763024, 7.960532557706212486 ) ) ;
#23115=CARTESIAN_POINT ( 'NONE',  ( -18.94512977948575738, 13.42499999726881654, -13.76444248337723231 ) ) ;
#23116=CARTESIAN_POINT ( 'NONE',  ( -2.162160676586881955E-15, 14.87500000273120193, -35.31076352940723240 ) ) ;
#23117=CARTESIAN_POINT ( 'NONE',  ( -26.29305231718579350, 20.30000000546239391, -19.10302069950537884 ) ) ;
#23118=CARTESIAN_POINT ( 'NONE',  ( -2.092463501923844636E-15, 65.49999999999998579, -34.17252228774368916 ) ) ;
#23119=CARTESIAN_POINT ( 'NONE',  ( 5.779280353836490358E-15, 24.50000000000000711, 32.49999999999999289 ) ) ;
#23121=CARTESIAN_POINT ( 'NONE',  ( 27.16883889988624290, 30.17500000273118488, 19.73931689729373673 ) ) ;
#23122=CARTESIAN_POINT ( 'NONE',  ( -13.91746824999999532, 79.47500000273117848, 4.522059556121122093 ) ) ;
#23125=CARTESIAN_POINT ( 'NONE',  ( -23.41746824999999887, 16.12499999726882294, -2.867812753649727150E-15 ) ) ;
#23126=CARTESIAN_POINT ( 'NONE',  ( 32.50000000000000000, 11.09999999999999964, -10.55989012756945833 ) ) ;
#23127=CARTESIAN_POINT ( 'NONE',  ( -20.08610463437156923, 52.30000000000000426, 27.64615127144130113 ) ) ;
#23129=CARTESIAN_POINT ( 'NONE',  ( -33.58253175000000113, 53.02500000273118985, -10.91162601494193218 ) ) ;
#23131=CARTESIAN_POINT ( 'NONE',  ( -27.16883889988623935, 41.57500000273117990, 19.73931689729374739 ) ) ;
#23134=CARTESIAN_POINT ( 'NONE',  ( 5.147494310547426899, 15.94874572391552903, -32.50000000000000000 ) ) ;
#23135=CARTESIAN_POINT ( 'NONE',  ( 32.50000000000000000, 51.50000000546239676, -3.980102097228898626E-15 ) ) ;
#23140=CYLINDRICAL_SURFACE ( 'NONE', #12666, 32.50000000000000000 ) ;
#23142=EDGE_CURVE ( 'NONE', #1179, #17842, #26115, .T. ) ;
#23145=CARTESIAN_POINT ( 'NONE',  ( 33.58253175000000113, 28.12500000273118772, -4.112674001490185761E-15 ) ) ;
#23146=CARTESIAN_POINT ( 'NONE',  ( 27.16883889988624290, 66.17500000273118133, 19.73931689729373673 ) ) ;
#23148=VERTEX_POINT ( 'NONE', #23648 ) ;
#23155=AXIS2_PLACEMENT_3D ( 'NONE', #22802, #22973, #12153 ) ;
#23161=CARTESIAN_POINT ( 'NONE',  ( -2.162160676586881955E-15, 36.87500000273116996, -35.31076352940723240 ) ) ;
#23162=CARTESIAN_POINT ( 'NONE',  ( -10.04305231718578462, 42.90000000546237402, 30.90933677959249337 ) ) ;
#23163=ADVANCED_FACE ( 'NONE', ( #12834 ), #10265, .T. ) ;
#23166=CARTESIAN_POINT ( 'NONE',  ( 27.16883889988623935, 24.32500000273119056, -19.73931689729374384 ) ) ;
#23168=CARTESIAN_POINT ( 'NONE',  ( -33.58253175000000113, 49.37500000273120548, 0.000000000000000000 ) ) ;
#23171=CARTESIAN_POINT ( 'NONE',  ( 10.04305231718578817, 25.40000000000000568, -30.90933677959249337 ) ) ;
#23173=CARTESIAN_POINT ( 'NONE',  ( 6.486482029760649416E-15, 71.62500000273119838, 35.31076352940723240 ) ) ;
#23175=CARTESIAN_POINT ( 'NONE',  ( -5.147494310547423346, 20.94874572391552547, 32.50000000000000000 ) ) ;
#23176=CARTESIAN_POINT ( 'NONE',  ( 27.16883889988624290, 60.17500000273118133, 19.73931689729373673 ) ) ;
#23178=CARTESIAN_POINT ( 'NONE',  ( 26.29305231718578995, 7.700000005462392494, -19.10302069950538240 ) ) ;
#23179=CARTESIAN_POINT ( 'NONE',  ( -33.58253175000000113, 9.025000002731184523, -10.91162601494193218 ) ) ;
#23180=CARTESIAN_POINT ( 'NONE',  ( 15.14183272437242245, 12.04999999453764126, -20.84094480462497856 ) ) ;
#23183=VECTOR ( 'NONE', #29657, 1000.000000000000000 ) ;
#23185=FACE_OUTER_BOUND ( 'NONE', #9044, .T. ) ;
#23186=CARTESIAN_POINT ( 'NONE',  ( 32.50000000000000000, 19.10000000000000497, -10.55989012756945833 ) ) ;
#23191=CARTESIAN_POINT ( 'NONE',  ( -24.50000000000000711, 2.849999994537638859, 7.960532557706201828 ) ) ;
#23193=CARTESIAN_POINT ( 'NONE',  ( 5.779280353836490358E-15, 54.49999999999999289, 32.49999999999999289 ) ) ;
#23194=CARTESIAN_POINT ( 'NONE',  ( -26.29305231718578995, 74.70000000546239960, 19.10302069950538595 ) ) ;
#23198=EDGE_LOOP ( 'NONE', ( #15436, #23587 ) ) ;
#23199=CARTESIAN_POINT ( 'NONE',  ( 27.16883889988624290, 76.17500000273119554, 19.73931689729373673 ) ) ;
#23204=CARTESIAN_POINT ( 'NONE',  ( -10.37757302488624411, 56.97500000273119980, -31.93888565452638417 ) ) ;
#23205=CARTESIAN_POINT ( 'NONE',  ( 32.50000000000000000, 61.60000000546236976, -10.55989012756945833 ) ) ;
#23207=CARTESIAN_POINT ( 'NONE',  ( -3.880418787951104953, 13.19874571299077459, 24.50000000000000711 ) ) ;
#23208=CARTESIAN_POINT ( 'NONE',  ( 6.486482029760649416E-15, 43.62500000273116285, 35.31076352940723240 ) ) ;
#23209=CARTESIAN_POINT ( 'NONE',  ( -4.523095164977116484E-15, 18.12499999726880517, 24.62258325217400312 ) ) ;
#23210=CARTESIAN_POINT ( 'NONE',  ( 6.486482029760649416E-15, 65.87500000273119838, 35.31076352940723240 ) ) ;
#23211=CARTESIAN_POINT ( 'NONE',  ( -2.092463501923844636E-15, 8.000000005462366559, -34.17252228774368916 ) ) ;
#23216=CARTESIAN_POINT ( 'NONE',  ( -26.29305231718578995, 48.19999999999999574, 19.10302069950538595 ) ) ;
#23217=CYLINDRICAL_SURFACE ( 'NONE', #75, 15.00000000000000000 ) ;
#23219=CARTESIAN_POINT ( 'NONE',  ( -10.37757302488623701, 11.77500000273118452, 31.93888565452638417 ) ) ;
#23220=CARTESIAN_POINT ( 'NONE',  ( -10.04305231718579172, 73.59999999999999432, -30.90933677959248982 ) ) ;
#23222=CARTESIAN_POINT ( 'NONE',  ( -13.91746824999999532, 70.97500000273116427, 4.522059556121122093 ) ) ;
#23223=CARTESIAN_POINT ( 'NONE',  ( -10.37757302488624411, 76.97500000273119269, -31.93888565452638417 ) ) ;
#23234=UNCERTAINTY_MEASURE_WITH_UNIT (LENGTH_MEASURE( 1.000000000000000082E-05 ), #9258, 'distance_accuracy_value', 'NONE');
#23238=CARTESIAN_POINT ( 'NONE',  ( -10.04305231718579172, 56.10000000546239107, -30.90933677959248982 ) ) ;
#23240=CARTESIAN_POINT ( 'NONE',  ( -10.37757302488623701, 47.52500000273118985, 31.93888565452638417 ) ) ;
#23243=CARTESIAN_POINT ( 'NONE',  ( 4.635254915624209993, 79.39999999999999147, -14.26584774442730463 ) ) ;
#23246=CARTESIAN_POINT ( 'NONE',  ( 3.000384657911015469E-15, 0.000000000000000000, -24.50000000000000000 ) ) ;
#23248=CARTESIAN_POINT ( 'NONE',  ( -20.75514604977248823, 73.07500000273115859, -28.56700777964554305 ) ) ;
#23249=ORIENTED_EDGE ( 'NONE', *, *, #28032, .T. ) ;
#23252=VERTEX_POINT ( 'NONE', #21079 ) ;
#23254=CARTESIAN_POINT ( 'NONE',  ( -27.16883889988623935, 63.32500000273119412, 19.73931689729374739 ) ) ;
#23257=CARTESIAN_POINT ( 'NONE',  ( -4.523095164977117273E-15, 4.624999997268820273, 24.62258325217400312 ) ) ;
#23258=CARTESIAN_POINT ( 'NONE',  ( 33.58253175000000113, 6.225000002731185589, -10.91162601494193751 ) ) ;
#23261=CARTESIAN_POINT ( 'NONE',  ( 15.00000000000000000, 75.00000000000001421, -1.836970198721029589E-15 ) ) ;
#23264=CYLINDRICAL_SURFACE ( 'NONE', #16668, 32.50000000000000000 ) ;
#23267=CARTESIAN_POINT ( 'NONE',  ( 4.635254915624209993, 71.65000000546240244, -14.26584774442730463 ) ) ;
#23269=CARTESIAN_POINT ( 'NONE',  ( -33.58253175000000113, 29.12500000273118772, 0.000000000000000000 ) ) ;
#23272=CARTESIAN_POINT ( 'NONE',  ( -33.58253175000000113, 19.37500000273118062, 0.000000000000000000 ) ) ;
#23274=CARTESIAN_POINT ( 'NONE',  ( 20.75514604977248467, 78.42500000273115290, -28.56700777964554305 ) ) ;
#23278=CARTESIAN_POINT ( 'NONE',  ( 33.58253175000000823, 66.02500000273118985, 10.91162601494192685 ) ) ;
#23281=CARTESIAN_POINT ( 'NONE',  ( -33.58253175000000113, 7.025000002731188964, -10.91162601494193041 ) ) ;
#23282=CARTESIAN_POINT ( 'NONE',  ( -14.47279130897151589, 17.82499999726881157, -19.92008829642072598 ) ) ;
#23284=VERTEX_POINT ( 'NONE', #15930 ) ;
#23286=ORIENTED_EDGE ( 'NONE', *, *, #5341, .T. ) ;
#23291=CARTESIAN_POINT ( 'NONE',  ( -2.162160676586881955E-15, 78.62500000273115575, -35.31076352940723240 ) ) ;
#23292=CARTESIAN_POINT ( 'NONE',  ( -7.236395654485763274, 2.524999997268823293, 22.27133577429736633 ) ) ;
#23293=CARTESIAN_POINT ( 'NONE',  ( 18.94512977948575738, 14.42499999726881654, 13.76444248337723408 ) ) ;
#23294=CARTESIAN_POINT ( 'NONE',  ( -10.37757302488624411, 14.97500000273119269, -31.93888565452638417 ) ) ;
#23295=CARTESIAN_POINT ( 'NONE',  ( -32.50000000000000000, 18.40000000546238823, -10.55989012756945478 ) ) ;
#23297=CARTESIAN_POINT ( 'NONE',  ( -20.08610463437156923, 68.30000000000001137, 27.64615127144130113 ) ) ;
#23298=CARTESIAN_POINT ( 'NONE',  ( 19.82091636218621389, 11.94999999453763628, -14.40073868116559197 ) ) ;
#23299=DIRECTION ( 'NONE',  ( -0.8660254037844402619, -0.4999999999999970579, 0.000000000000000000 ) ) ;
#23301=CARTESIAN_POINT ( 'NONE',  ( -5.147494310547430452, 32.05125428700920764, -32.49999999999999289 ) ) ;
#23305=PLANE ( 'NONE',  #17720 ) ;
#23306=CARTESIAN_POINT ( 'NONE',  ( 14.47279130897151589, 14.82499999726881690, 19.92008829642072953 ) ) ;
#23307=CARTESIAN_POINT ( 'NONE',  ( 10.04305231718579705, 8.599999999999996092, 30.90933677959248982 ) ) ;
#23309=DIRECTION ( 'NONE',  ( 0.000000000000000000, 0.000000000000000000, -1.000000000000000000 ) ) ;
#23311=CARTESIAN_POINT ( 'NONE',  ( -2.162160676586881955E-15, 52.62500000273117706, -35.31076352940723240 ) ) ;
#23313=CARTESIAN_POINT ( 'NONE',  ( -33.58253175000000113, 43.47500000273117138, 10.91162601494193929 ) ) ;
#23314=FACE_OUTER_BOUND ( 'NONE', #32501, .T. ) ;
#23316=CARTESIAN_POINT ( 'NONE',  ( -7.570916362186215665, 9.399999999999991473, 23.30088464923126423 ) ) ;
#23317=CARTESIAN_POINT ( 'NONE',  ( -20.08610463437157989, 22.20000000546238184, -27.64615127144129758 ) ) ;
#23322=CARTESIAN_POINT ( 'NONE',  ( 19.82091636218621034, 11.80000000000000426, 14.40073868116559730 ) ) ;
#23325=CARTESIAN_POINT ( 'NONE',  ( -24.50000000000000711, 10.84999999453761887, 7.960532557706201828 ) ) ;
#23327=CARTESIAN_POINT ( 'NONE',  ( -27.16883889988624290, 28.92500000273118133, -19.73931689729374028 ) ) ;
#23329=EDGE_LOOP ( 'NONE', ( #32214, #28885, #19788, #17077 ) ) ;
#23340=CARTESIAN_POINT ( 'NONE',  ( 33.58253175000000113, 32.47500000273117138, -10.91162601494193751 ) ) ;
#23341=CARTESIAN_POINT ( 'NONE',  ( -26.29305231718578995, 34.70000000546239249, 19.10302069950538595 ) ) ;
#23345=CARTESIAN_POINT ( 'NONE',  ( -20.75514604977248112, 21.42500000273120264, 28.56700777964554661 ) ) ;
#23347=CARTESIAN_POINT ( 'NONE',  ( -33.58253175000000113, 49.47500000273118559, 10.91162601494193929 ) ) ;
#23349=CARTESIAN_POINT ( 'NONE',  ( 6.277390505771533514E-15, 30.49999999999999645, 34.17252228774368916 ) ) ;
#23351=CARTESIAN_POINT ( 'NONE',  ( -33.58253175000000113, 67.22500000273117848, 10.91162601494193929 ) ) ;
#23354=CARTESIAN_POINT ( 'NONE',  ( -27.16883889988624290, 63.17500000273118843, -19.73931689729374028 ) ) ;
#23356=CARTESIAN_POINT ( 'NONE',  ( 10.37757302488624056, 12.52500000273118452, -31.93888565452638417 ) ) ;
#23361=DIRECTION ( 'NONE',  ( -0.000000000000000000, -1.000000000000000000, -0.000000000000000000 ) ) ;
#23366=AXIS2_PLACEMENT_3D ( 'NONE', #18595, #3136, #5538 ) ;
#23368=CARTESIAN_POINT ( 'NONE',  ( 20.08610463437158344, 63.20000000546237118, 27.64615127144129403 ) ) ;
#23369=CARTESIAN_POINT ( 'NONE',  ( -20.08610463437156923, 66.80000000546236549, 27.64615127144130113 ) ) ;
#23374=CARTESIAN_POINT ( 'NONE',  ( -33.58253175000000113, 77.47500000273120691, 10.91162601494193929 ) ) ;
#23378=CARTESIAN_POINT ( 'NONE',  ( 10.37757302488624767, 55.97500000273119980, 31.93888565452638417 ) ) ;
#23379=CARTESIAN_POINT ( 'NONE',  ( -32.50000000000000000, 54.40000000546238823, -10.55989012756945478 ) ) ;
#23381=CARTESIAN_POINT ( 'NONE',  ( -10.37757302488624411, 44.72500000273119269, -31.93888565452638417 ) ) ;
#23383=CARTESIAN_POINT ( 'NONE',  ( -20.75514604977248112, 71.67500000273116711, 28.56700777964554661 ) ) ;
#23385=CARTESIAN_POINT ( 'NONE',  ( -32.50000000000000000, 8.600000005462376862, 10.55989012756946366 ) ) ;
#23388=CARTESIAN_POINT ( 'NONE',  ( 20.08610463437158344, 48.70000000000000284, 27.64615127144129403 ) ) ;
#23390=CARTESIAN_POINT ( 'NONE',  ( -33.58253175000000113, 13.37500000273117351, 0.000000000000000000 ) ) ;
#23391=DIRECTION ( 'NONE',  ( 0.000000000000000000, 0.000000000000000000, -1.000000000000000000 ) ) ;
#23393=CARTESIAN_POINT ( 'NONE',  ( 13.91746824999999532, 78.47500000273116427, -4.522059556121118540 ) ) ;
#23394=CARTESIAN_POINT ( 'NONE',  ( 2.375766604868046361, 74.80125428700920054, 14.99999999999999822 ) ) ;
#23397=ORIENTED_EDGE ( 'NONE', *, *, #21114, .T. ) ;
#23398=VECTOR ( 'NONE', #13343, 1000.000000000000000 ) ;
#23410=CARTESIAN_POINT ( 'NONE',  ( -10.37757302488624411, 44.72500000273119269, -31.93888565452638417 ) ) ;
#23416=CARTESIAN_POINT ( 'NONE',  ( 20.75514604977248467, 72.67500000273118133, -28.56700777964554305 ) ) ;
#23417=EDGE_LOOP ( 'NONE', ( #24275, #9549, #29057, #32959, #12083, #11996 ) ) ;
#23422=( BOUNDED_CURVE ( )  B_SPLINE_CURVE ( 2, ( #6254, #29580, #18647, #26692, #26355, #2845, #23788, #255, #5589, #16070, #29254, #21383, #31828 ),
 .UNSPECIFIED., .F., .T. ) 
 B_SPLINE_CURVE_WITH_KNOTS ( ( 3, 2, 2, 2, 2, 2, 3 ),
 ( 0.05000000000000000278, 0.05999999999999999778, 0.08000000000000000167, 0.1000000000000000056, 0.1199999999999999956, 0.1400000000000000133, 0.1500000000000000222 ),
 .UNSPECIFIED. ) 
 CURVE ( )  GEOMETRIC_REPRESENTATION_ITEM ( )  RATIONAL_B_SPLINE_CURVE ( ( 0.9755282581475768211, 0.9755282581475768211, 1.000000000000000000, 0.9510565162951535312, 1.000000000000000000, 0.9510565162951535312, 1.000000000000000000, 0.9510565162951535312, 1.000000000000000000, 0.9510565162951535312, 1.000000000000000000, 0.9755282581475767101, 0.9755282581475768211 ) ) 
 REPRESENTATION_ITEM ( '' )  );
#23423=CARTESIAN_POINT ( 'NONE',  ( 20.08610463437157279, 29.80000000546237615, -27.64615127144129758 ) ) ;
#23424=CARTESIAN_POINT ( 'NONE',  ( 20.75514604977248467, 64.42500000273116711, -28.56700777964554305 ) ) ;
#23428=CARTESIAN_POINT ( 'NONE',  ( -23.41746824999999887, 4.024999997268810858, -7.608796670333730638 ) ) ;
#23430=CARTESIAN_POINT ( 'NONE',  ( -27.16883889988624290, 2.925000002731187543, -19.73931689729374028 ) ) ;
#23434=CARTESIAN_POINT ( 'NONE',  ( -10.04305231718579172, 3.599999999999992095, -30.90933677959248982 ) ) ;
#23438=CARTESIAN_POINT ( 'NONE',  ( -12.13525491562421088, 72.05000000546237970, -8.816778784387096835 ) ) ;
#23440=CARTESIAN_POINT ( 'NONE',  ( -10.37757302488623701, 29.52500000273117209, 31.93888565452638417 ) ) ;
#23443=CARTESIAN_POINT ( 'NONE',  ( 27.16883889988623935, 24.57500000273119056, -19.73931689729374384 ) ) ;
#23444=CARTESIAN_POINT ( 'NONE',  ( -1.778240108872766143E-15, 63.50000000000000000, -32.49999999999999289 ) ) ;
#23446=CARTESIAN_POINT ( 'NONE',  ( 6.486482029760648627E-15, 73.62500000273118417, 35.31076352940722529 ) ) ;
#23447=EDGE_CURVE ( 'NONE', #12812, #19067, #29413, .T. ) ;
#23448=DIRECTION ( 'NONE',  ( -0.000000000000000000, -1.000000000000000000, -0.000000000000000000 ) ) ;
#23450=LINE ( 'NONE', #33911, #22132 ) ;
#23451=CARTESIAN_POINT ( 'NONE',  ( 27.16883889988624290, 61.92500000273118133, 19.73931689729373673 ) ) ;
#23454=CARTESIAN_POINT ( 'NONE',  ( -10.37757302488624411, 6.725000002731185589, -31.93888565452638417 ) ) ;
#23455=CARTESIAN_POINT ( 'NONE',  ( -18.94512977948575738, 17.92499999726882010, -13.76444248337723231 ) ) ;
#23457=ORIENTED_EDGE ( 'NONE', *, *, #23095, .T. ) ;
#23463=CARTESIAN_POINT ( 'NONE',  ( -33.58253175000000113, 79.02500000273118985, -10.91162601494193218 ) ) ;
#23464=CARTESIAN_POINT ( 'NONE',  ( -14.47279130897152122, 6.424999997268821872, 19.92008829642072243 ) ) ;
#23465=CARTESIAN_POINT ( 'NONE',  ( -24.50000000000000355, 0.9000000000000005773, -7.960532557706207157 ) ) ;
#23466=CARTESIAN_POINT ( 'NONE',  ( -27.16883889988623935, 13.57500000273120833, 19.73931689729374739 ) ) ;
#23467=CARTESIAN_POINT ( 'NONE',  ( 6.277390505771533514E-15, 56.49999999999998579, 34.17252228774368916 ) ) ;
#23469=CARTESIAN_POINT ( 'NONE',  ( 0.000000000000000000, 80.00000000000001421, 0.000000000000000000 ) ) ;
#23471=CARTESIAN_POINT ( 'NONE',  ( -11.25946833292375793, 73.57500000273120122, 8.180482586598737171 ) ) ;
#23474=CARTESIAN_POINT ( 'NONE',  ( 0.000000000000000000, 82.00000000000001421, 0.000000000000000000 ) ) ;
#23475=CARTESIAN_POINT ( 'NONE',  ( 10.04305231718578817, 65.40000000000001990, -30.90933677959249337 ) ) ;
#23476=CARTESIAN_POINT ( 'NONE',  ( -10.04305231718578462, 10.39999999999999325, 30.90933677959249337 ) ) ;
#23477=VECTOR ( 'NONE', #7170, 1000.000000000000000 ) ;
#23480=CARTESIAN_POINT ( 'NONE',  ( -33.58253175000000113, 51.02500000273119696, -10.91162601494193218 ) ) ;
#23482=CARTESIAN_POINT ( 'NONE',  ( 33.58253175000000113, 40.37500000273119838, -4.112674001490185761E-15 ) ) ;
#23483=CARTESIAN_POINT ( 'NONE',  ( 26.29305231718578995, 25.19999999999999929, -19.10302069950538240 ) ) ;
#23488=VECTOR ( 'NONE', #19339, 1000.000000000000114 ) ;
#23490=CARTESIAN_POINT ( 'NONE',  ( 5.147494310547426899, 7.448745718453160691, -32.50000000000000000 ) ) ;
#23491=CARTESIAN_POINT ( 'NONE',  ( 0.000000000000000000, 80.00000000000001421, -32.50000000000000000 ) ) ;
#23492=CARTESIAN_POINT ( 'NONE',  ( -5.147494310547430452, 39.55125428154684641, -32.49999999999999289 ) ) ;
#23496=CARTESIAN_POINT ( 'NONE',  ( 4.023268246324634798E-14, 10.24999999453763166, -24.50000000000000355 ) ) ;
#23497=CARTESIAN_POINT ( 'NONE',  ( 10.37757302488624056, 28.52500000273120051, -31.93888565452638417 ) ) ;
#23499=EDGE_CURVE ( 'NONE', #28763, #27323, #12987, .T. ) ;
#23507=CARTESIAN_POINT ( 'NONE',  ( 23.41746824999999887, 18.87499999726882649, 0.000000000000000000 ) ) ;
#23508=CARTESIAN_POINT ( 'NONE',  ( 6.486482029760649416E-15, 35.87500000273118417, 35.31076352940723240 ) ) ;
#23509=CARTESIAN_POINT ( 'NONE',  ( -26.29305231718579350, 38.30000000546237970, -19.10302069950537884 ) ) ;
#23511=CARTESIAN_POINT ( 'NONE',  ( -1.778240108872766143E-15, 53.50000000000000000, -32.49999999999999289 ) ) ;
#23512=CARTESIAN_POINT ( 'NONE',  ( 33.58253175000000113, 26.12500000273118417, -4.112674001490185761E-15 ) ) ;
#23513=CARTESIAN_POINT ( 'NONE',  ( 27.16883889988624290, 50.17500000273117422, 19.73931689729373673 ) ) ;
#23515=CARTESIAN_POINT ( 'NONE',  ( 26.29305231718578995, 29.20000000000000284, -19.10302069950538240 ) ) ;
#23518=CARTESIAN_POINT ( 'NONE',  ( -10.37757302488623701, 67.52500000273120406, 31.93888565452638417 ) ) ;
#23521=CARTESIAN_POINT ( 'NONE',  ( 10.37757302488624056, 62.77500000273117564, -31.93888565452638417 ) ) ;
#23523=CARTESIAN_POINT ( 'NONE',  ( -10.37757302488624411, 12.72500000273119092, -31.93888565452638417 ) ) ;
#23526=CARTESIAN_POINT ( 'NONE',  ( -33.58253175000000113, 3.375000002731193049, 0.000000000000000000 ) ) ;
#23528=CARTESIAN_POINT ( 'NONE',  ( 32.50000000000000000, 45.50000000546239676, -3.980102097228898626E-15 ) ) ;
#23529=CARTESIAN_POINT ( 'NONE',  ( 20.08610463437157279, 19.30000000000000071, -27.64615127144129758 ) ) ;
#23533=EDGE_CURVE ( 'NONE', #20505, #16826, #7476, .T. ) ;
#23537=CARTESIAN_POINT ( 'NONE',  ( -26.29305231718579350, 53.80000000000001137, -19.10302069950537884 ) ) ;
#23538=ADVANCED_FACE ( 'NONE', ( #6453 ), #27385, .F. ) ;
#23539=CARTESIAN_POINT ( 'NONE',  ( 32.50000000000000711, 67.40000000546237402, 10.55989012756945122 ) ) ;
#23547=CARTESIAN_POINT ( 'NONE',  ( -20.08610463437157989, 35.70000000000000995, -27.64615127144129758 ) ) ;
#23548=CARTESIAN_POINT ( 'NONE',  ( 27.16883889988624290, 56.17500000273118133, 19.73931689729373673 ) ) ;
#23549=CARTESIAN_POINT ( 'NONE',  ( -10.04305231718579172, 54.10000000546239107, -30.90933677959248982 ) ) ;
#23550=CARTESIAN_POINT ( 'NONE',  ( 5.779280353836490358E-15, 11.00000000546238077, 32.49999999999999289 ) ) ;
#23551=CARTESIAN_POINT ( 'NONE',  ( -20.75514604977248823, 44.82500000273117990, -28.56700777964554305 ) ) ;
#23553=CARTESIAN_POINT ( 'NONE',  ( 27.16883889988624290, 70.17500000273119554, 19.73931689729373673 ) ) ;
#23557=CARTESIAN_POINT ( 'NONE',  ( 20.08610463437157279, 45.29999999999999005, -27.64615127144129758 ) ) ;
#23559=CARTESIAN_POINT ( 'NONE',  ( -20.75514604977248823, 13.07500000273120300, -28.56700777964554305 ) ) ;
#23562=CARTESIAN_POINT ( 'NONE',  ( 2.688165632520823219E-15, 79.87500000273118417, 14.63369212191046387 ) ) ;
#23563=CARTESIAN_POINT ( 'NONE',  ( 33.58253175000000113, 76.37500000273116996, -4.112674001490185761E-15 ) ) ;
#23564=CARTESIAN_POINT ( 'NONE',  ( -8.891200544363830713E-16, 75.50000000000000000, -15.00000000000000000 ) ) ;
#23566=ORIENTED_EDGE ( 'NONE', *, *, #2571, .T. ) ;
#23576=CARTESIAN_POINT ( 'NONE',  ( -5.147494310547423346, 56.94874572391554324, 32.50000000000000000 ) ) ;
#23577=CARTESIAN_POINT ( 'NONE',  ( 33.58253175000000823, 40.02500000273119696, 10.91162601494192685 ) ) ;
#23580=PRODUCT_DEFINITION_SHAPE ( 'NONE', 'NONE',  #78 ) ;
#23581=CARTESIAN_POINT ( 'NONE',  ( -10.04305231718579172, 2.100000005462371533, -30.90933677959248982 ) ) ;
#23584=CARTESIAN_POINT ( 'NONE',  ( -9.270509831248419985, 70.55000000546236549, 12.75976212528060039 ) ) ;
#23586=CARTESIAN_POINT ( 'NONE',  ( -20.75514604977248823, 77.07500000273117280, -28.56700777964554305 ) ) ;
#23587=ORIENTED_EDGE ( 'NONE', *, *, #18889, .F. ) ;
#23592=CARTESIAN_POINT ( 'NONE',  ( -20.75514604977248112, 63.42500000273118133, 28.56700777964554661 ) ) ;
#23595=CARTESIAN_POINT ( 'NONE',  ( -18.94512977948575738, 11.92499999726881477, -13.76444248337723231 ) ) ;
#23596=CARTESIAN_POINT ( 'NONE',  ( -27.16883889988623935, 3.325000002731171023, 19.73931689729374739 ) ) ;
#23597=CARTESIAN_POINT ( 'NONE',  ( -8.891200544363830713E-16, 77.75000000546236834, -15.00000000000000000 ) ) ;
#23599=CARTESIAN_POINT ( 'NONE',  ( 10.04305231718579705, 36.59999999999999432, 30.90933677959248982 ) ) ;
#23604=CARTESIAN_POINT ( 'NONE',  ( -12.13525491562421088, 74.05000000546237970, -8.816778784387096835 ) ) ;
#23606=CARTESIAN_POINT ( 'NONE',  ( -20.75514604977248823, 32.82500000273118701, -28.56700777964554305 ) ) ;
#23609=CARTESIAN_POINT ( 'NONE',  ( -27.16883889988624290, 13.17500000273119554, -19.73931689729374028 ) ) ;
#23610=CARTESIAN_POINT ( 'NONE',  ( -8.891200544363830713E-16, 79.50000000000001421, -15.00000000000000000 ) ) ;
#23612=CARTESIAN_POINT ( 'NONE',  ( 20.75514604977249178, 77.82500000273120122, 28.56700777964553950 ) ) ;
#23613=CARTESIAN_POINT ( 'NONE',  ( 24.50000000000000000, 7.900000000000012790, 7.960532557706212486 ) ) ;
#23615=CARTESIAN_POINT ( 'NONE',  ( 7.236395654485755280, 14.22499999726881192, 22.27133577429736988 ) ) ;
#23616=CARTESIAN_POINT ( 'NONE',  ( -33.58253175000000113, 59.22500000273119980, 10.91162601494193929 ) ) ;
#23618=ORIENTED_EDGE ( 'NONE', *, *, #10218, .T. ) ;
#23620=( BOUNDED_CURVE ( )  B_SPLINE_CURVE ( 2, ( #27331, #8964, #33139, #22349, #16869, #20125, #19948, #3818, #32796, #4155, #1565, #30224, #7066 ),
 .UNSPECIFIED., .F., .T. ) 
 B_SPLINE_CURVE_WITH_KNOTS ( ( 3, 2, 2, 2, 2, 2, 3 ),
 ( 0.04487179487179487197, 0.04615384615384615641, 0.04871794871794871834, 0.05128205128205128027, 0.05384615384615384914, 0.05641025641025641107, 0.05769230769230769551 ),
 .UNSPECIFIED. ) 
 CURVE ( )  GEOMETRIC_REPRESENTATION_ITEM ( )  RATIONAL_B_SPLINE_CURVE ( ( 0.9755282581475768211, 0.9755282581475768211, 1.000000000000000000, 0.9510565162951535312, 1.000000000000000000, 0.9510565162951535312, 1.000000000000000000, 0.9510565162951535312, 1.000000000000000000, 0.9510565162951535312, 1.000000000000000000, 0.9755282581475767101, 0.9755282581475768211 ) ) 
 REPRESENTATION_ITEM ( '' )  );
#23621=CARTESIAN_POINT ( 'NONE',  ( -20.75514604977248112, 9.425000002731202642, 28.56700777964554661 ) ) ;
#23622=CARTESIAN_POINT ( 'NONE',  ( -18.94512977948576093, 16.32499999726880091, 13.76444248337722698 ) ) ;
#23624=ADVANCED_FACE ( 'NONE', ( #25145 ), #5067, .F. ) ;
#23631=CARTESIAN_POINT ( 'NONE',  ( 5.147494310547426899, 27.94874572391553613, -32.50000000000000000 ) ) ;
#23634=CARTESIAN_POINT ( 'NONE',  ( -19.82091636218621034, 0.7999999999999951594, -14.40073868116559552 ) ) ;
#23635=CARTESIAN_POINT ( 'NONE',  ( 20.75514604977248467, 12.67500000273118488, -28.56700777964554305 ) ) ;
#23636=CARTESIAN_POINT ( 'NONE',  ( -32.50000000000000000, 60.00000000000000000, 0.000000000000000000 ) ) ;
#23637=CARTESIAN_POINT ( 'NONE',  ( 13.91746824999999532, 75.97500000273119269, -4.522059556121118540 ) ) ;
#23638=DIRECTION ( 'NONE',  ( -0.000000000000000000, -1.000000000000000000, -0.000000000000000000 ) ) ;
#23639=AXIS2_PLACEMENT_3D ( 'NONE', #33766, #17989, #5272 ) ;
#23641=CARTESIAN_POINT ( 'NONE',  ( -4.300734207923759378, 74.97500000273119269, -13.23629886949340495 ) ) ;
#23645=CYLINDRICAL_SURFACE ( 'NONE', #22304, 15.00000000000000000 ) ;
#23646=CARTESIAN_POINT ( 'NONE',  ( -3.880418787951136483, 12.55125428154685174, -24.50000000000000000 ) ) ;
#23647=CARTESIAN_POINT ( 'NONE',  ( 20.08610463437158344, 4.699999999999995737, 27.64615127144129403 ) ) ;
#23648=CARTESIAN_POINT ( 'NONE',  ( -33.58253175000000113, 79.12500000273119838, 0.000000000000000000 ) ) ;
#23650=CARTESIAN_POINT ( 'NONE',  ( 33.58253175000000823, 48.02500000273119696, 10.91162601494192863 ) ) ;
#23652=CARTESIAN_POINT ( 'NONE',  ( -33.58253175000000113, 35.47500000273119269, 10.91162601494193929 ) ) ;
#23653=CARTESIAN_POINT ( 'NONE',  ( 10.04305231718578817, 25.40000000000000568, -30.90933677959249337 ) ) ;
#23654=DIRECTION ( 'NONE',  ( -0.8660254037844410391, 0.4999999999999958367, 0.000000000000000000 ) ) ;
#23657=CARTESIAN_POINT ( 'NONE',  ( -1.778240108872766143E-15, 52.00000000546237544, -32.49999999999999289 ) ) ;
#23661=DIRECTION ( 'NONE',  ( -0.000000000000000000, -1.000000000000000000, -0.000000000000000000 ) ) ;
#23664=CARTESIAN_POINT ( 'NONE',  ( -4.223320258572819786E-15, 11.24999999453763344, 24.50000000000000000 ) ) ;
#23665=CARTESIAN_POINT ( 'NONE',  ( 20.75514604977249178, 27.82500000273116925, 28.56700777964553950 ) ) ;
#23668=ORIENTED_EDGE ( 'NONE', *, *, #27812, .F. ) ;
#23674=CARTESIAN_POINT ( 'NONE',  ( -7.236395654485757944, 1.224999997268799712, -22.27133577429736988 ) ) ;
#23675=CARTESIAN_POINT ( 'NONE',  ( 27.16883889988623935, 32.57500000273119412, -19.73931689729374384 ) ) ;
#23676=CARTESIAN_POINT ( 'NONE',  ( 20.08610463437158344, 39.20000000546237118, 27.64615127144129403 ) ) ;
#23677=CARTESIAN_POINT ( 'NONE',  ( 26.29305231718578995, 77.19999999999998863, -19.10302069950538240 ) ) ;
#23679=CARTESIAN_POINT ( 'NONE',  ( 5.147494310547440222, 77.44874571845315359, -32.50000000000000000 ) ) ;
#23680=CARTESIAN_POINT ( 'NONE',  ( 20.75514604977248467, 50.67500000273117422, -28.56700777964554305 ) ) ;
#23682=CARTESIAN_POINT ( 'NONE',  ( -10.04305231718578462, 20.40000000000000213, 30.90933677959249337 ) ) ;
#23685=CARTESIAN_POINT ( 'NONE',  ( 33.58253175000000113, 72.22500000273119269, -10.91162601494193751 ) ) ;
#23686=CARTESIAN_POINT ( 'NONE',  ( -10.04305231718578462, 78.39999999999999147, 30.90933677959249337 ) ) ;
#23688=CARTESIAN_POINT ( 'NONE',  ( 10.37757302488624056, 56.77500000273119696, -31.93888565452638417 ) ) ;
#23689=CARTESIAN_POINT ( 'NONE',  ( 10.04305231718578817, 39.90000000546237402, -30.90933677959249337 ) ) ;
#23690=CARTESIAN_POINT ( 'NONE',  ( 20.75514604977249178, 13.82500000273117813, 28.56700777964553950 ) ) ;
#23693=CARTESIAN_POINT ( 'NONE',  ( -2.162160676586882350E-15, 2.875000002731204596, -35.31076352940722529 ) ) ;
#23701=CARTESIAN_POINT ( 'NONE',  ( 5.779280353836490358E-15, 60.49999999999998579, 32.49999999999999289 ) ) ;
#23703=CARTESIAN_POINT ( 'NONE',  ( 18.94512977948576093, 7.324999997268822227, -13.76444248337722875 ) ) ;
#23704=CARTESIAN_POINT ( 'NONE',  ( 10.04305231718579705, 71.10000000546237686, 30.90933677959248982 ) ) ;
#23708=ORIENTED_EDGE ( 'NONE', *, *, #20503, .F. ) ;
#23712=DIRECTION ( 'NONE',  ( 0.000000000000000000, 0.000000000000000000, -1.000000000000000000 ) ) ;
#23713=CARTESIAN_POINT ( 'NONE',  ( 10.37757302488624056, 56.77500000273119696, -31.93888565452638417 ) ) ;
#23714=CARTESIAN_POINT ( 'NONE',  ( 20.08610463437157279, 53.80000000546237970, -27.64615127144129758 ) ) ;
#23715=( BOUNDED_CURVE ( )  B_SPLINE_CURVE ( 2, ( #25882, #2375, #21094, #5121, #23322, #15605, #13184, #2553, #28966, #24651, #22091, #13864, #8866 ),
 .UNSPECIFIED., .F., .T. ) 
 B_SPLINE_CURVE_WITH_KNOTS ( ( 3, 2, 2, 2, 2, 2, 3 ),
 ( 0.6388888888888889506, 0.6444444444444444864, 0.6555555555555555580, 0.6666666666666666297, 0.6777777777777778123, 0.6888888888888888840, 0.6944444444444444198 ),
 .UNSPECIFIED. ) 
 CURVE ( )  GEOMETRIC_REPRESENTATION_ITEM ( )  RATIONAL_B_SPLINE_CURVE ( ( 0.9755282581475768211, 0.9755282581475770431, 1.000000000000000000, 0.9510565162951535312, 1.000000000000000000, 0.9510565162951535312, 1.000000000000000000, 0.9510565162951535312, 1.000000000000000000, 0.9510565162951535312, 1.000000000000000000, 0.9755282581475768211, 0.9755282581475768211 ) ) 
 REPRESENTATION_ITEM ( '' )  );
#23717=CARTESIAN_POINT ( 'NONE',  ( -33.58253175000000113, 41.22500000273118559, 10.91162601494193929 ) ) ;
#23718=CARTESIAN_POINT ( 'NONE',  ( 5.779280353836490358E-15, 39.00000000546237544, 32.49999999999999289 ) ) ;
#23719=CARTESIAN_POINT ( 'NONE',  ( -27.16883889988624290, 69.17500000273119554, -19.73931689729374028 ) ) ;
#23723=CARTESIAN_POINT ( 'NONE',  ( 32.50000000000000711, 48.89999999999999858, 10.55989012756945122 ) ) ;
#23725=EDGE_CURVE ( 'NONE', #14241, #11374, #16493, .T. ) ;
#23726=CARTESIAN_POINT ( 'NONE',  ( 20.75514604977249178, 8.075000002731185234, 28.56700777964553950 ) ) ;
#23727=CARTESIAN_POINT ( 'NONE',  ( 10.04305231718578817, 35.90000000546239534, -30.90933677959249337 ) ) ;
#23729=CARTESIAN_POINT ( 'NONE',  ( -4.300734207923755825, 71.77500000273117564, 13.23629886949340673 ) ) ;
#23730=CARTESIAN_POINT ( 'NONE',  ( 10.37757302488624767, 77.97500000273119269, 31.93888565452638417 ) ) ;
#23731=LINE ( 'NONE', #21165, #5079 ) ;
#23735=ORIENTED_EDGE ( 'NONE', *, *, #9203, .T. ) ;
#23736=LINE ( 'NONE', #18427, #21726 ) ;
#23746=CARTESIAN_POINT ( 'NONE',  ( 27.16883889988624290, 41.92500000273119554, 19.73931689729373673 ) ) ;
#23750=VERTEX_POINT ( 'NONE', #22880 ) ;
#23754=CARTESIAN_POINT ( 'NONE',  ( 20.75514604977248467, 68.67500000273119554, -28.56700777964554305 ) ) ;
#23755=ORIENTED_EDGE ( 'NONE', *, *, #5517, .T. ) ;
#23759=EDGE_LOOP ( 'NONE', ( #1430, #16736, #3402, #25041 ) ) ;
#23760=CARTESIAN_POINT ( 'NONE',  ( -20.08610463437157989, 14.20000000546237473, -27.64615127144129758 ) ) ;
#23761=CARTESIAN_POINT ( 'NONE',  ( 33.58253175000000113, 64.12500000273119838, -4.112674001490185761E-15 ) ) ;
#23764=CARTESIAN_POINT ( 'NONE',  ( 18.94512977948576093, 7.324999997268822227, -13.76444248337722875 ) ) ;
#23765=CARTESIAN_POINT ( 'NONE',  ( 10.37757302488624056, 4.525000002731205839, -31.93888565452638417 ) ) ;
#23766=CARTESIAN_POINT ( 'NONE',  ( 27.16883889988623935, 28.57500000273119412, -19.73931689729374384 ) ) ;
#23767=CARTESIAN_POINT ( 'NONE',  ( 26.29305231718578995, 5.700000005462390718, -19.10302069950538240 ) ) ;
#23770=CARTESIAN_POINT ( 'NONE',  ( -20.08610463437156923, 32.29999999999999716, 27.64615127144130113 ) ) ;
#23771=CARTESIAN_POINT ( 'NONE',  ( -1.778240108872766143E-15, 3.500000000000004441, -32.49999999999999289 ) ) ;
#23774=ADVANCED_FACE ( 'NONE', ( #16885 ), #4512, .T. ) ;
#23777=CARTESIAN_POINT ( 'NONE',  ( 4.635254915624212657, 70.85000000546237686, 14.26584774442730286 ) ) ;
#23779=CARTESIAN_POINT ( 'NONE',  ( 27.16883889988624290, 21.92500000273117777, 19.73931689729373673 ) ) ;
#23782=CARTESIAN_POINT ( 'NONE',  ( 27.16883889988623935, 12.57500000273120655, -19.73931689729374384 ) ) ;
#23783=CARTESIAN_POINT ( 'NONE',  ( -5.147494310547478413, 64.44874571845315359, 32.49999999999998579 ) ) ;
#23785=CARTESIAN_POINT ( 'NONE',  ( 20.75514604977249178, 71.82500000273117280, 28.56700777964553950 ) ) ;
#23788=CARTESIAN_POINT ( 'NONE',  ( 15.00000000000000000, 79.25000000546239676, -1.836970198721029589E-15 ) ) ;
#23789=CARTESIAN_POINT ( 'NONE',  ( 33.58253175000000113, 60.22500000273119980, -10.91162601494193574 ) ) ;
#23790=EDGE_CURVE ( 'NONE', #16901, #7704, #19968, .T. ) ;
#23795=CARTESIAN_POINT ( 'NONE',  ( -18.94512977948576093, 1.824999997268816898, 13.76444248337722698 ) ) ;
#23800=VERTEX_POINT ( 'NONE', #32813 ) ;
#23802=CARTESIAN_POINT ( 'NONE',  ( -1.778240108872766143E-15, 5.500000000000003553, -32.49999999999999289 ) ) ;
#23804=CARTESIAN_POINT ( 'NONE',  ( 3.000384657911015469E-15, 0.000000000000000000, -24.50000000000000000 ) ) ;
#23807=CARTESIAN_POINT ( 'NONE',  ( 15.14183272437242245, 0.2999999999999904965, -20.84094480462497856 ) ) ;
#23808=CARTESIAN_POINT ( 'NONE',  ( 10.37757302488624767, 11.97500000273118914, 31.93888565452638417 ) ) ;
#23809=CARTESIAN_POINT ( 'NONE',  ( -26.29305231718579350, 57.80000000000001847, -19.10302069950537884 ) ) ;
#23810=CARTESIAN_POINT ( 'NONE',  ( -4.300734207923755825, 77.27500000273118985, 13.23629886949340673 ) ) ;
#23811=CARTESIAN_POINT ( 'NONE',  ( 26.29305231718579350, 73.30000000546237970, 19.10302069950537529 ) ) ;
#23813=CARTESIAN_POINT ( 'NONE',  ( 13.91746824999999532, 76.47500000273117848, -4.522059556121118540 ) ) ;
#23815=CARTESIAN_POINT ( 'NONE',  ( -1.778240108872766143E-15, 34.00000000546236834, -32.49999999999999289 ) ) ;
#23816=CARTESIAN_POINT ( 'NONE',  ( 26.29305231718579350, 64.79999999999999716, 19.10302069950537529 ) ) ;
#23817=CARTESIAN_POINT ( 'NONE',  ( 10.04305231718579705, 2.599999999999991207, 30.90933677959248982 ) ) ;
#23820=CARTESIAN_POINT ( 'NONE',  ( -33.58253175000000113, 47.12500000273117706, 0.000000000000000000 ) ) ;
#23823=CARTESIAN_POINT ( 'NONE',  ( -2.162160676586882350E-15, 36.87500000273117706, -35.31076352940722529 ) ) ;
#23824=( BOUNDED_CURVE ( )  B_SPLINE_CURVE ( 2, ( #25711, #4941, #5288, #15423, #28616, #15770, #20913, #26225, #20579, #2547, #33601, #10780, #31702 ),
 .UNSPECIFIED., .F., .T. ) 
 B_SPLINE_CURVE_WITH_KNOTS ( ( 3, 2, 2, 2, 2, 2, 3 ),
 ( 0.2243589743589743668, 0.2256410256410256443, 0.2282051282051281993, 0.2307692307692307820, 0.2333333333333333370, 0.2358974358974358920, 0.2371794871794871973 ),
 .UNSPECIFIED. ) 
 CURVE ( )  GEOMETRIC_REPRESENTATION_ITEM ( )  RATIONAL_B_SPLINE_CURVE ( ( 0.9755282581475768211, 0.9755282581475768211, 1.000000000000000000, 0.9510565162951535312, 1.000000000000000000, 0.9510565162951535312, 1.000000000000000000, 0.9510565162951535312, 1.000000000000000000, 0.9510565162951535312, 1.000000000000000000, 0.9755282581475764880, 0.9755282581475768211 ) ) 
 REPRESENTATION_ITEM ( '' )  );
#23825=CARTESIAN_POINT ( 'NONE',  ( 23.41746824999999887, 18.62499999726882649, 0.000000000000000000 ) ) ;
#23827=CARTESIAN_POINT ( 'NONE',  ( 32.50000000000000000, 15.60000000546238930, -10.55989012756945833 ) ) ;
#23832=CARTESIAN_POINT ( 'NONE',  ( -1.778240108872766143E-15, 65.50000000000000000, -32.49999999999999289 ) ) ;
#23833=CARTESIAN_POINT ( 'NONE',  ( -26.29305231718578995, 40.20000000000001705, 19.10302069950538595 ) ) ;
#23836=CARTESIAN_POINT ( 'NONE',  ( -19.82091636218621389, 10.94999999453763451, 14.40073868116558842 ) ) ;
#23837=CARTESIAN_POINT ( 'NONE',  ( -27.16883889988624290, 22.92500000273117777, -19.73931689729374028 ) ) ;
#23847=CARTESIAN_POINT ( 'NONE',  ( 10.37757302488624056, 26.77500000273119696, -31.93888565452638417 ) ) ;
#23848=AXIS2_PLACEMENT_3D ( 'NONE', #4653, #19473, #29923 ) ;
#23849=CARTESIAN_POINT ( 'NONE',  ( -10.04305231718578462, 34.90000000546239534, 30.90933677959249337 ) ) ;
#23851=CARTESIAN_POINT ( 'NONE',  ( -26.29305231718578995, 54.70000000546237828, 19.10302069950538595 ) ) ;
#23852=CARTESIAN_POINT ( 'NONE',  ( 10.04305231718578817, 77.39999999999999147, -30.90933677959249337 ) ) ;
#23853=CARTESIAN_POINT ( 'NONE',  ( 20.75514604977249178, 40.07500000273118701, 28.56700777964553950 ) ) ;
#23855=CARTESIAN_POINT ( 'NONE',  ( -10.04305231718579172, 19.60000000000000497, -30.90933677959248982 ) ) ;
#23858=CARTESIAN_POINT ( 'NONE',  ( -27.16883889988623935, 69.32500000273117280, 19.73931689729374739 ) ) ;
#23860=CARTESIAN_POINT ( 'NONE',  ( -20.08610463437157989, 76.20000000546235697, -27.64615127144129758 ) ) ;
#23861=CARTESIAN_POINT ( 'NONE',  ( -33.58253175000000113, 51.27500000273118275, -10.91162601494193041 ) ) ;
#23863=CARTESIAN_POINT ( 'NONE',  ( -33.58253175000000113, 9.125000002731198379, 0.000000000000000000 ) ) ;
#23868=CARTESIAN_POINT ( 'NONE',  ( -26.29305231718578995, 18.70000000546237473, 19.10302069950538595 ) ) ;
#23875=CARTESIAN_POINT ( 'NONE',  ( 10.04305231718579705, 69.10000000546237686, 30.90933677959248982 ) ) ;
#23879=ORIENTED_EDGE ( 'NONE', *, *, #12596, .F. ) ;
#23884=CARTESIAN_POINT ( 'NONE',  ( -27.16883889988623935, 53.57500000273118701, 19.73931689729374739 ) ) ;
#23885=CARTESIAN_POINT ( 'NONE',  ( 10.04305231718578817, 57.90000000546238823, -30.90933677959249337 ) ) ;
#23887=CARTESIAN_POINT ( 'NONE',  ( -33.58253175000000113, 33.22500000273117138, 10.91162601494193929 ) ) ;
#23889=CARTESIAN_POINT ( 'NONE',  ( 33.58253175000000113, 66.47500000273119269, -10.91162601494193751 ) ) ;
#23893=CARTESIAN_POINT ( 'NONE',  ( -26.29305231718578995, 38.20000000000000995, 19.10302069950538595 ) ) ;
#23895=CARTESIAN_POINT ( 'NONE',  ( 6.486482029760649416E-15, 9.875000002731187720, 35.31076352940723240 ) ) ;
#23898=CARTESIAN_POINT ( 'NONE',  ( -11.25946833292375793, 73.57500000273120122, 8.180482586598737171 ) ) ;
#23899=CARTESIAN_POINT ( 'NONE',  ( -33.58253175000000113, 75.27500000273118985, -10.91162601494193041 ) ) ;
#23902=ORIENTED_EDGE ( 'NONE', *, *, #24568, .F. ) ;
#23905=VECTOR ( 'NONE', #14261, 1000.000000000000000 ) ;
#23914=CARTESIAN_POINT ( 'NONE',  ( -27.16883889988624290, 36.92500000273118843, -19.73931689729374028 ) ) ;
#23916=CARTESIAN_POINT ( 'NONE',  ( 5.779280353836490358E-15, 34.49999999999998579, 32.49999999999999289 ) ) ;
#23917=CYLINDRICAL_SURFACE ( 'NONE', #4059, 24.50000000000000000 ) ;
#23919=ADVANCED_FACE ( 'NONE', ( #4598 ), #22965, .T. ) ;
#23921=( BOUNDED_CURVE ( )  B_SPLINE_CURVE ( 2, ( #32366, #11119, #19345, #26564, #8696, #32530, #21587, #465, #5628, #8530, #24645, #1119, #13531 ),
 .UNSPECIFIED., .F., .T. ) 
 B_SPLINE_CURVE_WITH_KNOTS ( ( 3, 2, 2, 2, 2, 2, 3 ),
 ( 0.4294871794871795156, 0.4307692307692307931, 0.4333333333333333481, 0.4358974358974359031, 0.4384615384615384581, 0.4410256410256410131, 0.4423076923076922906 ),
 .UNSPECIFIED. ) 
 CURVE ( )  GEOMETRIC_REPRESENTATION_ITEM ( )  RATIONAL_B_SPLINE_CURVE ( ( 0.9755282581475768211, 0.9755282581475772652, 1.000000000000000000, 0.9510565162951535312, 1.000000000000000000, 0.9510565162951535312, 1.000000000000000000, 0.9510565162951535312, 1.000000000000000000, 0.9510565162951535312, 1.000000000000000000, 0.9755282581475768211, 0.9755282581475768211 ) ) 
 REPRESENTATION_ITEM ( '' )  );
#23922=CARTESIAN_POINT ( 'NONE',  ( -2.165007332552593587E-13, 51.00000000546238255, 32.50000000000000000 ) ) ;
#23924=CARTESIAN_POINT ( 'NONE',  ( -33.58253175000000113, 69.37500000273119838, 0.000000000000000000 ) ) ;
#23926=VERTEX_POINT ( 'NONE', #25708 ) ;
#23929=ORIENTED_EDGE ( 'NONE', *, *, #15128, .T. ) ;
#23930=CARTESIAN_POINT ( 'NONE',  ( -1.778240108872766143E-15, 32.00000000546237544, -32.49999999999999289 ) ) ;
#23931=CARTESIAN_POINT ( 'NONE',  ( 27.16883889988623935, 60.32500000273119412, -19.73931689729374384 ) ) ;
#23933=CARTESIAN_POINT ( 'NONE',  ( -32.50000000000000000, 16.50000000546236834, 0.000000000000000000 ) ) ;
#23934=CARTESIAN_POINT ( 'NONE',  ( 24.50000000000000355, 17.89999999999998437, 7.960532557706212486 ) ) ;
#23935=CARTESIAN_POINT ( 'NONE',  ( -18.94512977948575738, 5.924999997268809437, -13.76444248337723231 ) ) ;
#23936=CARTESIAN_POINT ( 'NONE',  ( 20.75514604977249178, 28.07500000273119412, 28.56700777964553950 ) ) ;
#23937=CARTESIAN_POINT ( 'NONE',  ( -15.00000000000000000, 78.15000000546235981, -4.873795443493594171 ) ) ;
#23940=CARTESIAN_POINT ( 'NONE',  ( -13.91746824999999887, 78.87500000273118417, 0.000000000000000000 ) ) ;
#23941=CARTESIAN_POINT ( 'NONE',  ( 32.50000000000000000, 75.60000000546236265, -10.55989012756945833 ) ) ;
#23945=CARTESIAN_POINT ( 'NONE',  ( 13.91746825000000065, 73.77500000273118985, 4.522059556121114987 ) ) ;
#23947=CARTESIAN_POINT ( 'NONE',  ( -33.58253175000000113, 25.02500000273117209, -10.91162601494193218 ) ) ;
#23950=CARTESIAN_POINT ( 'NONE',  ( 27.16883889988623935, 18.57500000273118346, -19.73931689729374384 ) ) ;
#23952=CARTESIAN_POINT ( 'NONE',  ( 33.58253175000000113, 72.12500000273119838, -4.112674001490185761E-15 ) ) ;
#23953=CARTESIAN_POINT ( 'NONE',  ( 26.29305231718578995, 3.700000005462389385, -19.10302069950538240 ) ) ;
#23955=DIRECTION ( 'NONE',  ( -0.000000000000000000, -1.000000000000000000, -0.000000000000000000 ) ) ;
#23956=CARTESIAN_POINT ( 'NONE',  ( 20.75514604977249178, 59.82500000273117280, 28.56700777964553950 ) ) ;
#23962=CARTESIAN_POINT ( 'NONE',  ( 4.445600272181915325E-13, 15.49999999999999822, -32.50000000000000000 ) ) ;
#23963=CARTESIAN_POINT ( 'NONE',  ( -14.47279130897151589, 15.82499999726881335, -19.92008829642072598 ) ) ;
#23967=CARTESIAN_POINT ( 'NONE',  ( 5.779280353836490358E-15, 43.00000000546236834, 32.49999999999999289 ) ) ;
#23968=EDGE_LOOP ( 'NONE', ( #3161, #17500, #3477, #3321 ) ) ;
#23971=CARTESIAN_POINT ( 'NONE',  ( -15.00000000000000000, 82.00000000000001421, 0.000000000000000000 ) ) ;
#23973=CARTESIAN_POINT ( 'NONE',  ( -14.47279130897152122, 17.92499999726880588, 19.92008829642072243 ) ) ;
#23974=CARTESIAN_POINT ( 'NONE',  ( -33.58253175000000113, 9.475000002731201576, 10.91162601494193929 ) ) ;
#23975=CARTESIAN_POINT ( 'NONE',  ( -32.50000000000000000, 61.89999999999999147, -10.55989012756945478 ) ) ;
#23976=CARTESIAN_POINT ( 'NONE',  ( -11.25946833292375793, 80.67500000273119554, -8.180482586598733619 ) ) ;
#23977=DIRECTION ( 'NONE',  ( -0.000000000000000000, -1.000000000000000000, -0.000000000000000000 ) ) ;
#23979=CARTESIAN_POINT ( 'NONE',  ( 11.25946833292375793, 78.17500000273119554, 8.180482586598731842 ) ) ;
#23983=FACE_OUTER_BOUND ( 'NONE', #1960, .T. ) ;
#23984=CARTESIAN_POINT ( 'NONE',  ( -32.50000000000000000, 2.000000000000001776, 0.000000000000000000 ) ) ;
#23986=CARTESIAN_POINT ( 'NONE',  ( -33.58253175000000113, 45.02500000273117564, -10.91162601494193218 ) ) ;
#23989=CARTESIAN_POINT ( 'NONE',  ( -2.162160676586882350E-15, 32.87500000273118417, -35.31076352940722529 ) ) ;
#23990=CARTESIAN_POINT ( 'NONE',  ( 32.50000000000000000, 25.09999999999999432, -10.55989012756945833 ) ) ;
#23993=DIRECTION ( 'NONE',  ( -0.000000000000000000, -1.000000000000000000, -0.000000000000000000 ) ) ;
#23997=CARTESIAN_POINT ( 'NONE',  ( 7.236395654485755280, 4.224999997268802154, 22.27133577429736988 ) ) ;
#23998=CARTESIAN_POINT ( 'NONE',  ( 19.82091636218621034, 9.549999994537621717, 14.40073868116559730 ) ) ;
#24001=CARTESIAN_POINT ( 'NONE',  ( -33.58253175000000113, 17.22500000273118914, 10.91162601494193929 ) ) ;
#24003=ORIENTED_EDGE ( 'NONE', *, *, #5812, .T. ) ;
#24005=ORIENTED_EDGE ( 'NONE', *, *, #6826, .T. ) ;
#24010=FACE_OUTER_BOUND ( 'NONE', #6576, .T. ) ;
#24011=CARTESIAN_POINT ( 'NONE',  ( -27.16883889988624290, 27.17500000273118133, -19.73931689729374028 ) ) ;
#24012=AXIS2_PLACEMENT_3D ( 'NONE', #7634, #20862, #13296 ) ;
#24013=CARTESIAN_POINT ( 'NONE',  ( 26.29305231718579350, 37.30000000546237970, 19.10302069950537529 ) ) ;
#24015=CARTESIAN_POINT ( 'NONE',  ( 32.50000000000000000, 33.50000000546238255, -3.980102097228898626E-15 ) ) ;
#24016=CARTESIAN_POINT ( 'NONE',  ( 32.50000000000000000, 37.50000000546238255, -3.980102097228898626E-15 ) ) ;
#24017=CARTESIAN_POINT ( 'NONE',  ( -27.16883889988624290, 45.17500000273119554, -19.73931689729374028 ) ) ;
#24021=CARTESIAN_POINT ( 'NONE',  ( -32.50000000000000000, 23.99999999999999289, 0.000000000000000000 ) ) ;
#24023=( BOUNDED_CURVE ( )  B_SPLINE_CURVE ( 2, ( #33815, #10136, #10308, #30712, #14940, #17866, #7207, #15115, #20618, #23004, #20436, #20786, #33461 ),
 .UNSPECIFIED., .F., .T. ) 
 B_SPLINE_CURVE_WITH_KNOTS ( ( 3, 2, 2, 2, 2, 2, 3 ),
 ( 0.8055555555555555802, 0.8111111111111111160, 0.8222222222222221877, 0.8333333333333333703, 0.8444444444444444420, 0.8555555555555555136, 0.8611111111111111605 ),
 .UNSPECIFIED. ) 
 CURVE ( )  GEOMETRIC_REPRESENTATION_ITEM ( )  RATIONAL_B_SPLINE_CURVE ( ( 0.9755282581475768211, 0.9755282581475768211, 1.000000000000000000, 0.9510565162951535312, 1.000000000000000000, 0.9510565162951535312, 1.000000000000000000, 0.9510565162951535312, 1.000000000000000000, 0.9510565162951535312, 1.000000000000000000, 0.9755282581475765991, 0.9755282581475768211 ) ) 
 REPRESENTATION_ITEM ( '' )  );
#24024=CARTESIAN_POINT ( 'NONE',  ( 10.37757302488624767, 61.72500000273117848, 31.93888565452638417 ) ) ;
#24027=CARTESIAN_POINT ( 'NONE',  ( -2.162160676586882350E-15, 50.87500000273119838, -35.31076352940722529 ) ) ;
#24030=CARTESIAN_POINT ( 'NONE',  ( 33.58253175000000823, 6.025000002731191628, 10.91162601494192863 ) ) ;
#24032=CARTESIAN_POINT ( 'NONE',  ( 10.04305231718578817, 25.90000000546238823, -30.90933677959249337 ) ) ;
#24037=CARTESIAN_POINT ( 'NONE',  ( -1.778240108872766143E-15, 58.00000000546237544, -32.49999999999999289 ) ) ;
#24041=CARTESIAN_POINT ( 'NONE',  ( 32.50000000000000000, 48.99999999999998579, -3.980102097228898626E-15 ) ) ;
#24044=CARTESIAN_POINT ( 'NONE',  ( 6.277390505771533514E-15, 71.00000000546235412, 34.17252228774368916 ) ) ;
#24050=EDGE_CURVE ( 'NONE', #3462, #2966, #30502, .T. ) ;
#24052=CARTESIAN_POINT ( 'NONE',  ( 0.000000000000000000, 80.00000000000001421, 0.000000000000000000 ) ) ;
#24053=CARTESIAN_POINT ( 'NONE',  ( 20.75514604977248467, 50.67500000273117422, -28.56700777964554305 ) ) ;
#24054=CARTESIAN_POINT ( 'NONE',  ( -20.08610463437156923, 58.80000000546239391, 27.64615127144130113 ) ) ;
#24056=CARTESIAN_POINT ( 'NONE',  ( 33.58253175000000823, 38.02500000273117564, 10.91162601494192863 ) ) ;
#24057=CARTESIAN_POINT ( 'NONE',  ( 5.147494310547426899, 55.44874571845315359, -32.50000000000000000 ) ) ;
#24058=CARTESIAN_POINT ( 'NONE',  ( -33.58253175000000113, 59.47500000273118559, 10.91162601494193929 ) ) ;
#24062=ADVANCED_FACE ( 'NONE', ( #13351 ), #13011, .T. ) ;
#24064=CARTESIAN_POINT ( 'NONE',  ( -32.50000000000000000, 40.00000000000000711, 0.000000000000000000 ) ) ;
#24066=CARTESIAN_POINT ( 'NONE',  ( 10.37757302488624056, 4.775000002731177418, -31.93888565452638417 ) ) ;
#24067=CARTESIAN_POINT ( 'NONE',  ( 5.147494310547426899, 35.94874572391554324, -32.50000000000000000 ) ) ;
#24069=CARTESIAN_POINT ( 'NONE',  ( -33.58253175000000113, 71.27500000273118985, -10.91162601494193041 ) ) ;
#24070=CARTESIAN_POINT ( 'NONE',  ( -15.14183272437242778, 19.04999999453762172, 20.84094480462497856 ) ) ;
#24073=VERTEX_POINT ( 'NONE', #23825 ) ;
#24074=DIRECTION ( 'NONE',  ( -0.000000000000000000, -1.000000000000000000, -0.000000000000000000 ) ) ;
#24084=CARTESIAN_POINT ( 'NONE',  ( 10.37757302488624767, 37.72500000273118559, 31.93888565452638417 ) ) ;
#24087=DIRECTION ( 'NONE',  ( 0.000000000000000000, 0.000000000000000000, 1.000000000000000000 ) ) ;
#24088=ORIENTED_EDGE ( 'NONE', *, *, #4457, .F. ) ;
#24090=CARTESIAN_POINT ( 'NONE',  ( -20.08610463437156923, 50.80000000546237970, 27.64615127144130113 ) ) ;
#24092=CARTESIAN_POINT ( 'NONE',  ( -33.58253175000000113, 71.47500000273119269, 10.91162601494193929 ) ) ;
#24096=ORIENTED_EDGE ( 'NONE', *, *, #8182, .T. ) ;
#24097=CARTESIAN_POINT ( 'NONE',  ( -32.50000000000000000, 48.40000000546237402, -10.55989012756945300 ) ) ;
#24098=CARTESIAN_POINT ( 'NONE',  ( -20.75514604977248823, 52.82500000273116569, -28.56700777964554305 ) ) ;
#24100=CARTESIAN_POINT ( 'NONE',  ( 32.50000000000000000, 19.60000000546237686, -10.55989012756945833 ) ) ;
#24102=CARTESIAN_POINT ( 'NONE',  ( 7.236395654485760609, 9.524999997268801977, -22.27133577429736633 ) ) ;
#24103=CARTESIAN_POINT ( 'NONE',  ( -33.58253175000000113, 27.27500000273119340, -10.91162601494193218 ) ) ;
#24106=CARTESIAN_POINT ( 'NONE',  ( 4.300734207923757602, 80.27500000273118985, -13.23629886949340673 ) ) ;
#24107=CARTESIAN_POINT ( 'NONE',  ( 26.29305231718579350, 8.800000000000002487, 19.10302069950537529 ) ) ;
#24111=CARTESIAN_POINT ( 'NONE',  ( 13.91746824999999532, 77.97500000273119269, -4.522059556121118540 ) ) ;
#24113=EDGE_CURVE ( 'NONE', #16121, #21853, #10985, .T. ) ;
#24114=CARTESIAN_POINT ( 'NONE',  ( -33.58253175000000113, 25.12500000273118417, 0.000000000000000000 ) ) ;
#24117=CARTESIAN_POINT ( 'NONE',  ( 6.486482029760648627E-15, 17.87500000273119838, 35.31076352940722529 ) ) ;
#24119=CARTESIAN_POINT ( 'NONE',  ( 10.37757302488624767, 71.72500000273119269, 31.93888565452638417 ) ) ;
#24120=DIRECTION ( 'NONE',  ( -0.000000000000000000, -1.000000000000000000, -0.000000000000000000 ) ) ;
#24121=( BOUNDED_CURVE ( )  B_SPLINE_CURVE ( 2, ( #3829, #30756, #30067, #22361, #20305, #6573, #32808, #27, #15680, #7766, #10181, #23394, #5364 ),
 .UNSPECIFIED., .F., .T. ) 
 B_SPLINE_CURVE_WITH_KNOTS ( ( 3, 2, 2, 2, 2, 2, 3 ),
 ( 0.4500000000000000111, 0.4600000000000000200, 0.4799999999999999822, 0.5000000000000000000, 0.5200000000000000178, 0.5400000000000000355, 0.5500000000000000444 ),
 .UNSPECIFIED. ) 
 CURVE ( )  GEOMETRIC_REPRESENTATION_ITEM ( )  RATIONAL_B_SPLINE_CURVE ( ( 0.9755282581475768211, 0.9755282581475768211, 1.000000000000000000, 0.9510565162951535312, 1.000000000000000000, 0.9510565162951535312, 1.000000000000000000, 0.9510565162951535312, 1.000000000000000000, 0.9510565162951535312, 1.000000000000000000, 0.9755282581475768211, 0.9755282581475768211 ) ) 
 REPRESENTATION_ITEM ( '' )  );
#24124=CARTESIAN_POINT ( 'NONE',  ( 20.75514604977248467, 60.42500000273118133, -28.56700777964554305 ) ) ;
#24128=CARTESIAN_POINT ( 'NONE',  ( -20.08610463437157989, 15.69999999999999929, -27.64615127144129758 ) ) ;
#24129=CARTESIAN_POINT ( 'NONE',  ( 7.236395654485760609, 9.024999997268800200, -22.27133577429736633 ) ) ;
#24136=CARTESIAN_POINT ( 'NONE',  ( 32.50000000000000000, 5.099999999999983658, -10.55989012756945833 ) ) ;
#24137=CARTESIAN_POINT ( 'NONE',  ( -3.880418787951142701, 3.448745718453164244, 24.49999999999999645 ) ) ;
#24138=CARTESIAN_POINT ( 'NONE',  ( 20.75514604977249178, 71.82500000273118701, 28.56700777964553950 ) ) ;
#24140=CARTESIAN_POINT ( 'NONE',  ( -24.50000000000000000, 9.000000000000007105, -3.000384657911015469E-15 ) ) ;
#24141=CARTESIAN_POINT ( 'NONE',  ( -20.75514604977248112, 9.675000002731193760, 28.56700777964554661 ) ) ;
#24142=CARTESIAN_POINT ( 'NONE',  ( -10.37757302488624411, 24.72500000273119980, -31.93888565452638417 ) ) ;
#24143=CARTESIAN_POINT ( 'NONE',  ( 8.601468415847516980, 78.17500000273118133, -11.83890561707634603 ) ) ;
#24146=CARTESIAN_POINT ( 'NONE',  ( -4.300734207923759378, 78.97500000273119269, -13.23629886949340495 ) ) ;
#24149=CARTESIAN_POINT ( 'NONE',  ( -20.08610463437156923, 38.80000000546237260, 27.64615127144130113 ) ) ;
#24151=CARTESIAN_POINT ( 'NONE',  ( -33.58253175000000113, 41.12500000273119838, 0.000000000000000000 ) ) ;
#24154=CARTESIAN_POINT ( 'NONE',  ( 20.75514604977248467, 36.67500000273118843, -28.56700777964554305 ) ) ;
#24156=ADVANCED_FACE ( 'NONE', ( #23314 ), #33779, .T. ) ;
#24162=CARTESIAN_POINT ( 'NONE',  ( 18.94512977948575738, 2.424999997268806329, 13.76444248337723408 ) ) ;
#24165=CARTESIAN_POINT ( 'NONE',  ( -26.29305231718578995, 60.20000000000000284, 19.10302069950538595 ) ) ;
#24166=CARTESIAN_POINT ( 'NONE',  ( -10.37757302488624411, 20.72500000273119625, -31.93888565452638417 ) ) ;
#24175=ORIENTED_EDGE ( 'NONE', *, *, #26197, .F. ) ;
#24177=CARTESIAN_POINT ( 'NONE',  ( 20.75514604977249178, 28.07500000273119412, 28.56700777964553950 ) ) ;
#24178=CARTESIAN_POINT ( 'NONE',  ( 26.29305231718578995, 29.70000000546238539, -19.10302069950538240 ) ) ;
#24179=CARTESIAN_POINT ( 'NONE',  ( 10.04305231718578817, 79.39999999999999147, -30.90933677959249337 ) ) ;
#24181=CARTESIAN_POINT ( 'NONE',  ( -3.880418787951104953, 11.44874571845314293, 24.50000000000000711 ) ) ;
#24182=CARTESIAN_POINT ( 'NONE',  ( -33.58253175000000113, 45.47500000273119980, 10.91162601494193929 ) ) ;
#24184=CARTESIAN_POINT ( 'NONE',  ( 32.50000000000000000, 18.99999999999998934, -3.980102097228898626E-15 ) ) ;
#24185=AXIS2_PLACEMENT_3D ( 'NONE', #9806, #15135, #7573 ) ;
#24187=CARTESIAN_POINT ( 'NONE',  ( -33.58253175000000113, 63.22500000273119269, 10.91162601494193929 ) ) ;
#24189=CARTESIAN_POINT ( 'NONE',  ( 27.16883889988624290, 56.17500000273118133, 19.73931689729373673 ) ) ;
#24191=CARTESIAN_POINT ( 'NONE',  ( 3.880418787951134707, 9.551254281546839309, 24.50000000000000000 ) ) ;
#24192=CARTESIAN_POINT ( 'NONE',  ( -33.58253175000000113, 7.125000002731196602, 0.000000000000000000 ) ) ;
#24193=ADVANCED_FACE ( 'NONE', ( #15936 ), #18683, .F. ) ;
#24194=EDGE_CURVE ( 'NONE', #27363, #19688, #3556, .T. ) ;
#24197=CARTESIAN_POINT ( 'NONE',  ( -20.08610463437157989, 19.69999999999998863, -27.64615127144129758 ) ) ;
#24205=LINE ( 'NONE', #6167, #699 ) ;
#24207=ORIENTED_EDGE ( 'NONE', *, *, #2759, .F. ) ;
#24211=DIRECTION ( 'NONE',  ( -0.000000000000000000, -1.000000000000000000, -0.000000000000000000 ) ) ;
#24212=ORIENTED_EDGE ( 'NONE', *, *, #27904, .F. ) ;
#24215=( BOUNDED_CURVE ( )  B_SPLINE_CURVE ( 2, ( #6684, #1183, #12001, #14084, #22146, #32423, #19904, #30353, #6855, #8920, #24382, #27286, #11335 ),
 .UNSPECIFIED., .F., .F. ) 
 B_SPLINE_CURVE_WITH_KNOTS ( ( 3, 2, 2, 2, 2, 2, 3 ),
 ( 0.1730769230769230727, 0.1743589743589743501, 0.1769230769230769329, 0.1794871794871794879, 0.1820512820512820429, 0.1846153846153846256, 0.1858974358974359031 ),
 .UNSPECIFIED. ) 
 CURVE ( )  GEOMETRIC_REPRESENTATION_ITEM ( )  RATIONAL_B_SPLINE_CURVE ( ( 0.9755282581475768211, 0.9755282581475768211, 1.000000000000000000, 0.9510565162951535312, 1.000000000000000000, 0.9510565162951535312, 1.000000000000000000, 0.9510565162951535312, 1.000000000000000000, 0.9510565162951535312, 1.000000000000000000, 0.9755282581475768211, 0.9755282581475768211 ) ) 
 REPRESENTATION_ITEM ( '' )  );
#24217=CARTESIAN_POINT ( 'NONE',  ( -1.778240108872766143E-15, 21.50000000000000000, -32.49999999999999289 ) ) ;
#24218=CARTESIAN_POINT ( 'NONE',  ( -2.162160676586881955E-15, 44.87500000273119127, -35.31076352940723240 ) ) ;
#24219=CARTESIAN_POINT ( 'NONE',  ( -10.04305231718578462, 48.90000000546238113, 30.90933677959249337 ) ) ;
#24221=CARTESIAN_POINT ( 'NONE',  ( 10.37757302488624056, 38.52500000273118275, -31.93888565452638417 ) ) ;
#24224=CARTESIAN_POINT ( 'NONE',  ( -10.37757302488624411, 64.97500000273120691, -31.93888565452638417 ) ) ;
#24226=CARTESIAN_POINT ( 'NONE',  ( -32.50000000000000000, 42.09999999999997300, 10.55989012756946366 ) ) ;
#24228=CARTESIAN_POINT ( 'NONE',  ( -10.37757302488623701, 5.775000002731179194, 31.93888565452638417 ) ) ;
#24230=CARTESIAN_POINT ( 'NONE',  ( 4.300734207923757602, 74.77500000273118985, -13.23629886949340673 ) ) ;
#24231=CARTESIAN_POINT ( 'NONE',  ( -33.58253175000000113, 75.47500000273116427, 10.91162601494193929 ) ) ;
#24246=CARTESIAN_POINT ( 'NONE',  ( -10.37757302488624411, 40.72500000273118559, -31.93888565452638417 ) ) ;
#24250=CARTESIAN_POINT ( 'NONE',  ( -4.223320258572819786E-15, 5.249999994537622783, 24.50000000000000000 ) ) ;
#24251=VERTEX_POINT ( 'NONE', #21420 ) ;
#24253=CYLINDRICAL_SURFACE ( 'NONE', #5315, 24.50000000000000000 ) ;
#24255=CARTESIAN_POINT ( 'NONE',  ( -10.37757302488623701, 69.77500000273117564, 31.93888565452638417 ) ) ;
#24256=EDGE_LOOP ( 'NONE', ( #26449, #7830, #22266, #6889 ) ) ;
#24262=VECTOR ( 'NONE', #28119, 1000.000000000000000 ) ;
#24264=CARTESIAN_POINT ( 'NONE',  ( 10.37757302488624767, 55.72500000273117138, 31.93888565452638417 ) ) ;
#24266=CARTESIAN_POINT ( 'NONE',  ( 6.277390505771533514E-15, 21.00000000546236478, 34.17252228774368916 ) ) ;
#24268=CARTESIAN_POINT ( 'NONE',  ( 3.880418787951140036, 16.19874571299077459, -24.49999999999999645 ) ) ;
#24269=CARTESIAN_POINT ( 'NONE',  ( 18.94512977948575738, 8.924999997268812990, 13.76444248337723408 ) ) ;
#24270=CARTESIAN_POINT ( 'NONE',  ( -20.75514604977248112, 23.67500000273118843, 28.56700777964554661 ) ) ;
#24272=CARTESIAN_POINT ( 'NONE',  ( -8.960552108402742093E-16, 80.37500000273115575, -14.63369212191046387 ) ) ;
#24275=ORIENTED_EDGE ( 'NONE', *, *, #26774, .T. ) ;
#24277=CARTESIAN_POINT ( 'NONE',  ( -8.601468415847518756, 76.57500000273115859, -11.83890561707634781 ) ) ;
#24279=CARTESIAN_POINT ( 'NONE',  ( -27.16883889988624290, 22.92500000273117777, -19.73931689729374028 ) ) ;
#24283=CARTESIAN_POINT ( 'NONE',  ( -33.58253175000000113, 7.475000002731175819, 10.91162601494193929 ) ) ;
#24285=CARTESIAN_POINT ( 'NONE',  ( -20.75514604977248112, 69.42500000273116711, 28.56700777964554661 ) ) ;
#24287=CARTESIAN_POINT ( 'NONE',  ( -8.891200544363830713E-16, 73.50000000000001421, -15.00000000000000000 ) ) ;
#24288=CARTESIAN_POINT ( 'NONE',  ( -11.25946833292375793, 77.17500000273119554, -8.180482586598733619 ) ) ;
#24291=FACE_OUTER_BOUND ( 'NONE', #32048, .T. ) ;
#24292=CARTESIAN_POINT ( 'NONE',  ( -33.58253175000000113, 61.12500000273119127, 0.000000000000000000 ) ) ;
#24296=CARTESIAN_POINT ( 'NONE',  ( -10.04305231718578462, 16.39999999999999858, 30.90933677959249337 ) ) ;
#24297=CARTESIAN_POINT ( 'NONE',  ( -23.41746825000000243, 9.524999997268810858, -7.608796670333730638 ) ) ;
#24303=CARTESIAN_POINT ( 'NONE',  ( 26.29305231718578995, 5.199999999999982414, -19.10302069950538240 ) ) ;
#24304=CARTESIAN_POINT ( 'NONE',  ( -20.75514604977248112, 73.42500000273118133, 28.56700777964554661 ) ) ;
#24306=CARTESIAN_POINT ( 'NONE',  ( 24.50000000000000355, 3.899999999999992806, 7.960532557706212486 ) ) ;
#24307=CARTESIAN_POINT ( 'NONE',  ( -10.37757302488623701, 11.77500000273118452, 31.93888565452638417 ) ) ;
#24308=CARTESIAN_POINT ( 'NONE',  ( -20.75514604977248823, 16.82500000273120122, -28.56700777964554305 ) ) ;
#24309=CARTESIAN_POINT ( 'NONE',  ( -8.601468415847518756, 80.57500000273120122, -11.83890561707634603 ) ) ;
#24310=CYLINDRICAL_SURFACE ( 'NONE', #17605, 32.50000000000000000 ) ;
#24312=CARTESIAN_POINT ( 'NONE',  ( -12.13525491562421088, 77.80000000000001137, -8.816778784387096835 ) ) ;
#24315=CARTESIAN_POINT ( 'NONE',  ( -26.29305231718579350, 38.30000000546237970, -19.10302069950537884 ) ) ;
#24318=CARTESIAN_POINT ( 'NONE',  ( 33.58253175000000113, 44.22500000273117138, -10.91162601494193751 ) ) ;
#24321=CARTESIAN_POINT ( 'NONE',  ( 10.37757302488624056, 36.77500000273120406, -31.93888565452638417 ) ) ;
#24324=CARTESIAN_POINT ( 'NONE',  ( -10.04305231718578462, 18.39999999999999858, 30.90933677959249337 ) ) ;
#24325=DIRECTION ( 'NONE',  ( -0.000000000000000000, -1.000000000000000000, -0.000000000000000000 ) ) ;
#24328=CARTESIAN_POINT ( 'NONE',  ( -23.41746824999999887, 5.524999997268821517, -7.608796670333730638 ) ) ;
#24329=CARTESIAN_POINT ( 'NONE',  ( -20.08610463437157989, 52.20000000546236407, -27.64615127144129758 ) ) ;
#24331=CARTESIAN_POINT ( 'NONE',  ( 0.000000000000000000, 0.000000000000000000, 0.000000000000000000 ) ) ;
#24332=CARTESIAN_POINT ( 'NONE',  ( -20.75514604977248823, 22.82500000273118701, -28.56700777964554305 ) ) ;
#24333=CARTESIAN_POINT ( 'NONE',  ( -23.41746825000000243, 6.024999997268805529, -7.608796670333730638 ) ) ;
#24334=VECTOR ( 'NONE', #14771, 1000.000000000000000 ) ;
#24337=ORIENTED_EDGE ( 'NONE', *, *, #26284, .T. ) ;
#24339=EDGE_CURVE ( 'NONE', #30070, #5024, #12069, .T. ) ;
#24345=CARTESIAN_POINT ( 'NONE',  ( -23.41746825000000598, 7.724999997268809260, 7.608796670333726198 ) ) ;
#24346=CARTESIAN_POINT ( 'NONE',  ( 33.58253175000000113, 26.37500000273118417, -4.112674001490185761E-15 ) ) ;
#24347=CARTESIAN_POINT ( 'NONE',  ( 32.50000000000000000, 33.60000000546237686, -10.55989012756945833 ) ) ;
#24348=CARTESIAN_POINT ( 'NONE',  ( 6.277390505771533514E-15, 76.50000000000001421, 34.17252228774368916 ) ) ;
#24349=CARTESIAN_POINT ( 'NONE',  ( -26.29305231718579350, 54.30000000546236549, -19.10302069950537884 ) ) ;
#24350=FACE_OUTER_BOUND ( 'NONE', #11576, .T. ) ;
#24351=CARTESIAN_POINT ( 'NONE',  ( -2.162160676586881955E-15, 40.87500000273119838, -35.31076352940723240 ) ) ;
#24354=CARTESIAN_POINT ( 'NONE',  ( -20.08610463437157989, 21.69999999999998153, -27.64615127144129758 ) ) ;
#24357=CARTESIAN_POINT ( 'NONE',  ( 6.486482029760649416E-15, 65.62500000273116996, 35.31076352940723240 ) ) ;
#24358=CARTESIAN_POINT ( 'NONE',  ( 10.37757302488624767, 55.97500000273119980, 31.93888565452638417 ) ) ;
#24360=CARTESIAN_POINT ( 'NONE',  ( 32.50000000000000000, 39.50000000546238965, -3.980102097228898626E-15 ) ) ;
#24361=CARTESIAN_POINT ( 'NONE',  ( -10.37757302488624411, 6.725000002731185589, -31.93888565452638417 ) ) ;
#24368=CARTESIAN_POINT ( 'NONE',  ( -4.405589869732278832E-13, 31.00000000546236834, 32.50000000000000000 ) ) ;
#24376=EDGE_CURVE ( 'NONE', #27572, #7428, #6116, .T. ) ;
#24382=CARTESIAN_POINT ( 'NONE',  ( -10.04305231718579172, 64.10000000546240528, -30.90933677959248982 ) ) ;
#24383=CARTESIAN_POINT ( 'NONE',  ( -2.162160676586881955E-15, 46.87500000273118417, -35.31076352940723240 ) ) ;
#24384=CARTESIAN_POINT ( 'NONE',  ( 6.277390505771533514E-15, 53.00000000546237544, 34.17252228774368916 ) ) ;
#24386=CARTESIAN_POINT ( 'NONE',  ( 10.37757302488624767, 35.72500000273118559, 31.93888565452638417 ) ) ;
#24387=CARTESIAN_POINT ( 'NONE',  ( 20.75514604977248467, 64.67500000273118133, -28.56700777964554305 ) ) ;
#24388=CARTESIAN_POINT ( 'NONE',  ( -20.08610463437157989, 39.70000000000000284, -27.64615127144129758 ) ) ;
#24390=CARTESIAN_POINT ( 'NONE',  ( 33.58253175000000113, 6.375000002731168181, -4.112674001490185761E-15 ) ) ;
#24391=LINE ( 'NONE', #30193, #2513 ) ;
#24393=CARTESIAN_POINT ( 'NONE',  ( 27.16883889988624290, 74.17500000273119554, 19.73931689729373673 ) ) ;
#24394=DIRECTION ( 'NONE',  ( -0.000000000000000000, -1.000000000000000000, -0.000000000000000000 ) ) ;
#24410=CARTESIAN_POINT ( 'NONE',  ( -7.570916362186215665, 5.149999994537635573, 23.30088464923126423 ) ) ;
#24413=CARTESIAN_POINT ( 'NONE',  ( -15.00000000000000000, 70.25000000546238255, 0.000000000000000000 ) ) ;
#24415=CARTESIAN_POINT ( 'NONE',  ( 33.58253175000000823, 68.27500000273120406, 10.91162601494192863 ) ) ;
#24419=ORIENTED_EDGE ( 'NONE', *, *, #9334, .F. ) ;
#24420=CARTESIAN_POINT ( 'NONE',  ( 10.04305231718578817, 65.90000000546237402, -30.90933677959249337 ) ) ;
#24421=CARTESIAN_POINT ( 'NONE',  ( 27.16883889988624290, 57.92500000273120975, 19.73931689729373673 ) ) ;
#24423=CARTESIAN_POINT ( 'NONE',  ( 6.277390505771533514E-15, 11.00000000546238788, 34.17252228774368916 ) ) ;
#24425=CARTESIAN_POINT ( 'NONE',  ( 14.47279130897151944, 17.42499999726882365, -19.92008829642072598 ) ) ;
#24426=CARTESIAN_POINT ( 'NONE',  ( -33.58253175000000113, 25.27500000273119696, -10.91162601494193218 ) ) ;
#24428=CARTESIAN_POINT ( 'NONE',  ( 15.00000000000000355, 76.89999999999999147, 4.873795443493592394 ) ) ;
#24430=CARTESIAN_POINT ( 'NONE',  ( -4.300734207923759378, 80.47500000273119269, -13.23629886949340495 ) ) ;
#24433=VERTEX_POINT ( 'NONE', #29455 ) ;
#24435=CARTESIAN_POINT ( 'NONE',  ( -8.960552108402742093E-16, 74.37500000273118417, -14.63369212191046387 ) ) ;
#24437=CARTESIAN_POINT ( 'NONE',  ( 6.486482029760649416E-15, 23.62500000273119127, 35.31076352940723240 ) ) ;
#24441=CARTESIAN_POINT ( 'NONE',  ( -27.16883889988623935, 7.575000002731202997, 19.73931689729374739 ) ) ;
#24443=CARTESIAN_POINT ( 'NONE',  ( -27.16883889988623935, 69.32500000273117280, 19.73931689729374739 ) ) ;
#24446=CARTESIAN_POINT ( 'NONE',  ( 13.91746824999999532, 78.47500000273116427, -4.522059556121118540 ) ) ;
#24448=CARTESIAN_POINT ( 'NONE',  ( -15.00000000000000000, 72.25000000546238255, 0.000000000000000000 ) ) ;
#24449=CARTESIAN_POINT ( 'NONE',  ( -2.162160676586882350E-15, 50.62500000273117706, -35.31076352940722529 ) ) ;
#24451=ORIENTED_EDGE ( 'NONE', *, *, #32906, .F. ) ;
#24453=CARTESIAN_POINT ( 'NONE',  ( 27.16883889988623935, 2.325000002731170134, -19.73931689729374384 ) ) ;
#24454=AXIS2_PLACEMENT_3D ( 'NONE', #8436, #13093, #29204 ) ;
#24455=CARTESIAN_POINT ( 'NONE',  ( 7.236395654485755280, 6.224999997268803931, 22.27133577429736988 ) ) ;
#24457=VERTEX_POINT ( 'NONE', #22249 ) ;
#24460=ORIENTED_EDGE ( 'NONE', *, *, #21344, .T. ) ;
#24462=CARTESIAN_POINT ( 'NONE',  ( 33.58253175000000113, 60.37500000273119127, -4.112674001490185761E-15 ) ) ;
#24464=CARTESIAN_POINT ( 'NONE',  ( -27.16883889988623935, 77.32500000273118701, 19.73931689729374739 ) ) ;
#24467=CARTESIAN_POINT ( 'NONE',  ( 15.14183272437241889, 3.699999999999999289, 20.84094480462498211 ) ) ;
#24468=CARTESIAN_POINT ( 'NONE',  ( -20.75514604977248823, 7.075000002731188786, -28.56700777964554305 ) ) ;
#24469=CARTESIAN_POINT ( 'NONE',  ( 33.58253175000000823, 16.02500000273119340, 10.91162601494192863 ) ) ;
#24470=CARTESIAN_POINT ( 'NONE',  ( -11.25946833292375793, 74.67500000273119554, -8.180482586598733619 ) ) ;
#24472=CARTESIAN_POINT ( 'NONE',  ( -8.960552108402742093E-16, 72.87500000273115575, -14.63369212191046387 ) ) ;
#24475=CARTESIAN_POINT ( 'NONE',  ( -24.50000000000000711, 8.849999994537624204, 7.960532557706201828 ) ) ;
#24478=CARTESIAN_POINT ( 'NONE',  ( 6.486482029760649416E-15, 45.62500000273118417, 35.31076352940723240 ) ) ;
#24481=CARTESIAN_POINT ( 'NONE',  ( -10.37757302488624411, 30.97500000273117848, -31.93888565452638417 ) ) ;
#24482=CARTESIAN_POINT ( 'NONE',  ( 19.82091636218621034, 17.80000000000001137, 14.40073868116559730 ) ) ;
#24485=VECTOR ( 'NONE', #5874, 1000.000000000000000 ) ;
#24486=CARTESIAN_POINT ( 'NONE',  ( -15.00000000000000000, 75.90000000000000568, -4.873795443493594171 ) ) ;
#24489=CARTESIAN_POINT ( 'NONE',  ( 7.236395654485760609, 7.024999997268799312, -22.27133577429736633 ) ) ;
#24490=CARTESIAN_POINT ( 'NONE',  ( -5.147494310547430452, 52.05125428700922185, -32.49999999999999289 ) ) ;
#24493=CARTESIAN_POINT ( 'NONE',  ( -33.58253175000000113, 17.02500000273119340, -10.91162601494193041 ) ) ;
#24494=CARTESIAN_POINT ( 'NONE',  ( -7.236395654485757944, 3.724999997268802154, -22.27133577429736988 ) ) ;
#24496=ORIENTED_EDGE ( 'NONE', *, *, #11361, .F. ) ;
#24499=VERTEX_POINT ( 'NONE', #626 ) ;
#24502=CARTESIAN_POINT ( 'NONE',  ( 24.50000000000000000, 15.74999999453763344, 0.000000000000000000 ) ) ;
#24503=CARTESIAN_POINT ( 'NONE',  ( 23.41746825000000243, 8.524999997268812635, 7.608796670333735079 ) ) ;
#24504=CARTESIAN_POINT ( 'NONE',  ( -33.58253175000000113, 31.47500000273117493, 10.91162601494193929 ) ) ;
#24505=CARTESIAN_POINT ( 'NONE',  ( -32.50000000000000000, 28.60000000546238397, 10.55989012756946366 ) ) ;
#24506=( BOUNDED_CURVE ( )  B_SPLINE_CURVE ( 2, ( #14320, #33653, #14487, #10151, #14154, #16733, #2246, #22377, #4822, #28336, #12720, #20453, #25596 ),
 .UNSPECIFIED., .F., .T. ) 
 B_SPLINE_CURVE_WITH_KNOTS ( ( 3, 2, 2, 2, 2, 2, 3 ),
 ( 0.2115384615384615363, 0.2128205128205128138, 0.2153846153846153966, 0.2179487179487179516, 0.2205128205128205066, 0.2230769230769230893, 0.2243589743589743668 ),
 .UNSPECIFIED. ) 
 CURVE ( )  GEOMETRIC_REPRESENTATION_ITEM ( )  RATIONAL_B_SPLINE_CURVE ( ( 0.9755282581475768211, 0.9755282581475768211, 1.000000000000000000, 0.9510565162951535312, 1.000000000000000000, 0.9510565162951535312, 1.000000000000000000, 0.9510565162951535312, 1.000000000000000000, 0.9510565162951535312, 1.000000000000000000, 0.9755282581475768211, 0.9755282581475768211 ) ) 
 REPRESENTATION_ITEM ( '' )  );
#24507=CARTESIAN_POINT ( 'NONE',  ( 6.277390505771533514E-15, 70.50000000000001421, 34.17252228774368916 ) ) ;
#24509=DIRECTION ( 'NONE',  ( 0.000000000000000000, 0.000000000000000000, -1.000000000000000000 ) ) ;
#24511=CARTESIAN_POINT ( 'NONE',  ( -2.162160676586881955E-15, 44.87500000273119127, -35.31076352940723240 ) ) ;
#24514=CARTESIAN_POINT ( 'NONE',  ( 18.94512977948576093, 9.324999997268824004, -13.76444248337722875 ) ) ;
#24515=CARTESIAN_POINT ( 'NONE',  ( -20.08610463437156923, 12.29999999999999183, 27.64615127144130113 ) ) ;
#24518=CARTESIAN_POINT ( 'NONE',  ( 27.16883889988623935, 64.32500000273120122, -19.73931689729374384 ) ) ;
#24519=CARTESIAN_POINT ( 'NONE',  ( -20.75514604977248823, 49.07500000273117280, -28.56700777964554305 ) ) ;
#24522=CARTESIAN_POINT ( 'NONE',  ( 20.75514604977248467, 4.425000002731183990, -28.56700777964554305 ) ) ;
#24524=EDGE_CURVE ( 'NONE', #31336, #21143, #32363, .T. ) ;
#24525=CARTESIAN_POINT ( 'NONE',  ( 32.50000000000000000, 25.50000000546237544, -3.980102097228898626E-15 ) ) ;
#24528=CARTESIAN_POINT ( 'NONE',  ( 5.779280353836490358E-15, 22.49999999999999645, 32.49999999999999289 ) ) ;
#24542=CARTESIAN_POINT ( 'NONE',  ( -32.50000000000000000, 46.60000000546236976, 10.55989012756946366 ) ) ;
#24543=CARTESIAN_POINT ( 'NONE',  ( -20.75514604977248823, 45.07500000273117990, -28.56700777964554305 ) ) ;
#24544=CARTESIAN_POINT ( 'NONE',  ( 26.29305231718579350, 47.30000000546235839, 19.10302069950537529 ) ) ;
#24546=CARTESIAN_POINT ( 'NONE',  ( -10.37757302488624411, 34.72500000273118559, -31.93888565452638417 ) ) ;
#24548=CARTESIAN_POINT ( 'NONE',  ( -10.37757302488623701, 59.77500000273119696, 31.93888565452638417 ) ) ;
#24550=CARTESIAN_POINT ( 'NONE',  ( 20.08610463437157279, 37.30000000000001847, -27.64615127144129758 ) ) ;
#24552=CARTESIAN_POINT ( 'NONE',  ( -33.58253175000000113, 7.475000002731175819, 10.91162601494193929 ) ) ;
#24553=CARTESIAN_POINT ( 'NONE',  ( 0.000000000000000000, 80.00000000000001421, 0.000000000000000000 ) ) ;
#24555=CARTESIAN_POINT ( 'NONE',  ( -20.75514604977248112, 71.67500000273118133, 28.56700777964554661 ) ) ;
#24556=CARTESIAN_POINT ( 'NONE',  ( -19.82091636218621389, 5.200000000000009948, 14.40073868116558842 ) ) ;
#24558=ORIENTED_EDGE ( 'NONE', *, *, #25513, .T. ) ;
#24559=CARTESIAN_POINT ( 'NONE',  ( 1.577395562988744260E-15, 4.249999994537624559, -25.76082449383753925 ) ) ;
#24561=EDGE_CURVE ( 'NONE', #14202, #28636, #14484, .T. ) ;
#24562=CARTESIAN_POINT ( 'NONE',  ( 15.00000000000000355, 74.89999999999999147, 4.873795443493592394 ) ) ;
#24568=EDGE_CURVE ( 'NONE', #5896, #29590, #15610, .T. ) ;
#24574=CARTESIAN_POINT ( 'NONE',  ( -24.50000000000000000, 17.00000000000001421, -3.000384657911015469E-15 ) ) ;
#24585=CARTESIAN_POINT ( 'NONE',  ( -2.162160676586881955E-15, 52.62500000273117706, -35.31076352940723240 ) ) ;
#24587=CARTESIAN_POINT ( 'NONE',  ( -20.08610463437157989, 12.20000000546237828, -27.64615127144129758 ) ) ;
#24589=CARTESIAN_POINT ( 'NONE',  ( 1.507698388325705758E-15, 15.62499999726882116, -24.62258325217400312 ) ) ;
#24590=CARTESIAN_POINT ( 'NONE',  ( 26.29305231718578995, 57.20000000000000284, -19.10302069950538240 ) ) ;
#24591=CARTESIAN_POINT ( 'NONE',  ( -27.16883889988623935, 25.57500000273119056, 19.73931689729374739 ) ) ;
#24592=CARTESIAN_POINT ( 'NONE',  ( -32.50000000000000000, 24.50000000546237544, 0.000000000000000000 ) ) ;
#24594=CARTESIAN_POINT ( 'NONE',  ( -11.25946833292375793, 77.07500000273121543, 8.180482586598737171 ) ) ;
#24595=CARTESIAN_POINT ( 'NONE',  ( 1.555960095263670572E-15, 12.50000000000000355, -24.50000000000000000 ) ) ;
#24599=CARTESIAN_POINT ( 'NONE',  ( -8.601468415847518756, 74.57500000273117280, -11.83890561707634781 ) ) ;
#24601=CARTESIAN_POINT ( 'NONE',  ( -20.75514604977248112, 15.42500000273118843, 28.56700777964554661 ) ) ;
#24605=CARTESIAN_POINT ( 'NONE',  ( -20.75514604977248112, 7.675000002731198201, 28.56700777964554661 ) ) ;
#24609=CARTESIAN_POINT ( 'NONE',  ( 13.91746825000000065, 80.27500000273117564, 4.522059556121115875 ) ) ;
#24612=CARTESIAN_POINT ( 'NONE',  ( -10.37757302488624411, 52.72500000273119980, -31.93888565452638417 ) ) ;
#24614=EDGE_LOOP ( 'NONE', ( #21473, #18987, #7453, #8205 ) ) ;
#24616=DIRECTION ( 'NONE',  ( 0.000000000000000000, 0.000000000000000000, 1.000000000000000000 ) ) ;
#24617=CARTESIAN_POINT ( 'NONE',  ( 23.41746825000000243, 6.724999997268811924, -7.608796670333727974 ) ) ;
#24619=EDGE_LOOP ( 'NONE', ( #32255, #23708, #31998, #18282 ) ) ;
#24621=CARTESIAN_POINT ( 'NONE',  ( 3.980102097228898626E-15, 80.00000000000001421, 32.50000000000000000 ) ) ;
#24623=ORIENTED_EDGE ( 'NONE', *, *, #19597, .F. ) ;
#24625=CARTESIAN_POINT ( 'NONE',  ( 33.58253175000000823, 62.27500000273118275, 10.91162601494192863 ) ) ;
#24627=CARTESIAN_POINT ( 'NONE',  ( 6.486482029760649416E-15, 73.62500000273118417, 35.31076352940723240 ) ) ;
#24629=CARTESIAN_POINT ( 'NONE',  ( -24.50000000000000000, 7.000000000000006217, -3.000384657911015469E-15 ) ) ;
#24630=CARTESIAN_POINT ( 'NONE',  ( -2.162160676586881955E-15, 2.875000002731204596, -35.31076352940723240 ) ) ;
#24631=CARTESIAN_POINT ( 'NONE',  ( 33.58253175000000113, 16.12500000273120548, -4.112674001490185761E-15 ) ) ;
#24632=DIRECTION ( 'NONE',  ( 0.000000000000000000, 0.000000000000000000, -1.000000000000000000 ) ) ;
#24634=CARTESIAN_POINT ( 'NONE',  ( 12.13525491562420910, 79.19999999999998863, -8.816778784387098611 ) ) ;
#24636=CARTESIAN_POINT ( 'NONE',  ( -20.08610463437157989, 38.20000000546236407, -27.64615127144129758 ) ) ;
#24638=CARTESIAN_POINT ( 'NONE',  ( -33.58253175000000113, 35.12500000273119127, 0.000000000000000000 ) ) ;
#24641=CARTESIAN_POINT ( 'NONE',  ( -20.75514604977248112, 25.67500000273118488, 28.56700777964554661 ) ) ;
#24645=CARTESIAN_POINT ( 'NONE',  ( -10.04305231718579172, 44.10000000546238397, -30.90933677959248982 ) ) ;
#24648=CARTESIAN_POINT ( 'NONE',  ( -14.47279130897151767, 7.324999997268822227, -19.92008829642072598 ) ) ;
#24650=EDGE_CURVE ( 'NONE', #20831, #31469, #12456, .T. ) ;
#24651=CARTESIAN_POINT ( 'NONE',  ( 15.14183272437242422, 12.29999999999999183, -20.84094480462497856 ) ) ;
#24653=CARTESIAN_POINT ( 'NONE',  ( -32.50000000000000000, 60.00000000000000000, 0.000000000000000000 ) ) ;
#24654=CARTESIAN_POINT ( 'NONE',  ( -33.58253175000000113, 13.22500000273119802, 10.91162601494193929 ) ) ;
#24655=CARTESIAN_POINT ( 'NONE',  ( 7.236395654485755280, 4.724999997268803043, 22.27133577429736988 ) ) ;
#24658=ORIENTED_EDGE ( 'NONE', *, *, #26052, .T. ) ;
#24664=CARTESIAN_POINT ( 'NONE',  ( 24.50000000000000000, 17.74999999453763522, 0.000000000000000000 ) ) ;
#24665=EDGE_CURVE ( 'NONE', #17459, #18081, #12175, .T. ) ;
#24666=CARTESIAN_POINT ( 'NONE',  ( -23.41746825000000243, 3.524999997268826402, -7.608796670333730638 ) ) ;
#24667=CARTESIAN_POINT ( 'NONE',  ( 10.37757302488624767, 23.97500000273117138, 31.93888565452638417 ) ) ;
#24668=CARTESIAN_POINT ( 'NONE',  ( 20.08610463437158344, 31.20000000546238894, 27.64615127144129403 ) ) ;
#24669=CARTESIAN_POINT ( 'NONE',  ( 32.50000000000000000, 73.00000000000001421, -3.980102097228898626E-15 ) ) ;
#24670=CARTESIAN_POINT ( 'NONE',  ( 6.001560367445586717E-15, 3.249999994537631665, 24.50000000000000000 ) ) ;
#24671=CARTESIAN_POINT ( 'NONE',  ( 7.890940483122900408E-14, 10.49999999999999112, -24.50000000000000000 ) ) ;
#24673=CARTESIAN_POINT ( 'NONE',  ( 10.37757302488624056, 36.77500000273120406, -31.93888565452638417 ) ) ;
#24677=CARTESIAN_POINT ( 'NONE',  ( 14.47279130897151767, 7.424999997268820096, -19.92008829642072598 ) ) ;
#24678=CARTESIAN_POINT ( 'NONE',  ( -32.50000000000000000, 13.89999999999999858, -10.55989012756945478 ) ) ;
#24681=CARTESIAN_POINT ( 'NONE',  ( 10.37757302488624056, 60.52500000273119696, -31.93888565452638417 ) ) ;
#24682=CARTESIAN_POINT ( 'NONE',  ( -10.37757302488623701, 47.77500000273118985, 31.93888565452638417 ) ) ;
#24685=CARTESIAN_POINT ( 'NONE',  ( -33.58253175000000113, 5.025000002731194293, -10.91162601494193218 ) ) ;
#24687=CARTESIAN_POINT ( 'NONE',  ( 26.29305231718579350, 25.30000000546236905, 19.10302069950537529 ) ) ;
#24688=CARTESIAN_POINT ( 'NONE',  ( 2.067204126564591252E-14, 4.499999999999996447, -24.50000000000000000 ) ) ;
#24691=DIRECTION ( 'NONE',  ( 0.000000000000000000, -1.000000000000000000, 0.000000000000000000 ) ) ;
#24692=CARTESIAN_POINT ( 'NONE',  ( 0.000000000000000000, 80.00000000000001421, 0.000000000000000000 ) ) ;
#24698=ORIENTED_EDGE ( 'NONE', *, *, #22050, .T. ) ;
#24702=ORIENTED_EDGE ( 'NONE', *, *, #31274, .F. ) ;
#24706=CARTESIAN_POINT ( 'NONE',  ( 32.50000000000000000, 21.10000000000000142, -10.55989012756945833 ) ) ;
#24707=CARTESIAN_POINT ( 'NONE',  ( -27.16883889988623935, 45.57500000273117990, 19.73931689729374739 ) ) ;
#24708=CARTESIAN_POINT ( 'NONE',  ( -32.50000000000000000, 50.50000000546239676, 0.000000000000000000 ) ) ;
#24710=CARTESIAN_POINT ( 'NONE',  ( -33.58253175000000113, 27.12500000273118772, 0.000000000000000000 ) ) ;
#24712=CARTESIAN_POINT ( 'NONE',  ( -27.16883889988623935, 57.57500000273119412, 19.73931689729374739 ) ) ;
#24715=CARTESIAN_POINT ( 'NONE',  ( 32.50000000000000000, 33.00000000000000000, -3.980102097228898626E-15 ) ) ;
#24717=CARTESIAN_POINT ( 'NONE',  ( 33.58253175000000113, 2.375000002731192161, -4.112674001490185761E-15 ) ) ;
#24721=CARTESIAN_POINT ( 'NONE',  ( 20.75514604977248467, 64.67500000273116711, -28.56700777964554305 ) ) ;
#24722=CARTESIAN_POINT ( 'NONE',  ( -15.14183272437242067, 18.44999999453760964, -20.84094480462497856 ) ) ;
#24725=CARTESIAN_POINT ( 'NONE',  ( 19.82091636218621034, 7.549999994537620829, 14.40073868116559730 ) ) ;
#24727=CARTESIAN_POINT ( 'NONE',  ( 12.13525491562421088, 74.80000000000001137, 8.816778784387095058 ) ) ;
#24737=FACE_OUTER_BOUND ( 'NONE', #7275, .T. ) ;
#24738=CARTESIAN_POINT ( 'NONE',  ( 10.04305231718578817, 13.90000000546237580, -30.90933677959249337 ) ) ;
#24748=CARTESIAN_POINT ( 'NONE',  ( 20.08610463437158344, 26.70000000000000284, 27.64615127144129403 ) ) ;
#24749=CARTESIAN_POINT ( 'NONE',  ( 27.16883889988623935, 52.32500000273118701, -19.73931689729374384 ) ) ;
#24751=EDGE_CURVE ( 'NONE', #11875, #14813, #33214, .T. ) ;
#24752=CARTESIAN_POINT ( 'NONE',  ( 10.04305231718579705, 9.100000005462376862, 30.90933677959248982 ) ) ;
#24754=CARTESIAN_POINT ( 'NONE',  ( -23.41746825000000243, 18.22499999726879238, 7.608796670333725309 ) ) ;
#24755=CARTESIAN_POINT ( 'NONE',  ( -26.29305231718579350, 55.80000000000001847, -19.10302069950537884 ) ) ;
#24756=CARTESIAN_POINT ( 'NONE',  ( -10.37757302488623701, 25.77500000273119696, 31.93888565452638417 ) ) ;
#24758=CARTESIAN_POINT ( 'NONE',  ( -4.300734207923759378, 74.47500000273119269, -13.23629886949340495 ) ) ;
#24760=CARTESIAN_POINT ( 'NONE',  ( -1.778240108872766143E-15, 33.50000000000000000, -32.49999999999999289 ) ) ;
#24762=ORIENTED_EDGE ( 'NONE', *, *, #3570, .F. ) ;
#24769=CARTESIAN_POINT ( 'NONE',  ( 10.37757302488624767, 9.975000002731187365, 31.93888565452638417 ) ) ;
#24773=CARTESIAN_POINT ( 'NONE',  ( 2.688165632520823219E-15, 79.87500000273119838, 14.63369212191046209 ) ) ;
#24776=CARTESIAN_POINT ( 'NONE',  ( -20.75514604977248823, 54.82500000273118701, -28.56700777964554305 ) ) ;
#24778=ORIENTED_EDGE ( 'NONE', *, *, #24561, .T. ) ;
#24782=CARTESIAN_POINT ( 'NONE',  ( -23.41746825000000598, 7.724999997268809260, 7.608796670333726198 ) ) ;
#24784=ORIENTED_EDGE ( 'NONE', *, *, #29543, .F. ) ;
#24786=CARTESIAN_POINT ( 'NONE',  ( -26.29305231718579350, 34.30000000546237970, -19.10302069950537884 ) ) ;
#24789=CARTESIAN_POINT ( 'NONE',  ( 10.37757302488624056, 62.77500000273117564, -31.93888565452638417 ) ) ;
#24791=CARTESIAN_POINT ( 'NONE',  ( 33.58253175000000113, 74.22500000273119269, -10.91162601494193751 ) ) ;
#24793=CARTESIAN_POINT ( 'NONE',  ( -24.50000000000000000, 5.000000000000004441, -3.000384657911015469E-15 ) ) ;
#24794=CARTESIAN_POINT ( 'NONE',  ( -20.75514604977248112, 1.675000002731184434, 28.56700777964554661 ) ) ;
#24796=CARTESIAN_POINT ( 'NONE',  ( 10.37757302488624056, 14.52500000273118630, -31.93888565452638417 ) ) ;
#24798=CARTESIAN_POINT ( 'NONE',  ( -13.91746824999999532, 72.97500000273117848, 4.522059556121122093 ) ) ;
#24800=CARTESIAN_POINT ( 'NONE',  ( -15.00000000000000000, 79.90000000000001990, -4.873795443493594171 ) ) ;
#24804=CARTESIAN_POINT ( 'NONE',  ( 4.635254915624209993, 75.65000000546237402, -14.26584774442730463 ) ) ;
#24806=CARTESIAN_POINT ( 'NONE',  ( 20.75514604977248467, 36.42500000273118843, -28.56700777964554305 ) ) ;
#24809=CARTESIAN_POINT ( 'NONE',  ( 33.58253175000000113, 28.37500000273118772, -4.112674001490185761E-15 ) ) ;
#24810=EDGE_CURVE ( 'NONE', #24251, #32007, #13292, .T. ) ;
#24812=AXIS2_PLACEMENT_3D ( 'NONE', #13090, #26302, #18757 ) ;
#24814=CARTESIAN_POINT ( 'NONE',  ( -4.223320258572821363E-15, 80.49999999999998579, 15.00000000000000355 ) ) ;
#24816=CARTESIAN_POINT ( 'NONE',  ( 7.236395654485760609, 13.02499999726880375, -22.27133577429736633 ) ) ;
#24820=CARTESIAN_POINT ( 'NONE',  ( 10.37757302488624056, 14.52500000273118630, -31.93888565452638417 ) ) ;
#24821=CARTESIAN_POINT ( 'NONE',  ( -18.94512977948575738, 7.924999997268811214, -13.76444248337723231 ) ) ;
#24829=CARTESIAN_POINT ( 'NONE',  ( 5.779280353836490358E-15, 73.00000000546236834, 32.49999999999999289 ) ) ;
#24830=CARTESIAN_POINT ( 'NONE',  ( 24.50000000000000000, 13.74999999453763166, 0.000000000000000000 ) ) ;
#24832=CARTESIAN_POINT ( 'NONE',  ( -23.41746824999999887, 5.624999997268814944, -2.867812753649727150E-15 ) ) ;
#24833=CARTESIAN_POINT ( 'NONE',  ( -2.162160676586881955E-15, 20.87500000273119127, -35.31076352940723240 ) ) ;
#24834=CARTESIAN_POINT ( 'NONE',  ( 26.29305231718579350, 23.30000000546236905, 19.10302069950537529 ) ) ;
#24835=CARTESIAN_POINT ( 'NONE',  ( 32.50000000000000000, 71.00000000000001421, -3.980102097228898626E-15 ) ) ;
#24836=DIRECTION ( 'NONE',  ( 0.000000000000000000, -1.000000000000000000, 0.000000000000000000 ) ) ;
#24839=CARTESIAN_POINT ( 'NONE',  ( -27.16883889988623935, 33.57500000273120122, 19.73931689729374739 ) ) ;
#24843=CARTESIAN_POINT ( 'NONE',  ( -4.523095164977116484E-15, 8.624999997268810503, 24.62258325217400312 ) ) ;
#24844=CARTESIAN_POINT ( 'NONE',  ( -10.04305231718579172, 17.60000000000000497, -30.90933677959248982 ) ) ;
#24847=CARTESIAN_POINT ( 'NONE',  ( 33.58253175000000113, 56.22500000273117138, -10.91162601494193751 ) ) ;
#24848=CARTESIAN_POINT ( 'NONE',  ( -27.16883889988624290, 47.17500000273119554, -19.73931689729374028 ) ) ;
#24850=CARTESIAN_POINT ( 'NONE',  ( 23.95873412499999944, 0.3124999986344190184, 0.000000000000000000 ) ) ;
#24851=CARTESIAN_POINT ( 'NONE',  ( 5.779280353836490358E-15, 6.500000000000002665, 32.49999999999999289 ) ) ;
#24854=CYLINDRICAL_SURFACE ( 'NONE', #19860, 32.50000000000000000 ) ;
#24858=VECTOR ( 'NONE', #26059, 1000.000000000000000 ) ;
#24859=CARTESIAN_POINT ( 'NONE',  ( 24.50000000000000000, 14.00000000000001243, 0.000000000000000000 ) ) ;
#24862=CARTESIAN_POINT ( 'NONE',  ( -27.16883889988624290, 32.92500000273118843, -19.73931689729374028 ) ) ;
#24864=ORIENTED_EDGE ( 'NONE', *, *, #17404, .T. ) ;
#24867=DIRECTION ( 'NONE',  ( -0.000000000000000000, -1.000000000000000000, -0.000000000000000000 ) ) ;
#24872=CARTESIAN_POINT ( 'NONE',  ( 32.50000000000000000, 56.99999999999999289, -3.980102097228898626E-15 ) ) ;
#24873=CARTESIAN_POINT ( 'NONE',  ( 20.75514604977248467, 42.67500000273119554, -28.56700777964554305 ) ) ;
#24874=CARTESIAN_POINT ( 'NONE',  ( 20.08610463437157279, 47.80000000546239391, -27.64615127144129758 ) ) ;
#24875=EDGE_CURVE ( 'NONE', #7013, #31666, #21617, .T. ) ;
#24877=CARTESIAN_POINT ( 'NONE',  ( 27.16883889988623935, 28.32500000273119412, -19.73931689729374384 ) ) ;
#24879=VECTOR ( 'NONE', #30330, 1000.000000000000000 ) ;
#24880=CARTESIAN_POINT ( 'NONE',  ( 33.58253175000000113, 58.37500000273118417, -4.112674001490185761E-15 ) ) ;
#24882=CARTESIAN_POINT ( 'NONE',  ( 32.50000000000000000, 37.09999999999999432, -10.55989012756945833 ) ) ;
#24884=CARTESIAN_POINT ( 'NONE',  ( 27.16883889988624290, 73.92500000273119554, 19.73931689729373673 ) ) ;
#24885=CARTESIAN_POINT ( 'NONE',  ( 5.779280353836490358E-15, 2.500000000000005329, 32.49999999999999289 ) ) ;
#24887=CARTESIAN_POINT ( 'NONE',  ( 10.37757302488624056, 66.77500000273117564, -31.93888565452638417 ) ) ;
#24890=FACE_OUTER_BOUND ( 'NONE', #7106, .T. ) ;
#24897=( BOUNDED_CURVE ( )  B_SPLINE_CURVE ( 2, ( #32602, #3623, #9263, #29685, #9101, #13758, #12703, #12014, #25232, #30711, #2058, #23003, #9786 ),
 .UNSPECIFIED., .F., .T. ) 
 B_SPLINE_CURVE_WITH_KNOTS ( ( 3, 2, 2, 2, 2, 2, 3 ),
 ( 0.09615384615384615918, 0.09743589743589743668, 0.1000000000000000056, 0.1025641025641025605, 0.1051282051282051294, 0.1076923076923076983, 0.1089743589743589758 ),
 .UNSPECIFIED. ) 
 CURVE ( )  GEOMETRIC_REPRESENTATION_ITEM ( )  RATIONAL_B_SPLINE_CURVE ( ( 0.9755282581475767101, 0.9755282581475768211, 1.000000000000000000, 0.9510565162951535312, 1.000000000000000000, 0.9510565162951535312, 1.000000000000000000, 0.9510565162951535312, 1.000000000000000000, 0.9510565162951535312, 1.000000000000000000, 0.9755282581475768211, 0.9755282581475768211 ) ) 
 REPRESENTATION_ITEM ( '' )  );
#24903=( BOUNDED_CURVE ( )  B_SPLINE_CURVE ( 2, ( #30269, #25307, #25131, #19817, #22229, #12257, #30096, #6603, #33007, #3862, #4027, #22734, #20168 ),
 .UNSPECIFIED., .F., .T. ) 
 B_SPLINE_CURVE_WITH_KNOTS ( ( 3, 2, 2, 2, 2, 2, 3 ),
 ( 0.5320512820512820484, 0.5333333333333333259, 0.5358974358974358809, 0.5384615384615384359, 0.5410256410256409909, 0.5435897435897435459, 0.5448717948717948234 ),
 .UNSPECIFIED. ) 
 CURVE ( )  GEOMETRIC_REPRESENTATION_ITEM ( )  RATIONAL_B_SPLINE_CURVE ( ( 0.9755282581475768211, 0.9755282581475768211, 1.000000000000000000, 0.9510565162951535312, 1.000000000000000000, 0.9510565162951535312, 1.000000000000000000, 0.9510565162951535312, 1.000000000000000000, 0.9510565162951535312, 1.000000000000000000, 0.9755282581475768211, 0.9755282581475768211 ) ) 
 REPRESENTATION_ITEM ( '' )  );
#24905=CARTESIAN_POINT ( 'NONE',  ( -10.04305231718579172, 57.59999999999998721, -30.90933677959248982 ) ) ;
#24906=CARTESIAN_POINT ( 'NONE',  ( -1.778240108872766143E-15, 35.49999999999998579, -32.49999999999999289 ) ) ;
#24907=ORIENTED_EDGE ( 'NONE', *, *, #3887, .T. ) ;
#24909=CARTESIAN_POINT ( 'NONE',  ( -5.147494310547418017, 75.55125428154684641, -32.50000000000000000 ) ) ;
#24913=ORIENTED_EDGE ( 'NONE', *, *, #15322, .F. ) ;
#24915=CARTESIAN_POINT ( 'NONE',  ( 26.29305231718578995, 27.20000000000000284, -19.10302069950538240 ) ) ;
#24916=CARTESIAN_POINT ( 'NONE',  ( -2.162160676586881955E-15, 46.62500000273119127, -35.31076352940723240 ) ) ;
#24918=CARTESIAN_POINT ( 'NONE',  ( 6.277390505771533514E-15, 15.00000000546237722, 34.17252228774368916 ) ) ;
#24920=CARTESIAN_POINT ( 'NONE',  ( -14.47279130897151767, 15.82499999726881512, -19.92008829642072598 ) ) ;
#24921=CARTESIAN_POINT ( 'NONE',  ( 20.08610463437157279, 51.29999999999997584, -27.64615127144129758 ) ) ;
#24922=DIRECTION ( 'NONE',  ( 0.000000000000000000, 0.000000000000000000, 1.000000000000000000 ) ) ;
#24923=CARTESIAN_POINT ( 'NONE',  ( 6.486482029760649416E-15, 21.87500000273118062, 35.31076352940723240 ) ) ;
#24924=CARTESIAN_POINT ( 'NONE',  ( -5.147494310547423346, 24.94874572391553613, 32.50000000000000000 ) ) ;
#24926=CARTESIAN_POINT ( 'NONE',  ( -8.601468415847518756, 74.57500000273117280, -11.83890561707634781 ) ) ;
#24927=CARTESIAN_POINT ( 'NONE',  ( 5.779280353836490358E-15, 36.49999999999998579, 32.49999999999999289 ) ) ;
#24928=CARTESIAN_POINT ( 'NONE',  ( -32.50000000000000000, 28.50000000546237899, 0.000000000000000000 ) ) ;
#24930=ORIENTED_EDGE ( 'NONE', *, *, #13366, .F. ) ;
#24932=DIRECTION ( 'NONE',  ( -0.000000000000000000, -1.000000000000000000, -0.000000000000000000 ) ) ;
#24937=CARTESIAN_POINT ( 'NONE',  ( -33.58253175000000113, 9.375000002731169957, 0.000000000000000000 ) ) ;
#24941=CARTESIAN_POINT ( 'NONE',  ( 13.91746824999999532, 76.47500000273117848, -4.522059556121118540 ) ) ;
#24944=CARTESIAN_POINT ( 'NONE',  ( -15.14183272437242067, 2.449999994537622960, -20.84094480462497856 ) ) ;
#24945=CARTESIAN_POINT ( 'NONE',  ( -27.16883889988624290, 52.92500000273120264, -19.73931689729374028 ) ) ;
#24948=ORIENTED_EDGE ( 'NONE', *, *, #27898, .F. ) ;
#24950=CARTESIAN_POINT ( 'NONE',  ( 5.147494310547426899, 17.44874571845315359, -32.50000000000000000 ) ) ;
#24951=CARTESIAN_POINT ( 'NONE',  ( 14.47279130897151767, 12.92499999726881832, -19.92008829642072598 ) ) ;
#24953=ORIENTED_EDGE ( 'NONE', *, *, #9492, .F. ) ;
#24958=CARTESIAN_POINT ( 'NONE',  ( 27.16883889988623935, 58.57500000273119412, -19.73931689729374384 ) ) ;
#24960=DIRECTION ( 'NONE',  ( -0.000000000000000000, -1.000000000000000000, -0.000000000000000000 ) ) ;
#24961=CARTESIAN_POINT ( 'NONE',  ( 6.486482029760649416E-15, 67.62500000273119838, 35.31076352940723240 ) ) ;
#24962=VECTOR ( 'NONE', #31992, 1000.000000000000000 ) ;
#24964=CARTESIAN_POINT ( 'NONE',  ( -24.50000000000000000, 15.00000000000001421, -3.000384657911015469E-15 ) ) ;
#24965=CARTESIAN_POINT ( 'NONE',  ( 33.58253175000000113, 4.375000002731193938, -4.112674001490185761E-15 ) ) ;
#24966=CARTESIAN_POINT ( 'NONE',  ( -27.16883889988624290, 18.92500000273117422, -19.73931689729374028 ) ) ;
#24967=CARTESIAN_POINT ( 'NONE',  ( 5.779280353836490358E-15, 1.000000005462375885, 32.49999999999999289 ) ) ;
#24969=CARTESIAN_POINT ( 'NONE',  ( -4.635254915624211769, 81.60000000000000853, -14.26584774442730286 ) ) ;
#24973=CARTESIAN_POINT ( 'NONE',  ( 4.635254915624212657, 74.85000000546237686, 14.26584774442730286 ) ) ;
#24975=CARTESIAN_POINT ( 'NONE',  ( -10.37757302488624411, 36.72500000273118559, -31.93888565452638417 ) ) ;
#24978=CARTESIAN_POINT ( 'NONE',  ( -10.37757302488624411, 26.97500000273117493, -31.93888565452638417 ) ) ;
#24979=CARTESIAN_POINT ( 'NONE',  ( -10.04305231718579172, 12.10000000546238041, -30.90933677959248982 ) ) ;
#24980=CARTESIAN_POINT ( 'NONE',  ( -32.50000000000000000, 8.400000005462382902, -10.55989012756945300 ) ) ;
#24985=CARTESIAN_POINT ( 'NONE',  ( 23.41746824999999887, 10.62499999726881938, 0.000000000000000000 ) ) ;
#24987=EDGE_CURVE ( 'NONE', #11703, #6044, #19209, .T. ) ;
#24991=CARTESIAN_POINT ( 'NONE',  ( -33.58253175000000113, 11.12500000273120015, 0.000000000000000000 ) ) ;
#24992=CARTESIAN_POINT ( 'NONE',  ( 7.236395654485755280, 12.72499999726881015, 22.27133577429736988 ) ) ;
#24994=VERTEX_POINT ( 'NONE', #7636 ) ;
#24997=( BOUNDED_CURVE ( )  B_SPLINE_CURVE ( 2, ( #21112, #10128, #5483, #20778, #5313, #7547, #18372 ),
 .UNSPECIFIED., .F., .T. ) 
 B_SPLINE_CURVE_WITH_KNOTS ( ( 3, 2, 2, 3 ),
 ( 0.000000000000000000, 0.02000000000000000042, 0.04000000000000000083, 0.05000000000000000971 ),
 .UNSPECIFIED. ) 
 CURVE ( )  GEOMETRIC_REPRESENTATION_ITEM ( )  RATIONAL_B_SPLINE_CURVE ( ( 1.000000000000000000, 0.9510565162951535312, 1.000000000000000000, 0.9510565162951535312, 1.000000000000000000, 0.9755282581475768211, 0.9755282581475768211 ) ) 
 REPRESENTATION_ITEM ( '' )  );
#24998=ORIENTED_EDGE ( 'NONE', *, *, #20285, .T. ) ;
#25002=CARTESIAN_POINT ( 'NONE',  ( -4.732186688966233175E-15, 19.24999999453764232, 25.76082449383753925 ) ) ;
#25003=CARTESIAN_POINT ( 'NONE',  ( 23.41746825000000243, 6.524999997268818852, 7.608796670333735079 ) ) ;
#25004=CARTESIAN_POINT ( 'NONE',  ( -20.75514604977248112, 21.67500000273119554, 28.56700777964554661 ) ) ;
#25005=CARTESIAN_POINT ( 'NONE',  ( 6.277390505771533514E-15, 23.00000000546238610, 34.17252228774368916 ) ) ;
#25006=CARTESIAN_POINT ( 'NONE',  ( 10.04305231718578817, 71.40000000000001990, -30.90933677959249337 ) ) ;
#25007=CARTESIAN_POINT ( 'NONE',  ( 5.779280353836490358E-15, 33.00000000546238965, 32.49999999999999289 ) ) ;
#25010=CARTESIAN_POINT ( 'NONE',  ( 33.58253175000000113, 36.47500000273119269, -10.91162601494193751 ) ) ;
#25014=AXIS2_PLACEMENT_3D ( 'NONE', #26601, #2589, #26263 ) ;
#25015=CARTESIAN_POINT ( 'NONE',  ( -23.41746824999999887, 12.12499999726882116, -2.867812753649727150E-15 ) ) ;
#25016=CARTESIAN_POINT ( 'NONE',  ( -32.50000000000000000, 14.09999999999999254, 10.55989012756946366 ) ) ;
#25019=CARTESIAN_POINT ( 'NONE',  ( 6.486482029760649416E-15, 57.62500000273119127, 35.31076352940723240 ) ) ;
#25020=CARTESIAN_POINT ( 'NONE',  ( -33.58253175000000113, 47.27500000273116854, -10.91162601494193041 ) ) ;
#25021=CARTESIAN_POINT ( 'NONE',  ( 32.50000000000000711, 44.90000000000001279, 10.55989012756945122 ) ) ;
#25026=CARTESIAN_POINT ( 'NONE',  ( -4.223320258572819786E-15, 3.500000000000004441, 24.50000000000000000 ) ) ;
#25028=FACE_OUTER_BOUND ( 'NONE', #6030, .T. ) ;
#25030=CARTESIAN_POINT ( 'NONE',  ( 0.000000000000000000, 80.00000000000001421, -32.50000000000000000 ) ) ;
#25033=CARTESIAN_POINT ( 'NONE',  ( 15.00000000000000000, 71.25000000546238255, -1.836970198721029589E-15 ) ) ;
#25034=CARTESIAN_POINT ( 'NONE',  ( 27.16883889988623935, 34.32500000273120122, -19.73931689729374384 ) ) ;
#25041=ORIENTED_EDGE ( 'NONE', *, *, #26052, .F. ) ;
#25044=AXIS2_PLACEMENT_3D ( 'NONE', #22382, #1259, #6761 ) ;
#25046=CARTESIAN_POINT ( 'NONE',  ( 10.04305231718578817, 57.40000000000000568, -30.90933677959249337 ) ) ;
#25047=CARTESIAN_POINT ( 'NONE',  ( -10.37757302488624411, 40.97500000273118559, -31.93888565452638417 ) ) ;
#25048=CARTESIAN_POINT ( 'NONE',  ( 6.277390505771533514E-15, 43.00000000546236123, 34.17252228774368916 ) ) ;
#25050=CARTESIAN_POINT ( 'NONE',  ( -2.162160676586881955E-15, 30.62500000273119838, -35.31076352940723240 ) ) ;
#25051=CARTESIAN_POINT ( 'NONE',  ( -32.50000000000000000, 23.99999999999999289, 0.000000000000000000 ) ) ;
#25052=CARTESIAN_POINT ( 'NONE',  ( 27.16883889988624290, 54.17500000273117422, 19.73931689729373673 ) ) ;
#25054=CARTESIAN_POINT ( 'NONE',  ( 32.50000000000000711, 32.89999999999997726, 10.55989012756945122 ) ) ;
#25056=CARTESIAN_POINT ( 'NONE',  ( 27.16883889988624290, 77.92500000273116711, 19.73931689729373673 ) ) ;
#25059=CARTESIAN_POINT ( 'NONE',  ( 27.16883889988623935, 68.57500000273120122, -19.73931689729374384 ) ) ;
#25061=ORIENTED_EDGE ( 'NONE', *, *, #18602, .F. ) ;
#25062=DIRECTION ( 'NONE',  ( -0.000000000000000000, 1.000000000000000000, -0.000000000000000000 ) ) ;
#25064=CARTESIAN_POINT ( 'NONE',  ( 24.50000000000000000, 7.649999994537632908, 7.960532557706212486 ) ) ;
#25081=ADVANCED_FACE ( 'NONE', ( #12790 ), #23264, .T. ) ;
#25084=CARTESIAN_POINT ( 'NONE',  ( 32.50000000000000000, 61.50000000546238255, -3.980102097228898626E-15 ) ) ;
#25085=EDGE_LOOP ( 'NONE', ( #26983, #15358, #16990, #12343 ) ) ;
#25087=CARTESIAN_POINT ( 'NONE',  ( -33.58253175000000113, 51.02500000273119696, -10.91162601494193218 ) ) ;
#25088=CARTESIAN_POINT ( 'NONE',  ( 20.08610463437158344, 55.20000000546238539, 27.64615127144129403 ) ) ;
#25090=CARTESIAN_POINT ( 'NONE',  ( 26.29305231718579350, 13.30000000546238681, 19.10302069950537529 ) ) ;
#25091=EDGE_CURVE ( 'NONE', #19067, #7360, #9572, .T. ) ;
#25093=CARTESIAN_POINT ( 'NONE',  ( -18.94512977948575738, 17.92499999726882010, -13.76444248337723231 ) ) ;
#25095=CARTESIAN_POINT ( 'NONE',  ( 6.277390505771533514E-15, 50.50000000000000000, 34.17252228774368916 ) ) ;
#25096=CARTESIAN_POINT ( 'NONE',  ( 7.570916362186207671, 1.599999999999990319, 23.30088464923126779 ) ) ;
#25097=CARTESIAN_POINT ( 'NONE',  ( 27.16883889988624290, 20.17500000273120264, 19.73931689729373673 ) ) ;
#25098=CARTESIAN_POINT ( 'NONE',  ( 15.00000000000000000, 77.09999999999998010, -4.873795443493596835 ) ) ;
#25100=CARTESIAN_POINT ( 'NONE',  ( 13.91746825000000065, 71.77500000273120406, 4.522059556121114987 ) ) ;
#25101=CARTESIAN_POINT ( 'NONE',  ( -3.880418787951142701, 13.44874571845315536, 24.49999999999999645 ) ) ;
#25102=CARTESIAN_POINT ( 'NONE',  ( -32.50000000000000000, 22.09999999999999787, 10.55989012756946366 ) ) ;
#25105=ORIENTED_EDGE ( 'NONE', *, *, #32006, .T. ) ;
#25107=CARTESIAN_POINT ( 'NONE',  ( 8.601468415847516980, 72.17500000273118133, -11.83890561707634781 ) ) ;
#25109=( BOUNDED_CURVE ( )  B_SPLINE_CURVE ( 2, ( #29596, #11582, #8675, #22063, #604, #29269, #5772, #32010, #16252, #26708, #26871, #24137, #8505 ),
 .UNSPECIFIED., .F., .T. ) 
 B_SPLINE_CURVE_WITH_KNOTS ( ( 3, 2, 2, 2, 2, 2, 3 ),
 ( 0.1388888888888888673, 0.1444444444444444309, 0.1555555555555555580, 0.1666666666666666574, 0.1777777777777777846, 0.1888888888888888840, 0.1944444444444444475 ),
 .UNSPECIFIED. ) 
 CURVE ( )  GEOMETRIC_REPRESENTATION_ITEM ( )  RATIONAL_B_SPLINE_CURVE ( ( 0.9755282581475768211, 0.9755282581475768211, 1.000000000000000000, 0.9510565162951535312, 1.000000000000000000, 0.9510565162951535312, 1.000000000000000000, 0.9510565162951535312, 1.000000000000000000, 0.9510565162951535312, 1.000000000000000000, 0.9755282581475768211, 0.9755282581475768211 ) ) 
 REPRESENTATION_ITEM ( '' )  );
#25113=CARTESIAN_POINT ( 'NONE',  ( -33.58253175000000113, 5.275000002731187188, -10.91162601494193041 ) ) ;
#25116=CARTESIAN_POINT ( 'NONE',  ( 5.779280353836490358E-15, 62.50000000000000000, 32.49999999999999289 ) ) ;
#25118=CARTESIAN_POINT ( 'NONE',  ( -20.75514604977248112, 53.42500000273117422, 28.56700777964554661 ) ) ;
#25122=CARTESIAN_POINT ( 'NONE',  ( 5.147494310547434893, 16.55125428154684641, 32.49999999999999289 ) ) ;
#25123=CARTESIAN_POINT ( 'NONE',  ( 23.41746824999999887, 10.62499999726881938, 0.000000000000000000 ) ) ;
#25130=CARTESIAN_POINT ( 'NONE',  ( 20.75514604977248467, 58.67500000273118843, -28.56700777964554305 ) ) ;
#25131=CARTESIAN_POINT ( 'NONE',  ( -10.04305231718578462, 36.90000000546236691, 30.90933677959249337 ) ) ;
#25132=CARTESIAN_POINT ( 'NONE',  ( -20.75514604977248823, 70.82500000273117280, -28.56700777964554305 ) ) ;
#25134=CARTESIAN_POINT ( 'NONE',  ( -7.570916362186215665, 13.39999999999999503, 23.30088464923126423 ) ) ;
#25135=CARTESIAN_POINT ( 'NONE',  ( -10.37757302488624411, 2.975000002731182036, -31.93888565452638417 ) ) ;
#25136=EDGE_CURVE ( 'NONE', #5936, #30261, #26227, .T. ) ;
#25137=CARTESIAN_POINT ( 'NONE',  ( -33.58253175000000113, 11.12500000273120015, 0.000000000000000000 ) ) ;
#25138=CARTESIAN_POINT ( 'NONE',  ( -8.601468415847515203, 73.17500000273119554, 11.83890561707634959 ) ) ;
#25140=CARTESIAN_POINT ( 'NONE',  ( 20.08610463437157279, 37.30000000000001137, -27.64615127144129758 ) ) ;
#25143=CARTESIAN_POINT ( 'NONE',  ( 10.04305231718578817, 61.90000000546235981, -30.90933677959249337 ) ) ;
#25145=FACE_OUTER_BOUND ( 'NONE', #33753, .T. ) ;
#25147=CARTESIAN_POINT ( 'NONE',  ( 33.58253175000000113, 40.22500000273119269, -10.91162601494193751 ) ) ;
#25150=CARTESIAN_POINT ( 'NONE',  ( 27.16883889988624290, 26.17500000273118133, 19.73931689729373673 ) ) ;
#25151=CARTESIAN_POINT ( 'NONE',  ( -1.778240108872766143E-15, 41.49999999999999289, -32.49999999999999289 ) ) ;
#25152=CARTESIAN_POINT ( 'NONE',  ( -5.147494310547640062, 8.948745723915518369, 32.49999999999992895 ) ) ;
#25153=CARTESIAN_POINT ( 'NONE',  ( 5.147494310547429563, 79.44874571845315359, -32.50000000000000000 ) ) ;
#25155=CARTESIAN_POINT ( 'NONE',  ( 14.47279130897151944, 8.924999997268800556, -19.92008829642072598 ) ) ;
#25160=CARTESIAN_POINT ( 'NONE',  ( -33.58253175000000113, 13.12500000273120193, 0.000000000000000000 ) ) ;
#25161=CARTESIAN_POINT ( 'NONE',  ( -14.47279130897152122, 12.42499999726880766, 19.92008829642072243 ) ) ;
#25163=ORIENTED_EDGE ( 'NONE', *, *, #21114, .F. ) ;
#25170=CARTESIAN_POINT ( 'NONE',  ( -24.50000000000000355, 16.64999999453763735, -7.960532557706207157 ) ) ;
#25171=CARTESIAN_POINT ( 'NONE',  ( 7.236395654485755280, 12.22499999726881015, 22.27133577429736988 ) ) ;
#25173=CARTESIAN_POINT ( 'NONE',  ( 33.58253175000000823, 20.27500000273117564, 10.91162601494192863 ) ) ;
#25174=CARTESIAN_POINT ( 'NONE',  ( 10.04305231718579705, 23.10000000546236265, 30.90933677959248982 ) ) ;
#25175=EDGE_CURVE ( 'NONE', #3077, #24457, #15713, .T. ) ;
#25176=CARTESIAN_POINT ( 'NONE',  ( -20.08610463437156923, 70.30000000000001137, 27.64615127144130113 ) ) ;
#25177=CARTESIAN_POINT ( 'NONE',  ( 20.08610463437157279, 47.80000000546238681, -27.64615127144129758 ) ) ;
#25180=CARTESIAN_POINT ( 'NONE',  ( -10.37757302488624411, 38.97500000273118559, -31.93888565452638417 ) ) ;
#25181=CARTESIAN_POINT ( 'NONE',  ( -8.601468415847518756, 81.07500000273120122, -11.83890561707634781 ) ) ;
#25185=CARTESIAN_POINT ( 'NONE',  ( -4.523095164977116484E-15, 12.62499999726879985, 24.62258325217400312 ) ) ;
#25186=CARTESIAN_POINT ( 'NONE',  ( 10.04305231718579705, 12.59999999999999964, 30.90933677959248982 ) ) ;
#25189=CARTESIAN_POINT ( 'NONE',  ( -10.37757302488624411, 58.72500000273117848, -31.93888565452638417 ) ) ;
#25190=CARTESIAN_POINT ( 'NONE',  ( -2.162160676586882350E-15, 48.87500000273117706, -35.31076352940722529 ) ) ;
#25193=CARTESIAN_POINT ( 'NONE',  ( 20.75514604977249178, 1.825000002731179460, 28.56700777964553950 ) ) ;
#25196=CARTESIAN_POINT ( 'NONE',  ( -26.29305231718578995, 42.20000000000001705, 19.10302069950538595 ) ) ;
#25198=DIRECTION ( 'NONE',  ( -0.000000000000000000, -1.000000000000000000, -0.000000000000000000 ) ) ;
#25200=CARTESIAN_POINT ( 'NONE',  ( 5.147494310547434893, 41.05125428700921475, 32.49999999999999289 ) ) ;
#25203=( BOUNDED_CURVE ( )  B_SPLINE_CURVE ( 2, ( #20223, #30663, #7160, #17643, #25535, #27343, #29113, #18504, #18674, #28950, #1068, #26384, #21411 ),
 .UNSPECIFIED., .F., .T. ) 
 B_SPLINE_CURVE_WITH_KNOTS ( ( 3, 2, 2, 2, 2, 2, 3 ),
 ( 0.02777777777777777624, 0.03333333333333333287, 0.04444444444444444614, 0.05555555555555555247, 0.06666666666666667962, 0.07777777777777777901, 0.08333333333333334259 ),
 .UNSPECIFIED. ) 
 CURVE ( )  GEOMETRIC_REPRESENTATION_ITEM ( )  RATIONAL_B_SPLINE_CURVE ( ( 0.9755282581475768211, 0.9755282581475768211, 1.000000000000000000, 0.9510565162951535312, 1.000000000000000000, 0.9510565162951535312, 1.000000000000000000, 0.9510565162951535312, 1.000000000000000000, 0.9510565162951535312, 1.000000000000000000, 0.9755282581475767101, 0.9755282581475768211 ) ) 
 REPRESENTATION_ITEM ( '' )  );
#25204=CARTESIAN_POINT ( 'NONE',  ( -32.50000000000000000, 60.50000000546237544, 0.000000000000000000 ) ) ;
#25205=CARTESIAN_POINT ( 'NONE',  ( -2.162160676586882350E-15, 30.62500000273119838, -35.31076352940722529 ) ) ;
#25208=ORIENTED_EDGE ( 'NONE', *, *, #23447, .T. ) ;
#25211=CARTESIAN_POINT ( 'NONE',  ( -1.778240108872766143E-15, 69.49999999999998579, -32.49999999999999289 ) ) ;
#25212=EDGE_LOOP ( 'NONE', ( #17664, #2042, #26132, #3643 ) ) ;
#25218=LINE ( 'NONE', #2212, #6964 ) ;
#25219=CARTESIAN_POINT ( 'NONE',  ( 10.37757302488624056, 38.77500000273118275, -31.93888565452638417 ) ) ;
#25220=CARTESIAN_POINT ( 'NONE',  ( -26.29305231718579350, 42.30000000546238681, -19.10302069950537884 ) ) ;
#25222=CARTESIAN_POINT ( 'NONE',  ( 33.58253175000000113, 32.12500000273119127, -4.112674001490185761E-15 ) ) ;
#25224=CARTESIAN_POINT ( 'NONE',  ( -33.58253175000000113, 53.27500000273117564, -10.91162601494193218 ) ) ;
#25226=EDGE_CURVE ( 'NONE', #13932, #15993, #29705, .T. ) ;
#25229=CARTESIAN_POINT ( 'NONE',  ( 6.277390505771533514E-15, 32.49999999999999289, 34.17252228774368916 ) ) ;
#25231=CARTESIAN_POINT ( 'NONE',  ( 10.37757302488624056, 78.52500000273118985, -31.93888565452638417 ) ) ;
#25232=CARTESIAN_POINT ( 'NONE',  ( -26.29305231718579350, 70.30000000546237970, -19.10302069950537884 ) ) ;
#25233=CARTESIAN_POINT ( 'NONE',  ( -32.50000000000000000, 38.00000000000000711, 0.000000000000000000 ) ) ;
#25234=CARTESIAN_POINT ( 'NONE',  ( 27.16883889988624290, 68.17500000273119554, 19.73931689729373673 ) ) ;
#25237=CARTESIAN_POINT ( 'NONE',  ( -33.58253175000000113, 15.22500000273119447, 10.91162601494193929 ) ) ;
#25238=CARTESIAN_POINT ( 'NONE',  ( 15.14183272437242245, 8.049999994537621717, -20.84094480462497856 ) ) ;
#25240=DIRECTION ( 'NONE',  ( -0.000000000000000000, -1.000000000000000000, -0.000000000000000000 ) ) ;
#25249=DIRECTION ( 'NONE',  ( -0.000000000000000000, -1.000000000000000000, -0.000000000000000000 ) ) ;
#25250=CARTESIAN_POINT ( 'NONE',  ( -32.50000000000000000, 74.60000000546234844, 10.55989012756946366 ) ) ;
#25255=CARTESIAN_POINT ( 'NONE',  ( 27.16883889988624290, 72.17500000273119554, 19.73931689729373673 ) ) ;
#25259=CARTESIAN_POINT ( 'NONE',  ( 26.29305231718578995, 65.70000000546238539, -19.10302069950538240 ) ) ;
#25261=CARTESIAN_POINT ( 'NONE',  ( -24.50000000000000000, 12.64999999453762136, -7.960532557706207157 ) ) ;
#25262=AXIS2_PLACEMENT_3D ( 'NONE', #23469, #23638, #10422 ) ;
#25263=CARTESIAN_POINT ( 'NONE',  ( -10.37757302488623701, 47.52500000273118985, 31.93888565452638417 ) ) ;
#25264=CARTESIAN_POINT ( 'NONE',  ( 23.41746825000000243, 16.72499999726881725, -7.608796670333727974 ) ) ;
#25266=CARTESIAN_POINT ( 'NONE',  ( -32.50000000000000000, 8.500000005462361230, 0.000000000000000000 ) ) ;
#25269=CARTESIAN_POINT ( 'NONE',  ( -2.092463501923844636E-15, 55.49999999999999289, -34.17252228774368916 ) ) ;
#25270=CARTESIAN_POINT ( 'NONE',  ( 7.570916362186213000, 2.400000000000013234, -23.30088464923126423 ) ) ;
#25271=CARTESIAN_POINT ( 'NONE',  ( -10.37757302488623701, 17.77500000273118985, 31.93888565452638417 ) ) ;
#25272=CARTESIAN_POINT ( 'NONE',  ( 24.50000000000000000, 0.000000000000000000, 0.000000000000000000 ) ) ;
#25274=CARTESIAN_POINT ( 'NONE',  ( 11.25946833292375793, 72.07500000273120122, -8.180482586598735395 ) ) ;
#25276=CARTESIAN_POINT ( 'NONE',  ( -32.50000000000000000, 43.99999999999998579, 0.000000000000000000 ) ) ;
#25280=CARTESIAN_POINT ( 'NONE',  ( -4.934616302121927505E-14, 71.00000000546238255, 32.50000000000000000 ) ) ;
#25281=AXIS2_PLACEMENT_3D ( 'NONE', #27319, #3809, #14280 ) ;
#25286=CARTESIAN_POINT ( 'NONE',  ( -20.75514604977248823, 3.075000002731198112, -28.56700777964554305 ) ) ;
#25290=CARTESIAN_POINT ( 'NONE',  ( 26.29305231718579350, 68.79999999999999716, 19.10302069950537529 ) ) ;
#25294=CARTESIAN_POINT ( 'NONE',  ( -27.16883889988624290, 42.92500000273119554, -19.73931689729374028 ) ) ;
#25300=CARTESIAN_POINT ( 'NONE',  ( 32.50000000000000711, 16.89999999999998792, 10.55989012756945122 ) ) ;
#25301=CARTESIAN_POINT ( 'NONE',  ( 7.236395654485755280, 12.22499999726881015, 22.27133577429736988 ) ) ;
#25303=VERTEX_POINT ( 'NONE', #30068 ) ;
#25305=DIRECTION ( 'NONE',  ( -0.000000000000000000, -1.000000000000000000, -0.000000000000000000 ) ) ;
#25307=CARTESIAN_POINT ( 'NONE',  ( -5.147494310547423346, 36.94874572391552903, 32.50000000000000000 ) ) ;
#25308=CARTESIAN_POINT ( 'NONE',  ( 27.16883889988623935, 66.32500000273117280, -19.73931689729374384 ) ) ;
#25310=CARTESIAN_POINT ( 'NONE',  ( 24.50000000000000000, 10.00000000000000888, 0.000000000000000000 ) ) ;
#25311=CARTESIAN_POINT ( 'NONE',  ( 20.75514604977249178, 2.075000002731171467, 28.56700777964553950 ) ) ;
#25312=CARTESIAN_POINT ( 'NONE',  ( 10.37757302488624767, 7.725000002731185589, 31.93888565452638417 ) ) ;
#25313=CARTESIAN_POINT ( 'NONE',  ( 20.08610463437157279, 29.30000000000000782, -27.64615127144129758 ) ) ;
#25315=CARTESIAN_POINT ( 'NONE',  ( 15.00000000000000355, 72.90000000000000568, 4.873795443493592394 ) ) ;
#25320=CARTESIAN_POINT ( 'NONE',  ( 15.00000000000000355, 77.15000000546240244, 4.873795443493592394 ) ) ;
#25322=CARTESIAN_POINT ( 'NONE',  ( -10.37757302488623701, 37.52500000273117564, 31.93888565452638417 ) ) ;
#25325=CARTESIAN_POINT ( 'NONE',  ( -33.58253175000000113, 23.27500000273116854, -10.91162601494193041 ) ) ;
#25326=CARTESIAN_POINT ( 'NONE',  ( -32.50000000000000000, 18.00000000000001421, 0.000000000000000000 ) ) ;
#25328=VECTOR ( 'NONE', #29792, 1000.000000000000000 ) ;
#25329=CARTESIAN_POINT ( 'NONE',  ( -14.47279130897152299, 11.92499999726882187, 19.92008829642072243 ) ) ;
#25334=CARTESIAN_POINT ( 'NONE',  ( 33.58253175000000113, 16.12500000273120548, -4.112674001490185761E-15 ) ) ;
#25335=CARTESIAN_POINT ( 'NONE',  ( 14.47279130897151767, 11.42499999726880944, -19.92008829642072598 ) ) ;
#25338=ORIENTED_EDGE ( 'NONE', *, *, #27400, .F. ) ;
#25341=EDGE_LOOP ( 'NONE', ( #27662, #14457, #31546, #10875 ) ) ;
#25344=CARTESIAN_POINT ( 'NONE',  ( 14.47279130897151767, 1.424999997268804997, -19.92008829642072598 ) ) ;
#25345=CARTESIAN_POINT ( 'NONE',  ( -18.94512977948576093, 13.82499999726882756, 13.76444248337722698 ) ) ;
#25346=CARTESIAN_POINT ( 'NONE',  ( -33.58253175000000113, 21.37500000273118062, 0.000000000000000000 ) ) ;
#25347=CARTESIAN_POINT ( 'NONE',  ( -26.29305231718579350, 22.30000000546239391, -19.10302069950537884 ) ) ;
#25349=CARTESIAN_POINT ( 'NONE',  ( -26.29305231718579350, 65.79999999999999716, -19.10302069950537884 ) ) ;
#25353=CARTESIAN_POINT ( 'NONE',  ( -27.16883889988623935, 37.57500000273117280, 19.73931689729374739 ) ) ;
#25354=CARTESIAN_POINT ( 'NONE',  ( 10.04305231718578817, 43.90000000546237402, -30.90933677959249337 ) ) ;
#25358=CARTESIAN_POINT ( 'NONE',  ( -7.236395654485763274, 14.52499999726880553, 22.27133577429736633 ) ) ;
#25359=CARTESIAN_POINT ( 'NONE',  ( 26.29305231718578995, 11.19999999999998863, -19.10302069950538240 ) ) ;
#25362=CARTESIAN_POINT ( 'NONE',  ( -2.162160676586881955E-15, 54.62500000273116996, -35.31076352940723240 ) ) ;
#25364=CARTESIAN_POINT ( 'NONE',  ( -33.58253175000000113, 41.27500000273118275, -10.91162601494193041 ) ) ;
#25366=CARTESIAN_POINT ( 'NONE',  ( 3.880418787951178228, 10.44874571845314293, -24.49999999999998224 ) ) ;
#25370=CARTESIAN_POINT ( 'NONE',  ( -20.08610463437156923, 42.30000000000000426, 27.64615127144130113 ) ) ;
#25372=CARTESIAN_POINT ( 'NONE',  ( -4.405589869732278832E-13, 31.00000000546236834, 32.50000000000000000 ) ) ;
#25374=FACE_OUTER_BOUND ( 'NONE', #24256, .T. ) ;
#25378=CARTESIAN_POINT ( 'NONE',  ( 5.147494310547434893, 34.55125428154683220, 32.49999999999999289 ) ) ;
#25379=CIRCLE ( 'NONE', #13335, 24.50000000000000000 ) ;
#25380=CARTESIAN_POINT ( 'NONE',  ( 27.16883889988623935, 32.32500000273119412, -19.73931689729374384 ) ) ;
#25382=EDGE_CURVE ( 'NONE', #19851, #31882, #3859, .T. ) ;
#25383=ORIENTED_EDGE ( 'NONE', *, *, #22154, .T. ) ;
#25387=CARTESIAN_POINT ( 'NONE',  ( -26.29305231718579350, 16.30000000546239036, -19.10302069950537884 ) ) ;
#25394=CARTESIAN_POINT ( 'NONE',  ( -33.58253175000000113, 43.37500000273119838, 0.000000000000000000 ) ) ;
#25395=CARTESIAN_POINT ( 'NONE',  ( 10.04305231718579705, 45.10000000546238397, 30.90933677959248982 ) ) ;
#25397=CARTESIAN_POINT ( 'NONE',  ( 27.16883889988624290, 29.92500000273118488, 19.73931689729373673 ) ) ;
#25399=CARTESIAN_POINT ( 'NONE',  ( -27.16883889988623935, 55.57500000273118701, 19.73931689729374739 ) ) ;
#25401=CARTESIAN_POINT ( 'NONE',  ( 10.04305231718579705, 32.59999999999998721, 30.90933677959248982 ) ) ;
#25403=CARTESIAN_POINT ( 'NONE',  ( 33.58253175000000823, 76.02500000273118985, 10.91162601494192863 ) ) ;
#25406=CARTESIAN_POINT ( 'NONE',  ( 33.58253175000000113, 68.47500000273119269, -10.91162601494193574 ) ) ;
#25408=VECTOR ( 'NONE', #19221, 1000.000000000000114 ) ;
#25410=CARTESIAN_POINT ( 'NONE',  ( 10.37757302488624056, 20.52500000273119340, -31.93888565452638417 ) ) ;
#25411=CARTESIAN_POINT ( 'NONE',  ( 7.570916362186207671, 11.34999999453761887, 23.30088464923126779 ) ) ;
#25413=( BOUNDED_CURVE ( )  B_SPLINE_CURVE ( 2, ( #17964, #9881, #33909, #20878, #33384, #10235, #31497, #4728, #20716, #31326, #20539, #7301, #15731 ),
 .UNSPECIFIED., .F., .T. ) 
 B_SPLINE_CURVE_WITH_KNOTS ( ( 3, 2, 2, 2, 2, 2, 3 ),
 ( 0.1730769230769230727, 0.1743589743589743501, 0.1769230769230769329, 0.1794871794871794879, 0.1820512820512820429, 0.1846153846153846256, 0.1858974358974359031 ),
 .UNSPECIFIED. ) 
 CURVE ( )  GEOMETRIC_REPRESENTATION_ITEM ( )  RATIONAL_B_SPLINE_CURVE ( ( 0.9755282581475768211, 0.9755282581475768211, 1.000000000000000000, 0.9510565162951535312, 1.000000000000000000, 0.9510565162951535312, 1.000000000000000000, 0.9510565162951535312, 1.000000000000000000, 0.9510565162951535312, 1.000000000000000000, 0.9755282581475768211, 0.9755282581475768211 ) ) 
 REPRESENTATION_ITEM ( '' )  );
#25425=CARTESIAN_POINT ( 'NONE',  ( -5.147494310547430452, 53.55125428154684641, -32.49999999999999289 ) ) ;
#25426=CARTESIAN_POINT ( 'NONE',  ( -2.092463501923844636E-15, 78.00000000546238255, -34.17252228774368916 ) ) ;
#25431=CARTESIAN_POINT ( 'NONE',  ( -27.16883889988624290, 73.17500000273119554, -19.73931689729374028 ) ) ;
#25436=CARTESIAN_POINT ( 'NONE',  ( 32.50000000000000000, 63.60000000546238397, -10.55989012756945833 ) ) ;
#25437=ORIENTED_EDGE ( 'NONE', *, *, #21950, .F. ) ;
#25438=CARTESIAN_POINT ( 'NONE',  ( 10.04305231718578817, 27.40000000000000924, -30.90933677959249337 ) ) ;
#25439=CARTESIAN_POINT ( 'NONE',  ( 10.37757302488624767, 47.72500000273119269, 31.93888565452638417 ) ) ;
#25440=CARTESIAN_POINT ( 'NONE',  ( -4.523095164977116484E-15, 16.12499999726880873, 24.62258325217400312 ) ) ;
#25441=APPLICATION_CONTEXT ( 'automotive_design' ) ;
#25442=CARTESIAN_POINT ( 'NONE',  ( 26.29305231718579350, 7.300000005462381480, 19.10302069950537529 ) ) ;
#25443=CARTESIAN_POINT ( 'NONE',  ( -4.635254915624211769, 77.60000000000000853, -14.26584774442730286 ) ) ;
#25445=CARTESIAN_POINT ( 'NONE',  ( -26.29305231718578995, 50.19999999999999574, 19.10302069950538595 ) ) ;
#25447=CARTESIAN_POINT ( 'NONE',  ( 20.75514604977249178, 16.07500000273119412, 28.56700777964553950 ) ) ;
#25448=CARTESIAN_POINT ( 'NONE',  ( -20.08610463437156923, 74.30000000000001137, 27.64615127144130113 ) ) ;
#25450=CARTESIAN_POINT ( 'NONE',  ( 13.91746825000000065, 78.27500000273116143, 4.522059556121114987 ) ) ;
#25463=CARTESIAN_POINT ( 'NONE',  ( -10.37757302488623701, 5.775000002731179194, 31.93888565452638417 ) ) ;
#25467=CARTESIAN_POINT ( 'NONE',  ( 10.04305231718578817, 69.40000000000001990, -30.90933677959249337 ) ) ;
#25469=CARTESIAN_POINT ( 'NONE',  ( 20.75514604977249178, 47.82500000273117990, 28.56700777964553950 ) ) ;
#25474=CARTESIAN_POINT ( 'NONE',  ( 5.779280353836490358E-15, 5.000000005462372776, 32.49999999999999289 ) ) ;
#25475=CARTESIAN_POINT ( 'NONE',  ( 18.94512977948575738, 14.42499999726881654, 13.76444248337723408 ) ) ;
#25477=CARTESIAN_POINT ( 'NONE',  ( -27.16883889988623935, 77.57500000273121543, 19.73931689729374739 ) ) ;
#25478=VERTEX_POINT ( 'NONE', #11716 ) ;
#25480=CARTESIAN_POINT ( 'NONE',  ( -5.147494310547423346, 34.94874572391554324, 32.50000000000000000 ) ) ;
#25484=CARTESIAN_POINT ( 'NONE',  ( 27.16883889988624290, 65.92500000273118133, 19.73931689729373673 ) ) ;
#25486=CARTESIAN_POINT ( 'NONE',  ( -19.82091636218621034, 12.80000000000000604, -14.40073868116559552 ) ) ;
#25487=CARTESIAN_POINT ( 'NONE',  ( 7.236395654485755280, 4.724999997268803043, 22.27133577429736988 ) ) ;
#25488=CARTESIAN_POINT ( 'NONE',  ( -33.58253175000000113, 7.025000002731188964, -10.91162601494193218 ) ) ;
#25491=CARTESIAN_POINT ( 'NONE',  ( 12.13525491562421088, 72.79999999999999716, 8.816778784387095058 ) ) ;
#25495=CARTESIAN_POINT ( 'NONE',  ( 12.13525491562421088, 75.05000000546237970, 8.816778784387095058 ) ) ;
#25497=CARTESIAN_POINT ( 'NONE',  ( 10.37757302488624056, 30.52500000273117209, -31.93888565452638417 ) ) ;
#25500=CARTESIAN_POINT ( 'NONE',  ( -10.37757302488623701, 19.77500000273118985, 31.93888565452638417 ) ) ;
#25501=CARTESIAN_POINT ( 'NONE',  ( 32.50000000000000000, 41.00000000000000711, -3.980102097228898626E-15 ) ) ;
#25502=CARTESIAN_POINT ( 'NONE',  ( -19.82091636218621034, 14.54999999453762705, -14.40073868116559552 ) ) ;
#25506=CARTESIAN_POINT ( 'NONE',  ( -23.41746824999999887, 9.524999997268810858, -7.608796670333730638 ) ) ;
#25507=CARTESIAN_POINT ( 'NONE',  ( 10.37757302488624767, 65.72500000273117848, 31.93888565452638417 ) ) ;
#25510=CARTESIAN_POINT ( 'NONE',  ( -27.16883889988624290, 6.925000002731191096, -19.73931689729374028 ) ) ;
#25511=CARTESIAN_POINT ( 'NONE',  ( -14.47279130897151589, 9.824999997268802687, -19.92008829642072598 ) ) ;
#25513=EDGE_CURVE ( 'NONE', #11893, #19899, #7371, .T. ) ;
#25522=CARTESIAN_POINT ( 'NONE',  ( 23.41746825000000243, 5.224999997268802154, -7.608796670333727974 ) ) ;
#25524=EDGE_CURVE ( 'NONE', #21829, #25478, #20313, .T. ) ;
#25525=CARTESIAN_POINT ( 'NONE',  ( -7.236395654485763274, 14.02499999726880553, 22.27133577429736633 ) ) ;
#25526=CARTESIAN_POINT ( 'NONE',  ( -33.58253175000000113, 15.37500000273117706, 0.000000000000000000 ) ) ;
#25527=CARTESIAN_POINT ( 'NONE',  ( 10.04305231718579705, 27.10000000546236620, 30.90933677959248982 ) ) ;
#25528=CARTESIAN_POINT ( 'NONE',  ( -20.08610463437157989, 67.70000000000000284, -27.64615127144129758 ) ) ;
#25532=CARTESIAN_POINT ( 'NONE',  ( -33.58253175000000113, 29.37500000273118772, 0.000000000000000000 ) ) ;
#25533=FACE_OUTER_BOUND ( 'NONE', #7143, .T. ) ;
#25535=CARTESIAN_POINT ( 'NONE',  ( -19.82091636218621034, 0.7999999999999951594, -14.40073868116559552 ) ) ;
#25536=CARTESIAN_POINT ( 'NONE',  ( 10.04305231718579705, 6.599999999999994316, 30.90933677959248982 ) ) ;
#25537=FACE_OUTER_BOUND ( 'NONE', #9282, .T. ) ;
#25539=CARTESIAN_POINT ( 'NONE',  ( 20.75514604977248467, 54.42500000273117422, -28.56700777964554305 ) ) ;
#25542=CARTESIAN_POINT ( 'NONE',  ( 33.58253175000000823, 42.27500000273118275, 10.91162601494192685 ) ) ;
#25549=CARTESIAN_POINT ( 'NONE',  ( 4.300734207923757602, 80.77500000273118985, -13.23629886949340673 ) ) ;
#25551=CARTESIAN_POINT ( 'NONE',  ( 0.000000000000000000, 0.000000000000000000, 24.50000000000000000 ) ) ;
#25555=CARTESIAN_POINT ( 'NONE',  ( 27.16883889988624290, 33.92500000273118843, 19.73931689729373673 ) ) ;
#25557=VERTEX_POINT ( 'NONE', #739 ) ;
#25558=ORIENTED_EDGE ( 'NONE', *, *, #19308, .F. ) ;
#25561=CARTESIAN_POINT ( 'NONE',  ( -1.778240108872766143E-15, 5.500000000000003553, -32.49999999999999289 ) ) ;
#25562=ORIENTED_EDGE ( 'NONE', *, *, #10218, .F. ) ;
#25568=CARTESIAN_POINT ( 'NONE',  ( 33.58253175000000113, 44.37500000273119838, -4.112674001490185761E-15 ) ) ;
#25569=CARTESIAN_POINT ( 'NONE',  ( 20.08610463437158344, 41.20000000546236407, 27.64615127144129403 ) ) ;
#25571=CARTESIAN_POINT ( 'NONE',  ( -2.162160676586881955E-15, 24.62500000273118772, -35.31076352940723240 ) ) ;
#25573=CARTESIAN_POINT ( 'NONE',  ( 33.58253175000000823, 46.27500000273120406, 10.91162601494192863 ) ) ;
#25575=CARTESIAN_POINT ( 'NONE',  ( -10.04305231718579172, 27.60000000000001208, -30.90933677959248982 ) ) ;
#25578=CARTESIAN_POINT ( 'NONE',  ( -33.58253175000000113, 79.12500000273119838, 0.000000000000000000 ) ) ;
#25580=CARTESIAN_POINT ( 'NONE',  ( 6.486482029760648627E-15, 59.87500000273118417, 35.31076352940722529 ) ) ;
#25583=CARTESIAN_POINT ( 'NONE',  ( 27.16883889988623935, 20.32500000273118701, -19.73931689729374384 ) ) ;
#25584=CARTESIAN_POINT ( 'NONE',  ( -24.50000000000000355, 8.649999994537630243, -7.960532557706207157 ) ) ;
#25586=CARTESIAN_POINT ( 'NONE',  ( 19.82091636218621389, 7.949999994537631842, -14.40073868116559197 ) ) ;
#25596=CARTESIAN_POINT ( 'NONE',  ( 5.779280353836490358E-15, 62.50000000000000000, 32.49999999999999289 ) ) ;
#25598=CARTESIAN_POINT ( 'NONE',  ( -1.778240108872766143E-15, 58.00000000546237544, -32.49999999999999289 ) ) ;
#25600=CARTESIAN_POINT ( 'NONE',  ( 26.29305231718578995, 73.70000000546239960, -19.10302069950538240 ) ) ;
#25604=ORIENTED_EDGE ( 'NONE', *, *, #29081, .F. ) ;
#25605=CARTESIAN_POINT ( 'NONE',  ( -33.58253175000000113, 75.47500000273116427, 10.91162601494193929 ) ) ;
#25608=CARTESIAN_POINT ( 'NONE',  ( 10.04305231718579705, 63.10000000546239818, 30.90933677959248982 ) ) ;
#25609=ORIENTED_EDGE ( 'NONE', *, *, #24339, .F. ) ;
#25611=CARTESIAN_POINT ( 'NONE',  ( -33.58253175000000113, 43.02500000273118275, -10.91162601494193218 ) ) ;
#25612=CARTESIAN_POINT ( 'NONE',  ( 23.41746824999999887, 18.62499999726882649, 0.000000000000000000 ) ) ;
#25613=CARTESIAN_POINT ( 'NONE',  ( -32.50000000000000000, 6.400000005462388231, -10.55989012756945478 ) ) ;
#25616=CARTESIAN_POINT ( 'NONE',  ( 32.50000000000000000, 46.99999999999998579, -3.980102097228898626E-15 ) ) ;
#25619=CARTESIAN_POINT ( 'NONE',  ( -20.75514604977248823, 15.07500000273116747, -28.56700777964554305 ) ) ;
#25620=CYLINDRICAL_SURFACE ( 'NONE', #14560, 24.50000000000000000 ) ;
#25622=CARTESIAN_POINT ( 'NONE',  ( 4.300734207923757602, 76.77500000273118985, -13.23629886949340673 ) ) ;
#25623=CARTESIAN_POINT ( 'NONE',  ( -4.223320258572819786E-15, 3.500000000000004441, 24.50000000000000000 ) ) ;
#25624=CARTESIAN_POINT ( 'NONE',  ( 32.50000000000000000, 53.60000000546238397, -10.55989012756945833 ) ) ;
#25638=CARTESIAN_POINT ( 'NONE',  ( -13.91746824999999532, 71.47500000273120691, 4.522059556121122093 ) ) ;
#25640=CARTESIAN_POINT ( 'NONE',  ( -27.16883889988623935, 47.32500000273117990, 19.73931689729374739 ) ) ;
#25642=CARTESIAN_POINT ( 'NONE',  ( 12.13525491562421088, 78.80000000000001137, 8.816778784387095058 ) ) ;
#25643=VERTEX_POINT ( 'NONE', #4337 ) ;
#25647=CARTESIAN_POINT ( 'NONE',  ( 27.16883889988624290, 78.17500000273119554, 19.73931689729373673 ) ) ;
#25652=DIRECTION ( 'NONE',  ( -0.000000000000000000, -1.000000000000000000, -0.000000000000000000 ) ) ;
#25653=CARTESIAN_POINT ( 'NONE',  ( 33.58253175000000113, 68.22500000273116427, -10.91162601494193751 ) ) ;
#25655=CARTESIAN_POINT ( 'NONE',  ( -4.732186688966233175E-15, 9.499999999999991118, 25.76082449383753925 ) ) ;
#25656=CARTESIAN_POINT ( 'NONE',  ( 7.236395654485760609, 3.524999997268824181, -22.27133577429736633 ) ) ;
#25657=CARTESIAN_POINT ( 'NONE',  ( -20.75514604977248112, 9.425000002731202642, 28.56700777964554661 ) ) ;
#25658=CARTESIAN_POINT ( 'NONE',  ( -19.82091636218621389, 6.949999994537630954, 14.40073868116558842 ) ) ;
#25660=CARTESIAN_POINT ( 'NONE',  ( -15.00000000000000000, 73.90000000000003411, -4.873795443493594171 ) ) ;
#25665=CARTESIAN_POINT ( 'NONE',  ( 15.00000000000000000, 73.25000000546239676, -1.836970198721029589E-15 ) ) ;
#25667=CARTESIAN_POINT ( 'NONE',  ( -20.75514604977248823, 30.82500000273119767, -28.56700777964554305 ) ) ;
#25670=CARTESIAN_POINT ( 'NONE',  ( -20.75514604977248112, 21.67500000273119198, 28.56700777964554661 ) ) ;
#25671=CARTESIAN_POINT ( 'NONE',  ( -26.29305231718578995, 68.19999999999998863, 19.10302069950538595 ) ) ;
#25672=CARTESIAN_POINT ( 'NONE',  ( -10.37757302488623701, 73.52500000273121827, 31.93888565452638417 ) ) ;
#25675=CARTESIAN_POINT ( 'NONE',  ( -33.58253175000000113, 67.12500000273119838, 0.000000000000000000 ) ) ;
#25677=EDGE_CURVE ( 'NONE', #2966, #16286, #11975, .T. ) ;
#25679=CARTESIAN_POINT ( 'NONE',  ( 6.486482029760648627E-15, 9.625000002731196602, 35.31076352940722529 ) ) ;
#25680=CARTESIAN_POINT ( 'NONE',  ( 1.507698388325705758E-15, 11.62499999726880340, -24.62258325217400312 ) ) ;
#25682=ORIENTED_EDGE ( 'NONE', *, *, #2853, .T. ) ;
#25684=ORIENTED_EDGE ( 'NONE', *, *, #21442, .F. ) ;
#25688=CARTESIAN_POINT ( 'NONE',  ( 5.334720326618300005E-14, 72.00000000546238255, -32.50000000000000000 ) ) ;
#25689=CARTESIAN_POINT ( 'NONE',  ( 7.236395654485760609, 5.524999997268825958, -22.27133577429736633 ) ) ;
#25690=CARTESIAN_POINT ( 'NONE',  ( 23.41746825000000243, 14.72499999726881903, -7.608796670333727974 ) ) ;
#25691=CARTESIAN_POINT ( 'NONE',  ( -33.58253175000000113, 17.27500000273118630, -10.91162601494193218 ) ) ;
#25692=CARTESIAN_POINT ( 'NONE',  ( 26.29305231718578995, 17.70000000546237473, -19.10302069950538240 ) ) ;
#25693=CARTESIAN_POINT ( 'NONE',  ( 32.50000000000000000, 63.10000000000001563, -10.55989012756945833 ) ) ;
#25694=CARTESIAN_POINT ( 'NONE',  ( 15.00000000000000355, 77.15000000546240244, 4.873795443493592394 ) ) ;
#25695=CARTESIAN_POINT ( 'NONE',  ( 26.29305231718578995, 73.70000000546239960, -19.10302069950538240 ) ) ;
#25697=CARTESIAN_POINT ( 'NONE',  ( -2.162160676586881955E-15, 30.87500000273119483, -35.31076352940723240 ) ) ;
#25698=CARTESIAN_POINT ( 'NONE',  ( -10.04305231718578462, 32.90000000546239534, 30.90933677959249337 ) ) ;
#25701=CARTESIAN_POINT ( 'NONE',  ( 1.507698388325705758E-15, 13.62499999726882827, -24.62258325217400312 ) ) ;
#25702=CARTESIAN_POINT ( 'NONE',  ( -26.29305231718578995, 8.199999999999985079, 19.10302069950538595 ) ) ;
#25705=CARTESIAN_POINT ( 'NONE',  ( 27.16883889988623935, 50.32500000273118701, -19.73931689729374384 ) ) ;
#25707=CARTESIAN_POINT ( 'NONE',  ( 33.58253175000000113, 42.47500000273119980, -10.91162601494193574 ) ) ;
#25708=CARTESIAN_POINT ( 'NONE',  ( -1.778240108872766143E-15, 13.50000000000000355, -32.49999999999999289 ) ) ;
#25711=CARTESIAN_POINT ( 'NONE',  ( 5.779280353836490358E-15, 62.50000000000000000, 32.49999999999999289 ) ) ;
#25714=CARTESIAN_POINT ( 'NONE',  ( 5.779280353836490358E-15, 6.500000000000002665, 32.49999999999999289 ) ) ;
#25717=FACE_OUTER_BOUND ( 'NONE', #29968, .T. ) ;
#25720=CARTESIAN_POINT ( 'NONE',  ( 20.08610463437157279, 11.29999999999999361, -27.64615127144129758 ) ) ;
#25721=CARTESIAN_POINT ( 'NONE',  ( -33.58253175000000113, 27.02500000273119340, -10.91162601494193041 ) ) ;
#25723=EDGE_CURVE ( 'NONE', #33045, #1732, #27317, .T. ) ;
#25734=CARTESIAN_POINT ( 'NONE',  ( 20.75514604977249178, 36.07500000273117990, 28.56700777964553950 ) ) ;
#25735=CARTESIAN_POINT ( 'NONE',  ( 6.277390505771533514E-15, 45.00000000546235412, 34.17252228774368916 ) ) ;
#25737=CARTESIAN_POINT ( 'NONE',  ( -27.16883889988623935, 23.32500000273118701, 19.73931689729374739 ) ) ;
#25738=CARTESIAN_POINT ( 'NONE',  ( 7.570916362186213000, 14.14999999453761603, -23.30088464923126423 ) ) ;
#25739=CARTESIAN_POINT ( 'NONE',  ( -20.75514604977248823, 51.07500000273116569, -28.56700777964554305 ) ) ;
#25741=CARTESIAN_POINT ( 'NONE',  ( 6.277390505771533514E-15, 28.50000000000000000, 34.17252228774368916 ) ) ;
#25743=CARTESIAN_POINT ( 'NONE',  ( -33.58253175000000113, 69.22500000273117848, 10.91162601494193929 ) ) ;
#25746=CARTESIAN_POINT ( 'NONE',  ( -10.37757302488624411, 60.97500000273120691, -31.93888565452638417 ) ) ;
#25748=CARTESIAN_POINT ( 'NONE',  ( -32.50000000000000000, 40.40000000546239534, -10.55989012756945300 ) ) ;
#25749=CARTESIAN_POINT ( 'NONE',  ( -27.16883889988624290, 16.92500000273117067, -19.73931689729374028 ) ) ;
#25750=CARTESIAN_POINT ( 'NONE',  ( 15.14183272437242245, 10.04999999453761639, -20.84094480462497856 ) ) ;
#25761=CARTESIAN_POINT ( 'NONE',  ( -3.880418787951138260, 3.198745712990784806, 24.50000000000000000 ) ) ;
#25763=CARTESIAN_POINT ( 'NONE',  ( 5.147494310547380714, 63.05125428700923607, 32.50000000000002132 ) ) ;
#25764=CARTESIAN_POINT ( 'NONE',  ( -10.04305231718578462, 74.90000000546237402, 30.90933677959249337 ) ) ;
#25769=CARTESIAN_POINT ( 'NONE',  ( 33.58253175000000113, 76.37500000273116996, -4.112674001490185761E-15 ) ) ;
#25773=CARTESIAN_POINT ( 'NONE',  ( 27.16883889988624290, 54.17500000273117422, 19.73931689729373673 ) ) ;
#25774=CARTESIAN_POINT ( 'NONE',  ( -20.08610463437157989, 62.20000000546237828, -27.64615127144129758 ) ) ;
#25776=CARTESIAN_POINT ( 'NONE',  ( -10.04305231718579172, 10.10000000546237864, -30.90933677959248982 ) ) ;
#25777=CARTESIAN_POINT ( 'NONE',  ( 33.58253175000000113, 44.12500000273117706, -4.112674001490185761E-15 ) ) ;
#25778=CARTESIAN_POINT ( 'NONE',  ( 20.75514604977248467, 66.67500000273119554, -28.56700777964554305 ) ) ;
#25779=CARTESIAN_POINT ( 'NONE',  ( 26.29305231718578995, 5.700000005462390718, -19.10302069950538240 ) ) ;
#25781=DIRECTION ( 'NONE',  ( 0.000000000000000000, 0.000000000000000000, -1.000000000000000000 ) ) ;
#25782=CARTESIAN_POINT ( 'NONE',  ( -32.50000000000000000, 48.09999999999999432, 10.55989012756946366 ) ) ;
#25783=CARTESIAN_POINT ( 'NONE',  ( 20.75514604977248467, 12.67500000273118488, -28.56700777964554305 ) ) ;
#25784=LINE ( 'NONE', #33679, #6881 ) ;
#25786=CARTESIAN_POINT ( 'NONE',  ( 11.25946833292375793, 80.57500000273121543, -8.180482586598735395 ) ) ;
#25787=CARTESIAN_POINT ( 'NONE',  ( 33.58253175000000113, 78.47500000273116427, -10.91162601494193574 ) ) ;
#25788=CARTESIAN_POINT ( 'NONE',  ( -10.04305231718578462, 22.40000000000000213, 30.90933677959249337 ) ) ;
#25801=CARTESIAN_POINT ( 'NONE',  ( -11.25946833292375793, 73.57500000273120122, 8.180482586598737171 ) ) ;
#25803=CARTESIAN_POINT ( 'NONE',  ( 27.16883889988624290, 45.92500000273119554, 19.73931689729373673 ) ) ;
#25807=EDGE_CURVE ( 'NONE', #30562, #17974, #5173, .T. ) ;
#25811=CARTESIAN_POINT ( 'NONE',  ( -33.58253175000000113, 75.27500000273118985, -10.91162601494193218 ) ) ;
#25812=ADVANCED_FACE ( 'NONE', ( #28527 ), #20664, .F. ) ;
#25813=EDGE_LOOP ( 'NONE', ( #5732, #24005, #33685, #10792 ) ) ;
#25817=( BOUNDED_CURVE ( )  B_SPLINE_CURVE ( 2, ( #15258, #32907, #30682, #25720, #2200, #32745, #10789, #10618, #18014, #13023, #28800, #26235, #20924 ),
 .UNSPECIFIED., .F., .T. ) 
 B_SPLINE_CURVE_WITH_KNOTS ( ( 3, 2, 2, 2, 2, 2, 3 ),
 ( 0.8782051282051281937, 0.8794871794871794712, 0.8820512820512820262, 0.8846153846153845812, 0.8871794871794871362, 0.8897435897435896912, 0.8910256410256410797 ),
 .UNSPECIFIED. ) 
 CURVE ( )  GEOMETRIC_REPRESENTATION_ITEM ( )  RATIONAL_B_SPLINE_CURVE ( ( 0.9755282581475768211, 0.9755282581475768211, 1.000000000000000000, 0.9510565162951535312, 1.000000000000000000, 0.9510565162951535312, 1.000000000000000000, 0.9510565162951535312, 1.000000000000000000, 0.9510565162951535312, 1.000000000000000000, 0.9755282581475757109, 0.9755282581475768211 ) ) 
 REPRESENTATION_ITEM ( '' )  );
#25818=CARTESIAN_POINT ( 'NONE',  ( 33.58253175000000113, 62.22500000273119269, -10.91162601494193751 ) ) ;
#25820=CARTESIAN_POINT ( 'NONE',  ( -19.82091636218621034, 16.80000000000000782, -14.40073868116559552 ) ) ;
#25821=DIRECTION ( 'NONE',  ( -0.000000000000000000, -1.000000000000000000, -0.000000000000000000 ) ) ;
#25823=CARTESIAN_POINT ( 'NONE',  ( 33.58253175000000113, 8.125000002731198379, -4.112674001490185761E-15 ) ) ;
#25825=CARTESIAN_POINT ( 'NONE',  ( -15.00000000000000000, 76.10000000000002274, 4.873795443493597723 ) ) ;
#25830=CARTESIAN_POINT ( 'NONE',  ( 12.13525491562421088, 73.05000000546237970, 8.816778784387095058 ) ) ;
#25832=CARTESIAN_POINT ( 'NONE',  ( 27.16883889988624290, 31.92500000273118488, 19.73931689729373673 ) ) ;
#25835=VECTOR ( 'NONE', #14889, 1000.000000000000114 ) ;
#25837=CARTESIAN_POINT ( 'NONE',  ( -33.58253175000000113, 21.27500000273117564, -10.91162601494193041 ) ) ;
#25838=CARTESIAN_POINT ( 'NONE',  ( -20.08610463437157989, 67.70000000000000284, -27.64615127144129758 ) ) ;
#25839=CARTESIAN_POINT ( 'NONE',  ( 6.486482029760648627E-15, 77.62500000273119838, 35.31076352940722529 ) ) ;
#25840=CARTESIAN_POINT ( 'NONE',  ( 5.147494310547481966, 59.94874572391551482, -32.49999999999998579 ) ) ;
#25842=CARTESIAN_POINT ( 'NONE',  ( -23.41746824999999887, 17.62499999726882649, -2.867812753649727150E-15 ) ) ;
#25843=CARTESIAN_POINT ( 'NONE',  ( 33.58253175000000823, 62.02500000273116854, 10.91162601494192685 ) ) ;
#25846=CARTESIAN_POINT ( 'NONE',  ( 10.37757302488624767, 5.725000002731183812, 31.93888565452638417 ) ) ;
#25847=CARTESIAN_POINT ( 'NONE',  ( -23.41746824999999887, 18.12499999726882649, -2.867812753649727150E-15 ) ) ;
#25856=LINE ( 'NONE', #23804, #30428 ) ;
#25857=CARTESIAN_POINT ( 'NONE',  ( -18.94512977948575738, 3.924999997268807661, -13.76444248337723231 ) ) ;
#25858=CARTESIAN_POINT ( 'NONE',  ( 14.47279130897151767, 14.92499999726881299, -19.92008829642072598 ) ) ;
#25859=CARTESIAN_POINT ( 'NONE',  ( -10.37757302488623701, 17.77500000273118985, 31.93888565452638417 ) ) ;
#25860=CARTESIAN_POINT ( 'NONE',  ( -32.50000000000000000, 18.50000000546236834, 0.000000000000000000 ) ) ;
#25861=CARTESIAN_POINT ( 'NONE',  ( -32.50000000000000000, 68.00000000000000000, 0.000000000000000000 ) ) ;
#25863=DIRECTION ( 'NONE',  ( -0.000000000000000000, 1.000000000000000000, -0.000000000000000000 ) ) ;
#25865=DIRECTION ( 'NONE',  ( 0.000000000000000000, 0.000000000000000000, -1.000000000000000000 ) ) ;
#25868=DIRECTION ( 'NONE',  ( -0.000000000000000000, -1.000000000000000000, -0.000000000000000000 ) ) ;
#25869=CARTESIAN_POINT ( 'NONE',  ( 18.94512977948576093, 17.32499999726880446, -13.76444248337722875 ) ) ;
#25870=CARTESIAN_POINT ( 'NONE',  ( 32.50000000000000711, 10.90000000000000568, 10.55989012756945122 ) ) ;
#25872=CARTESIAN_POINT ( 'NONE',  ( -33.58253175000000113, 53.22500000273118559, 10.91162601494193929 ) ) ;
#25874=CARTESIAN_POINT ( 'NONE',  ( -10.37757302488624411, 38.97500000273118559, -31.93888565452638417 ) ) ;
#25875=CARTESIAN_POINT ( 'NONE',  ( -1.778240108872766143E-15, 25.50000000000000711, -32.49999999999999289 ) ) ;
#25877=CARTESIAN_POINT ( 'NONE',  ( 20.08610463437158344, 51.20000000546237118, 27.64615127144129403 ) ) ;
#25881=CARTESIAN_POINT ( 'NONE',  ( 0.000000000000000000, 82.00000000000001421, -15.00000000000000000 ) ) ;
#25882=CARTESIAN_POINT ( 'NONE',  ( 7.313012447739250820E-14, 11.49999999999999112, 24.50000000000000000 ) ) ;
#25885=CARTESIAN_POINT ( 'NONE',  ( 0.000000000000000000, 80.00000000000001421, 0.000000000000000000 ) ) ;
#25886=CARTESIAN_POINT ( 'NONE',  ( 10.37757302488624767, 27.72500000273120335, 31.93888565452638417 ) ) ;
#25888=VERTEX_POINT ( 'NONE', #31607 ) ;
#25898=AXIS2_PLACEMENT_3D ( 'NONE', #13762, #11189, #3459 ) ;
#25900=DIRECTION ( 'NONE',  ( -0.000000000000000000, -1.000000000000000000, -0.000000000000000000 ) ) ;
#25901=CARTESIAN_POINT ( 'NONE',  ( 27.16883889988623935, 34.57500000273120122, -19.73931689729374384 ) ) ;
#25902=CARTESIAN_POINT ( 'NONE',  ( 10.04305231718578817, 37.90000000546236691, -30.90933677959249337 ) ) ;
#25905=CARTESIAN_POINT ( 'NONE',  ( -33.58253175000000113, 21.22500000273117848, 10.91162601494193929 ) ) ;
#25906=CARTESIAN_POINT ( 'NONE',  ( -4.405589869732278832E-13, 31.00000000546236834, 32.50000000000000000 ) ) ;
#25907=CARTESIAN_POINT ( 'NONE',  ( 33.58253175000000113, 48.47500000273118559, -10.91162601494193751 ) ) ;
#25910=CARTESIAN_POINT ( 'NONE',  ( 20.08610463437157279, 27.29999999999997939, -27.64615127144129758 ) ) ;
#25913=CARTESIAN_POINT ( 'NONE',  ( -20.75514604977248823, 68.82500000273118701, -28.56700777964554305 ) ) ;
#25914=CARTESIAN_POINT ( 'NONE',  ( -26.29305231718579350, 77.80000000000001137, -19.10302069950537884 ) ) ;
#25915=CARTESIAN_POINT ( 'NONE',  ( -20.08610463437157989, 20.20000000546238539, -27.64615127144129758 ) ) ;
#25916=CARTESIAN_POINT ( 'NONE',  ( 10.37757302488624767, 57.97500000273119980, 31.93888565452638417 ) ) ;
#25918=CARTESIAN_POINT ( 'NONE',  ( 27.16883889988623935, 10.32500000273117635, -19.73931689729374384 ) ) ;
#25923=CARTESIAN_POINT ( 'NONE',  ( 0.000000000000000000, 80.00000000000001421, -32.50000000000000000 ) ) ;
#25929=CARTESIAN_POINT ( 'NONE',  ( 1.836970198721029589E-15, 82.00000000000001421, 15.00000000000000000 ) ) ;
#25931=CARTESIAN_POINT ( 'NONE',  ( -20.08610463437157989, 53.69999999999998863, -27.64615127144129758 ) ) ;
#25932=CARTESIAN_POINT ( 'NONE',  ( -32.50000000000000000, 78.40000000546233139, -10.55989012756945478 ) ) ;
#25937=ORIENTED_EDGE ( 'NONE', *, *, #31468, .T. ) ;
#25938=CARTESIAN_POINT ( 'NONE',  ( -27.16883889988624290, 75.17500000273119554, -19.73931689729374028 ) ) ;
#25942=CARTESIAN_POINT ( 'NONE',  ( -10.37757302488623701, 55.77500000273119696, 31.93888565452638417 ) ) ;
#25943=CARTESIAN_POINT ( 'NONE',  ( -26.29305231718578995, 56.70000000546237828, 19.10302069950538595 ) ) ;
#25945=CARTESIAN_POINT ( 'NONE',  ( 10.37757302488624056, 40.52500000273118275, -31.93888565452638417 ) ) ;
#25946=FACE_OUTER_BOUND ( 'NONE', #31874, .T. ) ;
#25947=CARTESIAN_POINT ( 'NONE',  ( 27.16883889988623935, 68.57500000273120122, -19.73931689729374384 ) ) ;
#25948=CARTESIAN_POINT ( 'NONE',  ( 32.50000000000000000, 3.500000005462383434, -3.980102097228898626E-15 ) ) ;
#25949=AXIS2_PLACEMENT_3D ( 'NONE', #22930, #7651, #2508 ) ;
#25951=ADVANCED_FACE ( 'NONE', ( #31773, #28700 ), #28868, .T. ) ;
#25952=CARTESIAN_POINT ( 'NONE',  ( 0.000000000000000000, 80.00000000000001421, 0.000000000000000000 ) ) ;
#25953=CARTESIAN_POINT ( 'NONE',  ( -32.50000000000000000, 47.89999999999999858, -10.55989012756945478 ) ) ;
#25955=CARTESIAN_POINT ( 'NONE',  ( -33.58253175000000113, 13.47500000273118914, 10.91162601494193929 ) ) ;
#25957=CARTESIAN_POINT ( 'NONE',  ( -8.601468415847515203, 77.67500000273119554, 11.83890561707634959 ) ) ;
#25958=CARTESIAN_POINT ( 'NONE',  ( 33.58253175000000113, 76.47500000273117848, -10.91162601494193574 ) ) ;
#25975=CARTESIAN_POINT ( 'NONE',  ( 27.16883889988624290, 43.92500000273119554, 19.73931689729373673 ) ) ;
#25979=EDGE_LOOP ( 'NONE', ( #9204, #21680, #10211, #9660, #25684, #29012, #29135, #18317, #15617, #31130, #2472, #21641, #14287, #17897 ) ) ;
#25983=CARTESIAN_POINT ( 'NONE',  ( -10.37757302488623701, 73.77500000273118985, 31.93888565452638417 ) ) ;
#25987=VERTEX_POINT ( 'NONE', #23564 ) ;
#25988=CARTESIAN_POINT ( 'NONE',  ( -32.50000000000000000, 14.50000000546236478, 0.000000000000000000 ) ) ;
#25989=CARTESIAN_POINT ( 'NONE',  ( -33.58253175000000113, 59.02500000273120406, -10.91162601494193218 ) ) ;
#25992=CARTESIAN_POINT ( 'NONE',  ( -18.94512977948576093, 2.324999997268817342, 13.76444248337722698 ) ) ;
#25993=CARTESIAN_POINT ( 'NONE',  ( -10.37757302488624411, 6.725000002731185589, -31.93888565452638417 ) ) ;
#25997=CYLINDRICAL_SURFACE ( 'NONE', #19894, 32.50000000000000000 ) ;
#26002=CARTESIAN_POINT ( 'NONE',  ( -4.635254915624208216, 72.65000000546240244, 14.26584774442730463 ) ) ;
#26004=ADVANCED_FACE ( 'NONE', ( #33856 ), #7767, .T. ) ;
#26005=CARTESIAN_POINT ( 'NONE',  ( -27.16883889988623935, 33.32500000273120122, 19.73931689729374739 ) ) ;
#26008=CARTESIAN_POINT ( 'NONE',  ( 33.58253175000000823, 20.27500000273117564, 10.91162601494192685 ) ) ;
#26010=ADVANCED_FACE ( 'NONE', ( #15505 ), #5365, .T. ) ;
#26012=CARTESIAN_POINT ( 'NONE',  ( 33.58253175000000823, 76.02500000273118985, 10.91162601494192685 ) ) ;
#26015=CARTESIAN_POINT ( 'NONE',  ( -4.523095164977117273E-15, 18.12499999726880162, 24.62258325217400312 ) ) ;
#26016=CARTESIAN_POINT ( 'NONE',  ( 33.58253175000000113, 66.22500000273120691, -10.91162601494193574 ) ) ;
#26017=( BOUNDED_CURVE ( )  B_SPLINE_CURVE ( 2, ( #3357, #929, #24296, #29090, #11249, #8664, #3520, #18983, #26698, #24128, #5594, #3195, #23962 ),
 .UNSPECIFIED., .F., .F. ) 
 B_SPLINE_CURVE_WITH_KNOTS ( ( 3, 2, 2, 2, 2, 2, 3 ),
 ( 0.8141025641025640969, 0.8153846153846153744, 0.8179487179487179294, 0.8205128205128204844, 0.8230769230769230393, 0.8256410256410255943, 0.8269230769230769829 ),
 .UNSPECIFIED. ) 
 CURVE ( )  GEOMETRIC_REPRESENTATION_ITEM ( )  RATIONAL_B_SPLINE_CURVE ( ( 0.9755282581475768211, 0.9755282581475768211, 1.000000000000000000, 0.9510565162951535312, 1.000000000000000000, 0.9510565162951535312, 1.000000000000000000, 0.9510565162951535312, 1.000000000000000000, 0.9510565162951535312, 1.000000000000000000, 0.9755282581475757109, 0.9755282581475768211 ) ) 
 REPRESENTATION_ITEM ( '' )  );
#26022=CARTESIAN_POINT ( 'NONE',  ( 10.37757302488624056, 8.525000002731180970, -31.93888565452638417 ) ) ;
#26023=CARTESIAN_POINT ( 'NONE',  ( 7.236395654485760609, 3.024999997268823293, -22.27133577429736633 ) ) ;
#26025=ORIENTED_EDGE ( 'NONE', *, *, #13776, .T. ) ;
#26031=CARTESIAN_POINT ( 'NONE',  ( -14.47279130897151589, 5.824999997268811569, -19.92008829642072598 ) ) ;
#26032=CARTESIAN_POINT ( 'NONE',  ( 1.577395562988744260E-15, 0.5000000000000133227, -25.76082449383753925 ) ) ;
#26033=CARTESIAN_POINT ( 'NONE',  ( -33.58253175000000113, 17.37500000273117706, 0.000000000000000000 ) ) ;
#26034=CARTESIAN_POINT ( 'NONE',  ( -10.04305231718579172, 63.59999999999998721, -30.90933677959248982 ) ) ;
#26036=CARTESIAN_POINT ( 'NONE',  ( -20.08610463437157989, 29.69999999999999218, -27.64615127144129758 ) ) ;
#26038=CARTESIAN_POINT ( 'NONE',  ( 11.25946833292375793, 74.17500000273119554, 8.180482586598731842 ) ) ;
#26041=CARTESIAN_POINT ( 'NONE',  ( 8.891200544363830713E-16, 81.50000000000001421, -15.00000000000000000 ) ) ;
#26042=CARTESIAN_POINT ( 'NONE',  ( 23.41746824999999887, 19.12499999726882649, 0.000000000000000000 ) ) ;
#26043=CARTESIAN_POINT ( 'NONE',  ( 26.29305231718579350, 8.800000000000002487, 19.10302069950537529 ) ) ;
#26048=CARTESIAN_POINT ( 'NONE',  ( 10.37757302488624767, 49.72500000273119269, 31.93888565452638417 ) ) ;
#26050=CARTESIAN_POINT ( 'NONE',  ( 20.75514604977248467, 42.67500000273119554, -28.56700777964554305 ) ) ;
#26052=EDGE_CURVE ( 'NONE', #15393, #31882, #7936, .T. ) ;
#26053=DIRECTION ( 'NONE',  ( 0.000000000000000000, 0.000000000000000000, -1.000000000000000000 ) ) ;
#26056=CARTESIAN_POINT ( 'NONE',  ( 5.779280353836490358E-15, 28.50000000000000355, 32.49999999999999289 ) ) ;
#26059=DIRECTION ( 'NONE',  ( -0.000000000000000000, -1.000000000000000000, -0.000000000000000000 ) ) ;
#26060=DIRECTION ( 'NONE',  ( 0.000000000000000000, 0.000000000000000000, -1.000000000000000000 ) ) ;
#26063=CARTESIAN_POINT ( 'NONE',  ( 15.14183272437242422, 18.04999999453762172, -20.84094480462497856 ) ) ;
#26064=CARTESIAN_POINT ( 'NONE',  ( 27.16883889988623935, 26.32500000273119056, -19.73931689729374384 ) ) ;
#26074=CARTESIAN_POINT ( 'NONE',  ( -27.16883889988624290, 37.17500000273118843, -19.73931689729374028 ) ) ;
#26075=CARTESIAN_POINT ( 'NONE',  ( -20.08610463437156923, 36.80000000546239391, 27.64615127144130113 ) ) ;
#26079=CARTESIAN_POINT ( 'NONE',  ( -20.75514604977248112, 25.42500000273119198, 28.56700777964554661 ) ) ;
#26080=CARTESIAN_POINT ( 'NONE',  ( 24.50000000000000000, 5.649999994537638237, 7.960532557706212486 ) ) ;
#26081=CARTESIAN_POINT ( 'NONE',  ( 33.58253175000000113, 52.37500000273121259, -4.112674001490185761E-15 ) ) ;
#26084=CARTESIAN_POINT ( 'NONE',  ( 20.08610463437157279, 25.29999999999998650, -27.64615127144129758 ) ) ;
#26086=CARTESIAN_POINT ( 'NONE',  ( -10.37757302488624411, 68.72500000273117848, -31.93888565452638417 ) ) ;
#26088=CARTESIAN_POINT ( 'NONE',  ( -20.75514604977248823, 63.07500000273119412, -28.56700777964554305 ) ) ;
#26089=DIRECTION ( 'NONE',  ( 0.000000000000000000, 0.000000000000000000, -1.000000000000000000 ) ) ;
#26090=CARTESIAN_POINT ( 'NONE',  ( 20.75514604977248467, 14.42500000273119021, -28.56700777964554305 ) ) ;
#26093=CARTESIAN_POINT ( 'NONE',  ( -27.16883889988623935, 1.575000002731197224, 19.73931689729374739 ) ) ;
#26096=CARTESIAN_POINT ( 'NONE',  ( 0.000000000000000000, 80.00000000000001421, 0.000000000000000000 ) ) ;
#26103=CARTESIAN_POINT ( 'NONE',  ( -10.04305231718579172, 53.60000000000000853, -30.90933677959248982 ) ) ;
#26104=CARTESIAN_POINT ( 'NONE',  ( -32.50000000000000000, 70.60000000546234844, 10.55989012756946366 ) ) ;
#26113=CARTESIAN_POINT ( 'NONE',  ( -27.16883889988624290, 55.17500000273118133, -19.73931689729374028 ) ) ;
#26114=CARTESIAN_POINT ( 'NONE',  ( 10.04305231718579705, 57.10000000546239107, 30.90933677959248982 ) ) ;
#26115=( BOUNDED_CURVE ( )  B_SPLINE_CURVE ( 2, ( #28443, #2709, #4934, #31015, #18166, #17998, #26217, #13170, #15416, #33939, #21249, #2361, #20906 ),
 .UNSPECIFIED., .F., .F. ) 
 B_SPLINE_CURVE_WITH_KNOTS ( ( 3, 2, 2, 2, 2, 2, 3 ),
 ( 0.7500000000000000000, 0.7600000000000000089, 0.7800000000000000266, 0.8000000000000000444, 0.8199999999999999512, 0.8399999999999999689, 0.8499999999999999778 ),
 .UNSPECIFIED. ) 
 CURVE ( )  GEOMETRIC_REPRESENTATION_ITEM ( )  RATIONAL_B_SPLINE_CURVE ( ( 0.9755282581475768211, 0.9755282581475768211, 1.000000000000000000, 0.9510565162951535312, 1.000000000000000000, 0.9510565162951535312, 1.000000000000000000, 0.9510565162951535312, 1.000000000000000000, 0.9510565162951535312, 1.000000000000000000, 0.9755282581475768211, 0.9755282581475768211 ) ) 
 REPRESENTATION_ITEM ( '' )  );
#26117=CARTESIAN_POINT ( 'NONE',  ( -20.75514604977248823, 40.82500000273120122, -28.56700777964554305 ) ) ;
#26119=CARTESIAN_POINT ( 'NONE',  ( 33.58253175000000823, 68.27500000273120406, 10.91162601494192863 ) ) ;
#26120=CARTESIAN_POINT ( 'NONE',  ( 26.29305231718579350, 1.300000005462376151, 19.10302069950537529 ) ) ;
#26123=CARTESIAN_POINT ( 'NONE',  ( -26.29305231718579350, 49.80000000000001137, -19.10302069950537884 ) ) ;
#26125=CARTESIAN_POINT ( 'NONE',  ( -10.37757302488623701, 9.775000002731182747, 31.93888565452638417 ) ) ;
#26128=CARTESIAN_POINT ( 'NONE',  ( -8.960552108402742093E-16, 78.87500000273118417, -14.63369212191046387 ) ) ;
#26129=CARTESIAN_POINT ( 'NONE',  ( -33.58253175000000113, 79.27500000273120406, -10.91162601494193041 ) ) ;
#26130=CARTESIAN_POINT ( 'NONE',  ( -5.147494310547430452, 21.55125428154684286, -32.49999999999999289 ) ) ;
#26132=ORIENTED_EDGE ( 'NONE', *, *, #32426, .F. ) ;
#26145=CARTESIAN_POINT ( 'NONE',  ( -33.58253175000000113, 41.22500000273118559, 10.91162601494193929 ) ) ;
#26148=ADVANCED_FACE ( 'NONE', ( #20829 ), #15681, .T. ) ;
#26149=EDGE_CURVE ( 'NONE', #23750, #1559, #23731, .T. ) ;
#26151=EDGE_LOOP ( 'NONE', ( #21562, #3274, #8643, #13280 ) ) ;
#26153=CARTESIAN_POINT ( 'NONE',  ( -32.50000000000000000, 4.500000005462356789, 0.000000000000000000 ) ) ;
#26155=CARTESIAN_POINT ( 'NONE',  ( -33.58253175000000113, 75.47500000273116427, 10.91162601494193929 ) ) ;
#26158=ADVANCED_FACE ( 'NONE', ( #33683 ), #29032, .F. ) ;
#26160=( BOUNDED_CURVE ( )  B_SPLINE_CURVE ( 2, ( #26428, #13212, #23689, #15288, #13390, #15464, #24360, #21455, #5992, #16637, #3095, #21951, #6153 ),
 .UNSPECIFIED., .F., .T. ) 
 B_SPLINE_CURVE_WITH_KNOTS ( ( 3, 2, 2, 2, 2, 2, 3 ),
 ( 0.4935897435897436125, 0.4948717948717948900, 0.4974358974358974450, 0.5000000000000000000, 0.5025641025641025550, 0.5051282051282051100, 0.5064102564102563875 ),
 .UNSPECIFIED. ) 
 CURVE ( )  GEOMETRIC_REPRESENTATION_ITEM ( )  RATIONAL_B_SPLINE_CURVE ( ( 0.9755282581475768211, 0.9755282581475768211, 1.000000000000000000, 0.9510565162951535312, 1.000000000000000000, 0.9510565162951535312, 1.000000000000000000, 0.9510565162951535312, 1.000000000000000000, 0.9510565162951535312, 1.000000000000000000, 0.9755282581475768211, 0.9755282581475768211 ) ) 
 REPRESENTATION_ITEM ( '' )  );
#26161=ORIENTED_EDGE ( 'NONE', *, *, #23095, .F. ) ;
#26163=CARTESIAN_POINT ( 'NONE',  ( 20.75514604977248467, 58.42500000273119554, -28.56700777964554305 ) ) ;
#26165=VECTOR ( 'NONE', #2393, 1000.000000000000000 ) ;
#26167=CARTESIAN_POINT ( 'NONE',  ( -14.47279130897151767, 3.824999997268816454, -19.92008829642072598 ) ) ;
#26168=CARTESIAN_POINT ( 'NONE',  ( -20.75514604977248823, 2.825000002731177240, -28.56700777964554305 ) ) ;
#26169=CARTESIAN_POINT ( 'NONE',  ( -15.00000000000000000, 78.35000000546237686, 4.873795443493597723 ) ) ;
#26171=CARTESIAN_POINT ( 'NONE',  ( 27.16883889988624290, 78.17500000273119554, 19.73931689729373673 ) ) ;
#26173=CARTESIAN_POINT ( 'NONE',  ( -5.147494310547430452, 69.55125428154683220, -32.49999999999999289 ) ) ;
#26177=CARTESIAN_POINT ( 'NONE',  ( -11.25946833292375793, 80.67500000273119554, -8.180482586598733619 ) ) ;
#26179=CARTESIAN_POINT ( 'NONE',  ( 33.58253175000000113, 30.22500000273118559, -10.91162601494193751 ) ) ;
#26182=CARTESIAN_POINT ( 'NONE',  ( -33.58253175000000113, 13.27500000273119340, -10.91162601494193041 ) ) ;
#26184=CARTESIAN_POINT ( 'NONE',  ( -2.162160676586882350E-15, 76.62500000273116996, -35.31076352940722529 ) ) ;
#26185=DIRECTION ( 'NONE',  ( 0.000000000000000000, 0.000000000000000000, -1.000000000000000000 ) ) ;
#26187=CARTESIAN_POINT ( 'NONE',  ( 23.41746824999999887, 14.52499999726879842, 7.608796670333735079 ) ) ;
#26188=CARTESIAN_POINT ( 'NONE',  ( 27.16883889988623935, 62.32500000273119412, -19.73931689729374384 ) ) ;
#26192=CARTESIAN_POINT ( 'NONE',  ( 27.16883889988624290, 9.925000002731193760, 19.73931689729373673 ) ) ;
#26193=CARTESIAN_POINT ( 'NONE',  ( 23.41746824999999887, 17.12499999726882649, 0.000000000000000000 ) ) ;
#26197=EDGE_CURVE ( 'NONE', #4016, #2966, #16016, .T. ) ;
#26198=EDGE_LOOP ( 'NONE', ( #17416, #31840, #8462, #2630 ) ) ;
#26202=CARTESIAN_POINT ( 'NONE',  ( -32.50000000000000000, 71.89999999999999147, -10.55989012756945300 ) ) ;
#26204=CARTESIAN_POINT ( 'NONE',  ( 7.570916362186213000, 2.400000000000013234, -23.30088464923126423 ) ) ;
#26205=CARTESIAN_POINT ( 'NONE',  ( -20.75514604977248112, 13.67500000273118133, 28.56700777964554661 ) ) ;
#26206=CARTESIAN_POINT ( 'NONE',  ( -32.50000000000000000, 62.09999999999999432, 10.55989012756946366 ) ) ;
#26207=CARTESIAN_POINT ( 'NONE',  ( 20.08610463437157279, 57.80000000546236549, -27.64615127144129758 ) ) ;
#26208=CARTESIAN_POINT ( 'NONE',  ( -32.50000000000000000, 29.89999999999998437, -10.55989012756945300 ) ) ;
#26210=CARTESIAN_POINT ( 'NONE',  ( -11.25946833292375793, 79.17500000273119554, -8.180482586598733619 ) ) ;
#26213=LINE ( 'NONE', #18163, #23398 ) ;
#26214=CARTESIAN_POINT ( 'NONE',  ( -19.82091636218621034, 12.80000000000000604, -14.40073868116559552 ) ) ;
#26215=CARTESIAN_POINT ( 'NONE',  ( 32.50000000000000000, 5.099999999999983658, -10.55989012756945833 ) ) ;
#26217=CARTESIAN_POINT ( 'NONE',  ( -15.00000000000000000, 74.00000000000001421, 0.000000000000000000 ) ) ;
#26219=CARTESIAN_POINT ( 'NONE',  ( 27.16883889988623935, 48.32500000273117990, -19.73931689729374384 ) ) ;
#26221=CARTESIAN_POINT ( 'NONE',  ( 27.16883889988624290, 36.17500000273118843, 19.73931689729373673 ) ) ;
#26222=( BOUNDED_CURVE ( )  B_SPLINE_CURVE ( 2, ( #21111, #10299, #4158, #4972, #13040, #15449, #18200, #13201, #20776, #31555, #31220, #9469, #19951 ),
 .UNSPECIFIED., .F., .F. ) 
 B_SPLINE_CURVE_WITH_KNOTS ( ( 3, 2, 2, 2, 2, 2, 3 ),
 ( 0.4038461538461538547, 0.4051282051282051322, 0.4076923076923076872, 0.4102564102564102422, 0.4128205128205127972, 0.4153846153846154077, 0.4166666666666666852 ),
 .UNSPECIFIED. ) 
 CURVE ( )  GEOMETRIC_REPRESENTATION_ITEM ( )  RATIONAL_B_SPLINE_CURVE ( ( 0.9755282581475768211, 0.9755282581475768211, 1.000000000000000000, 0.9510565162951535312, 1.000000000000000000, 0.9510565162951535312, 1.000000000000000000, 0.9510565162951535312, 1.000000000000000000, 0.9510565162951535312, 1.000000000000000000, 0.9755282581475768211, 0.9755282581475768211 ) ) 
 REPRESENTATION_ITEM ( '' )  );
#26225=CARTESIAN_POINT ( 'NONE',  ( -32.50000000000000000, 61.89999999999999147, -10.55989012756945300 ) ) ;
#26227=( BOUNDED_CURVE ( )  B_SPLINE_CURVE ( 2, ( #410, #67, #31979, #12960, #3173, #5574, #31646, #13643, #31813, #8303, #23434, #5743, #23771 ),
 .UNSPECIFIED., .F., .F. ) 
 B_SPLINE_CURVE_WITH_KNOTS ( ( 3, 2, 2, 2, 2, 2, 3 ),
 ( 0.9679487179487179516, 0.9692307692307692291, 0.9717948717948717841, 0.9743589743589743390, 0.9769230769230768940, 0.9794871794871794490, 0.9807692307692307265 ),
 .UNSPECIFIED. ) 
 CURVE ( )  GEOMETRIC_REPRESENTATION_ITEM ( )  RATIONAL_B_SPLINE_CURVE ( ( 0.9755282581475768211, 0.9755282581475768211, 1.000000000000000000, 0.9510565162951535312, 1.000000000000000000, 0.9510565162951535312, 1.000000000000000000, 0.9510565162951535312, 1.000000000000000000, 0.9510565162951535312, 1.000000000000000000, 0.9755282581475768211, 0.9755282581475768211 ) ) 
 REPRESENTATION_ITEM ( '' )  );
#26232=CARTESIAN_POINT ( 'NONE',  ( 7.570916362186207671, 9.349999994537617098, 23.30088464923126779 ) ) ;
#26235=CARTESIAN_POINT ( 'NONE',  ( 5.147494310547217289, 10.55125428154683576, 32.50000000000007105 ) ) ;
#26236=CARTESIAN_POINT ( 'NONE',  ( -33.58253175000000113, 29.22500000273118914, 10.91162601494193929 ) ) ;
#26245=EDGE_CURVE ( 'NONE', #26701, #21850, #14390, .T. ) ;
#26246=CARTESIAN_POINT ( 'NONE',  ( -1.778240108872766143E-15, 9.499999999999992895, -32.49999999999999289 ) ) ;
#26247=CARTESIAN_POINT ( 'NONE',  ( -10.37757302488624411, 36.97500000273118559, -31.93888565452638417 ) ) ;
#26248=CARTESIAN_POINT ( 'NONE',  ( 10.04305231718578817, 35.90000000546239534, -30.90933677959249337 ) ) ;
#26249=CARTESIAN_POINT ( 'NONE',  ( 6.277390505771533514E-15, 78.49999999999998579, 34.17252228774368916 ) ) ;
#26250=CARTESIAN_POINT ( 'NONE',  ( -14.45873412499999944, 71.68750000136559208, 0.000000000000000000 ) ) ;
#26251=CARTESIAN_POINT ( 'NONE',  ( 10.04305231718579705, 31.10000000546236976, 30.90933677959248982 ) ) ;
#26252=CARTESIAN_POINT ( 'NONE',  ( -27.16883889988624290, 47.17500000273119554, -19.73931689729374028 ) ) ;
#26254=CARTESIAN_POINT ( 'NONE',  ( 32.50000000000000711, 24.90000000000000213, 10.55989012756945122 ) ) ;
#26256=CARTESIAN_POINT ( 'NONE',  ( 20.75514604977248467, 70.42500000273119554, -28.56700777964554305 ) ) ;
#26259=CARTESIAN_POINT ( 'NONE',  ( -27.16883889988624290, 57.17500000273118133, -19.73931689729374028 ) ) ;
#26260=CARTESIAN_POINT ( 'NONE',  ( 5.147494310547408247, 72.55125428154684641, 32.50000000000000711 ) ) ;
#26261=CARTESIAN_POINT ( 'NONE',  ( -20.75514604977248823, 12.82500000273118168, -28.56700777964554305 ) ) ;
#26263=DIRECTION ( 'NONE',  ( 0.000000000000000000, 0.000000000000000000, 1.000000000000000000 ) ) ;
#26264=CARTESIAN_POINT ( 'NONE',  ( -20.75514604977248112, 5.675000002731203530, 28.56700777964554661 ) ) ;
#26266=CARTESIAN_POINT ( 'NONE',  ( 5.779280353836490358E-15, 16.50000000000000000, 32.49999999999999289 ) ) ;
#26274=CARTESIAN_POINT ( 'NONE',  ( 7.236395654485760609, 3.524999997268824181, -22.27133577429736633 ) ) ;
#26275=CARTESIAN_POINT ( 'NONE',  ( 10.04305231718578817, 67.90000000546237402, -30.90933677959249337 ) ) ;
#26283=CARTESIAN_POINT ( 'NONE',  ( -5.147494310547430452, 35.55125428154683220, -32.49999999999999289 ) ) ;
#26284=EDGE_CURVE ( 'NONE', #7065, #16121, #16845, .T. ) ;
#26285=CARTESIAN_POINT ( 'NONE',  ( 33.58253175000000113, 56.37500000273118417, -4.112674001490185761E-15 ) ) ;
#26286=ADVANCED_FACE ( 'NONE', ( #1029 ), #8433, .T. ) ;
#26287=CARTESIAN_POINT ( 'NONE',  ( 6.277390505771533514E-15, 55.00000000546239676, 34.17252228774368916 ) ) ;
#26288=CARTESIAN_POINT ( 'NONE',  ( 7.313012447739250820E-14, 13.24999999453762456, 24.50000000000000000 ) ) ;
#26289=CARTESIAN_POINT ( 'NONE',  ( 10.37757302488624767, 39.72500000273118559, 31.93888565452638417 ) ) ;
#26290=CARTESIAN_POINT ( 'NONE',  ( 10.04305231718578817, 55.40000000000000568, -30.90933677959249337 ) ) ;
#26291=CARTESIAN_POINT ( 'NONE',  ( -10.37757302488623701, 69.77500000273117564, 31.93888565452638417 ) ) ;
#26295=CARTESIAN_POINT ( 'NONE',  ( -32.50000000000000000, 45.89999999999999858, -10.55989012756945478 ) ) ;
#26297=CARTESIAN_POINT ( 'NONE',  ( 33.58253175000000823, 10.27500000273117564, 10.91162601494192863 ) ) ;
#26298=CARTESIAN_POINT ( 'NONE',  ( 20.08610463437157279, 35.80000000546235839, -27.64615127144129758 ) ) ;
#26300=CARTESIAN_POINT ( 'NONE',  ( 13.91746824999999532, 72.47500000273119269, -4.522059556121118540 ) ) ;
#26301=CARTESIAN_POINT ( 'NONE',  ( 6.486482029760648627E-15, 77.87500000273118417, 35.31076352940722529 ) ) ;
#26302=DIRECTION ( 'NONE',  ( -0.000000000000000000, -1.000000000000000000, -0.000000000000000000 ) ) ;
#26304=ORIENTED_EDGE ( 'NONE', *, *, #8603, .F. ) ;
#26315=CARTESIAN_POINT ( 'NONE',  ( 10.37757302488624056, 36.52500000273117564, -31.93888565452638417 ) ) ;
#26318=CARTESIAN_POINT ( 'NONE',  ( 0.000000000000000000, 0.000000000000000000, 0.000000000000000000 ) ) ;
#26321=( BOUNDED_CURVE ( )  B_SPLINE_CURVE ( 2, ( #9698, #12097, #25143, #7290, #9524, #20005, #1619, #20347, #15199, #30452, #11932, #17775, #6949 ),
 .UNSPECIFIED., .F., .F. ) 
 B_SPLINE_CURVE_WITH_KNOTS ( ( 3, 2, 2, 2, 2, 2, 3 ),
 ( 0.2115384615384615363, 0.2128205128205128138, 0.2153846153846153966, 0.2179487179487179516, 0.2205128205128205066, 0.2230769230769230893, 0.2243589743589743668 ),
 .UNSPECIFIED. ) 
 CURVE ( )  GEOMETRIC_REPRESENTATION_ITEM ( )  RATIONAL_B_SPLINE_CURVE ( ( 0.9755282581475768211, 0.9755282581475768211, 1.000000000000000000, 0.9510565162951535312, 1.000000000000000000, 0.9510565162951535312, 1.000000000000000000, 0.9510565162951535312, 1.000000000000000000, 0.9510565162951535312, 1.000000000000000000, 0.9755282581475768211, 0.9755282581475768211 ) ) 
 REPRESENTATION_ITEM ( '' )  );
#26322=CARTESIAN_POINT ( 'NONE',  ( 32.50000000000000711, 50.89999999999999147, 10.55989012756945122 ) ) ;
#26324=CARTESIAN_POINT ( 'NONE',  ( -27.16883889988624290, 67.17500000273119554, -19.73931689729374028 ) ) ;
#26325=ORIENTED_EDGE ( 'NONE', *, *, #17014, .T. ) ;
#26328=ORIENTED_EDGE ( 'NONE', *, *, #1847, .F. ) ;
#26329=CARTESIAN_POINT ( 'NONE',  ( 5.779280353836490358E-15, 15.00000000546237899, 32.49999999999999289 ) ) ;
#26330=CARTESIAN_POINT ( 'NONE',  ( 10.37757302488624056, 62.52500000273120406, -31.93888565452638417 ) ) ;
#26333=CARTESIAN_POINT ( 'NONE',  ( 7.236395654485755280, 6.724999997268804819, 22.27133577429736988 ) ) ;
#26334=CARTESIAN_POINT ( 'NONE',  ( -27.16883889988624290, 6.925000002731191096, -19.73931689729374028 ) ) ;
#26335=CARTESIAN_POINT ( 'NONE',  ( 33.58253175000000113, 30.47500000273117493, -10.91162601494193751 ) ) ;
#26336=CARTESIAN_POINT ( 'NONE',  ( 5.147494310547426899, 5.948745723915523698, -32.50000000000000000 ) ) ;
#26339=CARTESIAN_POINT ( 'NONE',  ( -4.300734207923759378, 78.47500000273119269, -13.23629886949340495 ) ) ;
#26340=CARTESIAN_POINT ( 'NONE',  ( 5.779280353836490358E-15, 75.00000000546236834, 32.49999999999999289 ) ) ;
#26344=CARTESIAN_POINT ( 'NONE',  ( -15.00000000000000000, 72.15000000546237402, -4.873795443493594171 ) ) ;
#26346=CARTESIAN_POINT ( 'NONE',  ( 10.37757302488624767, 27.72500000273120335, 31.93888565452638417 ) ) ;
#26349=CARTESIAN_POINT ( 'NONE',  ( 20.75514604977249178, 14.07500000273119944, 28.56700777964553950 ) ) ;
#26352=CARTESIAN_POINT ( 'NONE',  ( 20.75514604977248467, 76.42500000273118133, -28.56700777964554305 ) ) ;
#26353=CARTESIAN_POINT ( 'NONE',  ( 0.000000000000000000, 80.00000000000001421, 0.000000000000000000 ) ) ;
#26355=CARTESIAN_POINT ( 'NONE',  ( 12.13525491562420910, 79.45000000546237118, -8.816778784387098611 ) ) ;
#26356=CARTESIAN_POINT ( 'NONE',  ( -20.75514604977248112, 55.42500000273120264, 28.56700777964554661 ) ) ;
#26359=ORIENTED_EDGE ( 'NONE', *, *, #16405, .F. ) ;
#26361=CARTESIAN_POINT ( 'NONE',  ( -33.58253175000000113, 1.225000002731198467, 10.91162601494193929 ) ) ;
#26362=CARTESIAN_POINT ( 'NONE',  ( -23.41746824999999887, 1.624999997268811169, -2.867812753649727150E-15 ) ) ;
#26372=CARTESIAN_POINT ( 'NONE',  ( -20.08610463437157989, 71.69999999999997442, -27.64615127144129758 ) ) ;
#26374=CARTESIAN_POINT ( 'NONE',  ( 19.82091636218621389, 0.2000000000000057288, -14.40073868116559197 ) ) ;
#26375=CARTESIAN_POINT ( 'NONE',  ( -20.75514604977248112, 7.675000002731199089, 28.56700777964554661 ) ) ;
#26376=CARTESIAN_POINT ( 'NONE',  ( 10.04305231718579705, 60.59999999999998721, 30.90933677959248982 ) ) ;
#26377=CARTESIAN_POINT ( 'NONE',  ( 4.300734207923757602, 78.27500000273118985, -13.23629886949340673 ) ) ;
#26378=CARTESIAN_POINT ( 'NONE',  ( 5.779280353836490358E-15, 30.49999999999999645, 32.49999999999999289 ) ) ;
#26380=CARTESIAN_POINT ( 'NONE',  ( -13.91746824999999532, 79.27500000273118985, -4.522059556121115875 ) ) ;
#26383=DIRECTION ( 'NONE',  ( -0.000000000000000000, -1.000000000000000000, -0.000000000000000000 ) ) ;
#26384=CARTESIAN_POINT ( 'NONE',  ( -3.880418787951138260, 1.448745718453166020, 24.50000000000000000 ) ) ;
#26385=CARTESIAN_POINT ( 'NONE',  ( -2.092463501923844636E-15, 3.500000000000005329, -34.17252228774368916 ) ) ;
#26388=CARTESIAN_POINT ( 'NONE',  ( -2.162160676586881955E-15, 44.62500000273119838, -35.31076352940723240 ) ) ;
#26391=CARTESIAN_POINT ( 'NONE',  ( -33.58253175000000113, 37.27500000273118985, -10.91162601494193041 ) ) ;
#26392=CARTESIAN_POINT ( 'NONE',  ( 5.779280353836490358E-15, 24.50000000000000711, 32.49999999999999289 ) ) ;
#26393=DIRECTION ( 'NONE',  ( -0.000000000000000000, -1.000000000000000000, -0.000000000000000000 ) ) ;
#26395=CARTESIAN_POINT ( 'NONE',  ( 32.50000000000000000, 51.60000000546239107, -10.55989012756945833 ) ) ;
#26398=CARTESIAN_POINT ( 'NONE',  ( -14.47279130897151767, 1.324999997268808238, -19.92008829642072598 ) ) ;
#26399=CARTESIAN_POINT ( 'NONE',  ( 24.50000000000000000, 9.849999994537622428, -7.960532557706203605 ) ) ;
#26402=CARTESIAN_POINT ( 'NONE',  ( -26.29305231718579350, 11.80000000000000426, -19.10302069950537884 ) ) ;
#26403=CARTESIAN_POINT ( 'NONE',  ( 20.75514604977249178, 23.82500000273118346, 28.56700777964553950 ) ) ;
#26406=ORIENTED_EDGE ( 'NONE', *, *, #16371, .F. ) ;
#26408=ORIENTED_EDGE ( 'NONE', *, *, #21950, .T. ) ;
#26413=DIRECTION ( 'NONE',  ( 0.000000000000000000, 0.000000000000000000, -1.000000000000000000 ) ) ;
#26414=CARTESIAN_POINT ( 'NONE',  ( 10.37757302488624767, 31.97500000273117848, 31.93888565452638417 ) ) ;
#26415=CARTESIAN_POINT ( 'NONE',  ( 20.08610463437158344, 35.20000000546237828, 27.64615127144129403 ) ) ;
#26416=CARTESIAN_POINT ( 'NONE',  ( 10.04305231718579705, 78.60000000000000853, 30.90933677959248982 ) ) ;
#26417=CARTESIAN_POINT ( 'NONE',  ( 20.08610463437157279, 53.29999999999999716, -27.64615127144129758 ) ) ;
#26418=CARTESIAN_POINT ( 'NONE',  ( 26.29305231718578995, 77.19999999999998863, -19.10302069950538240 ) ) ;
#26419=CARTESIAN_POINT ( 'NONE',  ( 33.58253175000000113, 44.37500000273119838, -4.112674001490185761E-15 ) ) ;
#26420=( BOUNDED_CURVE ( )  B_SPLINE_CURVE ( 2, ( #14467, #24924, #904, #21862, #19284, #16713, #24592, #29901, #17731, #2100, #12573, #9654, #30753 ),
 .UNSPECIFIED., .F., .T. ) 
 B_SPLINE_CURVE_WITH_KNOTS ( ( 3, 2, 2, 2, 2, 2, 3 ),
 ( 0.6858974358974359031, 0.6871794871794871806, 0.6897435897435897356, 0.6923076923076922906, 0.6948717948717948456, 0.6974358974358974006, 0.6987179487179486781 ),
 .UNSPECIFIED. ) 
 CURVE ( )  GEOMETRIC_REPRESENTATION_ITEM ( )  RATIONAL_B_SPLINE_CURVE ( ( 0.9755282581475768211, 0.9755282581475768211, 1.000000000000000000, 0.9510565162951535312, 1.000000000000000000, 0.9510565162951535312, 1.000000000000000000, 0.9510565162951535312, 1.000000000000000000, 0.9510565162951535312, 1.000000000000000000, 0.9755282581475768211, 0.9755282581475768211 ) ) 
 REPRESENTATION_ITEM ( '' )  );
#26422=CARTESIAN_POINT ( 'NONE',  ( -20.08610463437157989, 19.69999999999998863, -27.64615127144129758 ) ) ;
#26424=CARTESIAN_POINT ( 'NONE',  ( 27.16883889988624290, 71.92500000273119554, 19.73931689729373673 ) ) ;
#26426=CARTESIAN_POINT ( 'NONE',  ( -10.04305231718578462, 76.90000000546237402, 30.90933677959249337 ) ) ;
#26427=CARTESIAN_POINT ( 'NONE',  ( 27.16883889988624290, 54.17500000273117422, 19.73931689729373673 ) ) ;
#26428=CARTESIAN_POINT ( 'NONE',  ( -1.778240108872766143E-15, 40.00000000546237544, -32.49999999999999289 ) ) ;
#26429=CARTESIAN_POINT ( 'NONE',  ( -10.37757302488623701, 9.525000002731182747, 31.93888565452638417 ) ) ;
#26431=EDGE_CURVE ( 'NONE', #22217, #26665, #16998, .T. ) ;
#26436=CARTESIAN_POINT ( 'NONE',  ( 0.000000000000000000, 80.00000000000001421, -32.50000000000000000 ) ) ;
#26437=EDGE_CURVE ( 'NONE', #8956, #438, #2768, .T. ) ;
#26442=CARTESIAN_POINT ( 'NONE',  ( 10.04305231718579705, 60.59999999999998721, 30.90933677959248982 ) ) ;
#26445=CARTESIAN_POINT ( 'NONE',  ( -2.092463501923844636E-15, 72.00000000546236834, -34.17252228774368916 ) ) ;
#26448=FACE_OUTER_BOUND ( 'NONE', #7269, .T. ) ;
#26449=ORIENTED_EDGE ( 'NONE', *, *, #21220, .T. ) ;
#26453=CARTESIAN_POINT ( 'NONE',  ( 5.147494310547426899, 21.44874571845315003, -32.50000000000000000 ) ) ;
#26454=CARTESIAN_POINT ( 'NONE',  ( 6.486482029760649416E-15, 53.87500000273118417, 35.31076352940723240 ) ) ;
#26455=CARTESIAN_POINT ( 'NONE',  ( 32.50000000000000000, 53.50000000546237544, -3.980102097228898626E-15 ) ) ;
#26457=CARTESIAN_POINT ( 'NONE',  ( 27.16883889988623935, 38.32500000273120122, -19.73931689729374384 ) ) ;
#26459=CARTESIAN_POINT ( 'NONE',  ( -10.37757302488624411, 66.97500000273117848, -31.93888565452638417 ) ) ;
#26463=CARTESIAN_POINT ( 'NONE',  ( -32.50000000000000000, 40.09999999999998721, 10.55989012756946366 ) ) ;
#26465=CARTESIAN_POINT ( 'NONE',  ( 20.75514604977248467, 8.675000002731195536, -28.56700777964554305 ) ) ;
#26466=CARTESIAN_POINT ( 'NONE',  ( 24.50000000000000000, 19.74999999453763877, 0.000000000000000000 ) ) ;
#26468=DIRECTION ( 'NONE',  ( 0.000000000000000000, 0.000000000000000000, -1.000000000000000000 ) ) ;
#26469=CARTESIAN_POINT ( 'NONE',  ( -33.58253175000000113, 73.47500000273119269, 10.91162601494193929 ) ) ;
#26470=CARTESIAN_POINT ( 'NONE',  ( 3.980102097228898626E-15, 80.00000000000001421, 32.50000000000000000 ) ) ;
#26472=ORIENTED_EDGE ( 'NONE', *, *, #29672, .F. ) ;
#26475=EDGE_CURVE ( 'NONE', #18611, #5175, #27470, .T. ) ;
#26484=CARTESIAN_POINT ( 'NONE',  ( -2.162160676586882350E-15, 38.62500000273118417, -35.31076352940722529 ) ) ;
#26487=CARTESIAN_POINT ( 'NONE',  ( -4.405589869732278832E-13, 10.49999999999998934, 32.50000000000000000 ) ) ;
#26492=CARTESIAN_POINT ( 'NONE',  ( -10.37757302488623701, 71.77500000273117564, 31.93888565452638417 ) ) ;
#26493=ORIENTED_EDGE ( 'NONE', *, *, #9981, .F. ) ;
#26495=AXIS2_PLACEMENT_3D ( 'NONE', #31605, #18590, #26468 ) ;
#26498=CARTESIAN_POINT ( 'NONE',  ( 32.50000000000000000, 65.60000000546239107, -10.55989012756945833 ) ) ;
#26499=CARTESIAN_POINT ( 'NONE',  ( 10.37757302488624056, 64.52500000273120406, -31.93888565452638417 ) ) ;
#26501=CARTESIAN_POINT ( 'NONE',  ( -10.04305231718579172, 16.10000000546238397, -30.90933677959248982 ) ) ;
#26502=CARTESIAN_POINT ( 'NONE',  ( 1.577395562988744260E-15, 16.50000000000000000, -25.76082449383753925 ) ) ;
#26503=CARTESIAN_POINT ( 'NONE',  ( -18.94512977948576093, 8.324999997268822227, 13.76444248337722698 ) ) ;
#26504=CARTESIAN_POINT ( 'NONE',  ( 33.58253175000000823, 6.025000002731191628, 10.91162601494192863 ) ) ;
#26505=CARTESIAN_POINT ( 'NONE',  ( 10.37757302488624056, 32.77500000273120406, -31.93888565452638417 ) ) ;
#26509=CARTESIAN_POINT ( 'NONE',  ( -20.08610463437157989, 31.69999999999998508, -27.64615127144129758 ) ) ;
#26514=CARTESIAN_POINT ( 'NONE',  ( -11.25946833292375793, 73.07500000273120122, 8.180482586598737171 ) ) ;
#26516=CARTESIAN_POINT ( 'NONE',  ( 10.37757302488624056, 26.52500000273119696, -31.93888565452638417 ) ) ;
#26519=CARTESIAN_POINT ( 'NONE',  ( -33.58253175000000113, 15.27500000273118985, -10.91162601494193041 ) ) ;
#26522=CARTESIAN_POINT ( 'NONE',  ( -27.16883889988624290, 72.92500000273119554, -19.73931689729374028 ) ) ;
#26523=CARTESIAN_POINT ( 'NONE',  ( 5.147494310547426899, 3.948745723915525474, -32.50000000000000000 ) ) ;
#26524=( BOUNDED_CURVE ( )  B_SPLINE_CURVE ( 2, ( #30894, #30719, #1545, #7043, #12368, #14775, #2066, #4813, #17873, #12021, #9796, #22665, #14947 ),
 .UNSPECIFIED., .F., .T. ) 
 B_SPLINE_CURVE_WITH_KNOTS ( ( 3, 2, 2, 2, 2, 2, 3 ),
 ( 0.4166666666666666852, 0.4179487179487179627, 0.4205128205128205177, 0.4230769230769230727, 0.4256410256410256276, 0.4282051282051281826, 0.4294871794871795156 ),
 .UNSPECIFIED. ) 
 CURVE ( )  GEOMETRIC_REPRESENTATION_ITEM ( )  RATIONAL_B_SPLINE_CURVE ( ( 0.9755282581475768211, 0.9755282581475768211, 1.000000000000000000, 0.9510565162951535312, 1.000000000000000000, 0.9510565162951535312, 1.000000000000000000, 0.9510565162951535312, 1.000000000000000000, 0.9510565162951535312, 1.000000000000000000, 0.9755282581475762660, 0.9755282581475768211 ) ) 
 REPRESENTATION_ITEM ( '' )  );
#26526=CARTESIAN_POINT ( 'NONE',  ( -4.635254915624208216, 72.65000000546240244, 14.26584774442730463 ) ) ;
#26527=CARTESIAN_POINT ( 'NONE',  ( -10.37757302488623701, 55.52500000273119696, 31.93888565452638417 ) ) ;
#26532=CARTESIAN_POINT ( 'NONE',  ( -7.236395654485757944, 17.72499999726881370, -22.27133577429736988 ) ) ;
#26534=ORIENTED_EDGE ( 'NONE', *, *, #26437, .T. ) ;
#26536=CARTESIAN_POINT ( 'NONE',  ( -20.08610463437156923, 42.80000000546237970, 27.64615127144130113 ) ) ;
#26537=ORIENTED_EDGE ( 'NONE', *, *, #7796, .F. ) ;
#26539=CARTESIAN_POINT ( 'NONE',  ( 10.04305231718578817, 5.400000000000016342, -30.90933677959249337 ) ) ;
#26540=CARTESIAN_POINT ( 'NONE',  ( 23.95873412499999944, 19.43749999590321664, 0.000000000000000000 ) ) ;
#26542=CARTESIAN_POINT ( 'NONE',  ( 1.507698388325705758E-15, 17.12499999726880517, -24.62258325217400312 ) ) ;
#26543=CARTESIAN_POINT ( 'NONE',  ( -33.58253175000000113, 9.275000002731177418, -10.91162601494193218 ) ) ;
#26544=CARTESIAN_POINT ( 'NONE',  ( -20.08610463437157989, 61.69999999999999574, -27.64615127144129758 ) ) ;
#26545=CARTESIAN_POINT ( 'NONE',  ( 13.91746824999999532, 79.97500000273119269, -4.522059556121118540 ) ) ;
#26548=CARTESIAN_POINT ( 'NONE',  ( 13.91746824999999887, 74.37500000273116996, -1.704398294459741270E-15 ) ) ;
#26551=DIRECTION ( 'NONE',  ( -0.000000000000000000, -1.000000000000000000, -0.000000000000000000 ) ) ;
#26552=DIRECTION ( 'NONE',  ( 0.000000000000000000, 0.000000000000000000, -1.000000000000000000 ) ) ;
#26553=CARTESIAN_POINT ( 'NONE',  ( -26.29305231718578995, 2.199999999999979750, 19.10302069950538595 ) ) ;
#26556=CARTESIAN_POINT ( 'NONE',  ( -27.16883889988624290, 46.92500000273119554, -19.73931689729374028 ) ) ;
#26559=CARTESIAN_POINT ( 'NONE',  ( 33.58253175000000113, 34.37500000273119127, -4.112674001490185761E-15 ) ) ;
#26564=CARTESIAN_POINT ( 'NONE',  ( -20.08610463437156923, 44.80000000546236549, 27.64615127144130113 ) ) ;
#26567=CARTESIAN_POINT ( 'NONE',  ( -7.236395654485757944, 3.224999997268801266, -22.27133577429736988 ) ) ;
#26568=ADVANCED_FACE ( 'NONE', ( #31940 ), #21659, .T. ) ;
#26569=CYLINDRICAL_SURFACE ( 'NONE', #2329, 32.50000000000000000 ) ;
#26571=CARTESIAN_POINT ( 'NONE',  ( 33.58253175000000823, 18.02500000273118985, 10.91162601494192685 ) ) ;
#26581=VERTEX_POINT ( 'NONE', #30802 ) ;
#26582=CARTESIAN_POINT ( 'NONE',  ( -23.41746825000000598, 1.724999997268824581, 7.608796670333726198 ) ) ;
#26583=CARTESIAN_POINT ( 'NONE',  ( -10.37757302488623701, 25.77500000273119696, 31.93888565452638417 ) ) ;
#26584=COLOUR_RGB ( '', 0.09019608, 0.27058824, 0.51372549) ;
#26585=CARTESIAN_POINT ( 'NONE',  ( -10.04305231718579172, 36.10000000546237686, -30.90933677959248982 ) ) ;
#26586=CARTESIAN_POINT ( 'NONE',  ( -32.50000000000000000, 80.00000000000001421, 0.000000000000000000 ) ) ;
#26589=CARTESIAN_POINT ( 'NONE',  ( 6.486482029760649416E-15, 43.87500000273118417, 35.31076352940723240 ) ) ;
#26591=CARTESIAN_POINT ( 'NONE',  ( 20.08610463437158344, 20.69999999999998508, 27.64615127144129403 ) ) ;
#26593=CARTESIAN_POINT ( 'NONE',  ( 33.58253175000000113, 64.22500000273117848, -10.91162601494193751 ) ) ;
#26594=CARTESIAN_POINT ( 'NONE',  ( -20.08610463437156923, 78.29999999999999716, 27.64615127144130113 ) ) ;
#26596=CARTESIAN_POINT ( 'NONE',  ( -33.58253175000000113, 51.47500000273118559, 10.91162601494193929 ) ) ;
#26599=CARTESIAN_POINT ( 'NONE',  ( 33.58253175000000823, 10.02500000273118275, 10.91162601494192863 ) ) ;
#26601=CARTESIAN_POINT ( 'NONE',  ( 0.000000000000000000, 0.000000000000000000, 0.000000000000000000 ) ) ;
#26604=CARTESIAN_POINT ( 'NONE',  ( 5.779280353836490358E-15, 19.00000000546237544, 32.49999999999999289 ) ) ;
#26605=CARTESIAN_POINT ( 'NONE',  ( -32.50000000000000000, 58.40000000546237402, -10.55989012756945300 ) ) ;
#26612=CARTESIAN_POINT ( 'NONE',  ( 10.04305231718578817, 71.90000000546237402, -30.90933677959249337 ) ) ;
#26618=AXIS2_PLACEMENT_3D ( 'NONE', #12534, #28317, #19917 ) ;
#26621=CARTESIAN_POINT ( 'NONE',  ( 20.08610463437158344, 74.70000000000000284, 27.64615127144129403 ) ) ;
#26622=CARTESIAN_POINT ( 'NONE',  ( 33.58253175000000113, 50.37500000273120548, -4.112674001490185761E-15 ) ) ;
#26623=CARTESIAN_POINT ( 'NONE',  ( -32.50000000000000000, 58.60000000546236976, 10.55989012756946366 ) ) ;
#26624=ADVANCED_FACE ( 'NONE', ( #7124 ), #15553, .T. ) ;
#26626=CARTESIAN_POINT ( 'NONE',  ( -33.58253175000000113, 35.02500000273118275, -10.91162601494193218 ) ) ;
#26627=CARTESIAN_POINT ( 'NONE',  ( 9.270509831248425314, 72.95000000546238539, 12.75976212528059683 ) ) ;
#26628=CARTESIAN_POINT ( 'NONE',  ( 10.37757302488624767, 63.97500000273120691, 31.93888565452638417 ) ) ;
#26632=CARTESIAN_POINT ( 'NONE',  ( 26.29305231718578995, 41.20000000000001705, -19.10302069950538240 ) ) ;
#26634=CARTESIAN_POINT ( 'NONE',  ( 33.58253175000000823, 6.275000002731184523, 10.91162601494192863 ) ) ;
#26635=FACE_OUTER_BOUND ( 'NONE', #23329, .T. ) ;
#26636=CARTESIAN_POINT ( 'NONE',  ( 13.91746824999999532, 74.47500000273116427, -4.522059556121118540 ) ) ;
#26637=CARTESIAN_POINT ( 'NONE',  ( -33.58253175000000113, 73.27500000273120406, -10.91162601494193041 ) ) ;
#26638=CARTESIAN_POINT ( 'NONE',  ( 0.000000000000000000, 80.00000000000001421, -32.50000000000000000 ) ) ;
#26640=ORIENTED_EDGE ( 'NONE', *, *, #9990, .F. ) ;
#26651=CARTESIAN_POINT ( 'NONE',  ( -26.29305231718579350, 56.30000000546237260, -19.10302069950537884 ) ) ;
#26652=CARTESIAN_POINT ( 'NONE',  ( -20.75514604977248823, 38.82500000273120122, -28.56700777964554305 ) ) ;
#26658=CARTESIAN_POINT ( 'NONE',  ( 5.779280353836490358E-15, 50.50000000000000000, 32.49999999999999289 ) ) ;
#26660=CARTESIAN_POINT ( 'NONE',  ( 27.16883889988624290, 72.17500000273119554, 19.73931689729373673 ) ) ;
#26661=ORIENTED_EDGE ( 'NONE', *, *, #17983, .F. ) ;
#26665=VERTEX_POINT ( 'NONE', #21397 ) ;
#26667=CARTESIAN_POINT ( 'NONE',  ( -27.16883889988623935, 55.32500000273118701, 19.73931689729374739 ) ) ;
#26670=CARTESIAN_POINT ( 'NONE',  ( 32.50000000000000000, 15.60000000546238930, -10.55989012756945833 ) ) ;
#26671=CARTESIAN_POINT ( 'NONE',  ( 0.000000000000000000, 80.00000000000001421, -32.50000000000000000 ) ) ;
#26673=CARTESIAN_POINT ( 'NONE',  ( -7.236395654485757944, 9.724999997268806595, -22.27133577429736988 ) ) ;
#26674=CARTESIAN_POINT ( 'NONE',  ( -33.58253175000000113, 27.47500000273118204, 10.91162601494193929 ) ) ;
#26675=CARTESIAN_POINT ( 'NONE',  ( -2.375766604868044585, 78.69874572391553613, 14.99999999999999822 ) ) ;
#26677=CARTESIAN_POINT ( 'NONE',  ( -32.50000000000000000, 32.00000000000000000, 0.000000000000000000 ) ) ;
#26678=CARTESIAN_POINT ( 'NONE',  ( 5.147494310547440222, 75.94874572391553613, -32.50000000000000000 ) ) ;
#26682=CARTESIAN_POINT ( 'NONE',  ( 13.91746824999999887, 77.87500000273116996, -1.704398294459741270E-15 ) ) ;
#26684=CARTESIAN_POINT ( 'NONE',  ( 10.37757302488624767, 23.72500000273119980, 31.93888565452638417 ) ) ;
#26687=CARTESIAN_POINT ( 'NONE',  ( -10.37757302488623701, 13.77500000273118630, 31.93888565452638417 ) ) ;
#26689=CARTESIAN_POINT ( 'NONE',  ( 27.16883889988624290, 67.92500000273119554, 19.73931689729373673 ) ) ;
#26690=CARTESIAN_POINT ( 'NONE',  ( 3.980102097228898626E-15, 80.00000000000001421, 32.50000000000000000 ) ) ;
#26692=CARTESIAN_POINT ( 'NONE',  ( 9.270509831248421762, 79.55000000546237970, -12.75976212528059861 ) ) ;
#26693=CARTESIAN_POINT ( 'NONE',  ( -27.16883889988624290, 56.92500000273120975, -19.73931689729374028 ) ) ;
#26696=VERTEX_POINT ( 'NONE', #29763 ) ;
#26698=CARTESIAN_POINT ( 'NONE',  ( -26.29305231718579350, 15.79999999999998117, -19.10302069950537884 ) ) ;
#26699=CARTESIAN_POINT ( 'NONE',  ( 18.94512977948576093, 8.824999997268822227, -13.76444248337722875 ) ) ;
#26701=VERTEX_POINT ( 'NONE', #6270 ) ;
#26702=AXIS2_PLACEMENT_3D ( 'NONE', #12250, #24616, #1600 ) ;
#26705=ORIENTED_EDGE ( 'NONE', *, *, #24376, .T. ) ;
#26708=CARTESIAN_POINT ( 'NONE',  ( -15.14183272437242778, 3.300000000000012257, 20.84094480462497856 ) ) ;
#26709=CARTESIAN_POINT ( 'NONE',  ( 10.37757302488624056, 74.52500000273118985, -31.93888565452638417 ) ) ;
#26711=CARTESIAN_POINT ( 'NONE',  ( -7.570916362186215665, 1.400000000000012346, 23.30088464923126423 ) ) ;
#26713=CARTESIAN_POINT ( 'NONE',  ( -33.58253175000000113, 11.37500000273117351, 0.000000000000000000 ) ) ;
#26714=CARTESIAN_POINT ( 'NONE',  ( -27.16883889988624290, 20.92500000273117422, -19.73931689729374028 ) ) ;
#26715=CARTESIAN_POINT ( 'NONE',  ( 2.688165632520823219E-15, 77.37500000273116996, 14.63369212191046209 ) ) ;
#26718=CARTESIAN_POINT ( 'NONE',  ( 4.300734207923761154, 73.97500000273119269, 13.23629886949340495 ) ) ;
#26721=CARTESIAN_POINT ( 'NONE',  ( -4.934616302121927505E-14, 70.50000000000000000, 32.50000000000000000 ) ) ;
#26723=( BOUNDED_CURVE ( )  B_SPLINE_CURVE ( 2, ( #21629, #13573, #8574, #837, #11318, #16646, #30002, #26605, #27101, #11483, #32409, #21464, #24037 ),
 .UNSPECIFIED., .F., .T. ) 
 B_SPLINE_CURVE_WITH_KNOTS ( ( 3, 2, 2, 2, 2, 2, 3 ),
 ( 0.2500000000000000000, 0.2512820512820512775, 0.2538461538461538325, 0.2564102564102563875, 0.2589743589743589980, 0.2615384615384615530, 0.2628205128205128305 ),
 .UNSPECIFIED. ) 
 CURVE ( )  GEOMETRIC_REPRESENTATION_ITEM ( )  RATIONAL_B_SPLINE_CURVE ( ( 0.9755282581475768211, 0.9755282581475768211, 1.000000000000000000, 0.9510565162951535312, 1.000000000000000000, 0.9510565162951535312, 1.000000000000000000, 0.9510565162951535312, 1.000000000000000000, 0.9510565162951535312, 1.000000000000000000, 0.9755282581475768211, 0.9755282581475768211 ) ) 
 REPRESENTATION_ITEM ( '' )  );
#26724=CARTESIAN_POINT ( 'NONE',  ( -33.58253175000000113, 43.02500000273118275, -10.91162601494193218 ) ) ;
#26727=CARTESIAN_POINT ( 'NONE',  ( -27.16883889988624290, 37.17500000273118843, -19.73931689729374028 ) ) ;
#26728=CARTESIAN_POINT ( 'NONE',  ( 3.880418787951134707, 17.55125428154684641, 24.50000000000000000 ) ) ;
#26729=AXIS2_PLACEMENT_3D ( 'NONE', #1905, #23026, #4146 ) ;
#26732=EDGE_CURVE ( 'NONE', #601, #12338, #25109, .T. ) ;
#26736=CARTESIAN_POINT ( 'NONE',  ( -7.236395654485757944, 5.224999997268803043, -22.27133577429736988 ) ) ;
#26737=CARTESIAN_POINT ( 'NONE',  ( -32.50000000000000000, 52.50000000546236834, 0.000000000000000000 ) ) ;
#26740=CARTESIAN_POINT ( 'NONE',  ( -27.16883889988623935, 17.32500000273118346, 19.73931689729374739 ) ) ;
#26744=ORIENTED_EDGE ( 'NONE', *, *, #33, .T. ) ;
#26749=CARTESIAN_POINT ( 'NONE',  ( 6.486482029760649416E-15, 27.87500000273120193, 35.31076352940723240 ) ) ;
#26751=CARTESIAN_POINT ( 'NONE',  ( 10.04305231718579705, 31.10000000546236976, 30.90933677959248982 ) ) ;
#26753=CARTESIAN_POINT ( 'NONE',  ( -5.147494310547430452, 54.05125428700922185, -32.49999999999999289 ) ) ;
#26754=CARTESIAN_POINT ( 'NONE',  ( 32.50000000000000000, 37.60000000546235555, -10.55989012756945833 ) ) ;
#26755=CARTESIAN_POINT ( 'NONE',  ( 33.58253175000000113, 42.37500000273119838, -4.112674001490185761E-15 ) ) ;
#26758=CARTESIAN_POINT ( 'NONE',  ( 32.50000000000000000, 23.09999999999999787, -10.55989012756945833 ) ) ;
#26760=CARTESIAN_POINT ( 'NONE',  ( -33.58253175000000113, 61.12500000273119127, 0.000000000000000000 ) ) ;
#26762=CARTESIAN_POINT ( 'NONE',  ( -20.75514604977248823, 55.07500000273117990, -28.56700777964554305 ) ) ;
#26766=CARTESIAN_POINT ( 'NONE',  ( 33.58253175000000113, 8.125000002731198379, -4.112674001490185761E-15 ) ) ;
#26772=CARTESIAN_POINT ( 'NONE',  ( -20.08610463437157989, 18.20000000546239605, -27.64615127144129758 ) ) ;
#26774=EDGE_CURVE ( 'NONE', #33755, #28845, #19869, .T. ) ;
#26775=CARTESIAN_POINT ( 'NONE',  ( 15.14183272437242067, 13.70000000000000462, 20.84094480462498211 ) ) ;
#26778=CARTESIAN_POINT ( 'NONE',  ( 26.29305231718578995, 49.19999999999999574, -19.10302069950538240 ) ) ;
#26780=CARTESIAN_POINT ( 'NONE',  ( -10.04305231718579172, 68.10000000546237686, -30.90933677959248982 ) ) ;
#26787=CARTESIAN_POINT ( 'NONE',  ( 5.779280353836490358E-15, 74.50000000000001421, 32.49999999999999289 ) ) ;
#26788=CARTESIAN_POINT ( 'NONE',  ( -33.58253175000000113, 49.47500000273118559, 10.91162601494193929 ) ) ;
#26789=CARTESIAN_POINT ( 'NONE',  ( 10.04305231718579705, 51.10000000546238397, 30.90933677959248982 ) ) ;
#26791=CARTESIAN_POINT ( 'NONE',  ( -10.37757302488624411, 36.72500000273118559, -31.93888565452638417 ) ) ;
#26792=CARTESIAN_POINT ( 'NONE',  ( 0.000000000000000000, 70.00000000000000000, 24.50000000000000000 ) ) ;
#26793=CARTESIAN_POINT ( 'NONE',  ( 10.37757302488624767, 61.97500000273120691, 31.93888565452638417 ) ) ;
#26796=CARTESIAN_POINT ( 'NONE',  ( 6.277390505771533514E-15, 38.50000000000000711, 34.17252228774368916 ) ) ;
#26798=CARTESIAN_POINT ( 'NONE',  ( -33.58253175000000113, 7.375000002731169069, 0.000000000000000000 ) ) ;
#26800=CARTESIAN_POINT ( 'NONE',  ( -8.601468415847515203, 71.67500000273116711, 11.83890561707634959 ) ) ;
#26801=CARTESIAN_POINT ( 'NONE',  ( -20.75514604977248823, 71.07500000273117280, -28.56700777964554305 ) ) ;
#26802=CARTESIAN_POINT ( 'NONE',  ( 6.001560367445586717E-15, 3.249999994537631665, 24.50000000000000000 ) ) ;
#26804=EDGE_LOOP ( 'NONE', ( #22186, #13794, #3981, #12080 ) ) ;
#26807=CARTESIAN_POINT ( 'NONE',  ( -1.778240108872766143E-15, 25.50000000000000711, -32.49999999999999289 ) ) ;
#26816=CARTESIAN_POINT ( 'NONE',  ( -27.16883889988624290, 38.92500000273118843, -19.73931689729374028 ) ) ;
#26819=CARTESIAN_POINT ( 'NONE',  ( 32.50000000000000000, 13.60000000546239107, -10.55989012756945833 ) ) ;
#26820=ORIENTED_EDGE ( 'NONE', *, *, #28712, .T. ) ;
#26822=CARTESIAN_POINT ( 'NONE',  ( 5.147494310547434893, 50.55125428154684641, 32.49999999999999289 ) ) ;
#26824=CARTESIAN_POINT ( 'NONE',  ( -20.75514604977248112, 67.67500000273116711, 28.56700777964554661 ) ) ;
#26828=EDGE_LOOP ( 'NONE', ( #24451, #19110, #24864, #1542 ) ) ;
#26830=CARTESIAN_POINT ( 'NONE',  ( 33.58253175000000113, 54.22500000273117848, -10.91162601494193751 ) ) ;
#26832=CARTESIAN_POINT ( 'NONE',  ( 20.08610463437158344, 15.20000000546237118, 27.64615127144129403 ) ) ;
#26833=CARTESIAN_POINT ( 'NONE',  ( -4.223320258572819786E-15, 11.24999999453763344, 24.50000000000000000 ) ) ;
#26834=CARTESIAN_POINT ( 'NONE',  ( 18.94512977948575738, 10.92499999726881299, 13.76444248337723408 ) ) ;
#26835=CARTESIAN_POINT ( 'NONE',  ( 6.486482029760649416E-15, 23.87500000273117706, 35.31076352940723240 ) ) ;
#26839=CARTESIAN_POINT ( 'NONE',  ( 26.29305231718579350, 14.79999999999997939, 19.10302069950537529 ) ) ;
#26843=CARTESIAN_POINT ( 'NONE',  ( 11.25946833292375793, 77.67500000273119554, 8.180482586598731842 ) ) ;
#26845=CARTESIAN_POINT ( 'NONE',  ( -27.16883889988623935, 23.32500000273118701, 19.73931689729374739 ) ) ;
#26849=CARTESIAN_POINT ( 'NONE',  ( -33.58253175000000113, 17.27500000273118630, -10.91162601494193041 ) ) ;
#26851=CARTESIAN_POINT ( 'NONE',  ( -10.37757302488624411, 68.72500000273117848, -31.93888565452638417 ) ) ;
#26852=DIRECTION ( 'NONE',  ( -0.000000000000000000, 1.000000000000000000, -0.000000000000000000 ) ) ;
#26853=EDGE_CURVE ( 'NONE', #7955, #18361, #21424, .T. ) ;
#26854=CARTESIAN_POINT ( 'NONE',  ( -8.601468415847515203, 79.67500000273118133, 11.83890561707634959 ) ) ;
#26857=CARTESIAN_POINT ( 'NONE',  ( 6.486482029760648627E-15, 57.62500000273119127, 35.31076352940722529 ) ) ;
#26858=EDGE_CURVE ( 'NONE', #774, #390, #24903, .T. ) ;
#26860=ORIENTED_EDGE ( 'NONE', *, *, #8724, .F. ) ;
#26862=CARTESIAN_POINT ( 'NONE',  ( -33.58253175000000113, 1.125000002731191273, 0.000000000000000000 ) ) ;
#26863=CARTESIAN_POINT ( 'NONE',  ( -7.236395654485757944, 9.224999997268806595, -22.27133577429736988 ) ) ;
#26867=CARTESIAN_POINT ( 'NONE',  ( -26.29305231718578995, 42.70000000546237118, 19.10302069950538595 ) ) ;
#26868=ORIENTED_EDGE ( 'NONE', *, *, #11730, .F. ) ;
#26871=CARTESIAN_POINT ( 'NONE',  ( -7.570916362186215665, 3.400000000000014122, 23.30088464923126423 ) ) ;
#26872=CARTESIAN_POINT ( 'NONE',  ( 33.58253175000000823, 76.02500000273118985, 10.91162601494192863 ) ) ;
#26874=CARTESIAN_POINT ( 'NONE',  ( -24.50000000000001066, 9.100000000000004974, 7.960532557706201828 ) ) ;
#26875=CARTESIAN_POINT ( 'NONE',  ( 6.486482029760649416E-15, 9.875000002731187720, 35.31076352940723240 ) ) ;
#26876=CARTESIAN_POINT ( 'NONE',  ( -2.162160676586881955E-15, 16.62500000273120548, -35.31076352940723240 ) ) ;
#26877=CARTESIAN_POINT ( 'NONE',  ( 8.601468415847520532, 79.57500000273120122, 11.83890561707634603 ) ) ;
#26880=CARTESIAN_POINT ( 'NONE',  ( 2.897257156509938333E-15, 80.50000000000000000, 15.77193336357400710 ) ) ;
#26883=CARTESIAN_POINT ( 'NONE',  ( 26.29305231718579350, 70.79999999999999716, 19.10302069950537529 ) ) ;
#26885=CARTESIAN_POINT ( 'NONE',  ( -33.58253175000000113, 47.02500000273116854, -10.91162601494193218 ) ) ;
#26888=CARTESIAN_POINT ( 'NONE',  ( 27.16883889988623935, 32.57500000273119412, -19.73931689729374384 ) ) ;
#26894=CARTESIAN_POINT ( 'NONE',  ( 18.94512977948576093, 4.824999997268819563, -13.76444248337722875 ) ) ;
#26897=CARTESIAN_POINT ( 'NONE',  ( -4.635254915624211769, 75.85000000546237686, -14.26584774442730286 ) ) ;
#26898=CARTESIAN_POINT ( 'NONE',  ( -2.162160676586882350E-15, 18.62500000273117351, -35.31076352940722529 ) ) ;
#26899=CARTESIAN_POINT ( 'NONE',  ( -7.236395654485763274, 8.524999997268800200, 22.27133577429736633 ) ) ;
#26901=VERTEX_POINT ( 'NONE', #14334 ) ;
#26903=EDGE_LOOP ( 'NONE', ( #22033, #9987, #18823, #33179 ) ) ;
#26906=CARTESIAN_POINT ( 'NONE',  ( -5.147494310547640062, 10.44874571845314293, 32.49999999999992895 ) ) ;
#26907=CARTESIAN_POINT ( 'NONE',  ( 7.236395654485760609, 3.024999997268823293, -22.27133577429736633 ) ) ;
#26908=CARTESIAN_POINT ( 'NONE',  ( 10.37757302488624767, 29.97500000273117848, 31.93888565452638417 ) ) ;
#26909=CARTESIAN_POINT ( 'NONE',  ( -32.50000000000000000, 32.60000000546237686, 10.55989012756946366 ) ) ;
#26910=( BOUNDED_CURVE ( )  B_SPLINE_CURVE ( 2, ( #17661, #17154, #9406, #22630, #27613, #4268, #19723, #30169, #22300, #7352, #27955, #25378, #1858 ),
 .UNSPECIFIED., .F., .T. ) 
 B_SPLINE_CURVE_WITH_KNOTS ( ( 3, 2, 2, 2, 2, 2, 3 ),
 ( 0.5705128205128204844, 0.5717948717948717618, 0.5743589743589743168, 0.5769230769230768718, 0.5794871794871795379, 0.5820512820512820928, 0.5833333333333333703 ),
 .UNSPECIFIED. ) 
 CURVE ( )  GEOMETRIC_REPRESENTATION_ITEM ( )  RATIONAL_B_SPLINE_CURVE ( ( 0.9755282581475768211, 0.9755282581475768211, 1.000000000000000000, 0.9510565162951535312, 1.000000000000000000, 0.9510565162951535312, 1.000000000000000000, 0.9510565162951535312, 1.000000000000000000, 0.9510565162951535312, 1.000000000000000000, 0.9755282581475768211, 0.9755282581475768211 ) ) 
 REPRESENTATION_ITEM ( '' )  );
#26911=CARTESIAN_POINT ( 'NONE',  ( -10.04305231718579172, 77.60000000000000853, -30.90933677959248982 ) ) ;
#26912=CARTESIAN_POINT ( 'NONE',  ( 5.779280353836490358E-15, 55.00000000546238965, 32.49999999999999289 ) ) ;
#26913=CARTESIAN_POINT ( 'NONE',  ( 32.50000000000000711, 37.40000000546236691, 10.55989012756945122 ) ) ;
#26914=CARTESIAN_POINT ( 'NONE',  ( -20.75514604977248823, 41.07500000273119412, -28.56700777964554305 ) ) ;
#26917=CARTESIAN_POINT ( 'NONE',  ( -26.29305231718578995, 24.19999999999999929, 19.10302069950538595 ) ) ;
#26918=VECTOR ( 'NONE', #20112, 1000.000000000000000 ) ;
#26920=CARTESIAN_POINT ( 'NONE',  ( -27.16883889988623935, 65.32500000273117280, 19.73931689729374739 ) ) ;
#26921=CARTESIAN_POINT ( 'NONE',  ( 33.58253175000000113, 56.37500000273118417, -4.112674001490185761E-15 ) ) ;
#26924=CARTESIAN_POINT ( 'NONE',  ( -27.16883889988623935, 7.325000002731174575, 19.73931689729374739 ) ) ;
#26928=VECTOR ( 'NONE', #7595, 1000.000000000000000 ) ;
#26931=CARTESIAN_POINT ( 'NONE',  ( -32.50000000000000000, 30.40000000546238823, -10.55989012756945300 ) ) ;
#26934=CARTESIAN_POINT ( 'NONE',  ( -8.446640517145639571E-15, 78.49999999999998579, 32.49999999999999289 ) ) ;
#26937=ORIENTED_EDGE ( 'NONE', *, *, #6314, .F. ) ;
#26941=ORIENTED_EDGE ( 'NONE', *, *, #3988, .F. ) ;
#26946=CARTESIAN_POINT ( 'NONE',  ( 10.37757302488624767, 49.97500000273119269, 31.93888565452638417 ) ) ;
#26947=CARTESIAN_POINT ( 'NONE',  ( -26.29305231718578995, 48.70000000546237118, 19.10302069950538595 ) ) ;
#26949=CARTESIAN_POINT ( 'NONE',  ( 20.75514604977249178, 37.82500000273117280, 28.56700777964553950 ) ) ;
#26951=VECTOR ( 'NONE', #15714, 1000.000000000000000 ) ;
#26952=CARTESIAN_POINT ( 'NONE',  ( 33.58253175000000823, 60.27500000273116143, 10.91162601494192863 ) ) ;
#26953=CARTESIAN_POINT ( 'NONE',  ( 6.277390505771533514E-15, 40.50000000000000711, 34.17252228774368916 ) ) ;
#26955=CARTESIAN_POINT ( 'NONE',  ( -20.75514604977248112, 3.675000002731179549, 28.56700777964554661 ) ) ;
#26956=CARTESIAN_POINT ( 'NONE',  ( 20.08610463437158344, 12.70000000000000639, 27.64615127144129403 ) ) ;
#26957=CARTESIAN_POINT ( 'NONE',  ( 4.300734207923761154, 71.97500000273119269, 13.23629886949340495 ) ) ;
#26958=CARTESIAN_POINT ( 'NONE',  ( 33.58253175000000823, 72.27500000273118985, 10.91162601494192685 ) ) ;
#26959=DIRECTION ( 'NONE',  ( -0.000000000000000000, -1.000000000000000000, -0.000000000000000000 ) ) ;
#26962=CARTESIAN_POINT ( 'NONE',  ( 7.570916362186213000, 2.149999994537632464, -23.30088464923126423 ) ) ;
#26976=EDGE_CURVE ( 'NONE', #28845, #24251, #9512, .T. ) ;
#26977=CARTESIAN_POINT ( 'NONE',  ( 2.067204126564591252E-14, 4.249999994537631665, -24.50000000000000000 ) ) ;
#26978=EDGE_LOOP ( 'NONE', ( #28554, #13662, #27982, #2162 ) ) ;
#26982=CARTESIAN_POINT ( 'NONE',  ( 27.16883889988624290, 70.17500000273119554, 19.73931689729373673 ) ) ;
#26983=ORIENTED_EDGE ( 'NONE', *, *, #27320, .F. ) ;
#26987=VERTEX_POINT ( 'NONE', #28051 ) ;
#26988=ORIENTED_EDGE ( 'NONE', *, *, #32828, .T. ) ;
#26990=CARTESIAN_POINT ( 'NONE',  ( 20.75514604977248467, 54.42500000273117422, -28.56700777964554305 ) ) ;
#26992=CARTESIAN_POINT ( 'NONE',  ( 26.29305231718579350, 9.300000005462383257, 19.10302069950537529 ) ) ;
#26995=CARTESIAN_POINT ( 'NONE',  ( -23.41746824999999887, 8.024999997268800200, -7.608796670333730638 ) ) ;
#26996=CARTESIAN_POINT ( 'NONE',  ( -20.75514604977248112, 21.67500000273119554, 28.56700777964554661 ) ) ;
#26999=CARTESIAN_POINT ( 'NONE',  ( -11.25946833292375793, 78.67500000273119554, -8.180482586598733619 ) ) ;
#27002=ORIENTED_EDGE ( 'NONE', *, *, #29131, .F. ) ;
#27004=CARTESIAN_POINT ( 'NONE',  ( -11.25946833292375793, 76.67500000273119554, -8.180482586598733619 ) ) ;
#27006=( BOUNDED_CURVE ( )  B_SPLINE_CURVE ( 2, ( #32889, #9388, #30665, #22788, #30325, #6821, #17303, #14726, #1838, #12318, #33241, #9739, #20225 ),
 .UNSPECIFIED., .F., .T. ) 
 B_SPLINE_CURVE_WITH_KNOTS ( ( 3, 2, 2, 2, 2, 2, 3 ),
 ( 0.8782051282051281937, 0.8794871794871794712, 0.8820512820512820262, 0.8846153846153845812, 0.8871794871794871362, 0.8897435897435896912, 0.8910256410256410797 ),
 .UNSPECIFIED. ) 
 CURVE ( )  GEOMETRIC_REPRESENTATION_ITEM ( )  RATIONAL_B_SPLINE_CURVE ( ( 0.9755282581475768211, 0.9755282581475768211, 1.000000000000000000, 0.9510565162951535312, 1.000000000000000000, 0.9510565162951535312, 1.000000000000000000, 0.9510565162951535312, 1.000000000000000000, 0.9510565162951535312, 1.000000000000000000, 0.9755282581475757109, 0.9755282581475768211 ) ) 
 REPRESENTATION_ITEM ( '' )  );
#27007=CARTESIAN_POINT ( 'NONE',  ( 27.16883889988624290, 25.92500000273118133, 19.73931689729373673 ) ) ;
#27011=CARTESIAN_POINT ( 'NONE',  ( -20.75514604977248823, 7.075000002731187898, -28.56700777964554305 ) ) ;
#27013=CARTESIAN_POINT ( 'NONE',  ( 27.16883889988624290, 71.92500000273119554, 19.73931689729373673 ) ) ;
#27016=CARTESIAN_POINT ( 'NONE',  ( -8.601468415847515203, 75.67500000273119554, 11.83890561707634959 ) ) ;
#27019=CARTESIAN_POINT ( 'NONE',  ( -9.270509831248419985, 72.55000000546236549, 12.75976212528060039 ) ) ;
#27020=CARTESIAN_POINT ( 'NONE',  ( -20.75514604977248112, 57.42500000273119554, 28.56700777964554661 ) ) ;
#27021=VECTOR ( 'NONE', #25821, 1000.000000000000000 ) ;
#27023=VERTEX_POINT ( 'NONE', #9331 ) ;
#27025=CARTESIAN_POINT ( 'NONE',  ( -2.162160676586882350E-15, 2.625000002731183280, -35.31076352940722529 ) ) ;
#27026=CARTESIAN_POINT ( 'NONE',  ( 18.94512977948575738, 4.424999997268807661, 13.76444248337723408 ) ) ;
#27030=CARTESIAN_POINT ( 'NONE',  ( -1.778240108872766143E-15, 68.00000000546238255, -32.49999999999999289 ) ) ;
#27031=VERTEX_POINT ( 'NONE', #11920 ) ;
#27033=CARTESIAN_POINT ( 'NONE',  ( 27.16883889988623935, 62.57500000273119412, -19.73931689729374384 ) ) ;
#27034=CARTESIAN_POINT ( 'NONE',  ( -1.778240108872766143E-15, 70.00000000546238255, -32.49999999999999289 ) ) ;
#27035=CARTESIAN_POINT ( 'NONE',  ( -27.16883889988623935, 71.32500000273117280, 19.73931689729374739 ) ) ;
#27037=CARTESIAN_POINT ( 'NONE',  ( -19.82091636218621389, 5.200000000000009948, 14.40073868116558842 ) ) ;
#27038=CARTESIAN_POINT ( 'NONE',  ( 20.75514604977249178, 8.075000002731185234, 28.56700777964553950 ) ) ;
#27040=CARTESIAN_POINT ( 'NONE',  ( -20.75514604977248112, 17.42500000273117777, 28.56700777964554661 ) ) ;
#27041=CARTESIAN_POINT ( 'NONE',  ( 11.25946833292375793, 80.07500000273121543, -8.180482586598735395 ) ) ;
#27044=CARTESIAN_POINT ( 'NONE',  ( -12.13525491562421088, 79.80000000000001137, -8.816778784387096835 ) ) ;
#27048=CARTESIAN_POINT ( 'NONE',  ( -10.04305231718579172, 38.10000000546237686, -30.90933677959248982 ) ) ;
#27050=CARTESIAN_POINT ( 'NONE',  ( 6.486482029760649416E-15, 43.62500000273116285, 35.31076352940723240 ) ) ;
#27053=CARTESIAN_POINT ( 'NONE',  ( 33.58253175000000113, 28.47500000273117848, -10.91162601494193574 ) ) ;
#27054=CARTESIAN_POINT ( 'NONE',  ( -4.223320258572819786E-15, 17.50000000000000000, 24.50000000000000000 ) ) ;
#27057=CARTESIAN_POINT ( 'NONE',  ( -15.00000000000000000, 76.00000000000001421, 0.000000000000000000 ) ) ;
#27060=CARTESIAN_POINT ( 'NONE',  ( 23.41746824999999887, 6.524999997268818852, 7.608796670333735079 ) ) ;
#27061=CARTESIAN_POINT ( 'NONE',  ( -26.29305231718579350, 52.30000000546236549, -19.10302069950537884 ) ) ;
#27064=CARTESIAN_POINT ( 'NONE',  ( -33.58253175000000113, 19.22500000273118204, 10.91162601494193929 ) ) ;
#27065=CARTESIAN_POINT ( 'NONE',  ( 23.41746824999999887, 7.124999997268815832, 0.000000000000000000 ) ) ;
#27071=ORIENTED_EDGE ( 'NONE', *, *, #18882, .T. ) ;
#27074=CARTESIAN_POINT ( 'NONE',  ( 10.04305231718578817, 39.39999999999999147, -30.90933677959249337 ) ) ;
#27075=CARTESIAN_POINT ( 'NONE',  ( -4.732186688966233175E-15, 13.24999999453763166, 25.76082449383753925 ) ) ;
#27076=CARTESIAN_POINT ( 'NONE',  ( 14.47279130897151589, 8.324999997268818674, 19.92008829642072953 ) ) ;
#27077=CARTESIAN_POINT ( 'NONE',  ( 10.37757302488624767, 25.97500000273117493, 31.93888565452638417 ) ) ;
#27078=CARTESIAN_POINT ( 'NONE',  ( -10.04305231718578462, 30.90000000546239178, 30.90933677959249337 ) ) ;
#27080=CARTESIAN_POINT ( 'NONE',  ( -10.04305231718579172, 73.59999999999999432, -30.90933677959248982 ) ) ;
#27081=CARTESIAN_POINT ( 'NONE',  ( 10.04305231718578817, 53.40000000000000568, -30.90933677959249337 ) ) ;
#27082=CARTESIAN_POINT ( 'NONE',  ( 10.04305231718578817, 37.90000000546236691, -30.90933677959249337 ) ) ;
#27084=CARTESIAN_POINT ( 'NONE',  ( 20.75514604977248467, 44.67500000273118843, -28.56700777964554305 ) ) ;
#27085=ADVANCED_FACE ( 'NONE', ( #6939 ), #27883, .T. ) ;
#27086=CARTESIAN_POINT ( 'NONE',  ( 23.41746824999999887, 11.12499999726881938, 0.000000000000000000 ) ) ;
#27087=CARTESIAN_POINT ( 'NONE',  ( 32.50000000000000711, 20.90000000000000924, 10.55989012756945122 ) ) ;
#27090=CARTESIAN_POINT ( 'NONE',  ( -10.37757302488624411, 60.72500000273117848, -31.93888565452638417 ) ) ;
#27091=CARTESIAN_POINT ( 'NONE',  ( -27.16883889988623935, 51.57500000273118701, 19.73931689729374739 ) ) ;
#27093=CARTESIAN_POINT ( 'NONE',  ( 2.067204126564591252E-14, 4.249999994537631665, -24.50000000000000000 ) ) ;
#27094=CARTESIAN_POINT ( 'NONE',  ( -10.37757302488623701, 3.525000002731204507, 31.93888565452638417 ) ) ;
#27101=CARTESIAN_POINT ( 'NONE',  ( -26.29305231718579350, 58.30000000546237260, -19.10302069950537884 ) ) ;
#27102=CARTESIAN_POINT ( 'NONE',  ( 7.570916362186213000, 14.39999999999999680, -23.30088464923126423 ) ) ;
#27108=VERTEX_POINT ( 'NONE', #33363 ) ;
#27112=( BOUNDED_CURVE ( )  B_SPLINE_CURVE ( 2, ( #762, #13986, #26526, #27019, #3515, #31662, #24448, #18978, #5757, #21720, #21549, #31995, #3018 ),
 .UNSPECIFIED., .F., .T. ) 
 B_SPLINE_CURVE_WITH_KNOTS ( ( 3, 2, 2, 2, 2, 2, 3 ),
 ( 0.7500000000000000000, 0.7600000000000000089, 0.7800000000000000266, 0.8000000000000000444, 0.8199999999999999512, 0.8399999999999999689, 0.8499999999999999778 ),
 .UNSPECIFIED. ) 
 CURVE ( )  GEOMETRIC_REPRESENTATION_ITEM ( )  RATIONAL_B_SPLINE_CURVE ( ( 0.9755282581475768211, 0.9755282581475768211, 1.000000000000000000, 0.9510565162951535312, 1.000000000000000000, 0.9510565162951535312, 1.000000000000000000, 0.9510565162951535312, 1.000000000000000000, 0.9510565162951535312, 1.000000000000000000, 0.9755282581475768211, 0.9755282581475768211 ) ) 
 REPRESENTATION_ITEM ( '' )  );
#27118=CARTESIAN_POINT ( 'NONE',  ( -26.29305231718578995, 46.70000000546237118, 19.10302069950538595 ) ) ;
#27119=CARTESIAN_POINT ( 'NONE',  ( -33.58253175000000113, 45.27500000273116854, -10.91162601494193218 ) ) ;
#27120=CARTESIAN_POINT ( 'NONE',  ( 32.50000000000000000, 47.50000000546239676, -3.980102097228898626E-15 ) ) ;
#27122=CARTESIAN_POINT ( 'NONE',  ( -2.162160676586881955E-15, 36.62500000273119127, -35.31076352940723240 ) ) ;
#27124=CARTESIAN_POINT ( 'NONE',  ( 27.16883889988623935, 64.57500000273120122, -19.73931689729374384 ) ) ;
#27126=CARTESIAN_POINT ( 'NONE',  ( -26.29305231718579350, 37.79999999999999716, -19.10302069950537884 ) ) ;
#27128=CARTESIAN_POINT ( 'NONE',  ( 6.486482029760649416E-15, 1.875000002731177728, 35.31076352940723240 ) ) ;
#27129=DIRECTION ( 'NONE',  ( 0.000000000000000000, 0.000000000000000000, 1.000000000000000000 ) ) ;
#27130=CARTESIAN_POINT ( 'NONE',  ( 33.58253175000000113, 72.37500000273116996, -4.112674001490185761E-15 ) ) ;
#27131=CARTESIAN_POINT ( 'NONE',  ( -24.50000000000000000, 18.74999999453763522, -3.000384657911015469E-15 ) ) ;
#27133=ORIENTED_EDGE ( 'NONE', *, *, #5804, .T. ) ;
#27134=CARTESIAN_POINT ( 'NONE',  ( 7.570916362186207671, 5.349999994537613546, 23.30088464923126779 ) ) ;
#27137=CARTESIAN_POINT ( 'NONE',  ( 4.635254915624212657, 74.59999999999999432, 14.26584774442730286 ) ) ;
#27145=ADVANCED_FACE ( 'NONE', ( #9859 ), #30786, .F. ) ;
#27146=DIRECTION ( 'NONE',  ( 0.000000000000000000, 1.000000000000000000, 0.000000000000000000 ) ) ;
#27149=CARTESIAN_POINT ( 'NONE',  ( -24.50000000000000711, 17.10000000000001208, 7.960532557706201828 ) ) ;
#27150=ORIENTED_EDGE ( 'NONE', *, *, #21677, .F. ) ;
#27160=CARTESIAN_POINT ( 'NONE',  ( -33.58253175000000113, 53.12500000273118417, 0.000000000000000000 ) ) ;
#27162=CARTESIAN_POINT ( 'NONE',  ( 6.277390505771533514E-15, 13.00000000546238255, 34.17252228774368916 ) ) ;
#27163=CARTESIAN_POINT ( 'NONE',  ( -32.50000000000000000, 66.40000000546238823, -10.55989012756945300 ) ) ;
#27164=CARTESIAN_POINT ( 'NONE',  ( 18.94512977948575738, 12.92499999726881654, 13.76444248337723408 ) ) ;
#27165=CARTESIAN_POINT ( 'NONE',  ( 10.04305231718578817, 57.40000000000000568, -30.90933677959249337 ) ) ;
#27166=CARTESIAN_POINT ( 'NONE',  ( 10.37757302488624056, 22.77500000273119340, -31.93888565452638417 ) ) ;
#27167=LINE ( 'NONE', #6570, #10188 ) ;
#27169=CARTESIAN_POINT ( 'NONE',  ( -13.91746824999999532, 74.97500000273115006, 4.522059556121122093 ) ) ;
#27170=CARTESIAN_POINT ( 'NONE',  ( 0.000000000000000000, 80.00000000000001421, 0.000000000000000000 ) ) ;
#27171=CARTESIAN_POINT ( 'NONE',  ( -32.50000000000000000, 28.40000000546235981, -10.55989012756945300 ) ) ;
#27176=CARTESIAN_POINT ( 'NONE',  ( -11.25946833292375793, 75.07500000273120122, 8.180482586598737171 ) ) ;
#27178=CARTESIAN_POINT ( 'NONE',  ( -10.37757302488623701, 15.52500000273118808, 31.93888565452638417 ) ) ;
#27182=CARTESIAN_POINT ( 'NONE',  ( 33.58253175000000823, 6.275000002731184523, 10.91162601494192685 ) ) ;
#27184=EDGE_CURVE ( 'NONE', #33138, #21829, #6471, .T. ) ;
#27187=CARTESIAN_POINT ( 'NONE',  ( 8.601468415847516980, 74.67500000273118133, -11.83890561707634603 ) ) ;
#27190=CARTESIAN_POINT ( 'NONE',  ( -20.75514604977248823, 52.82500000273116569, -28.56700777964554305 ) ) ;
#27194=ORIENTED_EDGE ( 'NONE', *, *, #22056, .F. ) ;
#27196=CARTESIAN_POINT ( 'NONE',  ( 20.08610463437157279, 17.30000000000000782, -27.64615127144129758 ) ) ;
#27197=CARTESIAN_POINT ( 'NONE',  ( -18.94512977948576093, 7.824999997268822227, 13.76444248337722698 ) ) ;
#27202=ORIENTED_EDGE ( 'NONE', *, *, #33841, .F. ) ;
#27204=CARTESIAN_POINT ( 'NONE',  ( -33.58253175000000113, 63.47500000273117138, 10.91162601494193929 ) ) ;
#27206=CARTESIAN_POINT ( 'NONE',  ( -33.58253175000000113, 71.02500000273118985, -10.91162601494193218 ) ) ;
#27208=CARTESIAN_POINT ( 'NONE',  ( 7.570916362186213000, 6.399999999999988809, -23.30088464923126423 ) ) ;
#27209=CARTESIAN_POINT ( 'NONE',  ( 10.37757302488624767, 1.975000002731180926, 31.93888565452638417 ) ) ;
#27210=CARTESIAN_POINT ( 'NONE',  ( 33.58253175000000113, 18.12500000273117706, -4.112674001490185761E-15 ) ) ;
#27211=( BOUNDED_CURVE ( )  B_SPLINE_CURVE ( 2, ( #22995, #33454, #9256, #9953, #20428, #19741, #4118, #14592, #32925, #30531, #26251, #31055, #25906 ),
 .UNSPECIFIED., .F., .T. ) 
 B_SPLINE_CURVE_WITH_KNOTS ( ( 3, 2, 2, 2, 2, 2, 3 ),
 ( 0.5961538461538461453, 0.5974358974358974228, 0.5999999999999999778, 0.6025641025641025328, 0.6051282051282050878, 0.6076923076923076428, 0.6089743589743590313 ),
 .UNSPECIFIED. ) 
 CURVE ( )  GEOMETRIC_REPRESENTATION_ITEM ( )  RATIONAL_B_SPLINE_CURVE ( ( 0.9755282581475768211, 0.9755282581475768211, 1.000000000000000000, 0.9510565162951535312, 1.000000000000000000, 0.9510565162951535312, 1.000000000000000000, 0.9510565162951535312, 1.000000000000000000, 0.9510565162951535312, 1.000000000000000000, 0.9755282581475757109, 0.9755282581475768211 ) ) 
 REPRESENTATION_ITEM ( '' )  );
#27214=CARTESIAN_POINT ( 'NONE',  ( 4.635254915624209993, 77.39999999999999147, -14.26584774442730463 ) ) ;
#27217=CARTESIAN_POINT ( 'NONE',  ( 32.50000000000000711, 49.40000000546236691, 10.55989012756945122 ) ) ;
#27219=CARTESIAN_POINT ( 'NONE',  ( -10.37757302488624411, 34.72500000273118559, -31.93888565452638417 ) ) ;
#27222=CARTESIAN_POINT ( 'NONE',  ( -33.58253175000000113, 27.47500000273118204, 10.91162601494193929 ) ) ;
#27225=AXIS2_PLACEMENT_3D ( 'NONE', #15771, #28962, #2548 ) ;
#27226=CARTESIAN_POINT ( 'NONE',  ( 10.04305231718578817, 31.39999999999998437, -30.90933677959249337 ) ) ;
#27229=CARTESIAN_POINT ( 'NONE',  ( -18.94512977948575738, 7.424999997268811214, -13.76444248337723231 ) ) ;
#27234=CARTESIAN_POINT ( 'NONE',  ( -8.891200544363830713E-16, 75.75000000546236834, -15.00000000000000000 ) ) ;
#27235=CARTESIAN_POINT ( 'NONE',  ( -33.58253175000000113, 17.12500000273120548, 0.000000000000000000 ) ) ;
#27236=CARTESIAN_POINT ( 'NONE',  ( -23.41746825000000598, 6.224999997268827023, 7.608796670333726198 ) ) ;
#27238=ORIENTED_EDGE ( 'NONE', *, *, #15661, .F. ) ;
#27245=CARTESIAN_POINT ( 'NONE',  ( -19.82091636218621034, 18.54999999453762882, -14.40073868116559552 ) ) ;
#27246=CARTESIAN_POINT ( 'NONE',  ( 18.94512977948576093, 8.824999997268822227, -13.76444248337722875 ) ) ;
#27247=CARTESIAN_POINT ( 'NONE',  ( 20.75514604977249178, 20.07500000273118346, 28.56700777964553950 ) ) ;
#27248=CARTESIAN_POINT ( 'NONE',  ( -26.29305231718578995, 30.70000000546238539, 19.10302069950538595 ) ) ;
#27249=CARTESIAN_POINT ( 'NONE',  ( -26.29305231718578995, 74.19999999999998863, 19.10302069950538595 ) ) ;
#27250=CARTESIAN_POINT ( 'NONE',  ( -5.147494310547423346, 6.948745723915522809, 32.50000000000000000 ) ) ;
#27251=CARTESIAN_POINT ( 'NONE',  ( -8.891200544363830713E-16, 73.50000000000001421, -15.00000000000000000 ) ) ;
#27253=CARTESIAN_POINT ( 'NONE',  ( 27.16883889988624290, 38.17500000273118843, 19.73931689729373673 ) ) ;
#27255=AXIS2_PLACEMENT_3D ( 'NONE', #8752, #19736, #13915 ) ;
#27256=CARTESIAN_POINT ( 'NONE',  ( 7.236395654485755280, 8.724999997268806595, 22.27133577429736988 ) ) ;
#27257=CARTESIAN_POINT ( 'NONE',  ( 10.04305231718579705, 14.60000000000000142, 30.90933677959248982 ) ) ;
#27260=CARTESIAN_POINT ( 'NONE',  ( -27.16883889988623935, 63.32500000273119412, 19.73931689729374739 ) ) ;
#27261=CARTESIAN_POINT ( 'NONE',  ( -27.16883889988624290, 45.17500000273119554, -19.73931689729374028 ) ) ;
#27264=CARTESIAN_POINT ( 'NONE',  ( 27.16883889988623935, 8.325000002731176352, -19.73931689729374384 ) ) ;
#27270=FACE_OUTER_BOUND ( 'NONE', #7874, .T. ) ;
#27271=CARTESIAN_POINT ( 'NONE',  ( 32.50000000000000000, 1.600000005462365760, -10.55989012756945833 ) ) ;
#27277=EDGE_CURVE ( 'NONE', #17375, #4296, #9448, .T. ) ;
#27282=ORIENTED_EDGE ( 'NONE', *, *, #22716, .T. ) ;
#27286=CARTESIAN_POINT ( 'NONE',  ( -5.147494310547430452, 64.05125428700922896, -32.49999999999999289 ) ) ;
#27287=CARTESIAN_POINT ( 'NONE',  ( 27.16883889988624290, 50.17500000273117422, 19.73931689729373673 ) ) ;
#27288=CARTESIAN_POINT ( 'NONE',  ( 32.50000000000000000, 49.60000000546239818, -10.55989012756945833 ) ) ;
#27290=CARTESIAN_POINT ( 'NONE',  ( -33.58253175000000113, 31.02500000273118630, -10.91162601494193218 ) ) ;
#27292=CARTESIAN_POINT ( 'NONE',  ( -33.58253175000000113, 65.27500000273117564, -10.91162601494193218 ) ) ;
#27295=CARTESIAN_POINT ( 'NONE',  ( -32.50000000000000000, 34.00000000000000000, 0.000000000000000000 ) ) ;
#27297=CARTESIAN_POINT ( 'NONE',  ( 27.16883889988624290, 4.175000002731188431, 19.73931689729373673 ) ) ;
#27298=DIRECTION ( 'NONE',  ( -0.000000000000000000, -1.000000000000000000, -0.000000000000000000 ) ) ;
#27300=CARTESIAN_POINT ( 'NONE',  ( 10.37757302488624767, 67.97500000273117848, 31.93888565452638417 ) ) ;
#27301=CARTESIAN_POINT ( 'NONE',  ( 15.14183272437242422, 4.049999994537630599, -20.84094480462497856 ) ) ;
#27303=EDGE_LOOP ( 'NONE', ( #21277, #22895, #20596, #2606 ) ) ;
#27304=CARTESIAN_POINT ( 'NONE',  ( 15.14183272437241889, 5.449999994537614079, 20.84094480462498211 ) ) ;
#27305=CIRCLE ( 'NONE', #22927, 24.50000000000000000 ) ;
#27307=CARTESIAN_POINT ( 'NONE',  ( 2.375766604868043252, 75.44874571845315359, -14.99999999999999822 ) ) ;
#27317=( BOUNDED_CURVE ( )  B_SPLINE_CURVE ( 2, ( #28192, #9658, #33506, #17221, #20138, #25624, #30933, #28365, #12405, #22526, #22875, #20482, #33333 ),
 .UNSPECIFIED., .F., .T. ) 
 B_SPLINE_CURVE_WITH_KNOTS ( ( 3, 2, 2, 2, 2, 2, 3 ),
 ( 0.3141025641025640969, 0.3153846153846153744, 0.3179487179487179294, 0.3205128205128205399, 0.3230769230769230949, 0.3256410256410256499, 0.3269230769230769273 ),
 .UNSPECIFIED. ) 
 CURVE ( )  GEOMETRIC_REPRESENTATION_ITEM ( )  RATIONAL_B_SPLINE_CURVE ( ( 0.9755282581475768211, 0.9755282581475768211, 1.000000000000000000, 0.9510565162951535312, 1.000000000000000000, 0.9510565162951535312, 1.000000000000000000, 0.9510565162951535312, 1.000000000000000000, 0.9510565162951535312, 1.000000000000000000, 0.9755282581475768211, 0.9755282581475768211 ) ) 
 REPRESENTATION_ITEM ( '' )  );
#27319=CARTESIAN_POINT ( 'NONE',  ( 0.000000000000000000, 80.00000000000001421, 0.000000000000000000 ) ) ;
#27320=EDGE_CURVE ( 'NONE', #11374, #19067, #4881, .T. ) ;
#27323=VERTEX_POINT ( 'NONE', #28555 ) ;
#27331=CARTESIAN_POINT ( 'NONE',  ( 5.779280353836490358E-15, 75.00000000546236834, 32.49999999999999289 ) ) ;
#27332=CARTESIAN_POINT ( 'NONE',  ( -27.16883889988624290, 56.92500000273120975, -19.73931689729374028 ) ) ;
#27334=EDGE_CURVE ( 'NONE', #3193, #3734, #9774, .T. ) ;
#27335=CARTESIAN_POINT ( 'NONE',  ( 32.50000000000000000, 9.500000005462361230, -3.980102097228898626E-15 ) ) ;
#27337=CARTESIAN_POINT ( 'NONE',  ( 14.47279130897151767, 14.82499999726881690, 19.92008829642072953 ) ) ;
#27338=CARTESIAN_POINT ( 'NONE',  ( 26.29305231718579350, 56.80000000000001847, 19.10302069950537529 ) ) ;
#27339=CARTESIAN_POINT ( 'NONE',  ( -20.75514604977248112, 25.67500000273118488, 28.56700777964554661 ) ) ;
#27342=CARTESIAN_POINT ( 'NONE',  ( -13.91746824999999887, 76.87500000273116996, 0.000000000000000000 ) ) ;
#27343=CARTESIAN_POINT ( 'NONE',  ( -24.50000000000000000, 0.9000000000000005773, -7.960532557706207157 ) ) ;
#27344=CARTESIAN_POINT ( 'NONE',  ( -20.08610463437156923, 28.80000000546237970, 27.64615127144130113 ) ) ;
#27350=CARTESIAN_POINT ( 'NONE',  ( 10.37757302488624767, 15.72500000273119269, 31.93888565452638417 ) ) ;
#27354=CARTESIAN_POINT ( 'NONE',  ( -33.58253175000000113, 11.37500000273117351, 0.000000000000000000 ) ) ;
#27358=CARTESIAN_POINT ( 'NONE',  ( 13.91746824999999887, 74.37500000273116996, -1.704398294459741270E-15 ) ) ;
#27361=CARTESIAN_POINT ( 'NONE',  ( -20.75514604977248823, 48.82500000273117990, -28.56700777964554305 ) ) ;
#27363=VERTEX_POINT ( 'NONE', #17942 ) ;
#27365=CARTESIAN_POINT ( 'NONE',  ( -1.778240108872766143E-15, 17.50000000000000000, -32.49999999999999289 ) ) ;
#27366=CARTESIAN_POINT ( 'NONE',  ( 7.236395654485755280, 8.224999997268806595, 22.27133577429736988 ) ) ;
#27371=EDGE_LOOP ( 'NONE', ( #8478, #27835, #17624, #22183 ) ) ;
#27373=CARTESIAN_POINT ( 'NONE',  ( -10.37757302488624411, 60.97500000273120691, -31.93888565452638417 ) ) ;
#27374=CARTESIAN_POINT ( 'NONE',  ( 6.486482029760649416E-15, 75.62500000273121259, 35.31076352940723240 ) ) ;
#27376=CARTESIAN_POINT ( 'NONE',  ( -4.732186688966233175E-15, 7.499999999999995559, 25.76082449383753925 ) ) ;
#27377=CARTESIAN_POINT ( 'NONE',  ( -33.58253175000000113, 1.475000002731190474, 10.91162601494193929 ) ) ;
#27378=CARTESIAN_POINT ( 'NONE',  ( -33.58253175000000113, 17.22500000273118559, 10.91162601494193929 ) ) ;
#27379=CARTESIAN_POINT ( 'NONE',  ( 8.601468415847516980, 72.17500000273119554, -11.83890561707634603 ) ) ;
#27381=CARTESIAN_POINT ( 'NONE',  ( 4.635254915624209993, 81.40000000000000568, -14.26584774442730463 ) ) ;
#27383=CARTESIAN_POINT ( 'NONE',  ( -19.82091636218621389, 8.949999994537632730, 14.40073868116558842 ) ) ;
#27385=CYLINDRICAL_SURFACE ( 'NONE', #32406, 24.50000000000000000 ) ;
#27387=CARTESIAN_POINT ( 'NONE',  ( 27.16883889988624290, 37.92500000273118843, 19.73931689729373673 ) ) ;
#27390=CARTESIAN_POINT ( 'NONE',  ( -20.75514604977248112, 29.67500000273119909, 28.56700777964554661 ) ) ;
#27394=CARTESIAN_POINT ( 'NONE',  ( 32.50000000000000000, 79.10000000000000853, -10.55989012756945833 ) ) ;
#27396=CARTESIAN_POINT ( 'NONE',  ( 23.41746824999999887, 8.624999997268817609, 0.000000000000000000 ) ) ;
#27400=EDGE_CURVE ( 'NONE', #1133, #771, #1775, .T. ) ;
#27402=CARTESIAN_POINT ( 'NONE',  ( -10.37757302488624411, 10.72500000273118914, -31.93888565452638417 ) ) ;
#27403=CARTESIAN_POINT ( 'NONE',  ( 7.236395654485755280, 6.724999997268804819, 22.27133577429736988 ) ) ;
#27408=( BOUNDED_CURVE ( )  B_SPLINE_CURVE ( 2, ( #29617, #18686, #6120, #10948, #29295, #16603, #27057, #24486, #959, #6291, #16767, #16112, #29958 ),
 .UNSPECIFIED., .F., .T. ) 
 B_SPLINE_CURVE_WITH_KNOTS ( ( 3, 2, 2, 2, 2, 2, 3 ),
 ( 0.5500000000000000444, 0.5600000000000000533, 0.5799999999999999600, 0.5999999999999999778, 0.6199999999999999956, 0.6400000000000000133, 0.6500000000000000222 ),
 .UNSPECIFIED. ) 
 CURVE ( )  GEOMETRIC_REPRESENTATION_ITEM ( )  RATIONAL_B_SPLINE_CURVE ( ( 0.9755282581475768211, 0.9755282581475768211, 1.000000000000000000, 0.9510565162951535312, 1.000000000000000000, 0.9510565162951535312, 1.000000000000000000, 0.9510565162951535312, 1.000000000000000000, 0.9510565162951535312, 1.000000000000000000, 0.9755282581475768211, 0.9755282581475768211 ) ) 
 REPRESENTATION_ITEM ( '' )  );
#27409=ORIENTED_EDGE ( 'NONE', *, *, #33358, .F. ) ;
#27413=CARTESIAN_POINT ( 'NONE',  ( -19.82091636218621034, 14.54999999453762705, -14.40073868116559552 ) ) ;
#27414=CARTESIAN_POINT ( 'NONE',  ( -14.47279130897152122, 5.924999997268808549, 19.92008829642072243 ) ) ;
#27415=CARTESIAN_POINT ( 'NONE',  ( -33.58253175000000113, 19.27500000273117919, -10.91162601494193218 ) ) ;
#27416=CARTESIAN_POINT ( 'NONE',  ( 10.04305231718578817, 29.90000000546239178, -30.90933677959249337 ) ) ;
#27417=CARTESIAN_POINT ( 'NONE',  ( 32.50000000000000000, 73.09999999999996589, -10.55989012756945833 ) ) ;
#27420=CARTESIAN_POINT ( 'NONE',  ( -20.75514604977248112, 33.67500000273119554, 28.56700777964554661 ) ) ;
#27423=CARTESIAN_POINT ( 'NONE',  ( 14.47279130897151589, 10.82499999726880091, 19.92008829642072953 ) ) ;
#27424=CARTESIAN_POINT ( 'NONE',  ( 32.50000000000000000, 13.09999999999999432, -10.55989012756945833 ) ) ;
#27427=CARTESIAN_POINT ( 'NONE',  ( -2.162160676586881955E-15, 56.62500000273116996, -35.31076352940723240 ) ) ;
#27428=CARTESIAN_POINT ( 'NONE',  ( 27.16883889988623935, 44.57500000273117990, -19.73931689729374384 ) ) ;
#27430=CARTESIAN_POINT ( 'NONE',  ( 7.890940483122900408E-14, 10.49999999999999112, -24.50000000000000000 ) ) ;
#27433=DIRECTION ( 'NONE',  ( 0.000000000000000000, 0.000000000000000000, -1.000000000000000000 ) ) ;
#27434=CARTESIAN_POINT ( 'NONE',  ( 5.779280353836490358E-15, 42.49999999999999289, 32.49999999999999289 ) ) ;
#27436=CARTESIAN_POINT ( 'NONE',  ( 5.147494310547434893, 66.55125428154683220, 32.49999999999999289 ) ) ;
#27438=CARTESIAN_POINT ( 'NONE',  ( 10.04305231718579705, 1.100000005462370423, 30.90933677959248982 ) ) ;
#27441=( LENGTH_UNIT ( ) NAMED_UNIT ( * ) SI_UNIT ( .MILLI., .METRE. ) );
#27442=CARTESIAN_POINT ( 'NONE',  ( -2.162160676586882350E-15, 34.62500000273119127, -35.31076352940722529 ) ) ;
#27444=ORIENTED_EDGE ( 'NONE', *, *, #18568, .F. ) ;
#27448=FACE_OUTER_BOUND ( 'NONE', #14158, .T. ) ;
#27454=CARTESIAN_POINT ( 'NONE',  ( -27.16883889988624290, 43.17500000273119554, -19.73931689729374028 ) ) ;
#27455=CARTESIAN_POINT ( 'NONE',  ( -20.08610463437156923, 50.80000000546237970, 27.64615127144130113 ) ) ;
#27457=CARTESIAN_POINT ( 'NONE',  ( -33.58253175000000113, 29.12500000273118772, 0.000000000000000000 ) ) ;
#27458=CARTESIAN_POINT ( 'NONE',  ( 2.667360163309149608E-15, 78.00000000546238255, -32.50000000000000000 ) ) ;
#27459=CARTESIAN_POINT ( 'NONE',  ( -20.75514604977248112, 53.67500000273119554, 28.56700777964554661 ) ) ;
#27460=DIRECTION ( 'NONE',  ( 0.000000000000000000, 0.000000000000000000, 1.000000000000000000 ) ) ;
#27462=CARTESIAN_POINT ( 'NONE',  ( -32.50000000000000000, 34.10000000000000142, 10.55989012756946366 ) ) ;
#27465=CARTESIAN_POINT ( 'NONE',  ( -2.162160676586881955E-15, 78.62500000273115575, -35.31076352940723240 ) ) ;
#27466=CYLINDRICAL_SURFACE ( 'NONE', #9628, 32.50000000000000000 ) ;
#27469=CARTESIAN_POINT ( 'NONE',  ( -27.16883889988623935, 65.57500000273120122, 19.73931689729374739 ) ) ;
#27470=LINE ( 'NONE', #536, #18254 ) ;
#27471=EDGE_CURVE ( 'NONE', #27323, #12256, #8672, .T. ) ;
#27472=CARTESIAN_POINT ( 'NONE',  ( 3.980102097228898626E-15, 80.00000000000001421, 32.50000000000000000 ) ) ;
#27473=CARTESIAN_POINT ( 'NONE',  ( -24.50000000000000000, 2.749999994537621895, -3.000384657911015469E-15 ) ) ;
#27486=CARTESIAN_POINT ( 'NONE',  ( 32.50000000000000000, 59.09999999999999432, -10.55989012756945833 ) ) ;
#27487=ORIENTED_EDGE ( 'NONE', *, *, #5855, .T. ) ;
#27494=EDGE_LOOP ( 'NONE', ( #25937, #4877, #10794, #2477 ) ) ;
#27496=CARTESIAN_POINT ( 'NONE',  ( 7.890940483122900408E-14, 12.24999999453763166, -24.50000000000000000 ) ) ;
#27497=CARTESIAN_POINT ( 'NONE',  ( 33.58253175000000113, 48.22500000273119269, -10.91162601494193751 ) ) ;
#27499=CARTESIAN_POINT ( 'NONE',  ( 26.29305231718579350, 11.30000000546238503, 19.10302069950537529 ) ) ;
#27501=CARTESIAN_POINT ( 'NONE',  ( -18.94512977948576093, 14.32499999726882756, 13.76444248337722698 ) ) ;
#27502=CARTESIAN_POINT ( 'NONE',  ( -26.29305231718579350, 51.80000000000001137, -19.10302069950537884 ) ) ;
#27504=CARTESIAN_POINT ( 'NONE',  ( 27.16883889988624290, 24.17500000273117777, 19.73931689729373673 ) ) ;
#27507=CARTESIAN_POINT ( 'NONE',  ( 2.688165632520823219E-15, 77.37500000273118417, 14.63369212191046387 ) ) ;
#27510=( BOUNDED_CURVE ( )  B_SPLINE_CURVE ( 2, ( #14498, #25480, #12255, #33181, #14667, #1265, #19813, #30436, #24786, #9684, #19989, #22224, #28049 ),
 .UNSPECIFIED., .F., .T. ) 
 B_SPLINE_CURVE_WITH_KNOTS ( ( 3, 2, 2, 2, 2, 2, 3 ),
 ( 0.5576923076923077094, 0.5589743589743589869, 0.5615384615384615419, 0.5641025641025640969, 0.5666666666666666519, 0.5692307692307692069, 0.5705128205128204844 ),
 .UNSPECIFIED. ) 
 CURVE ( )  GEOMETRIC_REPRESENTATION_ITEM ( )  RATIONAL_B_SPLINE_CURVE ( ( 0.9755282581475768211, 0.9755282581475768211, 1.000000000000000000, 0.9510565162951535312, 1.000000000000000000, 0.9510565162951535312, 1.000000000000000000, 0.9510565162951535312, 1.000000000000000000, 0.9510565162951535312, 1.000000000000000000, 0.9755282581475768211, 0.9755282581475768211 ) ) 
 REPRESENTATION_ITEM ( '' )  );
#27516=( BOUNDED_CURVE ( )  B_SPLINE_CURVE ( 2, ( #11056, #897, #24420, #16043, #11379, #26498, #18952, #3162, #19277, #14128, #16376, #11216, #29719 ),
 .UNSPECIFIED., .F., .T. ) 
 B_SPLINE_CURVE_WITH_KNOTS ( ( 3, 2, 2, 2, 2, 2, 3 ),
 ( 0.1602564102564102699, 0.1615384615384615474, 0.1641025641025641024, 0.1666666666666666574, 0.1692307692307692402, 0.1717948717948717952, 0.1730769230769230727 ),
 .UNSPECIFIED. ) 
 CURVE ( )  GEOMETRIC_REPRESENTATION_ITEM ( )  RATIONAL_B_SPLINE_CURVE ( ( 0.9755282581475768211, 0.9755282581475770431, 1.000000000000000000, 0.9510565162951535312, 1.000000000000000000, 0.9510565162951535312, 1.000000000000000000, 0.9510565162951535312, 1.000000000000000000, 0.9510565162951535312, 1.000000000000000000, 0.9755282581475768211, 0.9755282581475768211 ) ) 
 REPRESENTATION_ITEM ( '' )  );
#27520=CARTESIAN_POINT ( 'NONE',  ( -10.37757302488623701, 9.775000002731182747, 31.93888565452638417 ) ) ;
#27523=CARTESIAN_POINT ( 'NONE',  ( 11.25946833292375793, 80.57500000273121543, -8.180482586598735395 ) ) ;
#27525=CARTESIAN_POINT ( 'NONE',  ( -10.37757302488624411, 54.72500000273117138, -31.93888565452638417 ) ) ;
#27530=AXIS2_PLACEMENT_3D ( 'NONE', #9753, #1510, #14910 ) ;
#27531=CARTESIAN_POINT ( 'NONE',  ( -14.47279130897151589, 11.32499999726881157, -19.92008829642072598 ) ) ;
#27535=AXIS2_PLACEMENT_3D ( 'NONE', #3366, #6098, #13836 ) ;
#27536=CARTESIAN_POINT ( 'NONE',  ( 1.555960095263670572E-15, 6.499999999999994671, -24.50000000000000000 ) ) ;
#27539=CARTESIAN_POINT ( 'NONE',  ( 20.75514604977249178, 62.07500000273118701, 28.56700777964553950 ) ) ;
#27540=CARTESIAN_POINT ( 'NONE',  ( 10.04305231718579705, 69.10000000546237686, 30.90933677959248982 ) ) ;
#27541=CARTESIAN_POINT ( 'NONE',  ( -10.37757302488624411, 64.72500000273117848, -31.93888565452638417 ) ) ;
#27543=CARTESIAN_POINT ( 'NONE',  ( -19.82091636218621034, 8.800000000000002487, -14.40073868116559552 ) ) ;
#27544=CARTESIAN_POINT ( 'NONE',  ( 6.486482029760649416E-15, 3.875000002731201931, 35.31076352940723240 ) ) ;
#27545=CARTESIAN_POINT ( 'NONE',  ( 20.75514604977249178, 13.82500000273117813, 28.56700777964553950 ) ) ;
#27546=CARTESIAN_POINT ( 'NONE',  ( -8.601468415847515203, 75.17500000273118133, 11.83890561707634959 ) ) ;
#27548=CARTESIAN_POINT ( 'NONE',  ( 15.00000000000000355, 80.89999999999997726, 4.873795443493592394 ) ) ;
#27550=CARTESIAN_POINT ( 'NONE',  ( -2.375766604868045029, 73.80125428700922896, -14.99999999999999822 ) ) ;
#27552=CARTESIAN_POINT ( 'NONE',  ( 12.13525491562420910, 75.45000000546237118, -8.816778784387098611 ) ) ;
#27554=CARTESIAN_POINT ( 'NONE',  ( 33.58253175000000823, 40.02500000273119696, 10.91162601494192863 ) ) ;
#27557=CARTESIAN_POINT ( 'NONE',  ( 10.37757302488624056, 30.77500000273120051, -31.93888565452638417 ) ) ;
#27558=CARTESIAN_POINT ( 'NONE',  ( 5.779280353836490358E-15, 40.49999999999999289, 32.49999999999999289 ) ) ;
#27564=CARTESIAN_POINT ( 'NONE',  ( -4.523095164977117273E-15, 8.124999997268826490, 24.62258325217400312 ) ) ;
#27569=CARTESIAN_POINT ( 'NONE',  ( 20.75514604977248467, 10.42500000273119909, -28.56700777964554305 ) ) ;
#27570=CARTESIAN_POINT ( 'NONE',  ( -14.47279130897152122, 14.42499999726880056, 19.92008829642072243 ) ) ;
#27572=VERTEX_POINT ( 'NONE', #23930 ) ;
#27578=CARTESIAN_POINT ( 'NONE',  ( -20.08610463437157989, 9.700000000000013500, -27.64615127144129758 ) ) ;
#27579=CARTESIAN_POINT ( 'NONE',  ( 7.570916362186213000, 18.14999999453761959, -23.30088464923126423 ) ) ;
#27580=CARTESIAN_POINT ( 'NONE',  ( 14.47279130897151767, 2.924999997268815655, -19.92008829642072598 ) ) ;
#27581=CARTESIAN_POINT ( 'NONE',  ( -20.75514604977248112, 23.67500000273118843, 28.56700777964554661 ) ) ;
#27582=CARTESIAN_POINT ( 'NONE',  ( 26.29305231718579350, 25.30000000546236905, 19.10302069950537529 ) ) ;
#27583=CARTESIAN_POINT ( 'NONE',  ( 26.29305231718578995, 73.19999999999998863, -19.10302069950538240 ) ) ;
#27584=DIRECTION ( 'NONE',  ( -0.000000000000000000, -1.000000000000000000, -0.000000000000000000 ) ) ;
#27587=CARTESIAN_POINT ( 'NONE',  ( -33.58253175000000113, 39.47500000273117848, 10.91162601494193929 ) ) ;
#27590=CARTESIAN_POINT ( 'NONE',  ( -18.94512977948575738, 9.924999997268812990, -13.76444248337723231 ) ) ;
#27591=CARTESIAN_POINT ( 'NONE',  ( -10.04305231718578462, 14.39999999999999680, 30.90933677959249337 ) ) ;
#27594=CARTESIAN_POINT ( 'NONE',  ( -33.58253175000000113, 55.22500000273117848, 10.91162601494193929 ) ) ;
#27595=CARTESIAN_POINT ( 'NONE',  ( -27.16883889988623935, 49.57500000273118701, 19.73931689729374739 ) ) ;
#27607=EDGE_CURVE ( 'NONE', #25303, #6411, #5563, .T. ) ;
#27608=CARTESIAN_POINT ( 'NONE',  ( 32.50000000000000000, 41.50000000546238965, -3.980102097228898626E-15 ) ) ;
#27609=ADVANCED_FACE ( 'NONE', ( #3651 ), #31802, .T. ) ;
#27612=( BOUNDED_CURVE ( )  B_SPLINE_CURVE ( 2, ( #31620, #23576, #385, #8118, #29044, #10870, #31786, #29213, #26651, #3146, #23238, #31119, #16360 ),
 .UNSPECIFIED., .F., .T. ) 
 B_SPLINE_CURVE_WITH_KNOTS ( ( 3, 2, 2, 2, 2, 2, 3 ),
 ( 0.2756410256410256610, 0.2769230769230769384, 0.2794871794871794934, 0.2820512820512820484, 0.2846153846153846034, 0.2871794871794871584, 0.2884615384615384914 ),
 .UNSPECIFIED. ) 
 CURVE ( )  GEOMETRIC_REPRESENTATION_ITEM ( )  RATIONAL_B_SPLINE_CURVE ( ( 0.9755282581475768211, 0.9755282581475768211, 1.000000000000000000, 0.9510565162951535312, 1.000000000000000000, 0.9510565162951535312, 1.000000000000000000, 0.9510565162951535312, 1.000000000000000000, 0.9510565162951535312, 1.000000000000000000, 0.9755282581475762660, 0.9755282581475768211 ) ) 
 REPRESENTATION_ITEM ( '' )  );
#27613=CARTESIAN_POINT ( 'NONE',  ( 26.29305231718578995, 35.20000000000000995, -19.10302069950538240 ) ) ;
#27614=CARTESIAN_POINT ( 'NONE',  ( 33.58253175000000823, 32.02500000273118985, 10.91162601494192685 ) ) ;
#27616=ORIENTED_EDGE ( 'NONE', *, *, #29497, .T. ) ;
#27617=EDGE_CURVE ( 'NONE', #12770, #22201, #27516, .T. ) ;
#27621=ORIENTED_EDGE ( 'NONE', *, *, #10902, .F. ) ;
#27626=CARTESIAN_POINT ( 'NONE',  ( 27.16883889988623935, 40.57500000273117280, -19.73931689729374384 ) ) ;
#27627=CARTESIAN_POINT ( 'NONE',  ( -20.08610463437157989, 44.20000000546238539, -27.64615127144129758 ) ) ;
#27629=CARTESIAN_POINT ( 'NONE',  ( 10.37757302488624767, 27.72500000273120335, 31.93888565452638417 ) ) ;
#27630=CARTESIAN_POINT ( 'NONE',  ( 1.555960095263670572E-15, 14.24999999453762278, -24.50000000000000000 ) ) ;
#27632=CARTESIAN_POINT ( 'NONE',  ( 6.486482029760649416E-15, 55.87500000273118417, 35.31076352940723240 ) ) ;
#27634=CARTESIAN_POINT ( 'NONE',  ( 32.50000000000000000, 37.00000000000000711, -3.980102097228898626E-15 ) ) ;
#27636=CARTESIAN_POINT ( 'NONE',  ( 33.58253175000000113, 78.12500000273119838, -4.112674001490185761E-15 ) ) ;
#27637=DIRECTION ( 'NONE',  ( 0.000000000000000000, 0.000000000000000000, -1.000000000000000000 ) ) ;
#27639=CARTESIAN_POINT ( 'NONE',  ( -20.75514604977248823, 69.07500000273117280, -28.56700777964554305 ) ) ;
#27643=CARTESIAN_POINT ( 'NONE',  ( -15.14183272437241889, 6.449999994537612302, -20.84094480462497856 ) ) ;
#27655=CARTESIAN_POINT ( 'NONE',  ( 5.779280353836490358E-15, 58.49999999999999289, 32.49999999999999289 ) ) ;
#27662=ORIENTED_EDGE ( 'NONE', *, *, #30013, .T. ) ;
#27665=CARTESIAN_POINT ( 'NONE',  ( 5.147494310547643614, 27.44874571845315714, -32.49999999999992895 ) ) ;
#27666=CARTESIAN_POINT ( 'NONE',  ( 33.58253175000000823, 50.02500000273118985, 10.91162601494192863 ) ) ;
#27667=CARTESIAN_POINT ( 'NONE',  ( 32.50000000000000000, 55.50000000546237544, -3.980102097228898626E-15 ) ) ;
#27669=CARTESIAN_POINT ( 'NONE',  ( -10.04305231718579172, 14.10000000546238219, -30.90933677959248982 ) ) ;
#27671=CARTESIAN_POINT ( 'NONE',  ( 14.47279130897151767, 16.82499999726881157, 19.92008829642072953 ) ) ;
#27673=CARTESIAN_POINT ( 'NONE',  ( 32.50000000000000711, 50.89999999999999858, 10.55989012756945122 ) ) ;
#27675=CARTESIAN_POINT ( 'NONE',  ( 27.16883889988624290, 14.17500000273119731, 19.73931689729373673 ) ) ;
#27678=CARTESIAN_POINT ( 'NONE',  ( -8.601468415847515203, 73.17500000273119554, 11.83890561707634959 ) ) ;
#27679=CARTESIAN_POINT ( 'NONE',  ( -4.223320258572819786E-15, 13.50000000000000355, 24.50000000000000000 ) ) ;
#27684=CARTESIAN_POINT ( 'NONE',  ( 11.25946833292375793, 72.07500000273120122, -8.180482586598735395 ) ) ;
#27689=CARTESIAN_POINT ( 'NONE',  ( -33.58253175000000113, 11.27500000273117209, -10.91162601494193041 ) ) ;
#27692=CARTESIAN_POINT ( 'NONE',  ( 13.91746824999999887, 72.37500000273119838, -1.704398294459741270E-15 ) ) ;
#27695=CARTESIAN_POINT ( 'NONE',  ( 6.486482029760648627E-15, 53.62500000273120548, 35.31076352940722529 ) ) ;
#27698=EDGE_LOOP ( 'NONE', ( #13956, #16127, #11783, #5844 ) ) ;
#27700=DIRECTION ( 'NONE',  ( -0.000000000000000000, -1.000000000000000000, -0.000000000000000000 ) ) ;
#27701=CARTESIAN_POINT ( 'NONE',  ( -7.236395654485757944, 13.22499999726881015, -22.27133577429736988 ) ) ;
#27706=FACE_OUTER_BOUND ( 'NONE', #24614, .T. ) ;
#27707=ORIENTED_EDGE ( 'NONE', *, *, #25513, .F. ) ;
#27709=CARTESIAN_POINT ( 'NONE',  ( -33.58253175000000113, 57.27500000273120406, -10.91162601494193218 ) ) ;
#27711=CARTESIAN_POINT ( 'NONE',  ( -27.16883889988624290, 68.92500000273119554, -19.73931689729374028 ) ) ;
#27714=CARTESIAN_POINT ( 'NONE',  ( -7.570916362186215665, 15.39999999999999680, 23.30088464923126423 ) ) ;
#27715=CARTESIAN_POINT ( 'NONE',  ( 10.37757302488624056, 2.775000002731176085, -31.93888565452638417 ) ) ;
#27716=CARTESIAN_POINT ( 'NONE',  ( 27.16883889988624290, 11.92500000273116711, 19.73931689729373673 ) ) ;
#27717=CARTESIAN_POINT ( 'NONE',  ( 13.91746824999999887, 71.87500000273119838, -1.704398294459741270E-15 ) ) ;
#27719=CARTESIAN_POINT ( 'NONE',  ( -12.13525491562421088, 75.80000000000001137, -8.816778784387096835 ) ) ;
#27722=CARTESIAN_POINT ( 'NONE',  ( 32.50000000000000000, 22.99999999999999289, -3.980102097228898626E-15 ) ) ;
#27724=CARTESIAN_POINT ( 'NONE',  ( 12.13525491562420910, 79.45000000546237118, -8.816778784387098611 ) ) ;
#27726=CARTESIAN_POINT ( 'NONE',  ( -33.58253175000000113, 39.22500000273119269, 10.91162601494193929 ) ) ;
#27729=CARTESIAN_POINT ( 'NONE',  ( 33.58253175000000113, 26.47500000273118559, -10.91162601494193574 ) ) ;
#27730=CARTESIAN_POINT ( 'NONE',  ( -3.880418787951136483, 16.30125427608446742, -24.50000000000000000 ) ) ;
#27732=CARTESIAN_POINT ( 'NONE',  ( 32.50000000000000711, 32.89999999999997726, 10.55989012756945122 ) ) ;
#27735=CARTESIAN_POINT ( 'NONE',  ( -18.94512977948576093, 7.824999997268822227, 13.76444248337722698 ) ) ;
#27738=CARTESIAN_POINT ( 'NONE',  ( 33.58253175000000113, 14.22500000273119447, -10.91162601494193574 ) ) ;
#27739=CARTESIAN_POINT ( 'NONE',  ( 1.507698388325705758E-15, 9.624999997268808727, -24.62258325217400312 ) ) ;
#27741=ORIENTED_EDGE ( 'NONE', *, *, #28451, .F. ) ;
#27745=EDGE_CURVE ( 'NONE', #15993, #18611, #23620, .T. ) ;
#27750=CARTESIAN_POINT ( 'NONE',  ( -24.50000000000000355, 14.64999999453761603, -7.960532557706207157 ) ) ;
#27751=CARTESIAN_POINT ( 'NONE',  ( -14.47279130897151589, 11.32499999726881157, -19.92008829642072598 ) ) ;
#27752=CARTESIAN_POINT ( 'NONE',  ( -10.37757302488623701, 21.77500000273119340, 31.93888565452638417 ) ) ;
#27753=CARTESIAN_POINT ( 'NONE',  ( -20.08610463437156923, 22.80000000546236194, 27.64615127144130113 ) ) ;
#27754=CARTESIAN_POINT ( 'NONE',  ( -26.29305231718579350, 69.79999999999999716, -19.10302069950537884 ) ) ;
#27755=CARTESIAN_POINT ( 'NONE',  ( 0.000000000000000000, 80.00000000000001421, 0.000000000000000000 ) ) ;
#27758=CARTESIAN_POINT ( 'NONE',  ( -33.58253175000000113, 35.37500000273119127, 0.000000000000000000 ) ) ;
#27763=CARTESIAN_POINT ( 'NONE',  ( -14.47279130897151589, 7.824999997268807128, -19.92008829642072598 ) ) ;
#27764=CARTESIAN_POINT ( 'NONE',  ( 20.08610463437158344, 16.69999999999999574, 27.64615127144129403 ) ) ;
#27768=CARTESIAN_POINT ( 'NONE',  ( 33.58253175000000113, 58.12500000273118417, -4.112674001490185761E-15 ) ) ;
#27769=CARTESIAN_POINT ( 'NONE',  ( -10.37757302488623701, 49.77500000273118985, 31.93888565452638417 ) ) ;
#27770=CARTESIAN_POINT ( 'NONE',  ( 20.08610463437157279, 45.29999999999999005, -27.64615127144129758 ) ) ;
#27775=CARTESIAN_POINT ( 'NONE',  ( 0.000000000000000000, 80.00000000000001421, 0.000000000000000000 ) ) ;
#27777=PLANE ( 'NONE',  #2350 ) ;
#27779=DIRECTION ( 'NONE',  ( -0.000000000000000000, -1.000000000000000000, -0.000000000000000000 ) ) ;
#27782=CARTESIAN_POINT ( 'NONE',  ( 4.635254915624209993, 71.65000000546240244, -14.26584774442730463 ) ) ;
#27783=CARTESIAN_POINT ( 'NONE',  ( 10.37757302488624767, 31.72500000273117848, 31.93888565452638417 ) ) ;
#27784=CARTESIAN_POINT ( 'NONE',  ( 27.16883889988624290, 64.17500000273118133, 19.73931689729373673 ) ) ;
#27786=ORIENTED_EDGE ( 'NONE', *, *, #1803, .F. ) ;
#27791=EDGE_LOOP ( 'NONE', ( #10247, #9638 ) ) ;
#27795=VECTOR ( 'NONE', #2734, 1000.000000000000000 ) ;
#27797=CARTESIAN_POINT ( 'NONE',  ( 10.04305231718578817, 21.40000000000000213, -30.90933677959249337 ) ) ;
#27798=CARTESIAN_POINT ( 'NONE',  ( 20.75514604977248467, 40.67500000273116711, -28.56700777964554305 ) ) ;
#27799=CARTESIAN_POINT ( 'NONE',  ( -26.29305231718578995, 46.70000000546237118, 19.10302069950538595 ) ) ;
#27801=CARTESIAN_POINT ( 'NONE',  ( 20.75514604977248467, 30.42500000273117777, -28.56700777964554305 ) ) ;
#27802=CARTESIAN_POINT ( 'NONE',  ( 24.50000000000000000, 13.84999999453764197, -7.960532557706203605 ) ) ;
#27803=CARTESIAN_POINT ( 'NONE',  ( 27.16883889988624290, 58.17500000273118133, 19.73931689729373673 ) ) ;
#27805=CARTESIAN_POINT ( 'NONE',  ( 32.50000000000000000, 35.00000000000000000, -3.980102097228898626E-15 ) ) ;
#27807=CARTESIAN_POINT ( 'NONE',  ( 33.58253175000000113, 74.22500000273119269, -10.91162601494193751 ) ) ;
#27808=LINE ( 'NONE', #22655, #3061 ) ;
#27810=CARTESIAN_POINT ( 'NONE',  ( 20.75514604977248467, 66.67500000273119554, -28.56700777964554305 ) ) ;
#27812=EDGE_CURVE ( 'NONE', #15526, #31469, #30815, .T. ) ;
#27814=CARTESIAN_POINT ( 'NONE',  ( 19.82091636218621389, 11.94999999453763628, -14.40073868116559197 ) ) ;
#27816=( BOUNDED_CURVE ( )  B_SPLINE_CURVE ( 2, ( #23657, #28285, #4772, #5458, #15939, #26395, #23135, #2888, #15600, #25877, #10274, #15250, #18006 ),
 .UNSPECIFIED., .F., .T. ) 
 B_SPLINE_CURVE_WITH_KNOTS ( ( 3, 2, 2, 2, 2, 2, 3 ),
 ( 0.3397435897435897578, 0.3410256410256410353, 0.3435897435897435903, 0.3461538461538461453, 0.3487179487179487003, 0.3512820512820512553, 0.3525641025641025883 ),
 .UNSPECIFIED. ) 
 CURVE ( )  GEOMETRIC_REPRESENTATION_ITEM ( )  RATIONAL_B_SPLINE_CURVE ( ( 0.9755282581475768211, 0.9755282581475768211, 1.000000000000000000, 0.9510565162951535312, 1.000000000000000000, 0.9510565162951535312, 1.000000000000000000, 0.9510565162951535312, 1.000000000000000000, 0.9510565162951535312, 1.000000000000000000, 0.9755282581475762660, 0.9755282581475768211 ) ) 
 REPRESENTATION_ITEM ( '' )  );
#27817=CARTESIAN_POINT ( 'NONE',  ( 0.000000000000000000, 70.00000000000000000, -30.50000000000000000 ) ) ;
#27828=CARTESIAN_POINT ( 'NONE',  ( -26.29305231718579350, 78.30000000546239391, -19.10302069950537884 ) ) ;
#27831=CARTESIAN_POINT ( 'NONE',  ( -32.50000000000000000, 76.00000000000001421, 0.000000000000000000 ) ) ;
#27832=ORIENTED_EDGE ( 'NONE', *, *, #26431, .T. ) ;
#27833=CARTESIAN_POINT ( 'NONE',  ( 33.58253175000000113, 72.37500000273116996, -4.112674001490185761E-15 ) ) ;
#27835=ORIENTED_EDGE ( 'NONE', *, *, #28647, .T. ) ;
#27837=CARTESIAN_POINT ( 'NONE',  ( 10.04305231718578817, 59.90000000546235981, -30.90933677959249337 ) ) ;
#27839=CARTESIAN_POINT ( 'NONE',  ( -26.29305231718579350, 55.80000000000001847, -19.10302069950537884 ) ) ;
#27840=CARTESIAN_POINT ( 'NONE',  ( -10.37757302488624411, 46.72500000273119269, -31.93888565452638417 ) ) ;
#27841=CARTESIAN_POINT ( 'NONE',  ( 26.29305231718579350, 55.30000000546236549, 19.10302069950537529 ) ) ;
#27844=CARTESIAN_POINT ( 'NONE',  ( 20.08610463437157279, 3.800000005462383257, -27.64615127144129758 ) ) ;
#27848=CARTESIAN_POINT ( 'NONE',  ( -26.29305231718578995, 52.19999999999999574, 19.10302069950538595 ) ) ;
#27850=CARTESIAN_POINT ( 'NONE',  ( -20.75514604977248823, 17.07500000273119056, -28.56700777964554305 ) ) ;
#27851=FACE_OUTER_BOUND ( 'NONE', #30, .T. ) ;
#27853=CARTESIAN_POINT ( 'NONE',  ( -4.300734207923755825, 73.27500000273118985, 13.23629886949340673 ) ) ;
#27864=CARTESIAN_POINT ( 'NONE',  ( -20.08610463437156923, 20.29999999999999716, 27.64615127144130113 ) ) ;
#27868=CARTESIAN_POINT ( 'NONE',  ( 0.000000000000000000, 80.00000000000001421, -32.50000000000000000 ) ) ;
#27870=CARTESIAN_POINT ( 'NONE',  ( -33.58253175000000113, 51.02500000273119696, -10.91162601494193041 ) ) ;
#27872=CARTESIAN_POINT ( 'NONE',  ( 32.50000000000000711, 21.40000000546237757, 10.55989012756945122 ) ) ;
#27875=CARTESIAN_POINT ( 'NONE',  ( 5.779280353836490358E-15, 4.500000000000003553, 32.49999999999999289 ) ) ;
#27876=CARTESIAN_POINT ( 'NONE',  ( -23.41746824999999887, 11.62499999726881938, -2.867812753649727150E-15 ) ) ;
#27880=CARTESIAN_POINT ( 'NONE',  ( 5.779280353836490358E-15, 56.49999999999998579, 32.49999999999999289 ) ) ;
#27883=CYLINDRICAL_SURFACE ( 'NONE', #15507, 32.50000000000000000 ) ;
#27884=CARTESIAN_POINT ( 'NONE',  ( -20.75514604977248112, 69.42500000273116711, 28.56700777964554661 ) ) ;
#27886=CARTESIAN_POINT ( 'NONE',  ( 24.50000000000000355, 10.10000000000000142, -7.960532557706203605 ) ) ;
#27887=CARTESIAN_POINT ( 'NONE',  ( -10.37757302488623701, 3.775000002731176973, 31.93888565452638417 ) ) ;
#27888=CARTESIAN_POINT ( 'NONE',  ( 6.486482029760649416E-15, 9.625000002731196602, 35.31076352940723240 ) ) ;
#27891=CARTESIAN_POINT ( 'NONE',  ( 9.270509831248423538, 77.30000000000001137, -12.75976212528059861 ) ) ;
#27896=CARTESIAN_POINT ( 'NONE',  ( 15.00000000000000000, 75.25000000546239676, -1.836970198721029589E-15 ) ) ;
#27898=EDGE_CURVE ( 'NONE', #7938, #7704, #15513, .T. ) ;
#27899=CARTESIAN_POINT ( 'NONE',  ( -33.58253175000000113, 35.02500000273118275, -10.91162601494193218 ) ) ;
#27902=CARTESIAN_POINT ( 'NONE',  ( -27.16883889988624290, 19.17500000273120264, -19.73931689729374028 ) ) ;
#27903=CARTESIAN_POINT ( 'NONE',  ( -24.50000000000000711, 16.84999999453763309, 7.960532557706201828 ) ) ;
#27904=EDGE_CURVE ( 'NONE', #3815, #25643, #11093, .T. ) ;
#27905=CARTESIAN_POINT ( 'NONE',  ( -24.50000000000000711, 14.84999999453763841, 7.960532557706201828 ) ) ;
#27906=CARTESIAN_POINT ( 'NONE',  ( 10.04305231718578817, 79.39999999999999147, -30.90933677959249337 ) ) ;
#27908=CARTESIAN_POINT ( 'NONE',  ( -23.41746824999999887, 11.62499999726881938, -2.867812753649727150E-15 ) ) ;
#27913=CARTESIAN_POINT ( 'NONE',  ( -27.16883889988624290, 14.92500000273117067, -19.73931689729374028 ) ) ;
#27914=CARTESIAN_POINT ( 'NONE',  ( 14.47279130897151767, 9.424999997268814766, -19.92008829642072598 ) ) ;
#27916=ORIENTED_EDGE ( 'NONE', *, *, #21266, .T. ) ;
#27919=EDGE_LOOP ( 'NONE', ( #24207, #30759, #5199, #94 ) ) ;
#27922=LINE ( 'NONE', #17804, #4672 ) ;
#27923=CARTESIAN_POINT ( 'NONE',  ( -23.41746825000000243, 4.024999997268810858, -7.608796670333730638 ) ) ;
#27924=CARTESIAN_POINT ( 'NONE',  ( -14.47279130897152122, 11.92499999726882010, 19.92008829642072243 ) ) ;
#27925=CARTESIAN_POINT ( 'NONE',  ( -33.58253175000000113, 23.47500000273119269, 10.91162601494193929 ) ) ;
#27926=CARTESIAN_POINT ( 'NONE',  ( 32.50000000000000000, 21.60000000546237331, -10.55989012756945833 ) ) ;
#27927=CARTESIAN_POINT ( 'NONE',  ( 10.04305231718579705, 68.59999999999999432, 30.90933677959248982 ) ) ;
#27928=CARTESIAN_POINT ( 'NONE',  ( -20.08610463437157989, 6.200000005462364960, -27.64615127144129758 ) ) ;
#27931=CARTESIAN_POINT ( 'NONE',  ( 27.16883889988623935, 34.57500000273120122, -19.73931689729374384 ) ) ;
#27932=CARTESIAN_POINT ( 'NONE',  ( 4.300734207923761154, 79.97500000273119269, 13.23629886949340495 ) ) ;
#27935=CARTESIAN_POINT ( 'NONE',  ( -18.94512977948575738, 15.92499999726881832, -13.76444248337723231 ) ) ;
#27936=CARTESIAN_POINT ( 'NONE',  ( 6.277390505771533514E-15, 14.50000000000000888, 34.17252228774368916 ) ) ;
#27940=CARTESIAN_POINT ( 'NONE',  ( -27.16883889988624290, 58.92500000273118133, -19.73931689729374028 ) ) ;
#27942=CARTESIAN_POINT ( 'NONE',  ( 27.16883889988623935, 50.57500000273118701, -19.73931689729374384 ) ) ;
#27944=LINE ( 'NONE', #32734, #31988 ) ;
#27945=CARTESIAN_POINT ( 'NONE',  ( -32.50000000000000000, 5.899999999999987921, -10.55989012756945300 ) ) ;
#27948=CARTESIAN_POINT ( 'NONE',  ( 24.50000000000000000, 3.899999999999992806, 7.960532557706212486 ) ) ;
#27950=DIRECTION ( 'NONE',  ( -0.000000000000000000, -1.000000000000000000, -0.000000000000000000 ) ) ;
#27955=CARTESIAN_POINT ( 'NONE',  ( 10.04305231718579705, 34.59999999999999432, 30.90933677959248982 ) ) ;
#27956=CARTESIAN_POINT ( 'NONE',  ( 6.486482029760648627E-15, 33.62500000273119127, 35.31076352940722529 ) ) ;
#27962=VERTEX_POINT ( 'NONE', #33319 ) ;
#27967=DIRECTION ( 'NONE',  ( -0.000000000000000000, -1.000000000000000000, -0.000000000000000000 ) ) ;
#27968=CARTESIAN_POINT ( 'NONE',  ( 33.58253175000000113, 38.47500000273118559, -10.91162601494193751 ) ) ;
#27969=CARTESIAN_POINT ( 'NONE',  ( 32.50000000000000711, 43.40000000546238113, 10.55989012756945122 ) ) ;
#27971=CARTESIAN_POINT ( 'NONE',  ( 20.75514604977248467, 32.42500000273116711, -28.56700777964554305 ) ) ;
#27972=CARTESIAN_POINT ( 'NONE',  ( -32.50000000000000000, 24.09999999999999787, 10.55989012756946366 ) ) ;
#27973=CARTESIAN_POINT ( 'NONE',  ( -10.37757302488624411, 56.97500000273119980, -31.93888565452638417 ) ) ;
#27975=CARTESIAN_POINT ( 'NONE',  ( 26.29305231718579350, 36.79999999999999716, 19.10302069950537529 ) ) ;
#27977=CARTESIAN_POINT ( 'NONE',  ( -10.37757302488624411, 74.72500000273119269, -31.93888565452638417 ) ) ;
#27980=CARTESIAN_POINT ( 'NONE',  ( -2.162160676586882350E-15, 68.87500000273118417, -35.31076352940722529 ) ) ;
#27982=ORIENTED_EDGE ( 'NONE', *, *, #480, .T. ) ;
#27983=CARTESIAN_POINT ( 'NONE',  ( 10.37757302488624056, 18.52500000273118985, -31.93888565452638417 ) ) ;
#27984=CARTESIAN_POINT ( 'NONE',  ( -4.732186688966233175E-15, 11.24999999453763699, 25.76082449383753925 ) ) ;
#27986=CARTESIAN_POINT ( 'NONE',  ( -20.08610463437157989, 25.69999999999999929, -27.64615127144129758 ) ) ;
#27996=LINE ( 'NONE', #9630, #26918 ) ;
#27997=CARTESIAN_POINT ( 'NONE',  ( 32.50000000000000711, 75.40000000546240244, 10.55989012756945122 ) ) ;
#28002=CARTESIAN_POINT ( 'NONE',  ( -27.16883889988623935, 75.57500000273120122, 19.73931689729374739 ) ) ;
#28004=VERTEX_POINT ( 'NONE', #15146 ) ;
#28006=CARTESIAN_POINT ( 'NONE',  ( -10.04305231718578462, 62.90000000546236691, 30.90933677959249337 ) ) ;
#28009=CARTESIAN_POINT ( 'NONE',  ( -33.58253175000000113, 49.02500000273116854, -10.91162601494193218 ) ) ;
#28010=CARTESIAN_POINT ( 'NONE',  ( -23.41746825000000243, 15.52499999726882507, -7.608796670333730638 ) ) ;
#28011=CARTESIAN_POINT ( 'NONE',  ( -10.04305231718579172, 8.100000005462376862, -30.90933677959248982 ) ) ;
#28012=CARTESIAN_POINT ( 'NONE',  ( -7.236395654485763274, 18.52499999726881086, 22.27133577429736633 ) ) ;
#28013=CARTESIAN_POINT ( 'NONE',  ( -20.08610463437157989, 53.69999999999999574, -27.64615127144129758 ) ) ;
#28014=CARTESIAN_POINT ( 'NONE',  ( 0.000000000000000000, 82.00000000000001421, 0.000000000000000000 ) ) ;
#28015=CARTESIAN_POINT ( 'NONE',  ( -33.58253175000000113, 15.47500000273118381, 10.91162601494193929 ) ) ;
#28018=CARTESIAN_POINT ( 'NONE',  ( 4.300734207923761154, 75.97500000273119269, 13.23629886949340495 ) ) ;
#28020=CARTESIAN_POINT ( 'NONE',  ( -26.29305231718578995, 44.20000000000001705, 19.10302069950538595 ) ) ;
#28022=ORIENTED_EDGE ( 'NONE', *, *, #1847, .T. ) ;
#28024=CARTESIAN_POINT ( 'NONE',  ( 5.147494310547408247, 71.05125428700921475, 32.50000000000000711 ) ) ;
#28032=EDGE_CURVE ( 'NONE', #16083, #22660, #28420, .T. ) ;
#28035=CARTESIAN_POINT ( 'NONE',  ( 32.50000000000000000, 3.000000000000002665, -3.980102097228898626E-15 ) ) ;
#28038=CARTESIAN_POINT ( 'NONE',  ( -2.162160676586882350E-15, 42.62500000273119838, -35.31076352940722529 ) ) ;
#28041=CARTESIAN_POINT ( 'NONE',  ( 15.00000000000000355, 78.89999999999997726, 4.873795443493592394 ) ) ;
#28042=VERTEX_POINT ( 'NONE', #5183 ) ;
#28045=CARTESIAN_POINT ( 'NONE',  ( -23.41746824999999887, 13.62499999726882116, -2.867812753649727150E-15 ) ) ;
#28047=ORIENTED_EDGE ( 'NONE', *, *, #32489, .F. ) ;
#28049=CARTESIAN_POINT ( 'NONE',  ( -1.778240108872766143E-15, 34.00000000546236834, -32.49999999999999289 ) ) ;
#28050=EDGE_LOOP ( 'NONE', ( #12117, #8668 ) ) ;
#28051=CARTESIAN_POINT ( 'NONE',  ( -1.778240108872766143E-15, 19.50000000000000000, -32.49999999999999289 ) ) ;
#28052=CARTESIAN_POINT ( 'NONE',  ( 10.37757302488624056, 66.52500000273120406, -31.93888565452638417 ) ) ;
#28054=CARTESIAN_POINT ( 'NONE',  ( 19.82091636218621034, 9.800000000000002487, 14.40073868116559730 ) ) ;
#28055=CARTESIAN_POINT ( 'NONE',  ( 18.94512977948576093, 1.324999997268816454, -13.76444248337722875 ) ) ;
#28056=CARTESIAN_POINT ( 'NONE',  ( -27.16883889988623935, 7.325000002731174575, 19.73931689729374739 ) ) ;
#28057=CARTESIAN_POINT ( 'NONE',  ( -3.880418787951124493, 7.198745712990782586, 24.50000000000000355 ) ) ;
#28059=CARTESIAN_POINT ( 'NONE',  ( 4.635254915624209993, 73.40000000000001990, -14.26584774442730463 ) ) ;
#28062=CARTESIAN_POINT ( 'NONE',  ( 5.147494310547434893, 22.55125428154684286, 32.49999999999999289 ) ) ;
#28064=DIRECTION ( 'NONE',  ( 0.000000000000000000, 0.000000000000000000, 1.000000000000000000 ) ) ;
#28066=CARTESIAN_POINT ( 'NONE',  ( -20.75514604977248112, 31.42500000273120619, 28.56700777964554661 ) ) ;
#28069=CARTESIAN_POINT ( 'NONE',  ( -20.75514604977248823, 23.07500000273117990, -28.56700777964554305 ) ) ;
#28070=CARTESIAN_POINT ( 'NONE',  ( -32.50000000000000000, 12.60000000546236620, 10.55989012756946366 ) ) ;
#28074=CARTESIAN_POINT ( 'NONE',  ( 23.41746824999999887, 10.52499999726880731, 7.608796670333735079 ) ) ;
#28075=CARTESIAN_POINT ( 'NONE',  ( -33.58253175000000113, 65.02500000273118985, -10.91162601494193041 ) ) ;
#28079=CARTESIAN_POINT ( 'NONE',  ( 20.75514604977249178, 11.82500000273118346, 28.56700777964553950 ) ) ;
#28080=CARTESIAN_POINT ( 'NONE',  ( -7.236395654485763274, 12.52499999726880375, 22.27133577429736633 ) ) ;
#28091=CARTESIAN_POINT ( 'NONE',  ( -23.41746825000000598, 6.224999997268827023, 7.608796670333726198 ) ) ;
#28092=CARTESIAN_POINT ( 'NONE',  ( -23.41746825000000243, 11.52499999726880553, -7.608796670333730638 ) ) ;
#28093=CARTESIAN_POINT ( 'NONE',  ( -27.16883889988623935, 17.57500000273118346, 19.73931689729374739 ) ) ;
#28094=CARTESIAN_POINT ( 'NONE',  ( -2.092463501923844636E-15, 26.00000000546237899, -34.17252228774368916 ) ) ;
#28096=CARTESIAN_POINT ( 'NONE',  ( 20.08610463437157279, 67.30000000000001137, -27.64615127144129758 ) ) ;
#28100=CARTESIAN_POINT ( 'NONE',  ( -10.37757302488623701, 27.77500000273119696, 31.93888565452638417 ) ) ;
#28101=CARTESIAN_POINT ( 'NONE',  ( -8.601468415847515203, 79.67500000273118133, 11.83890561707634959 ) ) ;
#28104=CARTESIAN_POINT ( 'NONE',  ( 18.94512977948575738, 14.92499999726881654, 13.76444248337723408 ) ) ;
#28105=CARTESIAN_POINT ( 'NONE',  ( 10.04305231718578817, 7.400000000000018119, -30.90933677959249337 ) ) ;
#28106=CARTESIAN_POINT ( 'NONE',  ( -20.08610463437157989, 51.69999999999999574, -27.64615127144129758 ) ) ;
#28108=CARTESIAN_POINT ( 'NONE',  ( 27.16883889988624290, 55.92500000273120975, 19.73931689729373673 ) ) ;
#28110=CARTESIAN_POINT ( 'NONE',  ( -10.37757302488624411, 40.97500000273118559, -31.93888565452638417 ) ) ;
#28112=CARTESIAN_POINT ( 'NONE',  ( 10.04305231718578817, 67.90000000546237402, -30.90933677959249337 ) ) ;
#28113=CARTESIAN_POINT ( 'NONE',  ( -10.37757302488623701, 1.525000002731202731, 31.93888565452638417 ) ) ;
#28117=CARTESIAN_POINT ( 'NONE',  ( -8.960552108402744065E-16, 80.87500000273118417, -14.63369212191046209 ) ) ;
#28119=DIRECTION ( 'NONE',  ( -0.000000000000000000, -1.000000000000000000, -0.000000000000000000 ) ) ;
#28123=CARTESIAN_POINT ( 'NONE',  ( 20.75514604977249178, 33.82500000273118701, 28.56700777964553950 ) ) ;
#28125=EDGE_LOOP ( 'NONE', ( #33793, #21191, #3650, #6934 ) ) ;
#28126=ORIENTED_EDGE ( 'NONE', *, *, #132, .T. ) ;
#28130=CARTESIAN_POINT ( 'NONE',  ( -32.50000000000000000, 16.60000000546238752, 10.55989012756946366 ) ) ;
#28137=CARTESIAN_POINT ( 'NONE',  ( 0.000000000000000000, 0.000000000000000000, 24.50000000000000000 ) ) ;
#28138=CARTESIAN_POINT ( 'NONE',  ( 33.58253175000000823, 38.27500000273118985, 10.91162601494192863 ) ) ;
#28139=CARTESIAN_POINT ( 'NONE',  ( 32.50000000000000000, 43.50000000546238965, -3.980102097228898626E-15 ) ) ;
#28141=CARTESIAN_POINT ( 'NONE',  ( 20.75514604977249178, 25.82500000273117280, 28.56700777964553950 ) ) ;
#28142=CARTESIAN_POINT ( 'NONE',  ( -13.91746824999999887, 80.87500000273118417, 0.000000000000000000 ) ) ;
#28143=CARTESIAN_POINT ( 'NONE',  ( -27.16883889988623935, 53.57500000273118701, 19.73931689729374739 ) ) ;
#28146=CARTESIAN_POINT ( 'NONE',  ( 32.50000000000000000, 29.10000000000000853, -10.55989012756945833 ) ) ;
#28148=CARTESIAN_POINT ( 'NONE',  ( -27.16883889988624290, 78.92500000273116711, -19.73931689729374028 ) ) ;
#28150=CARTESIAN_POINT ( 'NONE',  ( -32.50000000000000000, 20.50000000546237189, 0.000000000000000000 ) ) ;
#28151=CARTESIAN_POINT ( 'NONE',  ( 20.75514604977248467, 62.67500000273117422, -28.56700777964554305 ) ) ;
#28154=CARTESIAN_POINT ( 'NONE',  ( -20.75514604977248112, 17.42500000273117777, 28.56700777964554661 ) ) ;
#28155=CARTESIAN_POINT ( 'NONE',  ( 19.82091636218621389, 9.949999994537634507, -14.40073868116559197 ) ) ;
#28157=CARTESIAN_POINT ( 'NONE',  ( 15.14183272437242067, 7.449999994537640724, 20.84094480462498211 ) ) ;
#28166=CARTESIAN_POINT ( 'NONE',  ( -7.570916362186215665, 3.149999994537633352, 23.30088464923126423 ) ) ;
#28168=CARTESIAN_POINT ( 'NONE',  ( -20.08610463437156923, 72.80000000546239391, 27.64615127144130113 ) ) ;
#28173=CARTESIAN_POINT ( 'NONE',  ( 10.37757302488624056, 74.77500000273118985, -31.93888565452638417 ) ) ;
#28177=CARTESIAN_POINT ( 'NONE',  ( -26.29305231718578995, 64.70000000546238539, 19.10302069950538595 ) ) ;
#28178=ORIENTED_EDGE ( 'NONE', *, *, #33712, .T. ) ;
#28180=CARTESIAN_POINT ( 'NONE',  ( 10.37757302488624767, 51.72500000273119980, 31.93888565452638417 ) ) ;
#28181=CARTESIAN_POINT ( 'NONE',  ( 14.47279130897151589, 18.32499999726882578, 19.92008829642072953 ) ) ;
#28182=CARTESIAN_POINT ( 'NONE',  ( 32.50000000000000711, 3.400000005462366914, 10.55989012756945122 ) ) ;
#28183=CARTESIAN_POINT ( 'NONE',  ( 3.000384657911015469E-15, 0.000000000000000000, -24.50000000000000000 ) ) ;
#28185=CARTESIAN_POINT ( 'NONE',  ( -2.092463501923844636E-15, 47.49999999999997868, -34.17252228774368916 ) ) ;
#28187=CARTESIAN_POINT ( 'NONE',  ( -33.58253175000000113, 19.37500000273118062, 0.000000000000000000 ) ) ;
#28188=CARTESIAN_POINT ( 'NONE',  ( 15.14183272437242422, 0.2999999999999904965, -20.84094480462497856 ) ) ;
#28190=CARTESIAN_POINT ( 'NONE',  ( 2.688165632520823219E-15, 75.87500000273119838, 14.63369212191046387 ) ) ;
#28192=CARTESIAN_POINT ( 'NONE',  ( -1.778240108872766143E-15, 54.00000000546237544, -32.49999999999999289 ) ) ;
#28207=CARTESIAN_POINT ( 'NONE',  ( 20.08610463437158344, 68.70000000000001705, 27.64615127144129403 ) ) ;
#28209=CARTESIAN_POINT ( 'NONE',  ( -10.37757302488623701, 45.52500000273118985, 31.93888565452638417 ) ) ;
#28213=CARTESIAN_POINT ( 'NONE',  ( 10.04305231718579705, 42.60000000000000142, 30.90933677959248982 ) ) ;
#28215=CARTESIAN_POINT ( 'NONE',  ( 27.16883889988624290, 74.17500000273119554, 19.73931689729373673 ) ) ;
#28216=VERTEX_POINT ( 'NONE', #12906 ) ;
#28219=ORIENTED_EDGE ( 'NONE', *, *, #26732, .F. ) ;
#28220=( BOUNDED_CURVE ( )  B_SPLINE_CURVE ( 2, ( #29807, #6308, #27074, #1308, #13876, #8711, #19194, #17120, #3737, #645, #1138, #3568, #30137 ),
 .UNSPECIFIED., .F., .T. ) 
 B_SPLINE_CURVE_WITH_KNOTS ( ( 3, 2, 2, 2, 2, 2, 3 ),
 ( 0.5192307692307692735, 0.5205128205128205510, 0.5230769230769231060, 0.5256410256410256610, 0.5282051282051282159, 0.5307692307692307709, 0.5320512820512820484 ),
 .UNSPECIFIED. ) 
 CURVE ( )  GEOMETRIC_REPRESENTATION_ITEM ( )  RATIONAL_B_SPLINE_CURVE ( ( 0.9755282581475768211, 0.9755282581475768211, 1.000000000000000000, 0.9510565162951535312, 1.000000000000000000, 0.9510565162951535312, 1.000000000000000000, 0.9510565162951535312, 1.000000000000000000, 0.9510565162951535312, 1.000000000000000000, 0.9755282581475768211, 0.9755282581475768211 ) ) 
 REPRESENTATION_ITEM ( '' )  );
#28221=CARTESIAN_POINT ( 'NONE',  ( 10.04305231718579705, 29.10000000546236620, 30.90933677959248982 ) ) ;
#28222=CARTESIAN_POINT ( 'NONE',  ( -27.16883889988624290, 66.92500000273119554, -19.73931689729374028 ) ) ;
#28225=CARTESIAN_POINT ( 'NONE',  ( 7.570916362186207671, 9.599999999999997868, 23.30088464923126779 ) ) ;
#28227=CARTESIAN_POINT ( 'NONE',  ( -20.75514604977248823, 10.82500000273118701, -28.56700777964554305 ) ) ;
#28230=CARTESIAN_POINT ( 'NONE',  ( 2.897257156509938333E-15, 76.50000000000001421, 15.77193336357400710 ) ) ;
#28232=CARTESIAN_POINT ( 'NONE',  ( -4.934616302121927505E-14, 70.50000000000000000, 32.50000000000000000 ) ) ;
#28233=EDGE_CURVE ( 'NONE', #32300, #21391, #31410, .T. ) ;
#28235=CARTESIAN_POINT ( 'NONE',  ( -15.00000000000000000, 76.25000000546239676, 0.000000000000000000 ) ) ;
#28237=CARTESIAN_POINT ( 'NONE',  ( 10.37757302488624056, 32.52500000273117564, -31.93888565452638417 ) ) ;
#28240=CARTESIAN_POINT ( 'NONE',  ( 10.37757302488624056, 22.77500000273119340, -31.93888565452638417 ) ) ;
#28242=EDGE_CURVE ( 'NONE', #12293, #5896, #8419, .T. ) ;
#28243=CARTESIAN_POINT ( 'NONE',  ( -2.162160676586882350E-15, 74.62500000273116996, -35.31076352940722529 ) ) ;
#28245=CARTESIAN_POINT ( 'NONE',  ( 4.445600272181915325E-13, 26.00000000546237189, -32.50000000000000000 ) ) ;
#28247=CARTESIAN_POINT ( 'NONE',  ( 23.41746824999999887, 16.72499999726881725, -7.608796670333727974 ) ) ;
#28248=CARTESIAN_POINT ( 'NONE',  ( 6.486482029760648627E-15, 65.62500000273116996, 35.31076352940722529 ) ) ;
#28252=CARTESIAN_POINT ( 'NONE',  ( 10.37757302488624767, 3.725000002731182480, 31.93888565452638417 ) ) ;
#28253=CARTESIAN_POINT ( 'NONE',  ( 23.41746825000000243, 9.224999997268820806, -7.608796670333727974 ) ) ;
#28260=LINE ( 'NONE', #20891, #8377 ) ;
#28262=DIRECTION ( 'NONE',  ( -0.000000000000000000, -1.000000000000000000, -0.000000000000000000 ) ) ;
#28263=CARTESIAN_POINT ( 'NONE',  ( -7.236395654485757944, 5.724999997268803931, -22.27133577429736988 ) ) ;
#28264=CARTESIAN_POINT ( 'NONE',  ( -18.94512977948576093, 9.824999997268824004, 13.76444248337722698 ) ) ;
#28265=CARTESIAN_POINT ( 'NONE',  ( 20.75514604977249178, 14.07500000273119944, 28.56700777964553950 ) ) ;
#28266=CARTESIAN_POINT ( 'NONE',  ( -20.08610463437157989, 26.20000000546237828, -27.64615127144129758 ) ) ;
#28267=CARTESIAN_POINT ( 'NONE',  ( 10.04305231718578817, 67.40000000000001990, -30.90933677959249337 ) ) ;
#28268=CARTESIAN_POINT ( 'NONE',  ( 9.270509831248421762, 77.55000000546237970, -12.75976212528059861 ) ) ;
#28269=CARTESIAN_POINT ( 'NONE',  ( -5.147494310547430452, 29.55125428154684997, -32.49999999999999289 ) ) ;
#28271=CARTESIAN_POINT ( 'NONE',  ( 33.58253175000000113, 32.37500000273119127, -4.112674001490185761E-15 ) ) ;
#28272=CARTESIAN_POINT ( 'NONE',  ( 26.29305231718578995, 43.70000000546237118, -19.10302069950538240 ) ) ;
#28274=CARTESIAN_POINT ( 'NONE',  ( -23.41746824999999887, 18.12499999726882649, -2.867812753649727150E-15 ) ) ;
#28275=CARTESIAN_POINT ( 'NONE',  ( 20.08610463437157279, 7.300000000000001599, -27.64615127144129758 ) ) ;
#28276=CARTESIAN_POINT ( 'NONE',  ( -26.29305231718579350, 51.80000000000001137, -19.10302069950537884 ) ) ;
#28278=CARTESIAN_POINT ( 'NONE',  ( -20.75514604977248112, 47.42500000273118843, 28.56700777964554661 ) ) ;
#28281=CARTESIAN_POINT ( 'NONE',  ( 20.75514604977249178, 38.07500000273115859, 28.56700777964553950 ) ) ;
#28284=CARTESIAN_POINT ( 'NONE',  ( 32.50000000000000000, 15.50000000546236656, -3.980102097228898626E-15 ) ) ;
#28285=CARTESIAN_POINT ( 'NONE',  ( 5.147494310547426899, 51.94874572391552903, -32.50000000000000000 ) ) ;
#28288=CARTESIAN_POINT ( 'NONE',  ( -1.778240108872766143E-15, 7.500000000000001776, -32.49999999999999289 ) ) ;
#28292=CARTESIAN_POINT ( 'NONE',  ( 15.00000000000000000, 71.35000000546237686, -4.873795443493596835 ) ) ;
#28293=CARTESIAN_POINT ( 'NONE',  ( -2.162160676586882350E-15, 26.62500000273118417, -35.31076352940722529 ) ) ;
#28305=CARTESIAN_POINT ( 'NONE',  ( -26.29305231718579350, 45.80000000000000426, -19.10302069950537884 ) ) ;
#28306=CARTESIAN_POINT ( 'NONE',  ( -20.75514604977248112, 37.67500000273118133, 28.56700777964554661 ) ) ;
#28307=CARTESIAN_POINT ( 'NONE',  ( 10.04305231718578817, 45.90000000546237402, -30.90933677959249337 ) ) ;
#28309=CARTESIAN_POINT ( 'NONE',  ( 27.16883889988624290, 23.92500000273117777, 19.73931689729373673 ) ) ;
#28311=CARTESIAN_POINT ( 'NONE',  ( -10.37757302488623701, 47.77500000273118985, 31.93888565452638417 ) ) ;
#28313=CARTESIAN_POINT ( 'NONE',  ( -20.08610463437157989, 29.69999999999999574, -27.64615127144129758 ) ) ;
#28315=( BOUNDED_CURVE ( )  B_SPLINE_CURVE ( 2, ( #33148, #28359, #9652, #12913, #33500, #20132, #30751, #4846, #10003, #7073, #20301, #9475, #15327 ),
 .UNSPECIFIED., .F., .T. ) 
 B_SPLINE_CURVE_WITH_KNOTS ( ( 3, 2, 2, 2, 2, 2, 3 ),
 ( 0.8397435897435897578, 0.8410256410256410353, 0.8435897435897435903, 0.8461538461538461453, 0.8487179487179487003, 0.8512820512820512553, 0.8525641025641025328 ),
 .UNSPECIFIED. ) 
 CURVE ( )  GEOMETRIC_REPRESENTATION_ITEM ( )  RATIONAL_B_SPLINE_CURVE ( ( 0.9755282581475768211, 0.9755282581475768211, 1.000000000000000000, 0.9510565162951535312, 1.000000000000000000, 0.9510565162951535312, 1.000000000000000000, 0.9510565162951535312, 1.000000000000000000, 0.9510565162951535312, 1.000000000000000000, 0.9755282581475768211, 0.9755282581475768211 ) ) 
 REPRESENTATION_ITEM ( '' )  );
#28316=CARTESIAN_POINT ( 'NONE',  ( -33.58253175000000113, 71.12500000273119838, 0.000000000000000000 ) ) ;
#28317=DIRECTION ( 'NONE',  ( 0.000000000000000000, 1.000000000000000000, 0.000000000000000000 ) ) ;
#28319=CARTESIAN_POINT ( 'NONE',  ( -33.58253175000000113, 57.47500000273118559, 10.91162601494193929 ) ) ;
#28321=CARTESIAN_POINT ( 'NONE',  ( -27.16883889988624290, 18.92500000273117422, -19.73931689729374028 ) ) ;
#28322=CARTESIAN_POINT ( 'NONE',  ( 15.14183272437241889, 9.449999994537636283, 20.84094480462498211 ) ) ;
#28325=CARTESIAN_POINT ( 'NONE',  ( -32.50000000000000000, 26.09999999999999076, 10.55989012756946366 ) ) ;
#28330=ADVANCED_FACE ( 'NONE', ( #5311 ), #1440, .F. ) ;
#28336=CARTESIAN_POINT ( 'NONE',  ( 20.08610463437158344, 62.69999999999998863, 27.64615127144129403 ) ) ;
#28339=CIRCLE ( 'NONE', #382, 26.50000000000000355 ) ;
#28340=CARTESIAN_POINT ( 'NONE',  ( 32.50000000000000000, 77.60000000546239107, -10.55989012756945833 ) ) ;
#28345=CARTESIAN_POINT ( 'NONE',  ( 6.486482029760649416E-15, 77.87500000273118417, 35.31076352940723240 ) ) ;
#28348=CARTESIAN_POINT ( 'NONE',  ( 6.486482029760649416E-15, 55.87500000273118417, 35.31076352940723240 ) ) ;
#28349=CARTESIAN_POINT ( 'NONE',  ( -32.50000000000000000, 60.60000000546239107, 10.55989012756946366 ) ) ;
#28350=ORIENTED_EDGE ( 'NONE', *, *, #17349, .T. ) ;
#28352=CARTESIAN_POINT ( 'NONE',  ( 33.58253175000000113, 42.12500000273116996, -4.112674001490185761E-15 ) ) ;
#28353=LINE ( 'NONE', #2092, #17616 ) ;
#28354=CARTESIAN_POINT ( 'NONE',  ( 33.58253175000000823, 66.27500000273118985, 10.91162601494192863 ) ) ;
#28355=CARTESIAN_POINT ( 'NONE',  ( -26.29305231718578995, 2.700000005462388497, 19.10302069950538595 ) ) ;
#28357=DIRECTION ( 'NONE',  ( -0.000000000000000000, -1.000000000000000000, -0.000000000000000000 ) ) ;
#28358=CARTESIAN_POINT ( 'NONE',  ( -2.092463501923844636E-15, 45.49999999999998579, -34.17252228774368916 ) ) ;
#28359=CARTESIAN_POINT ( 'NONE',  ( -5.147494310547423346, 14.44874571845315536, 32.50000000000000000 ) ) ;
#28360=CARTESIAN_POINT ( 'NONE',  ( 10.37757302488624056, 14.77500000273118630, -31.93888565452638417 ) ) ;
#28361=CARTESIAN_POINT ( 'NONE',  ( -20.08610463437157989, 73.70000000000000284, -27.64615127144129758 ) ) ;
#28363=CARTESIAN_POINT ( 'NONE',  ( -13.91746824999999887, 70.87500000273119838, 0.000000000000000000 ) ) ;
#28364=CARTESIAN_POINT ( 'NONE',  ( -1.778240108872766143E-15, 68.00000000546238255, -32.49999999999999289 ) ) ;
#28365=CARTESIAN_POINT ( 'NONE',  ( 32.50000000000000711, 53.40000000546238113, 10.55989012756945122 ) ) ;
#28378=CARTESIAN_POINT ( 'NONE',  ( 11.25946833292375793, 74.17500000273119554, 8.180482586598731842 ) ) ;
#28380=CARTESIAN_POINT ( 'NONE',  ( -10.37757302488624411, 46.72500000273119269, -31.93888565452638417 ) ) ;
#28382=CARTESIAN_POINT ( 'NONE',  ( 20.08610463437157279, 21.80000000546236549, -27.64615127144129758 ) ) ;
#28383=EDGE_LOOP ( 'NONE', ( #8872, #4916, #21183, #21434 ) ) ;
#28385=CARTESIAN_POINT ( 'NONE',  ( 20.08610463437158344, 42.69999999999998153, 27.64615127144129403 ) ) ;
#28387=CARTESIAN_POINT ( 'NONE',  ( -33.58253175000000113, 73.27500000273118985, -10.91162601494193218 ) ) ;
#28391=ORIENTED_EDGE ( 'NONE', *, *, #9780, .F. ) ;
#28393=CARTESIAN_POINT ( 'NONE',  ( -27.16883889988623935, 59.32500000273119412, 19.73931689729374739 ) ) ;
#28395=CARTESIAN_POINT ( 'NONE',  ( 7.570916362186213000, 12.39999999999999503, -23.30088464923126423 ) ) ;
#28396=CARTESIAN_POINT ( 'NONE',  ( -18.94512977948575738, 1.924999997268805885, -13.76444248337723231 ) ) ;
#28397=CARTESIAN_POINT ( 'NONE',  ( 20.75514604977248467, 8.425000002731204418, -28.56700777964554305 ) ) ;
#28398=CARTESIAN_POINT ( 'NONE',  ( 32.50000000000000711, 28.89999999999998792, 10.55989012756945122 ) ) ;
#28400=CARTESIAN_POINT ( 'NONE',  ( 32.50000000000000000, 37.00000000000000711, -3.980102097228898626E-15 ) ) ;
#28405=CARTESIAN_POINT ( 'NONE',  ( 2.688165632520823219E-15, 79.37500000273119838, 14.63369212191046387 ) ) ;
#28407=CARTESIAN_POINT ( 'NONE',  ( 33.58253175000000113, 32.12500000273119127, -4.112674001490185761E-15 ) ) ;
#28410=CARTESIAN_POINT ( 'NONE',  ( 6.486482029760648627E-15, 21.87500000273118772, 35.31076352940722529 ) ) ;
#28411=CARTESIAN_POINT ( 'NONE',  ( -26.29305231718579350, 67.79999999999999716, -19.10302069950537884 ) ) ;
#28412=CARTESIAN_POINT ( 'NONE',  ( -33.58253175000000113, 75.22500000273119269, 10.91162601494193929 ) ) ;
#28413=CARTESIAN_POINT ( 'NONE',  ( 24.50000000000000000, 8.000000000000007105, 0.000000000000000000 ) ) ;
#28415=CARTESIAN_POINT ( 'NONE',  ( 7.236395654485755280, 16.22499999726881370, 22.27133577429736988 ) ) ;
#28416=CARTESIAN_POINT ( 'NONE',  ( -33.58253175000000113, 65.22500000273117848, 10.91162601494193929 ) ) ;
#28417=( BOUNDED_CURVE ( )  B_SPLINE_CURVE ( 2, ( #25474, #9852, #4874, #31127, #30779, #23068, #26153, #7619, #2123, #30604, #18099, #28546, #13110 ),
 .UNSPECIFIED., .F., .T. ) 
 B_SPLINE_CURVE_WITH_KNOTS ( ( 3, 2, 2, 2, 2, 2, 3 ),
 ( 0.9423076923076922906, 0.9435897435897435681, 0.9461538461538461231, 0.9487179487179486781, 0.9512820512820512331, 0.9538461538461538991, 0.9551282051282051766 ),
 .UNSPECIFIED. ) 
 CURVE ( )  GEOMETRIC_REPRESENTATION_ITEM ( )  RATIONAL_B_SPLINE_CURVE ( ( 0.9755282581475768211, 0.9755282581475768211, 1.000000000000000000, 0.9510565162951535312, 1.000000000000000000, 0.9510565162951535312, 1.000000000000000000, 0.9510565162951535312, 1.000000000000000000, 0.9510565162951535312, 1.000000000000000000, 0.9755282581475768211, 0.9755282581475768211 ) ) 
 REPRESENTATION_ITEM ( '' )  );
#28420=( BOUNDED_CURVE ( )  B_SPLINE_CURVE ( 2, ( #23550, #17721, #33669, #12391, #9817, #33492, #23035, #7587, #22861, #20650, #25776, #10338, #10166 ),
 .UNSPECIFIED., .F., .T. ) 
 B_SPLINE_CURVE_WITH_KNOTS ( ( 3, 2, 2, 2, 2, 2, 3 ),
 ( 0.8653846153846154188, 0.8666666666666666963, 0.8692307692307692513, 0.8717948717948718063, 0.8743589743589743613, 0.8769230769230769162, 0.8782051282051281937 ),
 .UNSPECIFIED. ) 
 CURVE ( )  GEOMETRIC_REPRESENTATION_ITEM ( )  RATIONAL_B_SPLINE_CURVE ( ( 0.9755282581475768211, 0.9755282581475768211, 1.000000000000000000, 0.9510565162951535312, 1.000000000000000000, 0.9510565162951535312, 1.000000000000000000, 0.9510565162951535312, 1.000000000000000000, 0.9510565162951535312, 1.000000000000000000, 0.9755282581475768211, 0.9755282581475768211 ) ) 
 REPRESENTATION_ITEM ( '' )  );
#28421=CARTESIAN_POINT ( 'NONE',  ( -20.75514604977248823, 8.825000002731192339, -28.56700777964554305 ) ) ;
#28422=CARTESIAN_POINT ( 'NONE',  ( -23.41746825000000243, 16.02499999726881086, -7.608796670333730638 ) ) ;
#28424=ORIENTED_EDGE ( 'NONE', *, *, #30398, .T. ) ;
#28426=ORIENTED_EDGE ( 'NONE', *, *, #6322, .T. ) ;
#28428=CARTESIAN_POINT ( 'NONE',  ( 5.779280353836490358E-15, 40.49999999999999289, 32.49999999999999289 ) ) ;
#28431=CARTESIAN_POINT ( 'NONE',  ( -23.41746825000000243, 2.024999997268815299, -7.608796670333730638 ) ) ;
#28432=CARTESIAN_POINT ( 'NONE',  ( -23.41746824999999887, 9.624999997268817609, -2.867812753649727150E-15 ) ) ;
#28433=CARTESIAN_POINT ( 'NONE',  ( 10.37757302488624767, 15.97500000273119269, 31.93888565452638417 ) ) ;
#28434=CARTESIAN_POINT ( 'NONE',  ( 32.50000000000000711, 21.40000000546237757, 10.55989012756945122 ) ) ;
#28435=CARTESIAN_POINT ( 'NONE',  ( -26.29305231718579350, 63.79999999999999716, -19.10302069950537884 ) ) ;
#28438=CARTESIAN_POINT ( 'NONE',  ( 0.000000000000000000, 80.00000000000001421, 0.000000000000000000 ) ) ;
#28441=CARTESIAN_POINT ( 'NONE',  ( 23.41746825000000243, 17.02499999726880731, 7.608796670333735079 ) ) ;
#28442=CARTESIAN_POINT ( 'NONE',  ( -20.08610463437156923, 8.300000000000000711, 27.64615127144130113 ) ) ;
#28443=CARTESIAN_POINT ( 'NONE',  ( 2.445080149700053643E-15, 74.50000000000001421, 15.00000000000000000 ) ) ;
#28445=CARTESIAN_POINT ( 'NONE',  ( -27.16883889988623935, 49.32500000273118701, 19.73931689729374739 ) ) ;
#28447=CARTESIAN_POINT ( 'NONE',  ( 33.58253175000000113, 42.37500000273119838, -4.112674001490185761E-15 ) ) ;
#28448=CARTESIAN_POINT ( 'NONE',  ( 32.50000000000000000, 45.10000000000000142, -10.55989012756945833 ) ) ;
#28451=EDGE_CURVE ( 'NONE', #26696, #28004, #14845, .T. ) ;
#28452=CARTESIAN_POINT ( 'NONE',  ( 0.000000000000000000, 80.00000000000001421, 0.000000000000000000 ) ) ;
#28455=CARTESIAN_POINT ( 'NONE',  ( -10.04305231718578462, 62.90000000546236691, 30.90933677959249337 ) ) ;
#28456=LINE ( 'NONE', #23491, #10076 ) ;
#28457=CARTESIAN_POINT ( 'NONE',  ( 15.14183272437242422, 10.04999999453761639, -20.84094480462497856 ) ) ;
#28460=CARTESIAN_POINT ( 'NONE',  ( -10.04305231718578462, 12.39999999999999503, 30.90933677959249337 ) ) ;
#28461=CARTESIAN_POINT ( 'NONE',  ( 33.58253175000000113, 24.12500000273118417, -4.112674001490185761E-15 ) ) ;
#28472=CARTESIAN_POINT ( 'NONE',  ( -10.04305231718578462, 46.39999999999999858, 30.90933677959249337 ) ) ;
#28473=CARTESIAN_POINT ( 'NONE',  ( -27.16883889988624290, 35.17500000273118843, -19.73931689729374028 ) ) ;
#28474=CARTESIAN_POINT ( 'NONE',  ( -20.08610463437157989, 38.20000000546236407, -27.64615127144129758 ) ) ;
#28477=CARTESIAN_POINT ( 'NONE',  ( -33.58253175000000113, 25.02500000273117209, -10.91162601494193218 ) ) ;
#28478=CARTESIAN_POINT ( 'NONE',  ( 24.50000000000000000, 5.849999994537632197, -7.960532557706203605 ) ) ;
#28479=CARTESIAN_POINT ( 'NONE',  ( 33.58253175000000823, 50.27500000273118985, 10.91162601494192863 ) ) ;
#28481=CARTESIAN_POINT ( 'NONE',  ( 10.04305231718579705, 28.60000000000001563, 30.90933677959248982 ) ) ;
#28483=CARTESIAN_POINT ( 'NONE',  ( 20.75514604977248467, 72.42500000273119554, -28.56700777964554305 ) ) ;
#28485=CARTESIAN_POINT ( 'NONE',  ( -33.58253175000000113, 59.27500000273119696, -10.91162601494193041 ) ) ;
#28486=CARTESIAN_POINT ( 'NONE',  ( -20.08610463437157989, 40.20000000546236407, -27.64615127144129758 ) ) ;
#28487=CARTESIAN_POINT ( 'NONE',  ( -33.58253175000000113, 15.02500000273120051, -10.91162601494193218 ) ) ;
#28492=CARTESIAN_POINT ( 'NONE',  ( 10.04305231718579705, 18.60000000000000497, 30.90933677959248982 ) ) ;
#28499=CARTESIAN_POINT ( 'NONE',  ( 20.08610463437157279, 73.80000000546239391, -27.64615127144129758 ) ) ;
#28504=CARTESIAN_POINT ( 'NONE',  ( 33.58253175000000113, 74.47500000273116427, -10.91162601494193751 ) ) ;
#28508=CARTESIAN_POINT ( 'NONE',  ( 27.16883889988624290, 52.17500000273117422, 19.73931689729373673 ) ) ;
#28509=CARTESIAN_POINT ( 'NONE',  ( 20.08610463437158344, 65.20000000546235697, 27.64615127144129403 ) ) ;
#28511=( BOUNDED_CURVE ( )  B_SPLINE_CURVE ( 2, ( #21284, #18032, #15962, #12868, #15795, #26080, #10465, #28478, #2739, #28644, #20943, #7882, #28817 ),
 .UNSPECIFIED., .F., .T. ) 
 B_SPLINE_CURVE_WITH_KNOTS ( ( 3, 2, 2, 2, 2, 2, 3 ),
 ( 0.1944444444444444475, 0.2000000000000000111, 0.2111111111111111105, 0.2222222222222222099, 0.2333333333333333370, 0.2444444444444444364, 0.2499999999999999722 ),
 .UNSPECIFIED. ) 
 CURVE ( )  GEOMETRIC_REPRESENTATION_ITEM ( )  RATIONAL_B_SPLINE_CURVE ( ( 0.9755282581475768211, 0.9755282581475768211, 1.000000000000000000, 0.9510565162951535312, 1.000000000000000000, 0.9510565162951535312, 1.000000000000000000, 0.9510565162951535312, 1.000000000000000000, 0.9510565162951535312, 1.000000000000000000, 0.9755282581475768211, 0.9755282581475768211 ) ) 
 REPRESENTATION_ITEM ( '' )  );
#28513=CARTESIAN_POINT ( 'NONE',  ( -27.16883889988623935, 41.32500000273120122, 19.73931689729374739 ) ) ;
#28514=CARTESIAN_POINT ( 'NONE',  ( 4.635254915624212657, 72.85000000546237686, 14.26584774442730286 ) ) ;
#28515=CARTESIAN_POINT ( 'NONE',  ( 33.58253175000000823, 70.27500000273118985, 10.91162601494192863 ) ) ;
#28516=ADVANCED_FACE ( 'NONE', ( #32678 ), #19658, .T. ) ;
#28517=CARTESIAN_POINT ( 'NONE',  ( 32.50000000000000711, 5.400000005462390895, 10.55989012756945122 ) ) ;
#28519=FACE_OUTER_BOUND ( 'NONE', #32648, .T. ) ;
#28520=CARTESIAN_POINT ( 'NONE',  ( 26.29305231718578995, 47.19999999999998863, -19.10302069950538240 ) ) ;
#28521=DIRECTION ( 'NONE',  ( 0.000000000000000000, 0.000000000000000000, -1.000000000000000000 ) ) ;
#28522=CARTESIAN_POINT ( 'NONE',  ( -10.37757302488623701, 7.775000002731180970, 31.93888565452638417 ) ) ;
#28523=CARTESIAN_POINT ( 'NONE',  ( -7.570916362186215665, 7.399999999999989697, 23.30088464923126423 ) ) ;
#28525=CARTESIAN_POINT ( 'NONE',  ( 13.91746824999999887, 78.37500000273116996, -1.704398294459741270E-15 ) ) ;
#28526=CARTESIAN_POINT ( 'NONE',  ( -1.778240108872766143E-15, 48.00000000546238255, -32.49999999999999289 ) ) ;
#28527=FACE_OUTER_BOUND ( 'NONE', #22424, .T. ) ;
#28541=CARTESIAN_POINT ( 'NONE',  ( 33.58253175000000113, 44.22500000273117848, -10.91162601494193574 ) ) ;
#28546=CARTESIAN_POINT ( 'NONE',  ( -5.147494310547430452, 4.051254287009220967, -32.49999999999999289 ) ) ;
#28547=CIRCLE ( 'NONE', #13759, 32.50000000000000000 ) ;
#28549=CARTESIAN_POINT ( 'NONE',  ( -33.58253175000000113, 77.37500000273116996, 0.000000000000000000 ) ) ;
#28550=VERTEX_POINT ( 'NONE', #3701 ) ;
#28554=ORIENTED_EDGE ( 'NONE', *, *, #18037, .F. ) ;
#28555=CARTESIAN_POINT ( 'NONE',  ( 5.779280353836490358E-15, 49.00000000546238255, 32.49999999999999289 ) ) ;
#28556=CARTESIAN_POINT ( 'NONE',  ( -33.58253175000000113, 59.22500000273119269, 10.91162601494193929 ) ) ;
#28559=CARTESIAN_POINT ( 'NONE',  ( -19.82091636218621389, 17.19999999999999218, 14.40073868116558842 ) ) ;
#28560=VECTOR ( 'NONE', #29357, 1000.000000000000000 ) ;
#28561=CARTESIAN_POINT ( 'NONE',  ( -27.16883889988624290, 4.925000002731189319, -19.73931689729374028 ) ) ;
#28562=CARTESIAN_POINT ( 'NONE',  ( -7.570916362186210335, 6.349999994537613546, -23.30088464923126779 ) ) ;
#28565=CARTESIAN_POINT ( 'NONE',  ( 5.147494310547426899, 9.448745718453144704, -32.50000000000000000 ) ) ;
#28569=CARTESIAN_POINT ( 'NONE',  ( -4.635254915624211769, 71.85000000546237686, -14.26584774442730286 ) ) ;
#28571=CARTESIAN_POINT ( 'NONE',  ( 20.75514604977249178, 29.82500000273119767, 28.56700777964553950 ) ) ;
#28575=CARTESIAN_POINT ( 'NONE',  ( 27.16883889988624290, 24.17500000273117777, 19.73931689729373673 ) ) ;
#28576=CARTESIAN_POINT ( 'NONE',  ( -10.04305231718579172, 67.59999999999999432, -30.90933677959248982 ) ) ;
#28578=CARTESIAN_POINT ( 'NONE',  ( -3.880418787951142701, 15.19874571299077282, 24.49999999999999645 ) ) ;
#28579=CARTESIAN_POINT ( 'NONE',  ( 0.000000000000000000, 80.00000000000001421, 0.000000000000000000 ) ) ;
#28581=CARTESIAN_POINT ( 'NONE',  ( 7.236395654485760609, 17.02499999726880731, -22.27133577429736633 ) ) ;
#28582=CARTESIAN_POINT ( 'NONE',  ( -20.75514604977248112, 63.42500000273118843, 28.56700777964554661 ) ) ;
#28585=CARTESIAN_POINT ( 'NONE',  ( -10.37757302488623701, 7.525000002731207616, 31.93888565452638417 ) ) ;
#28586=CARTESIAN_POINT ( 'NONE',  ( 23.41746824999999887, 19.12499999726882649, 0.000000000000000000 ) ) ;
#28588=ORIENTED_EDGE ( 'NONE', *, *, #17135, .T. ) ;
#28594=CARTESIAN_POINT ( 'NONE',  ( 23.41746824999999887, 3.124999997268812280, 0.000000000000000000 ) ) ;
#28595=CARTESIAN_POINT ( 'NONE',  ( -7.236395654485763274, 18.02499999726880731, 22.27133577429736633 ) ) ;
#28596=CARTESIAN_POINT ( 'NONE',  ( -20.75514604977248823, 17.07500000273119056, -28.56700777964554305 ) ) ;
#28597=CARTESIAN_POINT ( 'NONE',  ( -20.08610463437157989, 20.20000000546239249, -27.64615127144129758 ) ) ;
#28598=CARTESIAN_POINT ( 'NONE',  ( 26.29305231718578995, 65.20000000000000284, -19.10302069950538240 ) ) ;
#28599=CARTESIAN_POINT ( 'NONE',  ( 12.13525491562421088, 77.05000000546239391, 8.816778784387095058 ) ) ;
#28600=DIRECTION ( 'NONE',  ( -0.000000000000000000, -1.000000000000000000, -0.000000000000000000 ) ) ;
#28602=CARTESIAN_POINT ( 'NONE',  ( 11.25946833292375793, 80.57500000273121543, -8.180482586598735395 ) ) ;
#28606=CARTESIAN_POINT ( 'NONE',  ( 14.47279130897151589, 18.82499999726881157, 19.92008829642072953 ) ) ;
#28607=CARTESIAN_POINT ( 'NONE',  ( -10.04305231718579172, 5.599999999999994316, -30.90933677959248982 ) ) ;
#28608=DIRECTION ( 'NONE',  ( -0.000000000000000000, -1.000000000000000000, -0.000000000000000000 ) ) ;
#28610=CARTESIAN_POINT ( 'NONE',  ( 33.58253175000000823, 50.02500000273118985, 10.91162601494192863 ) ) ;
#28612=CARTESIAN_POINT ( 'NONE',  ( 33.58253175000000823, 44.27500000273120406, 10.91162601494192685 ) ) ;
#28613=( BOUNDED_SURFACE ( )  B_SPLINE_SURFACE ( 1, 2, ( 
 ( #6370, #872, #13933, #11681, #26962, #6540, #19252, #32607, #17012, #1543, #27473, #29692, #1375, #11850, #22329, #9106, #29869, #6198, #32774, #17185, #4131, #11352, #3961, #9437, #19587, #24559, #32441, #21993, #16678, #3463, #14606, #12019, #9268, #21830, #22488, #14103, #27134, #27304, #22165, #30035, #1033, #3629, #19752, #16848, #30200, #6702, #32276, #27643, #32939, #8942, #29528, #8769, #6031, #16510, #11513, #19420, #3795, #14268, #24725, #1200, #7212, #22834, #4641, #25238, #30717, #20099, #17695, #20441, #6870, #25584, #4471, #20622, #10140, #30370, #7041, #15290, #9966, #28322, #30892, #12540, #15120, #14945, #28155, #25750, #2064, #23011, #33115, #7387, #2234, #30545, #14773, #17871, #9617, #17524, #33466, #27984, #25411, #1889, #1713, #12366, #4811, #12709, #27814, #23180, #17351, #33643, #31064, #33294, #19924, #4298, #22662, #9794, #12191, #20270, #22428, #27075, #14209, #30479, #6642, #9375, #24830, #1649, #6808, #11459, #16786, #12125, #19364, #17287, #27413, #27750, #1484, #19855, #6309, #11958, #20033, #29976, #19692, #30309, #9048, #4238, #24502, #17121, #16621, #22104, #32384, #3569, #6482, #22597, #14041, #25170, #976, #3738, #9208, #14543, #32876, #22270, #3902, #30138, #8879, #11791, #24664, #32712, #14712, #21933, #27579, #19527, #29808, #9554, #27245, #1139, #33049, #11621, #32549, #16954, #4068, #25002, #14372, #1309, #18152, #23114, #33577 ),
 ( #10075, #17805, #1823, #25344, #20556, #4406, #17981, #30651, #31002, #28431, #2524, #4921, #7148, #12820, #23292, #33760, #7499, #7320, #17630, #10252, #28594, #20894, #15401, #12476, #12643, #22946, #5093, #20378, #25857, #27923, #15226, #4747, #2346, #14883, #20733, #31173, #6980, #9901, #7665, #12301, #17463, #25522, #22773, #15579, #25689, #33926, #28263, #26031, #33226, #2170, #12993, #28091, #9725, #23464, #4579, #10416, #20211, #15057, #30827, #2001, #33404, #19205, #1151, #24677, #21943, #29642, #6819, #27763, #1495, #16630, #17301, #16799, #32393, #29988, #14386, #24843, #27256, #19373, #22282, #19540, #6654, #11971, #24514, #30150, #1321, #11633, #22441, #11469, #27590, #22116, #4080, #29818, #8888, #6323, #11804, #6492, #16965, #27423, #8721, #3914, #27086, #3747, #14724, #32727, #30323, #6145, #9220, #32887, #14221, #3580, #25015, #14052, #9386, #984, #4249, #25185, #19704, #17137, #1662, #12137, #19870, #14554, #32231, #32560, #9059, #25701, #2182, #33239, #20390, #12656, #9913, #20046, #20745, #20569, #25358, #30842, #5106, #23306, #28104, #17474, #7678, #1836, #33590, #12489, #4761, #33416, #15238, #7333, #27935, #6992, #23125, #30491, #10091, #12314, #31013, #7511, #18164, #17995, #22786, #28441, #4932, #15414, #25869, #22958, #9737, #2359, #10263, #2537, #12832, #4591, #28274, #15067, #31188, #2014, #33772, #9568, #17817, #28606, #15590, #4419, #26042 ) ),
 .UNSPECIFIED., .F., .F., .T. ) 
 B_SPLINE_SURFACE_WITH_KNOTS ( ( 2, 2 ),
 ( 3, 2, 2, 2, 2, 2, 2, 2, 2, 2, 2, 2, 2, 2, 2, 2, 2, 2, 2, 2, 2, 2, 2, 2, 2, 2, 2, 2, 2, 2, 2, 2, 2, 2, 2, 2, 2, 2, 2, 2, 2, 2, 2, 2, 2, 2, 2, 2, 2, 2, 2, 2, 2, 2, 2, 2, 2, 2, 2, 2, 2, 2, 2, 2, 2, 2, 2, 2, 2, 2, 2, 2, 2, 2, 2, 2, 2, 2, 2, 2, 2, 2, 2, 2, 2, 2, 2, 2, 2, 2, 3 ),
 ( 0.000000000000000000, 1.000000000000000000 ),
 ( 0.000000000000000000, 0.01111111111111111154, 0.02222222222222222307, 0.03333333333333333287, 0.04444444444444444614, 0.05555555555555555247, 0.06666666666666666574, 0.07777777777777777901, 0.08888888888888889228, 0.1000000000000000056, 0.1111111111111111049, 0.1222222222222222182, 0.1333333333333333315, 0.1444444444444444309, 0.1555555555555555580, 0.1666666666666666574, 0.1777777777777777846, 0.1888888888888888840, 0.2000000000000000111, 0.2111111111111111105, 0.2222222222222222099, 0.2333333333333333370, 0.2444444444444444364, 0.2555555555555555358, 0.2666666666666666630, 0.2777777777777777901, 0.2888888888888888618, 0.2999999999999999889, 0.3111111111111111160, 0.3222222222222222432, 0.3333333333333333148, 0.3444444444444444420, 0.3555555555555555691, 0.3666666666666666408, 0.3777777777777777679, 0.3888888888888888951, 0.4000000000000000222, 0.4111111111111110938, 0.4222222222222222210, 0.4333333333333333481, 0.4444444444444444198, 0.4555555555555555469, 0.4666666666666666741, 0.4777777777777778012, 0.4888888888888888729, 0.5000000000000000000, 0.5111111111111110716, 0.5222222222222222543, 0.5333333333333333259, 0.5444444444444443976, 0.5555555555555555802, 0.5666666666666666519, 0.5777777777777777235, 0.5888888888888889062, 0.5999999999999999778, 0.6111111111111111605, 0.6222222222222222321, 0.6333333333333333037, 0.6444444444444444864, 0.6555555555555555580, 0.6666666666666666297, 0.6777777777777778123, 0.6888888888888888840, 0.6999999999999999556, 0.7111111111111111382, 0.7222222222222222099, 0.7333333333333332815, 0.7444444444444444642, 0.7555555555555555358, 0.7666666666666667185, 0.7777777777777777901, 0.7888888888888888618, 0.8000000000000000444, 0.8111111111111111160, 0.8222222222222221877, 0.8333333333333333703, 0.8444444444444444420, 0.8555555555555555136, 0.8666666666666666963, 0.8777777777777777679, 0.8888888888888888395, 0.9000000000000000222, 0.9111111111111110938, 0.9222222222222222765, 0.9333333333333333481, 0.9444444444444444198, 0.9555555555555556024, 0.9666666666666666741, 0.9777777777777777457, 0.9888888888888889284, 1.000000000000000000 ),
 .UNSPECIFIED. ) 
 GEOMETRIC_REPRESENTATION_ITEM ( )  RATIONAL_B_SPLINE_SURFACE ( (
 ( 1.000000000000000000, 0.9510565162951535312, 1.000000000000000000, 0.9510565162951535312, 1.000000000000000000, 0.9510565162951535312, 1.000000000000000000, 0.9510565162951535312, 1.000000000000000000, 0.9510565162951535312, 1.000000000000000000, 0.9510565162951535312, 1.000000000000000000, 0.9510565162951535312, 1.000000000000000000, 0.9510565162951535312, 1.000000000000000000, 0.9510565162951535312, 1.000000000000000000, 0.9510565162951535312, 1.000000000000000000, 0.9510565162951535312, 1.000000000000000000, 0.9510565162951535312, 1.000000000000000000, 0.9510565162951535312, 1.000000000000000000, 0.9510565162951535312, 1.000000000000000000, 0.9510565162951535312, 1.000000000000000000, 0.9510565162951535312, 1.000000000000000000, 0.9510565162951535312, 1.000000000000000000, 0.9510565162951535312, 1.000000000000000000, 0.9510565162951535312, 1.000000000000000000, 0.9510565162951535312, 1.000000000000000000, 0.9510565162951535312, 1.000000000000000000, 0.9510565162951535312, 1.000000000000000000, 0.9510565162951535312, 1.000000000000000000, 0.9510565162951535312, 1.000000000000000000, 0.9510565162951535312, 1.000000000000000000, 0.9510565162951535312, 1.000000000000000000, 0.9510565162951535312, 1.000000000000000000, 0.9510565162951535312, 1.000000000000000000, 0.9510565162951535312, 1.000000000000000000, 0.9510565162951535312, 1.000000000000000000, 0.9510565162951535312, 1.000000000000000000, 0.9510565162951535312, 1.000000000000000000, 0.9510565162951535312, 1.000000000000000000, 0.9510565162951535312, 1.000000000000000000, 0.9510565162951535312, 1.000000000000000000, 0.9510565162951535312, 1.000000000000000000, 0.9510565162951535312, 1.000000000000000000, 0.9510565162951535312, 1.000000000000000000, 0.9510565162951535312, 1.000000000000000000, 0.9510565162951535312, 1.000000000000000000, 0.9510565162951535312, 1.000000000000000000, 0.9510565162951535312, 1.000000000000000000, 0.9510565162951535312, 1.000000000000000000, 0.9510565162951535312, 1.000000000000000000, 0.9510565162951535312, 1.000000000000000000, 0.9510565162951535312, 1.000000000000000000, 0.9510565162951535312, 1.000000000000000000, 0.9510565162951535312, 1.000000000000000000, 0.9510565162951535312, 1.000000000000000000, 0.9510565162951535312, 1.000000000000000000, 0.9510565162951535312, 1.000000000000000000, 0.9510565162951535312, 1.000000000000000000, 0.9510565162951535312, 1.000000000000000000, 0.9510565162951535312, 1.000000000000000000, 0.9510565162951535312, 1.000000000000000000, 0.9510565162951535312, 1.000000000000000000, 0.9510565162951535312, 1.000000000000000000, 0.9510565162951535312, 1.000000000000000000, 0.9510565162951535312, 1.000000000000000000, 0.9510565162951535312, 1.000000000000000000, 0.9510565162951535312, 1.000000000000000000, 0.9510565162951535312, 1.000000000000000000, 0.9510565162951535312, 1.000000000000000000, 0.9510565162951535312, 1.000000000000000000, 0.9510565162951535312, 1.000000000000000000, 0.9510565162951535312, 1.000000000000000000, 0.9510565162951535312, 1.000000000000000000, 0.9510565162951535312, 1.000000000000000000, 0.9510565162951535312, 1.000000000000000000, 0.9510565162951535312, 1.000000000000000000, 0.9510565162951535312, 1.000000000000000000, 0.9510565162951535312, 1.000000000000000000, 0.9510565162951535312, 1.000000000000000000, 0.9510565162951535312, 1.000000000000000000, 0.9510565162951535312, 1.000000000000000000, 0.9510565162951535312, 1.000000000000000000, 0.9510565162951535312, 1.000000000000000000, 0.9510565162951535312, 1.000000000000000000, 0.9510565162951535312, 1.000000000000000000, 0.9510565162951535312, 1.000000000000000000, 0.9510565162951535312, 1.000000000000000000, 0.9510565162951535312, 1.000000000000000000, 0.9510565162951535312, 1.000000000000000000, 0.9510565162951535312, 1.000000000000000000, 0.9510565162951535312, 1.000000000000000000, 0.9510565162951535312, 1.000000000000000000, 0.9510565162951535312, 1.000000000000000000, 0.9510565162951535312, 1.000000000000000000, 0.9510565162951535312, 1.000000000000000000, 0.9510565162951535312, 1.000000000000000000),
 ( 1.000000000000000000, 0.9510565162951535312, 1.000000000000000000, 0.9510565162951535312, 1.000000000000000000, 0.9510565162951535312, 1.000000000000000000, 0.9510565162951535312, 1.000000000000000000, 0.9510565162951535312, 1.000000000000000000, 0.9510565162951535312, 1.000000000000000000, 0.9510565162951535312, 1.000000000000000000, 0.9510565162951535312, 1.000000000000000000, 0.9510565162951535312, 1.000000000000000000, 0.9510565162951535312, 1.000000000000000000, 0.9510565162951535312, 1.000000000000000000, 0.9510565162951535312, 1.000000000000000000, 0.9510565162951535312, 1.000000000000000000, 0.9510565162951535312, 1.000000000000000000, 0.9510565162951535312, 1.000000000000000000, 0.9510565162951535312, 1.000000000000000000, 0.9510565162951535312, 1.000000000000000000, 0.9510565162951535312, 1.000000000000000000, 0.9510565162951535312, 1.000000000000000000, 0.9510565162951535312, 1.000000000000000000, 0.9510565162951535312, 1.000000000000000000, 0.9510565162951535312, 1.000000000000000000, 0.9510565162951535312, 1.000000000000000000, 0.9510565162951535312, 1.000000000000000000, 0.9510565162951535312, 1.000000000000000000, 0.9510565162951535312, 1.000000000000000000, 0.9510565162951535312, 1.000000000000000000, 0.9510565162951535312, 1.000000000000000000, 0.9510565162951535312, 1.000000000000000000, 0.9510565162951535312, 1.000000000000000000, 0.9510565162951535312, 1.000000000000000000, 0.9510565162951535312, 1.000000000000000000, 0.9510565162951535312, 1.000000000000000000, 0.9510565162951535312, 1.000000000000000000, 0.9510565162951535312, 1.000000000000000000, 0.9510565162951535312, 1.000000000000000000, 0.9510565162951535312, 1.000000000000000000, 0.9510565162951535312, 1.000000000000000000, 0.9510565162951535312, 1.000000000000000000, 0.9510565162951535312, 1.000000000000000000, 0.9510565162951535312, 1.000000000000000000, 0.9510565162951535312, 1.000000000000000000, 0.9510565162951535312, 1.000000000000000000, 0.9510565162951535312, 1.000000000000000000, 0.9510565162951535312, 1.000000000000000000, 0.9510565162951535312, 1.000000000000000000, 0.9510565162951535312, 1.000000000000000000, 0.9510565162951535312, 1.000000000000000000, 0.9510565162951535312, 1.000000000000000000, 0.9510565162951535312, 1.000000000000000000, 0.9510565162951535312, 1.000000000000000000, 0.9510565162951535312, 1.000000000000000000, 0.9510565162951535312, 1.000000000000000000, 0.9510565162951535312, 1.000000000000000000, 0.9510565162951535312, 1.000000000000000000, 0.9510565162951535312, 1.000000000000000000, 0.9510565162951535312, 1.000000000000000000, 0.9510565162951535312, 1.000000000000000000, 0.9510565162951535312, 1.000000000000000000, 0.9510565162951535312, 1.000000000000000000, 0.9510565162951535312, 1.000000000000000000, 0.9510565162951535312, 1.000000000000000000, 0.9510565162951535312, 1.000000000000000000, 0.9510565162951535312, 1.000000000000000000, 0.9510565162951535312, 1.000000000000000000, 0.9510565162951535312, 1.000000000000000000, 0.9510565162951535312, 1.000000000000000000, 0.9510565162951535312, 1.000000000000000000, 0.9510565162951535312, 1.000000000000000000, 0.9510565162951535312, 1.000000000000000000, 0.9510565162951535312, 1.000000000000000000, 0.9510565162951535312, 1.000000000000000000, 0.9510565162951535312, 1.000000000000000000, 0.9510565162951535312, 1.000000000000000000, 0.9510565162951535312, 1.000000000000000000, 0.9510565162951535312, 1.000000000000000000, 0.9510565162951535312, 1.000000000000000000, 0.9510565162951535312, 1.000000000000000000, 0.9510565162951535312, 1.000000000000000000, 0.9510565162951535312, 1.000000000000000000, 0.9510565162951535312, 1.000000000000000000, 0.9510565162951535312, 1.000000000000000000, 0.9510565162951535312, 1.000000000000000000, 0.9510565162951535312, 1.000000000000000000, 0.9510565162951535312, 1.000000000000000000, 0.9510565162951535312, 1.000000000000000000, 0.9510565162951535312, 1.000000000000000000, 0.9510565162951535312, 1.000000000000000000, 0.9510565162951535312, 1.000000000000000000, 0.9510565162951535312, 1.000000000000000000) ) ) 
 REPRESENTATION_ITEM ( '' )  SURFACE ( )  );
#28614=CARTESIAN_POINT ( 'NONE',  ( 20.08610463437158344, 23.20000000546238539, 27.64615127144129403 ) ) ;
#28616=CARTESIAN_POINT ( 'NONE',  ( -26.29305231718578995, 62.20000000000000284, 19.10302069950538595 ) ) ;
#28618=( BOUNDED_CURVE ( )  B_SPLINE_CURVE ( 2, ( #16222, #8804, #16055, #23770, #18794, #13297, #26677, #6063, #238, #26509, #16546, #29238, #8143 ),
 .UNSPECIFIED., .F., .T. ) 
 B_SPLINE_CURVE_WITH_KNOTS ( ( 3, 2, 2, 2, 2, 2, 3 ),
 ( 0.6089743589743590313, 0.6102564102564103088, 0.6128205128205128638, 0.6153846153846154188, 0.6179487179487179738, 0.6205128205128205288, 0.6217948717948718063 ),
 .UNSPECIFIED. ) 
 CURVE ( )  GEOMETRIC_REPRESENTATION_ITEM ( )  RATIONAL_B_SPLINE_CURVE ( ( 0.9755282581475768211, 0.9755282581475778203, 1.000000000000000000, 0.9510565162951535312, 1.000000000000000000, 0.9510565162951535312, 1.000000000000000000, 0.9510565162951535312, 1.000000000000000000, 0.9510565162951535312, 1.000000000000000000, 0.9755282581475768211, 0.9755282581475768211 ) ) 
 REPRESENTATION_ITEM ( '' )  );
#28621=CARTESIAN_POINT ( 'NONE',  ( 20.08610463437157279, 7.300000000000001599, -27.64615127144129758 ) ) ;
#28626=CARTESIAN_POINT ( 'NONE',  ( 15.14183272437242067, 17.44999999453764516, 20.84094480462498211 ) ) ;
#28627=CARTESIAN_POINT ( 'NONE',  ( -27.16883889988624290, 26.92500000273118133, -19.73931689729374028 ) ) ;
#28635=VECTOR ( 'NONE', #25198, 1000.000000000000000 ) ;
#28636=VERTEX_POINT ( 'NONE', #22738 ) ;
#28639=CARTESIAN_POINT ( 'NONE',  ( -4.523095164977116484E-15, 2.124999997268812280, 24.62258325217400312 ) ) ;
#28640=CARTESIAN_POINT ( 'NONE',  ( -33.58253175000000113, 35.37500000273119127, 0.000000000000000000 ) ) ;
#28641=CARTESIAN_POINT ( 'NONE',  ( 20.08610463437158344, 37.20000000546237118, 27.64615127144129403 ) ) ;
#28643=CARTESIAN_POINT ( 'NONE',  ( 27.16883889988624290, 25.92500000273118133, 19.73931689729373673 ) ) ;
#28644=CARTESIAN_POINT ( 'NONE',  ( 15.14183272437242422, 6.049999994537626158, -20.84094480462497856 ) ) ;
#28645=CARTESIAN_POINT ( 'NONE',  ( -33.58253175000000113, 51.37500000273120548, 0.000000000000000000 ) ) ;
#28647=EDGE_CURVE ( 'NONE', #15956, #5936, #17766, .T. ) ;
#28649=CARTESIAN_POINT ( 'NONE',  ( 20.08610463437158344, 28.69999999999999574, 27.64615127144129403 ) ) ;
#28651=CARTESIAN_POINT ( 'NONE',  ( 33.58253175000000113, 70.22500000273120691, -10.91162601494193751 ) ) ;
#28653=CARTESIAN_POINT ( 'NONE',  ( -20.08610463437156923, 20.80000000546236905, 27.64615127144130113 ) ) ;
#28654=CARTESIAN_POINT ( 'NONE',  ( 20.75514604977249178, 62.07500000273119412, 28.56700777964553950 ) ) ;
#28655=EDGE_CURVE ( 'NONE', #15993, #23029, #12610, .T. ) ;
#28657=CARTESIAN_POINT ( 'NONE',  ( -5.147494310547430452, 40.05125428700921475, -32.49999999999999289 ) ) ;
#28658=CARTESIAN_POINT ( 'NONE',  ( 10.37757302488624056, 14.52500000273118630, -31.93888565452638417 ) ) ;
#28662=CARTESIAN_POINT ( 'NONE',  ( 10.37757302488624767, 1.975000002731180926, 31.93888565452638417 ) ) ;
#28664=CARTESIAN_POINT ( 'NONE',  ( 26.29305231718579350, 45.30000000546238681, 19.10302069950537529 ) ) ;
#28666=VECTOR ( 'NONE', #182, 1000.000000000000000 ) ;
#28667=EDGE_CURVE ( 'NONE', #27108, #25557, #4970, .T. ) ;
#28674=CARTESIAN_POINT ( 'NONE',  ( -20.08610463437156923, 70.80000000546235128, 27.64615127144130113 ) ) ;
#28683=CARTESIAN_POINT ( 'NONE',  ( -20.75514604977248112, 55.67500000273118843, 28.56700777964554661 ) ) ;
#28684=CARTESIAN_POINT ( 'NONE',  ( 26.29305231718579350, 55.30000000546236549, 19.10302069950537529 ) ) ;
#28686=CARTESIAN_POINT ( 'NONE',  ( -20.75514604977248112, 41.42500000273118133, 28.56700777964554661 ) ) ;
#28688=CARTESIAN_POINT ( 'NONE',  ( -27.16883889988624290, 71.17500000273119554, -19.73931689729374028 ) ) ;
#28693=CARTESIAN_POINT ( 'NONE',  ( -26.29305231718578995, 46.19999999999998863, 19.10302069950538595 ) ) ;
#28695=CARTESIAN_POINT ( 'NONE',  ( -10.37757302488624411, 10.97500000273118914, -31.93888565452638417 ) ) ;
#28696=CARTESIAN_POINT ( 'NONE',  ( 5.147494310547434893, 35.05125428700922896, 32.49999999999999289 ) ) ;
#28698=CARTESIAN_POINT ( 'NONE',  ( 13.91746825000000065, 80.27500000273117564, 4.522059556121114987 ) ) ;
#28699=CARTESIAN_POINT ( 'NONE',  ( 33.58253175000000823, 78.27500000273117564, 10.91162601494192685 ) ) ;
#28700=FACE_BOUND ( 'NONE', #1093, .T. ) ;
#28712=EDGE_CURVE ( 'NONE', #4197, #12209, #9650, .T. ) ;
#28713=DIRECTION ( 'NONE',  ( 0.000000000000000000, 0.000000000000000000, -1.000000000000000000 ) ) ;
#28715=CARTESIAN_POINT ( 'NONE',  ( -20.75514604977248112, 41.42500000273118133, 28.56700777964554661 ) ) ;
#28717=CARTESIAN_POINT ( 'NONE',  ( -26.29305231718579350, 2.300000005462377040, -19.10302069950537884 ) ) ;
#28718=VERTEX_POINT ( 'NONE', #12742 ) ;
#28720=( BOUNDED_CURVE ( )  B_SPLINE_CURVE ( 2, ( #24595, #23646, #5277, #15761, #26214, #108, #10599, #21077, #31525, #8019, #1578, #25101, #14303 ),
 .UNSPECIFIED., .F., .F. ) 
 B_SPLINE_CURVE_WITH_KNOTS ( ( 3, 2, 2, 2, 2, 2, 3 ),
 ( 0.6944444444444444198, 0.6999999999999999556, 0.7111111111111111382, 0.7222222222222222099, 0.7333333333333332815, 0.7444444444444444642, 0.7500000000000000000 ),
 .UNSPECIFIED. ) 
 CURVE ( )  GEOMETRIC_REPRESENTATION_ITEM ( )  RATIONAL_B_SPLINE_CURVE ( ( 0.9755282581475768211, 0.9755282581475768211, 1.000000000000000000, 0.9510565162951535312, 1.000000000000000000, 0.9510565162951535312, 1.000000000000000000, 0.9510565162951535312, 1.000000000000000000, 0.9510565162951535312, 1.000000000000000000, 0.9755282581475768211, 0.9755282581475768211 ) ) 
 REPRESENTATION_ITEM ( '' )  );
#28721=CARTESIAN_POINT ( 'NONE',  ( 3.980102097228898626E-15, 80.00000000000001421, 32.50000000000000000 ) ) ;
#28723=CARTESIAN_POINT ( 'NONE',  ( -10.37757302488624411, 76.97500000273119269, -31.93888565452638417 ) ) ;
#28728=CARTESIAN_POINT ( 'NONE',  ( -20.08610463437156923, 14.80000000546238503, 27.64615127144130113 ) ) ;
#28729=CARTESIAN_POINT ( 'NONE',  ( 10.37757302488624767, 59.72500000273117848, 31.93888565452638417 ) ) ;
#28731=CARTESIAN_POINT ( 'NONE',  ( -15.14183272437241889, 16.69999999999999574, -20.84094480462497856 ) ) ;
#28732=CARTESIAN_POINT ( 'NONE',  ( 23.41746824999999887, 3.024999997268813079, 7.608796670333735079 ) ) ;
#28733=CARTESIAN_POINT ( 'NONE',  ( -33.58253175000000113, 3.025000002731199622, -10.91162601494193218 ) ) ;
#28738=CARTESIAN_POINT ( 'NONE',  ( 20.08610463437158344, 75.20000000546239960, 27.64615127144129403 ) ) ;
#28742=CARTESIAN_POINT ( 'NONE',  ( 12.13525491562421088, 71.05000000546237970, 8.816778784387095058 ) ) ;
#28744=CARTESIAN_POINT ( 'NONE',  ( -2.162160676586881955E-15, 30.62500000273119838, -35.31076352940723240 ) ) ;
#28747=CARTESIAN_POINT ( 'NONE',  ( -27.16883889988623935, 13.57500000273120833, 19.73931689729374739 ) ) ;
#28748=CARTESIAN_POINT ( 'NONE',  ( -15.00000000000000000, 80.00000000000001421, 0.000000000000000000 ) ) ;
#28750=CARTESIAN_POINT ( 'NONE',  ( -33.58253175000000113, 73.12500000273119838, 0.000000000000000000 ) ) ;
#28751=CARTESIAN_POINT ( 'NONE',  ( -26.29305231718579350, 26.30000000546236905, -19.10302069950537884 ) ) ;
#28752=ADVANCED_FACE ( 'NONE', ( #15325 ), #17555, .T. ) ;
#28754=DIRECTION ( 'NONE',  ( 0.8660254037844399289, -0.4999999999999977240, 0.000000000000000000 ) ) ;
#28755=CARTESIAN_POINT ( 'NONE',  ( -20.75514604977248112, 65.42500000273116711, 28.56700777964554661 ) ) ;
#28756=ADVANCED_FACE ( 'NONE', ( #15151 ), #17904, .T. ) ;
#28760=CARTESIAN_POINT ( 'NONE',  ( 20.75514604977248467, 6.425000002731179549, -28.56700777964554305 ) ) ;
#28761=CARTESIAN_POINT ( 'NONE',  ( 7.236395654485755280, 2.224999997268800378, 22.27133577429736988 ) ) ;
#28763=VERTEX_POINT ( 'NONE', #2269 ) ;
#28765=ORIENTED_EDGE ( 'NONE', *, *, #32489, .T. ) ;
#28769=CARTESIAN_POINT ( 'NONE',  ( 20.75514604977249178, 77.82500000273120122, 28.56700777964553950 ) ) ;
#28771=CARTESIAN_POINT ( 'NONE',  ( 24.50000000000000355, 1.899999999999998135, 7.960532557706212486 ) ) ;
#28772=CARTESIAN_POINT ( 'NONE',  ( -2.162160676586881955E-15, 12.87500000273117884, -35.31076352940723240 ) ) ;
#28773=CARTESIAN_POINT ( 'NONE',  ( 20.08610463437157279, 59.30000000000001847, -27.64615127144129758 ) ) ;
#28774=CARTESIAN_POINT ( 'NONE',  ( 5.147494310547426899, 57.94874572391552192, -32.50000000000000000 ) ) ;
#28775=CARTESIAN_POINT ( 'NONE',  ( 5.779280353836490358E-15, 50.50000000000000000, 32.49999999999999289 ) ) ;
#28777=CARTESIAN_POINT ( 'NONE',  ( -13.91746824999999532, 73.27500000273118985, -4.522059556121115875 ) ) ;
#28780=DIRECTION ( 'NONE',  ( -0.000000000000000000, -1.000000000000000000, -0.000000000000000000 ) ) ;
#28781=CARTESIAN_POINT ( 'NONE',  ( -33.58253175000000113, 79.27500000273118985, -10.91162601494193218 ) ) ;
#28782=CARTESIAN_POINT ( 'NONE',  ( 20.08610463437158344, 17.20000000546236762, 27.64615127144129403 ) ) ;
#28784=CARTESIAN_POINT ( 'NONE',  ( -2.162160676586881955E-15, 48.62500000273118417, -35.31076352940723240 ) ) ;
#28786=CARTESIAN_POINT ( 'NONE',  ( -33.58253175000000113, 33.47500000273119269, 10.91162601494193929 ) ) ;
#28787=CARTESIAN_POINT ( 'NONE',  ( 5.147494310547434893, 23.05125428700921830, 32.49999999999999289 ) ) ;
#28790=CARTESIAN_POINT ( 'NONE',  ( -10.04305231718579172, 22.10000000546236265, -30.90933677959248982 ) ) ;
#28793=CARTESIAN_POINT ( 'NONE',  ( 32.50000000000000000, 7.000000000000006217, -3.980102097228898626E-15 ) ) ;
#28794=LINE ( 'NONE', #25881, #19388 ) ;
#28797=ADVANCED_FACE ( 'NONE', ( #28519 ), #7071, .T. ) ;
#28800=CARTESIAN_POINT ( 'NONE',  ( 10.04305231718579705, 10.59999999999999787, 30.90933677959248982 ) ) ;
#28801=CARTESIAN_POINT ( 'NONE',  ( -27.16883889988624290, 24.92500000273117777, -19.73931689729374028 ) ) ;
#28803=ORIENTED_EDGE ( 'NONE', *, *, #22998, .T. ) ;
#28805=AXIS2_PLACEMENT_3D ( 'NONE', #14362, #9541, #32865 ) ;
#28810=FACE_OUTER_BOUND ( 'NONE', #27919, .T. ) ;
#28811=CARTESIAN_POINT ( 'NONE',  ( -33.58253175000000113, 37.47500000273118559, 10.91162601494193929 ) ) ;
#28812=CARTESIAN_POINT ( 'NONE',  ( -20.08610463437157989, 36.20000000546237828, -27.64615127144129758 ) ) ;
#28816=CARTESIAN_POINT ( 'NONE',  ( -10.37757302488624411, 20.72500000273119625, -31.93888565452638417 ) ) ;
#28817=CARTESIAN_POINT ( 'NONE',  ( 2.067204126564591252E-14, 6.249999994537623671, -24.50000000000000000 ) ) ;
#28818=CARTESIAN_POINT ( 'NONE',  ( 27.16883889988623935, 48.57500000273118701, -19.73931689729374384 ) ) ;
#28820=CARTESIAN_POINT ( 'NONE',  ( -32.50000000000000000, 26.09999999999999076, 10.55989012756946366 ) ) ;
#28822=CARTESIAN_POINT ( 'NONE',  ( -2.162160676586881955E-15, 70.62500000273118417, -35.31076352940723240 ) ) ;
#28824=CARTESIAN_POINT ( 'NONE',  ( -5.147494310547430452, 37.55125428154684641, -32.49999999999999289 ) ) ;
#28825=CARTESIAN_POINT ( 'NONE',  ( -33.58253175000000113, 57.27500000273120406, -10.91162601494193041 ) ) ;
#28826=CARTESIAN_POINT ( 'NONE',  ( -1.778240108872766143E-15, 8.000000005462370112, -32.49999999999999289 ) ) ;
#28827=CARTESIAN_POINT ( 'NONE',  ( 33.58253175000000113, 12.22500000273120158, -10.91162601494193751 ) ) ;
#28830=CARTESIAN_POINT ( 'NONE',  ( -33.58253175000000113, 1.375000002731191495, 0.000000000000000000 ) ) ;
#28840=CARTESIAN_POINT ( 'NONE',  ( -32.50000000000000000, 53.99999999999999289, 0.000000000000000000 ) ) ;
#28841=CARTESIAN_POINT ( 'NONE',  ( 32.50000000000000000, 69.60000000546236265, -10.55989012756945833 ) ) ;
#28845=VERTEX_POINT ( 'NONE', #20863 ) ;
#28850=CARTESIAN_POINT ( 'NONE',  ( -27.16883889988623935, 55.57500000273118701, 19.73931689729374739 ) ) ;
#28851=CARTESIAN_POINT ( 'NONE',  ( 20.08610463437157279, 57.80000000546236549, -27.64615127144129758 ) ) ;
#28854=CARTESIAN_POINT ( 'NONE',  ( 20.75514604977248467, 40.42500000273117422, -28.56700777964554305 ) ) ;
#28855=CARTESIAN_POINT ( 'NONE',  ( 32.50000000000000000, 54.99999999999999289, -3.980102097228898626E-15 ) ) ;
#28856=CARTESIAN_POINT ( 'NONE',  ( 27.16883889988623935, 70.57500000273120122, -19.73931689729374384 ) ) ;
#28857=CARTESIAN_POINT ( 'NONE',  ( -20.08610463437157989, 2.200000005462375618, -27.64615127144129758 ) ) ;
#28861=CARTESIAN_POINT ( 'NONE',  ( -20.08610463437156923, 48.30000000000001847, 27.64615127144130113 ) ) ;
#28863=CARTESIAN_POINT ( 'NONE',  ( -33.58253175000000113, 13.27500000273119518, -10.91162601494193218 ) ) ;
#28867=CARTESIAN_POINT ( 'NONE',  ( 20.75514604977248467, 78.67500000273116711, -28.56700777964554305 ) ) ;
#28868=PLANE ( 'NONE',  #15580 ) ;
#28870=ORIENTED_EDGE ( 'NONE', *, *, #4613, .T. ) ;
#28882=CARTESIAN_POINT ( 'NONE',  ( -33.58253175000000113, 37.12500000273119838, 0.000000000000000000 ) ) ;
#28885=ORIENTED_EDGE ( 'NONE', *, *, #5798, .F. ) ;
#28887=CARTESIAN_POINT ( 'NONE',  ( 32.50000000000000000, 51.09999999999998721, -10.55989012756945833 ) ) ;
#28889=CARTESIAN_POINT ( 'NONE',  ( -2.162160676586881955E-15, 74.87500000273116996, -35.31076352940723240 ) ) ;
#28892=ORIENTED_EDGE ( 'NONE', *, *, #6119, .T. ) ;
#28893=CARTESIAN_POINT ( 'NONE',  ( 26.29305231718578995, 29.70000000546238539, -19.10302069950538240 ) ) ;
#28894=CARTESIAN_POINT ( 'NONE',  ( 20.75514604977249178, 61.82500000273116569, 28.56700777964553950 ) ) ;
#28898=CARTESIAN_POINT ( 'NONE',  ( 7.236395654485755280, 8.724999997268806595, 22.27133577429736988 ) ) ;
#28899=CARTESIAN_POINT ( 'NONE',  ( 20.75514604977249178, 1.825000002731179460, 28.56700777964553950 ) ) ;
#28900=CARTESIAN_POINT ( 'NONE',  ( 33.58253175000000113, 32.47500000273117138, -10.91162601494193751 ) ) ;
#28903=CARTESIAN_POINT ( 'NONE',  ( 5.779280353836490358E-15, 36.49999999999998579, 32.49999999999999289 ) ) ;
#28904=CARTESIAN_POINT ( 'NONE',  ( 4.300734207923757602, 78.27500000273118985, -13.23629886949340673 ) ) ;
#28908=CARTESIAN_POINT ( 'NONE',  ( 15.00000000000000000, 73.35000000546237686, -4.873795443493596835 ) ) ;
#28910=CARTESIAN_POINT ( 'NONE',  ( 33.58253175000000113, 22.22500000273117493, -10.91162601494193751 ) ) ;
#28913=CARTESIAN_POINT ( 'NONE',  ( 33.58253175000000823, 14.27500000273119340, 10.91162601494192685 ) ) ;
#28914=CARTESIAN_POINT ( 'NONE',  ( -4.223320258572821363E-15, 80.49999999999998579, 15.00000000000000355 ) ) ;
#28916=CARTESIAN_POINT ( 'NONE',  ( -4.223320258572819786E-15, 15.24999999453762278, 24.50000000000000000 ) ) ;
#28918=( BOUNDED_CURVE ( )  B_SPLINE_CURVE ( 2, ( #33559, #25840, #10059, #7484, #4903, #15384, #29252, #5587, #10738, #3186, #29745, #32327, #18645 ),
 .UNSPECIFIED., .F., .T. ) 
 B_SPLINE_CURVE_WITH_KNOTS ( ( 3, 2, 2, 2, 2, 2, 3 ),
 ( 0.2371794871794871973, 0.2384615384615384748, 0.2410256410256410298, 0.2435897435897435848, 0.2461538461538461675, 0.2487179487179487225, 0.2500000000000000000 ),
 .UNSPECIFIED. ) 
 CURVE ( )  GEOMETRIC_REPRESENTATION_ITEM ( )  RATIONAL_B_SPLINE_CURVE ( ( 0.9755282581475768211, 0.9755282581475770431, 1.000000000000000000, 0.9510565162951535312, 1.000000000000000000, 0.9510565162951535312, 1.000000000000000000, 0.9510565162951535312, 1.000000000000000000, 0.9510565162951535312, 1.000000000000000000, 0.9755282581475768211, 0.9755282581475768211 ) ) 
 REPRESENTATION_ITEM ( '' )  );
#28920=LINE ( 'NONE', #5420, #2952 ) ;
#28921=CARTESIAN_POINT ( 'NONE',  ( -10.37757302488624411, 58.72500000273117848, -31.93888565452638417 ) ) ;
#28924=EDGE_LOOP ( 'NONE', ( #30917, #7493, #10685, #24702 ) ) ;
#28926=CARTESIAN_POINT ( 'NONE',  ( 27.16883889988623935, 4.325000002731171911, -19.73931689729374384 ) ) ;
#28927=CARTESIAN_POINT ( 'NONE',  ( 14.47279130897151767, 17.42499999726882365, -19.92008829642072598 ) ) ;
#28932=ORIENTED_EDGE ( 'NONE', *, *, #10321, .F. ) ;
#28934=CARTESIAN_POINT ( 'NONE',  ( 26.29305231718579350, 11.30000000546238503, 19.10302069950537529 ) ) ;
#28936=CARTESIAN_POINT ( 'NONE',  ( -33.58253175000000113, 79.12500000273119838, 0.000000000000000000 ) ) ;
#28938=CARTESIAN_POINT ( 'NONE',  ( -18.94512977948576093, 15.82499999726880091, 13.76444248337722698 ) ) ;
#28939=CARTESIAN_POINT ( 'NONE',  ( -33.58253175000000113, 9.375000002731169957, 0.000000000000000000 ) ) ;
#28940=ADVANCED_FACE ( 'NONE', ( #17952 ), #25997, .T. ) ;
#28941=CARTESIAN_POINT ( 'NONE',  ( 26.29305231718578995, 61.20000000000000284, -19.10302069950538240 ) ) ;
#28942=CARTESIAN_POINT ( 'NONE',  ( 26.29305231718578995, 57.70000000546238539, -19.10302069950538240 ) ) ;
#28943=CARTESIAN_POINT ( 'NONE',  ( -32.50000000000000000, 30.10000000000000853, 10.55989012756946366 ) ) ;
#28945=CARTESIAN_POINT ( 'NONE',  ( -13.91746824999999532, 77.27500000273117564, -4.522059556121115875 ) ) ;
#28949=FACE_OUTER_BOUND ( 'NONE', #23759, .T. ) ;
#28950=CARTESIAN_POINT ( 'NONE',  ( -15.14183272437242778, 1.299999999999988054, 20.84094480462497856 ) ) ;
#28951=CARTESIAN_POINT ( 'NONE',  ( 20.08610463437157279, 3.299999999999983391, -27.64615127144129758 ) ) ;
#28955=CARTESIAN_POINT ( 'NONE',  ( 10.37757302488624056, 50.52500000273118985, -31.93888565452638417 ) ) ;
#28958=CARTESIAN_POINT ( 'NONE',  ( -10.37757302488623701, 31.77500000273120051, 31.93888565452638417 ) ) ;
#28959=CARTESIAN_POINT ( 'NONE',  ( 0.000000000000000000, 0.000000000000000000, 0.000000000000000000 ) ) ;
#28961=CARTESIAN_POINT ( 'NONE',  ( 20.08610463437158344, 15.20000000546237118, 27.64615127144129403 ) ) ;
#28962=DIRECTION ( 'NONE',  ( 0.000000000000000000, 1.000000000000000000, 0.000000000000000000 ) ) ;
#28965=CARTESIAN_POINT ( 'NONE',  ( 7.236395654485760609, 1.024999997268821739, -22.27133577429736633 ) ) ;
#28966=CARTESIAN_POINT ( 'NONE',  ( 19.82091636218621389, 12.19999999999998863, -14.40073868116559197 ) ) ;
#28969=CARTESIAN_POINT ( 'NONE',  ( -5.147494310547423346, 12.44874571845314115, 32.50000000000000000 ) ) ;
#28970=CARTESIAN_POINT ( 'NONE',  ( 33.58253175000000113, 28.22500000273118914, -10.91162601494193574 ) ) ;
#28974=ORIENTED_EDGE ( 'NONE', *, *, #32075, .T. ) ;
#28978=EDGE_LOOP ( 'NONE', ( #7363, #14964, #1778, #29709 ) ) ;
#28979=CARTESIAN_POINT ( 'NONE',  ( 18.94512977948575738, 2.424999997268806329, 13.76444248337723408 ) ) ;
#28980=CARTESIAN_POINT ( 'NONE',  ( 10.37757302488624056, 32.77500000273120406, -31.93888565452638417 ) ) ;
#28981=CARTESIAN_POINT ( 'NONE',  ( -2.092463501923844636E-15, 36.00000000546238255, -34.17252228774368916 ) ) ;
#28984=CARTESIAN_POINT ( 'NONE',  ( -1.778240108872766143E-15, 54.00000000546237544, -32.49999999999999289 ) ) ;
#28985=CARTESIAN_POINT ( 'NONE',  ( 33.58253175000000113, 46.47500000273118559, -10.91162601494193751 ) ) ;
#28988=CARTESIAN_POINT ( 'NONE',  ( -10.04305231718579172, 23.60000000000000853, -30.90933677959248982 ) ) ;
#28990=CARTESIAN_POINT ( 'NONE',  ( -10.37757302488624411, 66.72500000273117848, -31.93888565452638417 ) ) ;
#28992=CARTESIAN_POINT ( 'NONE',  ( -10.04305231718579172, 37.59999999999999432, -30.90933677959248982 ) ) ;
#28993=CARTESIAN_POINT ( 'NONE',  ( -27.16883889988624290, 53.17500000273117422, -19.73931689729374028 ) ) ;
#28994=CARTESIAN_POINT ( 'NONE',  ( -33.58253175000000113, 13.02500000273117564, -10.91162601494193218 ) ) ;
#28996=CARTESIAN_POINT ( 'NONE',  ( 15.14183272437242422, 2.049999994537635484, -20.84094480462497856 ) ) ;
#28999=CARTESIAN_POINT ( 'NONE',  ( 5.147494310547327423, 45.05125428700921475, 32.50000000000003553 ) ) ;
#29005=DIRECTION ( 'NONE',  ( -0.000000000000000000, -1.000000000000000000, -0.000000000000000000 ) ) ;
#29007=CARTESIAN_POINT ( 'NONE',  ( -23.41746825000000598, 8.224999997268824359, 7.608796670333726198 ) ) ;
#29008=CARTESIAN_POINT ( 'NONE',  ( 6.277390505771533514E-15, 67.00000000546236834, 34.17252228774368916 ) ) ;
#29012=ORIENTED_EDGE ( 'NONE', *, *, #23142, .F. ) ;
#29016=CARTESIAN_POINT ( 'NONE',  ( 32.50000000000000000, 75.00000000000001421, -3.980102097228898626E-15 ) ) ;
#29017=CARTESIAN_POINT ( 'NONE',  ( 33.58253175000000113, 52.37500000273121259, -4.112674001490185761E-15 ) ) ;
#29018=CARTESIAN_POINT ( 'NONE',  ( -32.50000000000000000, 54.60000000546237686, 10.55989012756946366 ) ) ;
#29020=CARTESIAN_POINT ( 'NONE',  ( 33.58253175000000113, 44.22500000273117138, -10.91162601494193751 ) ) ;
#29022=CARTESIAN_POINT ( 'NONE',  ( -20.75514604977248112, 67.67500000273116711, 28.56700777964554661 ) ) ;
#29025=CARTESIAN_POINT ( 'NONE',  ( -20.08610463437156923, 38.29999999999997584, 27.64615127144130113 ) ) ;
#29027=CARTESIAN_POINT ( 'NONE',  ( 20.75514604977249178, 12.07500000273120655, 28.56700777964553950 ) ) ;
#29028=CARTESIAN_POINT ( 'NONE',  ( -1.778240108872766143E-15, 36.00000000546238255, -32.49999999999999289 ) ) ;
#29030=CARTESIAN_POINT ( 'NONE',  ( 13.91746824999999887, 72.37500000273119838, -1.704398294459741270E-15 ) ) ;
#29031=CARTESIAN_POINT ( 'NONE',  ( -27.16883889988624290, 73.17500000273119554, -19.73931689729374028 ) ) ;
#29032=CYLINDRICAL_SURFACE ( 'NONE', #8356, 24.50000000000000000 ) ;
#29044=CARTESIAN_POINT ( 'NONE',  ( -26.29305231718578995, 56.70000000546237828, 19.10302069950538595 ) ) ;
#29045=CARTESIAN_POINT ( 'NONE',  ( -20.75514604977248823, 40.82500000273119412, -28.56700777964554305 ) ) ;
#29048=CYLINDRICAL_SURFACE ( 'NONE', #7890, 32.50000000000000000 ) ;
#29049=ORIENTED_EDGE ( 'NONE', *, *, #30013, .F. ) ;
#29051=CARTESIAN_POINT ( 'NONE',  ( 26.29305231718579350, 50.80000000000001137, 19.10302069950537529 ) ) ;
#29053=CARTESIAN_POINT ( 'NONE',  ( -33.58253175000000113, 69.27500000273116143, -10.91162601494193218 ) ) ;
#29054=ORIENTED_EDGE ( 'NONE', *, *, #11771, .F. ) ;
#29057=ORIENTED_EDGE ( 'NONE', *, *, #24810, .T. ) ;
#29059=CARTESIAN_POINT ( 'NONE',  ( 27.16883889988623935, 64.32500000273120122, -19.73931689729374384 ) ) ;
#29061=CARTESIAN_POINT ( 'NONE',  ( -32.50000000000000000, 66.60000000546237686, 10.55989012756946366 ) ) ;
#29062=CARTESIAN_POINT ( 'NONE',  ( -23.41746825000000243, 10.22499999726881725, 7.608796670333725309 ) ) ;
#29063=CARTESIAN_POINT ( 'NONE',  ( 20.75514604977249178, 5.825000002731198556, 28.56700777964553950 ) ) ;
#29064=CARTESIAN_POINT ( 'NONE',  ( -27.16883889988624290, 33.17500000273118843, -19.73931689729374028 ) ) ;
#29065=CARTESIAN_POINT ( 'NONE',  ( -4.635254915624211769, 77.85000000546237686, -14.26584774442730286 ) ) ;
#29069=CARTESIAN_POINT ( 'NONE',  ( 10.04305231718578817, 9.399999999999991473, -30.90933677959249337 ) ) ;
#29074=CARTESIAN_POINT ( 'NONE',  ( -4.300734207923755825, 77.27500000273118985, 13.23629886949340673 ) ) ;
#29076=CARTESIAN_POINT ( 'NONE',  ( -20.75514604977248112, 23.42500000273119909, 28.56700777964554661 ) ) ;
#29079=CARTESIAN_POINT ( 'NONE',  ( -20.75514604977248112, 15.67500000273117777, 28.56700777964554661 ) ) ;
#29081=EDGE_CURVE ( 'NONE', #21432, #1133, #5404, .T. ) ;
#29082=CARTESIAN_POINT ( 'NONE',  ( 20.75514604977248467, 70.42500000273119554, -28.56700777964554305 ) ) ;
#29086=CARTESIAN_POINT ( 'NONE',  ( -33.58253175000000113, 57.02500000273118275, -10.91162601494193041 ) ) ;
#29090=CARTESIAN_POINT ( 'NONE',  ( -20.08610463437156923, 16.29999999999997939, 27.64615127144130113 ) ) ;
#29091=CARTESIAN_POINT ( 'NONE',  ( -23.41746825000000243, 18.02499999726880731, -7.608796670333730638 ) ) ;
#29095=CARTESIAN_POINT ( 'NONE',  ( -32.50000000000000000, 68.50000000546238255, 0.000000000000000000 ) ) ;
#29096=VERTEX_POINT ( 'NONE', #21368 ) ;
#29100=CARTESIAN_POINT ( 'NONE',  ( 33.58253175000000113, 78.22500000273119269, -10.91162601494193751 ) ) ;
#29102=CARTESIAN_POINT ( 'NONE',  ( -15.14183272437241889, 2.700000000000001954, -20.84094480462497856 ) ) ;
#29103=CARTESIAN_POINT ( 'NONE',  ( 33.58253175000000823, 8.275000002731179194, 10.91162601494192863 ) ) ;
#29104=CARTESIAN_POINT ( 'NONE',  ( -32.50000000000000000, 58.10000000000000142, 10.55989012756946366 ) ) ;
#29105=CARTESIAN_POINT ( 'NONE',  ( -8.601468415847518756, 78.57500000273120122, -11.83890561707634603 ) ) ;
#29106=DIRECTION ( 'NONE',  ( 0.000000000000000000, 0.000000000000000000, -1.000000000000000000 ) ) ;
#29109=CARTESIAN_POINT ( 'NONE',  ( 8.601468415847516980, 76.67500000273116711, -11.83890561707634781 ) ) ;
#29113=CARTESIAN_POINT ( 'NONE',  ( -24.50000000000000000, 1.000000000000000888, -3.000384657911015469E-15 ) ) ;
#29114=CARTESIAN_POINT ( 'NONE',  ( 6.277390505771533514E-15, 2.500000000000008882, 34.17252228774368916 ) ) ;
#29118=CARTESIAN_POINT ( 'NONE',  ( -20.75514604977248112, 41.42500000273118133, 28.56700777964554661 ) ) ;
#29121=CARTESIAN_POINT ( 'NONE',  ( -20.75514604977248112, 35.67500000273118843, 28.56700777964554661 ) ) ;
#29122=CARTESIAN_POINT ( 'NONE',  ( 32.50000000000000711, 23.40000000546237402, 10.55989012756945122 ) ) ;
#29125=CARTESIAN_POINT ( 'NONE',  ( -1.778240108872766143E-15, 49.50000000000000000, -32.49999999999999289 ) ) ;
#29128=CARTESIAN_POINT ( 'NONE',  ( 18.94512977948576093, 6.824999997268821339, -13.76444248337722875 ) ) ;
#29129=DIRECTION ( 'NONE',  ( -0.000000000000000000, -1.000000000000000000, -0.000000000000000000 ) ) ;
#29131=EDGE_CURVE ( 'NONE', #684, #7428, #28618, .T. ) ;
#29132=CARTESIAN_POINT ( 'NONE',  ( -1.778240108872766143E-15, 11.49999999999999112, -32.49999999999999289 ) ) ;
#29133=CARTESIAN_POINT ( 'NONE',  ( 33.58253175000000823, 22.02500000273118275, 10.91162601494192685 ) ) ;
#29135=ORIENTED_EDGE ( 'NONE', *, *, #15884, .F. ) ;
#29137=EDGE_LOOP ( 'NONE', ( #32633, #4741 ) ) ;
#29141=ORIENTED_EDGE ( 'NONE', *, *, #3192, .F. ) ;
#29142=CARTESIAN_POINT ( 'NONE',  ( -14.47279130897151589, 1.324999997268808238, -19.92008829642072598 ) ) ;
#29143=CARTESIAN_POINT ( 'NONE',  ( -10.37757302488624411, 26.97500000273117493, -31.93888565452638417 ) ) ;
#29144=CARTESIAN_POINT ( 'NONE',  ( 26.29305231718578995, 37.70000000546236407, -19.10302069950538240 ) ) ;
#29145=CARTESIAN_POINT ( 'NONE',  ( -32.50000000000000000, 79.90000000000001990, -10.55989012756945478 ) ) ;
#29147=CARTESIAN_POINT ( 'NONE',  ( 20.75514604977249178, 46.07500000273117280, 28.56700777964553950 ) ) ;
#29149=CARTESIAN_POINT ( 'NONE',  ( -20.08610463437157989, 23.70000000000000639, -27.64615127144129758 ) ) ;
#29151=CARTESIAN_POINT ( 'NONE',  ( 20.75514604977249178, 65.82500000273115859, 28.56700777964553950 ) ) ;
#29153=CARTESIAN_POINT ( 'NONE',  ( -26.29305231718579350, 76.30000000546239391, -19.10302069950537884 ) ) ;
#29154=CARTESIAN_POINT ( 'NONE',  ( -10.37757302488623701, 53.77500000273119696, 31.93888565452638417 ) ) ;
#29157=CARTESIAN_POINT ( 'NONE',  ( -27.16883889988624290, 14.92500000273117067, -19.73931689729374028 ) ) ;
#29164=DIRECTION ( 'NONE',  ( 0.000000000000000000, 0.000000000000000000, -1.000000000000000000 ) ) ;
#29168=ADVANCED_FACE ( 'NONE', ( #13966 ), #29505, .F. ) ;
#29171=CIRCLE ( 'NONE', #23155, 15.00000000000000000 ) ;
#29175=CARTESIAN_POINT ( 'NONE',  ( 20.08610463437157279, 71.80000000546236549, -27.64615127144129758 ) ) ;
#29183=CARTESIAN_POINT ( 'NONE',  ( -26.29305231718579350, 35.79999999999999716, -19.10302069950537884 ) ) ;
#29184=CARTESIAN_POINT ( 'NONE',  ( 20.75514604977249178, 48.07500000273120122, 28.56700777964553950 ) ) ;
#29185=CARTESIAN_POINT ( 'NONE',  ( 10.04305231718578817, 55.90000000546238823, -30.90933677959249337 ) ) ;
#29187=CARTESIAN_POINT ( 'NONE',  ( -33.58253175000000113, 37.12500000273119838, 0.000000000000000000 ) ) ;
#29189=CARTESIAN_POINT ( 'NONE',  ( -20.75514604977248823, 59.07500000273119412, -28.56700777964554305 ) ) ;
#29193=CARTESIAN_POINT ( 'NONE',  ( -20.08610463437156923, 40.30000000000001137, 27.64615127144130113 ) ) ;
#29195=CARTESIAN_POINT ( 'NONE',  ( 6.486482029760649416E-15, 7.875000002731193049, 35.31076352940723240 ) ) ;
#29198=CARTESIAN_POINT ( 'NONE',  ( 11.25946833292375793, 74.17500000273119554, 8.180482586598731842 ) ) ;
#29199=CARTESIAN_POINT ( 'NONE',  ( -20.75514604977248823, 75.07500000273118701, -28.56700777964554305 ) ) ;
#29200=DIRECTION ( 'NONE',  ( -0.000000000000000000, -1.000000000000000000, -0.000000000000000000 ) ) ;
#29201=AXIS2_PLACEMENT_3D ( 'NONE', #4898, #4554, #17438 ) ;
#29203=EDGE_LOOP ( 'NONE', ( #11092, #14034, #888, #19290 ) ) ;
#29204=DIRECTION ( 'NONE',  ( 0.000000000000000000, 0.000000000000000000, -1.000000000000000000 ) ) ;
#29213=CARTESIAN_POINT ( 'NONE',  ( -32.50000000000000000, 56.40000000546237402, -10.55989012756945300 ) ) ;
#29214=CARTESIAN_POINT ( 'NONE',  ( 33.58253175000000823, 36.02500000273117564, 10.91162601494192685 ) ) ;
#29217=CARTESIAN_POINT ( 'NONE',  ( 7.890940483122900408E-14, 10.49999999999999112, -24.50000000000000000 ) ) ;
#29218=ORIENTED_EDGE ( 'NONE', *, *, #10945, .F. ) ;
#29222=CARTESIAN_POINT ( 'NONE',  ( 10.37757302488624056, 70.77500000273117564, -31.93888565452638417 ) ) ;
#29227=ORIENTED_EDGE ( 'NONE', *, *, #8182, .F. ) ;
#29228=CARTESIAN_POINT ( 'NONE',  ( -26.29305231718578995, 48.70000000546237118, 19.10302069950538595 ) ) ;
#29229=CARTESIAN_POINT ( 'NONE',  ( -33.58253175000000113, 57.22500000273117848, 10.91162601494193929 ) ) ;
#29231=CARTESIAN_POINT ( 'NONE',  ( 20.08610463437157279, 19.80000000546237260, -27.64615127144129758 ) ) ;
#29233=CARTESIAN_POINT ( 'NONE',  ( -23.41746824999999887, 10.02499999726882507, -7.608796670333730638 ) ) ;
#29235=CARTESIAN_POINT ( 'NONE',  ( 6.486482029760649416E-15, 27.87500000273120193, 35.31076352940723240 ) ) ;
#29238=CARTESIAN_POINT ( 'NONE',  ( -5.147494310547430452, 31.55125428154683576, -32.49999999999999289 ) ) ;
#29243=CARTESIAN_POINT ( 'NONE',  ( -4.300734207923759378, 72.47500000273119269, -13.23629886949340495 ) ) ;
#29245=CARTESIAN_POINT ( 'NONE',  ( -33.58253175000000113, 27.22500000273119269, 10.91162601494193929 ) ) ;
#29248=CARTESIAN_POINT ( 'NONE',  ( 6.486482029760648627E-15, 13.87500000273117706, 35.31076352940722529 ) ) ;
#29251=CARTESIAN_POINT ( 'NONE',  ( 27.16883889988623935, 68.32500000273117280, -19.73931689729374384 ) ) ;
#29252=CARTESIAN_POINT ( 'NONE',  ( 32.50000000000000000, 59.50000000546237544, -3.980102097228898626E-15 ) ) ;
#29254=CARTESIAN_POINT ( 'NONE',  ( 4.635254915624212657, 78.85000000546239107, 14.26584774442730286 ) ) ;
#29255=CARTESIAN_POINT ( 'NONE',  ( -10.37757302488624411, 56.72500000273117138, -31.93888565452638417 ) ) ;
#29259=CARTESIAN_POINT ( 'NONE',  ( -27.16883889988624290, 2.925000002731187543, -19.73931689729374028 ) ) ;
#29260=CARTESIAN_POINT ( 'NONE',  ( -7.236395654485757944, 5.224999997268803043, -22.27133577429736988 ) ) ;
#29262=ADVANCED_FACE ( 'NONE', ( #18422 ), #10855, .F. ) ;
#29263=ORIENTED_EDGE ( 'NONE', *, *, #7038, .F. ) ;
#29265=CARTESIAN_POINT ( 'NONE',  ( -5.147494310547430452, 42.05125428700921475, -32.49999999999999289 ) ) ;
#29269=CARTESIAN_POINT ( 'NONE',  ( -24.50000000000000000, 2.899999999999995470, -7.960532557706207157 ) ) ;
#29270=CARTESIAN_POINT ( 'NONE',  ( 5.147494310547434893, 27.05125428700921475, 32.49999999999999289 ) ) ;
#29274=CARTESIAN_POINT ( 'NONE',  ( 7.236395654485755280, 18.22499999726881370, 22.27133577429736988 ) ) ;
#29275=CARTESIAN_POINT ( 'NONE',  ( -27.16883889988624290, 9.175000002731191984, -19.73931689729374028 ) ) ;
#29276=CARTESIAN_POINT ( 'NONE',  ( 10.04305231718579705, 58.59999999999998721, 30.90933677959248982 ) ) ;
#29277=CARTESIAN_POINT ( 'NONE',  ( 13.91746824999999532, 77.97500000273119269, -4.522059556121118540 ) ) ;
#29280=CARTESIAN_POINT ( 'NONE',  ( 11.25946833292375793, 74.57500000273120122, -8.180482586598735395 ) ) ;
#29282=EDGE_CURVE ( 'NONE', #23148, #14306, #534, .T. ) ;
#29284=CARTESIAN_POINT ( 'NONE',  ( 20.08610463437158344, 70.70000000000000284, 27.64615127144129403 ) ) ;
#29286=CARTESIAN_POINT ( 'NONE',  ( -20.75514604977248823, 40.82500000273120122, -28.56700777964554305 ) ) ;
#29289=CARTESIAN_POINT ( 'NONE',  ( 20.75514604977249178, 34.07500000273117990, 28.56700777964553950 ) ) ;
#29290=ADVANCED_FACE ( 'NONE', ( #31938 ), #21824, .F. ) ;
#29291=DIRECTION ( 'NONE',  ( 1.000000000000000000, 0.000000000000000000, -0.000000000000000000 ) ) ;
#29293=LINE ( 'NONE', #8695, #15240 ) ;
#29295=CARTESIAN_POINT ( 'NONE',  ( -12.13525491562420910, 76.19999999999998863, 8.816778784387098611 ) ) ;
#29298=CARTESIAN_POINT ( 'NONE',  ( -14.47279130897152299, 1.924999997268818541, 19.92008829642072243 ) ) ;
#29301=CARTESIAN_POINT ( 'NONE',  ( -1.778240108872766143E-15, 54.00000000546237544, -32.49999999999999289 ) ) ;
#29302=CARTESIAN_POINT ( 'NONE',  ( 6.486482029760648627E-15, 21.62500000273119127, 35.31076352940722529 ) ) ;
#29304=ORIENTED_EDGE ( 'NONE', *, *, #21531, .F. ) ;
#29306=ORIENTED_EDGE ( 'NONE', *, *, #6700, .F. ) ;
#29310=ORIENTED_EDGE ( 'NONE', *, *, #29672, .T. ) ;
#29312=CARTESIAN_POINT ( 'NONE',  ( 33.58253175000000113, 28.47500000273118204, -10.91162601494193751 ) ) ;
#29313=CARTESIAN_POINT ( 'NONE',  ( 32.50000000000000711, 33.40000000546238113, 10.55989012756945122 ) ) ;
#29315=CARTESIAN_POINT ( 'NONE',  ( 26.29305231718579350, 78.79999999999998295, 19.10302069950537529 ) ) ;
#29316=CARTESIAN_POINT ( 'NONE',  ( -10.04305231718578462, 54.90000000546238823, 30.90933677959249337 ) ) ;
#29317=CARTESIAN_POINT ( 'NONE',  ( 2.375766604868043252, 73.44874571845316780, -14.99999999999999822 ) ) ;
#29318=CARTESIAN_POINT ( 'NONE',  ( 27.16883889988624290, 44.17500000273119554, 19.73931689729373673 ) ) ;
#29321=CARTESIAN_POINT ( 'NONE',  ( 10.04305231718578817, 19.40000000000000213, -30.90933677959249337 ) ) ;
#29323=CARTESIAN_POINT ( 'NONE',  ( -2.162160676586881955E-15, 64.62500000273121259, -35.31076352940723240 ) ) ;
#29326=CARTESIAN_POINT ( 'NONE',  ( -33.58253175000000113, 55.47500000273120691, 10.91162601494193929 ) ) ;
#29329=CARTESIAN_POINT ( 'NONE',  ( -33.58253175000000113, 3.125000002731193049, 0.000000000000000000 ) ) ;
#29331=CARTESIAN_POINT ( 'NONE',  ( 10.04305231718579705, 25.10000000546236265, 30.90933677959248982 ) ) ;
#29335=CARTESIAN_POINT ( 'NONE',  ( -1.778240108872766143E-15, 18.00000000546237544, -32.49999999999999289 ) ) ;
#29336=CYLINDRICAL_SURFACE ( 'NONE', #15558, 32.50000000000000000 ) ;
#29341=CARTESIAN_POINT ( 'NONE',  ( 20.08610463437157279, 49.29999999999998295, -27.64615127144129758 ) ) ;
#29344=CARTESIAN_POINT ( 'NONE',  ( -26.29305231718578995, 70.70000000546239960, 19.10302069950538595 ) ) ;
#29349=VECTOR ( 'NONE', #3512, 1000.000000000000000 ) ;
#29353=CARTESIAN_POINT ( 'NONE',  ( -33.58253175000000113, 49.37500000273120548, 0.000000000000000000 ) ) ;
#29354=CARTESIAN_POINT ( 'NONE',  ( 20.08610463437158344, 47.20000000546238539, 27.64615127144129403 ) ) ;
#29356=CARTESIAN_POINT ( 'NONE',  ( -10.37757302488623701, 35.52500000273117564, 31.93888565452638417 ) ) ;
#29357=DIRECTION ( 'NONE',  ( -0.000000000000000000, -1.000000000000000000, -0.000000000000000000 ) ) ;
#29358=CARTESIAN_POINT ( 'NONE',  ( -10.37757302488624411, 58.97500000273120691, -31.93888565452638417 ) ) ;
#29359=CARTESIAN_POINT ( 'NONE',  ( -32.50000000000000000, 0.5000000054623809920, 0.000000000000000000 ) ) ;
#29361=CARTESIAN_POINT ( 'NONE',  ( 32.50000000000000000, 39.10000000000002274, -10.55989012756945833 ) ) ;
#29364=CARTESIAN_POINT ( 'NONE',  ( -27.16883889988623935, 5.575000002731201221, 19.73931689729374739 ) ) ;
#29366=CARTESIAN_POINT ( 'NONE',  ( 13.91746825000000065, 74.27500000273117564, 4.522059556121114987 ) ) ;
#29367=CARTESIAN_POINT ( 'NONE',  ( 20.75514604977248467, 74.67500000273118133, -28.56700777964554305 ) ) ;
#29368=CARTESIAN_POINT ( 'NONE',  ( -24.50000000000000000, 4.899999999999990585, -7.960532557706207157 ) ) ;
#29374=CARTESIAN_POINT ( 'NONE',  ( 2.445080149700053643E-15, 76.50000000000000000, 15.00000000000000000 ) ) ;
#29383=DIRECTION ( 'NONE',  ( 0.000000000000000000, -0.000000000000000000, 1.000000000000000000 ) ) ;
#29384=CARTESIAN_POINT ( 'NONE',  ( 33.58253175000000113, 40.22500000273118559, -10.91162601494193574 ) ) ;
#29388=ORIENTED_EDGE ( 'NONE', *, *, #2231, .T. ) ;
#29390=DIRECTION ( 'NONE',  ( -0.000000000000000000, -1.000000000000000000, -0.000000000000000000 ) ) ;
#29392=CARTESIAN_POINT ( 'NONE',  ( 10.37757302488624767, 67.97500000273117848, 31.93888565452638417 ) ) ;
#29393=ORIENTED_EDGE ( 'NONE', *, *, #26431, .F. ) ;
#29396=ORIENTED_EDGE ( 'NONE', *, *, #24524, .T. ) ;
#29397=CARTESIAN_POINT ( 'NONE',  ( -10.04305231718578462, 48.90000000546238113, 30.90933677959249337 ) ) ;
#29398=CARTESIAN_POINT ( 'NONE',  ( -33.58253175000000113, 57.02500000273118275, -10.91162601494193218 ) ) ;
#29400=CARTESIAN_POINT ( 'NONE',  ( -32.50000000000000000, 18.60000000546238041, 10.55989012756946366 ) ) ;
#29402=CARTESIAN_POINT ( 'NONE',  ( -18.94512977948575738, 9.924999997268812990, -13.76444248337723231 ) ) ;
#29403=CARTESIAN_POINT ( 'NONE',  ( 20.75514604977248467, 26.67500000273118133, -28.56700777964554305 ) ) ;
#29406=CARTESIAN_POINT ( 'NONE',  ( -13.91746824999999532, 78.77500000273116143, -4.522059556121115875 ) ) ;
#29407=CARTESIAN_POINT ( 'NONE',  ( -10.04305231718579172, 28.10000000546236620, -30.90933677959248982 ) ) ;
#29411=CARTESIAN_POINT ( 'NONE',  ( 4.300734207923761154, 73.47500000273119269, 13.23629886949340495 ) ) ;
#29413=( BOUNDED_CURVE ( )  B_SPLINE_CURVE ( 2, ( #16927, #6282, #11272, #19005, #19171, #3379, #32357, #32193, #26883, #29284, #21906, #16265, #26721 ),
 .UNSPECIFIED., .F., .F. ) 
 B_SPLINE_CURVE_WITH_KNOTS ( ( 3, 2, 2, 2, 2, 2, 3 ),
 ( 0.1089743589743589758, 0.1102564102564102533, 0.1128205128205128221, 0.1153846153846153910, 0.1179487179487179460, 0.1205128205128205149, 0.1217948717948718063 ),
 .UNSPECIFIED. ) 
 CURVE ( )  GEOMETRIC_REPRESENTATION_ITEM ( )  RATIONAL_B_SPLINE_CURVE ( ( 0.9755282581475768211, 0.9755282581475768211, 1.000000000000000000, 0.9510565162951535312, 1.000000000000000000, 0.9510565162951535312, 1.000000000000000000, 0.9510565162951535312, 1.000000000000000000, 0.9510565162951535312, 1.000000000000000000, 0.9755282581475765991, 0.9755282581475767101 ) ) 
 REPRESENTATION_ITEM ( '' )  );
#29414=CARTESIAN_POINT ( 'NONE',  ( 27.16883889988623935, 24.32500000273119056, -19.73931689729374384 ) ) ;
#29417=CARTESIAN_POINT ( 'NONE',  ( -10.37757302488624411, 14.97500000273119269, -31.93888565452638417 ) ) ;
#29419=CARTESIAN_POINT ( 'NONE',  ( 33.58253175000000113, 70.22500000273120691, -10.91162601494193574 ) ) ;
#29420=LINE ( 'NONE', #16562, #29349 ) ;
#29421=CARTESIAN_POINT ( 'NONE',  ( 2.688165632520823219E-15, 75.87500000273119838, 14.63369212191046209 ) ) ;
#29424=CARTESIAN_POINT ( 'NONE',  ( -33.58253175000000113, 55.02500000273118985, -10.91162601494193041 ) ) ;
#29429=CARTESIAN_POINT ( 'NONE',  ( 18.94512977948575738, 6.424999997268809437, 13.76444248337723408 ) ) ;
#29431=ORIENTED_EDGE ( 'NONE', *, *, #16975, .T. ) ;
#29433=DIRECTION ( 'NONE',  ( -0.000000000000000000, -1.000000000000000000, -0.000000000000000000 ) ) ;
#29434=ORIENTED_EDGE ( 'NONE', *, *, #8408, .F. ) ;
#29436=CARTESIAN_POINT ( 'NONE',  ( 32.50000000000000000, 11.50000000546236301, -3.980102097228898626E-15 ) ) ;
#29438=CARTESIAN_POINT ( 'NONE',  ( 33.58253175000000113, 76.22500000273119269, -10.91162601494193751 ) ) ;
#29440=CARTESIAN_POINT ( 'NONE',  ( 24.50000000000000000, 6.000000000000005329, 0.000000000000000000 ) ) ;
#29441=CARTESIAN_POINT ( 'NONE',  ( -10.37757302488623701, 9.775000002731182747, 31.93888565452638417 ) ) ;
#29442=CARTESIAN_POINT ( 'NONE',  ( -20.75514604977248823, 14.82500000273117635, -28.56700777964554305 ) ) ;
#29443=CARTESIAN_POINT ( 'NONE',  ( 26.29305231718579350, 57.30000000546237260, 19.10302069950537529 ) ) ;
#29444=LINE ( 'NONE', #3536, #9350 ) ;
#29446=CARTESIAN_POINT ( 'NONE',  ( 4.300734207923757602, 76.77500000273118985, -13.23629886949340673 ) ) ;
#29448=FACE_OUTER_BOUND ( 'NONE', #1913, .T. ) ;
#29449=CARTESIAN_POINT ( 'NONE',  ( -10.04305231718578462, 38.90000000546237402, 30.90933677959249337 ) ) ;
#29451=CARTESIAN_POINT ( 'NONE',  ( -20.75514604977248112, 45.42500000273119554, 28.56700777964554661 ) ) ;
#29454=CARTESIAN_POINT ( 'NONE',  ( -10.37757302488624411, 32.97500000273117848, -31.93888565452638417 ) ) ;
#29455=CARTESIAN_POINT ( 'NONE',  ( 5.779280353836490358E-15, 66.50000000000000000, 32.49999999999999289 ) ) ;
#29458=CARTESIAN_POINT ( 'NONE',  ( 10.04305231718579705, 30.60000000000001563, 30.90933677959248982 ) ) ;
#29461=CARTESIAN_POINT ( 'NONE',  ( -14.47279130897151767, 3.324999997268803131, -19.92008829642072598 ) ) ;
#29462=CARTESIAN_POINT ( 'NONE',  ( 5.779280353836490358E-15, 53.00000000546238255, 32.49999999999999289 ) ) ;
#29465=CARTESIAN_POINT ( 'NONE',  ( 10.37757302488624767, 19.72500000273119625, 31.93888565452638417 ) ) ;
#29467=VERTEX_POINT ( 'NONE', #1883 ) ;
#29469=ORIENTED_EDGE ( 'NONE', *, *, #13656, .T. ) ;
#29472=CARTESIAN_POINT ( 'NONE',  ( -10.04305231718579172, 9.599999999999997868, -30.90933677959248982 ) ) ;
#29473=CARTESIAN_POINT ( 'NONE',  ( -7.236395654485757944, 7.224999997268804819, -22.27133577429736988 ) ) ;
#29474=CARTESIAN_POINT ( 'NONE',  ( -2.162160676586881955E-15, 30.87500000273119483, -35.31076352940723240 ) ) ;
#29476=CARTESIAN_POINT ( 'NONE',  ( 20.08610463437157279, 33.80000000546235839, -27.64615127144129758 ) ) ;
#29477=CARTESIAN_POINT ( 'NONE',  ( 20.08610463437158344, 78.70000000000000284, 27.64615127144129403 ) ) ;
#29478=CARTESIAN_POINT ( 'NONE',  ( 5.147494310547426899, 53.44874571845315359, -32.50000000000000000 ) ) ;
#29479=LINE ( 'NONE', #3247, #6151 ) ;
#29480=CARTESIAN_POINT ( 'NONE',  ( 33.58253175000000113, 42.47500000273119980, -10.91162601494193751 ) ) ;
#29482=CARTESIAN_POINT ( 'NONE',  ( 32.50000000000000000, 19.10000000000000497, -10.55989012756945833 ) ) ;
#29484=EDGE_CURVE ( 'NONE', #30610, #11703, #9985, .T. ) ;
#29485=CARTESIAN_POINT ( 'NONE',  ( -33.58253175000000113, 65.02500000273118985, -10.91162601494193218 ) ) ;
#29486=CARTESIAN_POINT ( 'NONE',  ( 33.58253175000000823, 52.27500000273118275, 10.91162601494192685 ) ) ;
#29489=CARTESIAN_POINT ( 'NONE',  ( 20.75514604977248467, 2.425000002731189763, -28.56700777964554305 ) ) ;
#29496=CARTESIAN_POINT ( 'NONE',  ( 24.50000000000000000, 14.09999999999999076, -7.960532557706203605 ) ) ;
#29497=EDGE_CURVE ( 'NONE', #11025, #29752, #24023, .T. ) ;
#29500=CARTESIAN_POINT ( 'NONE',  ( 5.779280353836490358E-15, 48.50000000000000000, 32.49999999999999289 ) ) ;
#29502=VERTEX_POINT ( 'NONE', #30886 ) ;
#29505=( BOUNDED_SURFACE ( )  B_SPLINE_SURFACE ( 1, 2, ( 
 ( #29562, #18632, #5573, #13642, #24430, #24272, #24106, #5742, #21530, #3002, #5908, #11387, #31978, #8475, #21864, #18962, #11225, #13475, #13804, #2828, #23940, #29406, #26999, #16385, #26339, #21701, #28904, #15882, #409, #10895, #574, #12054, #11547, #1411, #12227, #27507, #22524, #29729, #24594, #17219, #27342, #6234, #30233, #22029, #16715, #3996, #14137, #6737, #14810, #1236, #14469, #1067, #4336, #30066, #19961, #14302, #16879, #32975, #17046, #27169, #22197, #33152, #19286, #24926, #24758, #19620, #32473, #3662, #6908, #8974, #4168, #9479, #19456, #9300, #6572, #19784, #27853, #27678, #17388, #3828, #11714, #29903, #11888, #6405, #9139, #14640, #32644, #22360, #25274, #32807, #1747, #25100, #1577, #30409, #22700, #7765, #15503, #1926, #5020, #23222, #28363 ),
 ( #7245, #20827, #10008, #4506, #18251, #7598, #14980, #20480, #25786, #33681, #17910, #28698, #2275, #18076, #12575, #23562, #15679, #15331, #12749, #5195, #30931, #10180, #12917, #20662, #12403, #26128, #23046, #2625, #9828, #23393, #28525, #25450, #13088, #17561, #31102, #33504, #20304, #25957, #9656, #4850, #7424, #2451, #33855, #10349, #22873, #31271, #25622, #20136, #33331, #30755, #30581, #17733, #2102, #7077, #28018, #28190, #4678, #15157, #21657, #11187, #32102, #3294, #8431, #8600, #195, #13760, #24230, #5363, #19083, #26636, #13430, #29366, #29198, #8263, #10682, #18920, #701, #5866, #23898, #29523, #16344, #31442, #6026, #20993, #369, #21163, #16504, #5533, #15843, #26300, #29030, #13255, #3130, #13603, #26957, #3457, #23729, #26800, #16014, #8103, #13928 ) ),
 .UNSPECIFIED., .F., .F., .T. ) 
 B_SPLINE_SURFACE_WITH_KNOTS ( ( 2, 2 ),
 ( 3, 2, 2, 2, 2, 2, 2, 2, 2, 2, 2, 2, 2, 2, 2, 2, 2, 2, 2, 2, 2, 2, 2, 2, 2, 2, 2, 2, 2, 2, 2, 2, 2, 2, 2, 2, 2, 2, 2, 2, 2, 2, 2, 2, 2, 2, 2, 2, 2, 2, 3 ),
 ( 0.000000000000000000, 1.000000000000000000 ),
 ( 0.000000000000000000, 0.02000000000000000042, 0.04000000000000000083, 0.05999999999999999778, 0.08000000000000000167, 0.1000000000000000056, 0.1199999999999999956, 0.1400000000000000133, 0.1600000000000000033, 0.1799999999999999933, 0.2000000000000000111, 0.2200000000000000011, 0.2399999999999999911, 0.2600000000000000089, 0.2800000000000000266, 0.2999999999999999889, 0.3200000000000000067, 0.3400000000000000244, 0.3599999999999999867, 0.3800000000000000044, 0.4000000000000000222, 0.4199999999999999845, 0.4400000000000000022, 0.4600000000000000200, 0.4799999999999999822, 0.5000000000000000000, 0.5200000000000000178, 0.5400000000000000355, 0.5600000000000000533, 0.5799999999999999600, 0.5999999999999999778, 0.6199999999999999956, 0.6400000000000000133, 0.6600000000000000311, 0.6800000000000000488, 0.6999999999999999556, 0.7199999999999999734, 0.7399999999999999911, 0.7600000000000000089, 0.7800000000000000266, 0.8000000000000000444, 0.8199999999999999512, 0.8399999999999999689, 0.8599999999999999867, 0.8800000000000000044, 0.9000000000000000222, 0.9200000000000000400, 0.9399999999999999467, 0.9599999999999999645, 0.9799999999999999822, 1.000000000000000000 ),
 .UNSPECIFIED. ) 
 GEOMETRIC_REPRESENTATION_ITEM ( )  RATIONAL_B_SPLINE_SURFACE ( (
 ( 1.000000000000000000, 0.9510565162951535312, 1.000000000000000000, 0.9510565162951535312, 1.000000000000000000, 0.9510565162951535312, 1.000000000000000000, 0.9510565162951535312, 1.000000000000000000, 0.9510565162951535312, 1.000000000000000000, 0.9510565162951535312, 1.000000000000000000, 0.9510565162951535312, 1.000000000000000000, 0.9510565162951535312, 1.000000000000000000, 0.9510565162951535312, 1.000000000000000000, 0.9510565162951535312, 1.000000000000000000, 0.9510565162951535312, 1.000000000000000000, 0.9510565162951535312, 1.000000000000000000, 0.9510565162951535312, 1.000000000000000000, 0.9510565162951535312, 1.000000000000000000, 0.9510565162951535312, 1.000000000000000000, 0.9510565162951535312, 1.000000000000000000, 0.9510565162951535312, 1.000000000000000000, 0.9510565162951535312, 1.000000000000000000, 0.9510565162951535312, 1.000000000000000000, 0.9510565162951535312, 1.000000000000000000, 0.9510565162951535312, 1.000000000000000000, 0.9510565162951535312, 1.000000000000000000, 0.9510565162951535312, 1.000000000000000000, 0.9510565162951535312, 1.000000000000000000, 0.9510565162951535312, 1.000000000000000000, 0.9510565162951535312, 1.000000000000000000, 0.9510565162951535312, 1.000000000000000000, 0.9510565162951535312, 1.000000000000000000, 0.9510565162951535312, 1.000000000000000000, 0.9510565162951535312, 1.000000000000000000, 0.9510565162951535312, 1.000000000000000000, 0.9510565162951535312, 1.000000000000000000, 0.9510565162951535312, 1.000000000000000000, 0.9510565162951535312, 1.000000000000000000, 0.9510565162951535312, 1.000000000000000000, 0.9510565162951535312, 1.000000000000000000, 0.9510565162951535312, 1.000000000000000000, 0.9510565162951535312, 1.000000000000000000, 0.9510565162951535312, 1.000000000000000000, 0.9510565162951535312, 1.000000000000000000, 0.9510565162951535312, 1.000000000000000000, 0.9510565162951535312, 1.000000000000000000, 0.9510565162951535312, 1.000000000000000000, 0.9510565162951535312, 1.000000000000000000, 0.9510565162951535312, 1.000000000000000000, 0.9510565162951535312, 1.000000000000000000, 0.9510565162951535312, 1.000000000000000000, 0.9510565162951535312, 1.000000000000000000, 0.9510565162951535312, 1.000000000000000000, 0.9510565162951535312, 1.000000000000000000),
 ( 1.000000000000000000, 0.9510565162951535312, 1.000000000000000000, 0.9510565162951535312, 1.000000000000000000, 0.9510565162951535312, 1.000000000000000000, 0.9510565162951535312, 1.000000000000000000, 0.9510565162951535312, 1.000000000000000000, 0.9510565162951535312, 1.000000000000000000, 0.9510565162951535312, 1.000000000000000000, 0.9510565162951535312, 1.000000000000000000, 0.9510565162951535312, 1.000000000000000000, 0.9510565162951535312, 1.000000000000000000, 0.9510565162951535312, 1.000000000000000000, 0.9510565162951535312, 1.000000000000000000, 0.9510565162951535312, 1.000000000000000000, 0.9510565162951535312, 1.000000000000000000, 0.9510565162951535312, 1.000000000000000000, 0.9510565162951535312, 1.000000000000000000, 0.9510565162951535312, 1.000000000000000000, 0.9510565162951535312, 1.000000000000000000, 0.9510565162951535312, 1.000000000000000000, 0.9510565162951535312, 1.000000000000000000, 0.9510565162951535312, 1.000000000000000000, 0.9510565162951535312, 1.000000000000000000, 0.9510565162951535312, 1.000000000000000000, 0.9510565162951535312, 1.000000000000000000, 0.9510565162951535312, 1.000000000000000000, 0.9510565162951535312, 1.000000000000000000, 0.9510565162951535312, 1.000000000000000000, 0.9510565162951535312, 1.000000000000000000, 0.9510565162951535312, 1.000000000000000000, 0.9510565162951535312, 1.000000000000000000, 0.9510565162951535312, 1.000000000000000000, 0.9510565162951535312, 1.000000000000000000, 0.9510565162951535312, 1.000000000000000000, 0.9510565162951535312, 1.000000000000000000, 0.9510565162951535312, 1.000000000000000000, 0.9510565162951535312, 1.000000000000000000, 0.9510565162951535312, 1.000000000000000000, 0.9510565162951535312, 1.000000000000000000, 0.9510565162951535312, 1.000000000000000000, 0.9510565162951535312, 1.000000000000000000, 0.9510565162951535312, 1.000000000000000000, 0.9510565162951535312, 1.000000000000000000, 0.9510565162951535312, 1.000000000000000000, 0.9510565162951535312, 1.000000000000000000, 0.9510565162951535312, 1.000000000000000000, 0.9510565162951535312, 1.000000000000000000, 0.9510565162951535312, 1.000000000000000000, 0.9510565162951535312, 1.000000000000000000, 0.9510565162951535312, 1.000000000000000000, 0.9510565162951535312, 1.000000000000000000) ) ) 
 REPRESENTATION_ITEM ( '' )  SURFACE ( )  );
#29512=CARTESIAN_POINT ( 'NONE',  ( -27.16883889988624290, 49.17500000273117422, -19.73931689729374028 ) ) ;
#29513=CARTESIAN_POINT ( 'NONE',  ( 20.08610463437158344, 49.20000000546237828, 27.64615127144129403 ) ) ;
#29515=CARTESIAN_POINT ( 'NONE',  ( 33.58253175000000113, 34.12500000273119127, -4.112674001490185761E-15 ) ) ;
#29516=CARTESIAN_POINT ( 'NONE',  ( -8.446640517145639571E-15, 77.00000000546236834, 32.49999999999999289 ) ) ;
#29517=CARTESIAN_POINT ( 'NONE',  ( -33.58253175000000113, 61.27500000273118985, -10.91162601494193218 ) ) ;
#29519=CARTESIAN_POINT ( 'NONE',  ( 10.04305231718579705, 42.60000000000000142, 30.90933677959248982 ) ) ;
#29521=CARTESIAN_POINT ( 'NONE',  ( -27.16883889988623935, 3.575000002731199000, 19.73931689729374739 ) ) ;
#29523=CARTESIAN_POINT ( 'NONE',  ( -13.91746824999999532, 73.47500000273117848, 4.522059556121122093 ) ) ;
#29524=CARTESIAN_POINT ( 'NONE',  ( 27.16883889988624290, 72.17500000273119554, 19.73931689729373673 ) ) ;
#29525=CARTESIAN_POINT ( 'NONE',  ( -24.50000000000000000, 5.000000000000004441, -3.000384657911015469E-15 ) ) ;
#29528=CARTESIAN_POINT ( 'NONE',  ( -24.50000000000000000, 6.749999994537625447, -3.000384657911015469E-15 ) ) ;
#29541=CARTESIAN_POINT ( 'NONE',  ( 5.147494310547434893, 13.05125428700922718, 32.49999999999999289 ) ) ;
#29542=VERTEX_POINT ( 'NONE', #7555 ) ;
#29543=EDGE_CURVE ( 'NONE', #29467, #726, #2572, .T. ) ;
#29545=CARTESIAN_POINT ( 'NONE',  ( 32.50000000000000000, 50.99999999999999289, -3.980102097228898626E-15 ) ) ;
#29547=CARTESIAN_POINT ( 'NONE',  ( -2.162160676586881955E-15, 66.87500000273119838, -35.31076352940723240 ) ) ;
#29548=EDGE_CURVE ( 'NONE', #32174, #13932, #6059, .T. ) ;
#29552=VERTEX_POINT ( 'NONE', #31400 ) ;
#29553=CARTESIAN_POINT ( 'NONE',  ( -1.778240108872766143E-15, 48.00000000546238255, -32.49999999999999289 ) ) ;
#29554=CARTESIAN_POINT ( 'NONE',  ( 10.37757302488624056, 54.52500000273119696, -31.93888565452638417 ) ) ;
#29556=CARTESIAN_POINT ( 'NONE',  ( 26.29305231718579350, 19.30000000546239391, 19.10302069950537529 ) ) ;
#29558=CARTESIAN_POINT ( 'NONE',  ( 1.507698388325705758E-15, 11.62499999726880340, -24.62258325217400312 ) ) ;
#29559=CARTESIAN_POINT ( 'NONE',  ( 10.37757302488624056, 20.77500000273119340, -31.93888565452638417 ) ) ;
#29562=CARTESIAN_POINT ( 'NONE',  ( -13.91746824999999887, 80.87500000273118417, 0.000000000000000000 ) ) ;
#29563=CARTESIAN_POINT ( 'NONE',  ( -5.147494310547423346, 28.94874572391553258, 32.50000000000000000 ) ) ;
#29567=CARTESIAN_POINT ( 'NONE',  ( 13.91746824999999887, 73.87500000273116996, -1.704398294459741270E-15 ) ) ;
#29569=CARTESIAN_POINT ( 'NONE',  ( 10.37757302488624056, 22.52500000273119340, -31.93888565452638417 ) ) ;
#29573=CARTESIAN_POINT ( 'NONE',  ( -33.58253175000000113, 9.475000002731199800, 10.91162601494193929 ) ) ;
#29575=CARTESIAN_POINT ( 'NONE',  ( 6.486482029760648627E-15, 71.62500000273118417, 35.31076352940722529 ) ) ;
#29577=DIRECTION ( 'NONE',  ( 0.000000000000000000, 0.000000000000000000, 1.000000000000000000 ) ) ;
#29578=CARTESIAN_POINT ( 'NONE',  ( -13.91746824999999887, 79.37500000273118417, 0.000000000000000000 ) ) ;
#29580=CARTESIAN_POINT ( 'NONE',  ( 2.375766604868044141, 79.69874572391552192, -14.99999999999999822 ) ) ;
#29581=CARTESIAN_POINT ( 'NONE',  ( -27.16883889988624290, 58.92500000273118133, -19.73931689729374028 ) ) ;
#29586=CARTESIAN_POINT ( 'NONE',  ( -33.58253175000000113, 3.125000002731193049, 0.000000000000000000 ) ) ;
#29587=CARTESIAN_POINT ( 'NONE',  ( -14.47279130897151589, 3.324999997268803131, -19.92008829642072598 ) ) ;
#29589=EDGE_CURVE ( 'NONE', #33710, #19766, #1637, .T. ) ;
#29590=VERTEX_POINT ( 'NONE', #28428 ) ;
#29592=CARTESIAN_POINT ( 'NONE',  ( -10.04305231718579172, 68.10000000546237686, -30.90933677959248982 ) ) ;
#29596=CARTESIAN_POINT ( 'NONE',  ( 2.067204126564591252E-14, 2.500000000000004885, -24.50000000000000000 ) ) ;
#29597=CARTESIAN_POINT ( 'NONE',  ( -20.75514604977248823, 72.82500000273118701, -28.56700777964554305 ) ) ;
#29599=CARTESIAN_POINT ( 'NONE',  ( 7.570916362186207671, 7.599999999999996092, 23.30088464923126779 ) ) ;
#29600=CARTESIAN_POINT ( 'NONE',  ( 20.75514604977248467, 6.675000002731201754, -28.56700777964554305 ) ) ;
#29601=CARTESIAN_POINT ( 'NONE',  ( 20.75514604977249178, 17.82500000273120122, 28.56700777964553950 ) ) ;
#29602=( BOUNDED_CURVE ( )  B_SPLINE_CURVE ( 2, ( #24368, #30003, #32247, #21796, #6001, #32576, #14404, #26931, #11160, #9075, #16475, #3429, #3765 ),
 .UNSPECIFIED., .F., .T. ) 
 B_SPLINE_CURVE_WITH_KNOTS ( ( 3, 2, 2, 2, 2, 2, 3 ),
 ( 0.6089743589743590313, 0.6102564102564103088, 0.6128205128205128638, 0.6153846153846154188, 0.6179487179487179738, 0.6205128205128205288, 0.6217948717948718063 ),
 .UNSPECIFIED. ) 
 CURVE ( )  GEOMETRIC_REPRESENTATION_ITEM ( )  RATIONAL_B_SPLINE_CURVE ( ( 0.9755282581475768211, 0.9755282581475778203, 1.000000000000000000, 0.9510565162951535312, 1.000000000000000000, 0.9510565162951535312, 1.000000000000000000, 0.9510565162951535312, 1.000000000000000000, 0.9510565162951535312, 1.000000000000000000, 0.9755282581475768211, 0.9755282581475768211 ) ) 
 REPRESENTATION_ITEM ( '' )  );
#29603=CARTESIAN_POINT ( 'NONE',  ( 11.25946833292375793, 75.67500000273119554, 8.180482586598731842 ) ) ;
#29606=CARTESIAN_POINT ( 'NONE',  ( -9.270509831248421762, 80.29999999999999716, 12.75976212528060039 ) ) ;
#29610=CARTESIAN_POINT ( 'NONE',  ( -33.58253175000000113, 45.22500000273117848, 10.91162601494193929 ) ) ;
#29613=CARTESIAN_POINT ( 'NONE',  ( -27.16883889988623935, 29.57500000273119412, 19.73931689729374739 ) ) ;
#29614=CARTESIAN_POINT ( 'NONE',  ( 24.50000000000000000, 18.00000000000001421, 0.000000000000000000 ) ) ;
#29617=CARTESIAN_POINT ( 'NONE',  ( 2.445080149700053643E-15, 76.49999999999998579, 15.00000000000000000 ) ) ;
#29620=CARTESIAN_POINT ( 'NONE',  ( -23.41746825000000243, 5.724999997268815477, 7.608796670333725309 ) ) ;
#29623=CARTESIAN_POINT ( 'NONE',  ( -32.50000000000000000, 60.09999999999999432, 10.55989012756946366 ) ) ;
#29624=CARTESIAN_POINT ( 'NONE',  ( -2.162160676586882350E-15, 20.62500000273119483, -35.31076352940722529 ) ) ;
#29625=CARTESIAN_POINT ( 'NONE',  ( -7.236395654485757944, 7.724999997268805707, -22.27133577429736988 ) ) ;
#29629=ORIENTED_EDGE ( 'NONE', *, *, #13776, .F. ) ;
#29632=VECTOR ( 'NONE', #32555, 1000.000000000000000 ) ;
#29634=CARTESIAN_POINT ( 'NONE',  ( 23.41746825000000243, 4.524999997268823293, 7.608796670333735079 ) ) ;
#29635=CARTESIAN_POINT ( 'NONE',  ( 6.486482029760649416E-15, 25.87500000273117351, 35.31076352940723240 ) ) ;
#29636=CARTESIAN_POINT ( 'NONE',  ( -32.50000000000000000, 30.60000000546238041, 10.55989012756946366 ) ) ;
#29637=CARTESIAN_POINT ( 'NONE',  ( 32.50000000000000000, 71.10000000000000853, -10.55989012756945833 ) ) ;
#29638=CARTESIAN_POINT ( 'NONE',  ( 3.980102097228898626E-15, 0.000000000000000000, 32.50000000000000000 ) ) ;
#29639=FACE_OUTER_BOUND ( 'NONE', #32748, .T. ) ;
#29641=CARTESIAN_POINT ( 'NONE',  ( -27.16883889988624290, 41.17500000273119554, -19.73931689729374028 ) ) ;
#29642=CARTESIAN_POINT ( 'NONE',  ( 1.507698388325705758E-15, 7.624999997268814056, -24.62258325217400312 ) ) ;
#29643=CARTESIAN_POINT ( 'NONE',  ( -10.04305231718578462, 22.40000000000000213, 30.90933677959249337 ) ) ;
#29644=AXIS2_PLACEMENT_3D ( 'NONE', #16860, #11693, #33126 ) ;
#29647=CARTESIAN_POINT ( 'NONE',  ( 27.16883889988624290, 61.92500000273118133, 19.73931689729373673 ) ) ;
#29648=CARTESIAN_POINT ( 'NONE',  ( 33.58253175000000113, 52.37500000273121259, -4.112674001490185761E-15 ) ) ;
#29651=CARTESIAN_POINT ( 'NONE',  ( 33.58253175000000113, 8.225000002731182036, -10.91162601494193751 ) ) ;
#29657=DIRECTION ( 'NONE',  ( -0.000000000000000000, 1.000000000000000000, -0.000000000000000000 ) ) ;
#29660=CARTESIAN_POINT ( 'NONE',  ( 10.04305231718578817, 1.900000005462365582, -30.90933677959249337 ) ) ;
#29668=CARTESIAN_POINT ( 'NONE',  ( 1.093617666956751375E-13, 60.00000000546237544, -32.50000000000000711 ) ) ;
#29672=EDGE_CURVE ( 'NONE', #32174, #8211, #28260, .T. ) ;
#29674=CARTESIAN_POINT ( 'NONE',  ( -5.147494310547423346, 46.94874572391552903, 32.50000000000000000 ) ) ;
#29675=CARTESIAN_POINT ( 'NONE',  ( -33.58253175000000113, 47.27500000273116143, -10.91162601494193218 ) ) ;
#29676=CARTESIAN_POINT ( 'NONE',  ( -2.092463501923844636E-15, 48.00000000546238255, -34.17252228774368916 ) ) ;
#29678=CARTESIAN_POINT ( 'NONE',  ( -10.37757302488623701, 33.52500000273117564, 31.93888565452638417 ) ) ;
#29679=CARTESIAN_POINT ( 'NONE',  ( 26.29305231718579350, 77.30000000546239391, 19.10302069950537529 ) ) ;
#29680=CARTESIAN_POINT ( 'NONE',  ( 10.37757302488624056, 62.77500000273117564, -31.93888565452638417 ) ) ;
#29682=CARTESIAN_POINT ( 'NONE',  ( -10.04305231718578462, 38.39999999999999147, 30.90933677959249337 ) ) ;
#29684=CARTESIAN_POINT ( 'NONE',  ( 6.486482029760649416E-15, 3.875000002731201931, 35.31076352940723240 ) ) ;
#29685=CARTESIAN_POINT ( 'NONE',  ( -20.08610463437156923, 70.80000000546235128, 27.64615127144130113 ) ) ;
#29687=CARTESIAN_POINT ( 'NONE',  ( 27.16883889988623935, 74.57500000273120122, -19.73931689729374384 ) ) ;
#29688=CARTESIAN_POINT ( 'NONE',  ( -19.82091636218621034, 18.54999999453762882, -14.40073868116559552 ) ) ;
#29691=VERTEX_POINT ( 'NONE', #2344 ) ;
#29692=CARTESIAN_POINT ( 'NONE',  ( -24.50000000000001066, 2.849999994537639303, 7.960532557706201828 ) ) ;
#29705=( BOUNDED_CURVE ( )  B_SPLINE_CURVE ( 2, ( #16224, #26678, #11065, #18633, #13476, #23941, #5234, #5061, #7804, #28738, #21034, #15883, #26340 ),
 .UNSPECIFIED., .F., .T. ) 
 B_SPLINE_CURVE_WITH_KNOTS ( ( 3, 2, 2, 2, 2, 2, 3 ),
 ( 0.03205128205128205537, 0.03333333333333333287, 0.03589743589743589480, 0.03846153846153846367, 0.04102564102564102561, 0.04358974358974358754, 0.04487179487179487197 ),
 .UNSPECIFIED. ) 
 CURVE ( )  GEOMETRIC_REPRESENTATION_ITEM ( )  RATIONAL_B_SPLINE_CURVE ( ( 0.9755282581475768211, 0.9755282581475768211, 1.000000000000000000, 0.9510565162951535312, 1.000000000000000000, 0.9510565162951535312, 1.000000000000000000, 0.9510565162951535312, 1.000000000000000000, 0.9510565162951535312, 1.000000000000000000, 0.9755282581475768211, 0.9755282581475768211 ) ) 
 REPRESENTATION_ITEM ( '' )  );
#29708=CARTESIAN_POINT ( 'NONE',  ( -15.14183272437242067, 16.69999999999999574, -20.84094480462497856 ) ) ;
#29709=ORIENTED_EDGE ( 'NONE', *, *, #5171, .F. ) ;
#29711=CARTESIAN_POINT ( 'NONE',  ( -20.08610463437157989, 75.69999999999998863, -27.64615127144129758 ) ) ;
#29713=CARTESIAN_POINT ( 'NONE',  ( 20.75514604977249178, 72.07500000273120122, 28.56700777964553950 ) ) ;
#29717=ORIENTED_EDGE ( 'NONE', *, *, #24050, .F. ) ;
#29718=AXIS2_PLACEMENT_3D ( 'NONE', #23047, #17911, #31443 ) ;
#29719=CARTESIAN_POINT ( 'NONE',  ( 5.779280353836490358E-15, 65.00000000546236834, 32.49999999999999289 ) ) ;
#29720=CARTESIAN_POINT ( 'NONE',  ( 20.75514604977249178, 57.82500000273118701, 28.56700777964553950 ) ) ;
#29722=CARTESIAN_POINT ( 'NONE',  ( 32.50000000000000711, 9.400000005462381125, 10.55989012756945122 ) ) ;
#29725=CARTESIAN_POINT ( 'NONE',  ( 7.236395654485760609, 17.52499999726880731, -22.27133577429736633 ) ) ;
#29726=CARTESIAN_POINT ( 'NONE',  ( -20.75514604977248823, 23.07500000273117635, -28.56700777964554305 ) ) ;
#29729=CARTESIAN_POINT ( 'NONE',  ( -8.601468415847515203, 77.17500000273120975, 11.83890561707634959 ) ) ;
#29730=DIRECTION ( 'NONE',  ( -0.000000000000000000, -1.000000000000000000, -0.000000000000000000 ) ) ;
#29731=CARTESIAN_POINT ( 'NONE',  ( 5.147494310547643614, 15.44874571845315181, -32.49999999999992895 ) ) ;
#29733=VERTEX_POINT ( 'NONE', #4744 ) ;
#29735=CARTESIAN_POINT ( 'NONE',  ( 11.25946833292375793, 78.07500000273121543, -8.180482586598735395 ) ) ;
#29738=CARTESIAN_POINT ( 'NONE',  ( 33.58253175000000823, 16.02500000273119340, 10.91162601494192863 ) ) ;
#29742=CARTESIAN_POINT ( 'NONE',  ( 33.58253175000000113, 6.475000002731177595, -10.91162601494193574 ) ) ;
#29745=CARTESIAN_POINT ( 'NONE',  ( 10.04305231718579705, 59.10000000546239107, 30.90933677959248982 ) ) ;
#29746=CARTESIAN_POINT ( 'NONE',  ( -4.300734207923755825, 75.77500000273118985, 13.23629886949340673 ) ) ;
#29749=CARTESIAN_POINT ( 'NONE',  ( -2.162160676586882350E-15, 54.62500000273116996, -35.31076352940722529 ) ) ;
#29752=VERTEX_POINT ( 'NONE', #17627 ) ;
#29755=CARTESIAN_POINT ( 'NONE',  ( 7.236395654485760609, 5.024999997268825069, -22.27133577429736633 ) ) ;
#29759=CARTESIAN_POINT ( 'NONE',  ( -32.50000000000000000, 68.40000000546240244, -10.55989012756945300 ) ) ;
#29762=CARTESIAN_POINT ( 'NONE',  ( -20.75514604977248112, 59.67500000273118133, 28.56700777964554661 ) ) ;
#29763=CARTESIAN_POINT ( 'NONE',  ( 3.445340210940985210E-14, 7.249999994537622783, 24.50000000000000000 ) ) ;
#29764=CARTESIAN_POINT ( 'NONE',  ( 20.75514604977248467, 72.42500000273119554, -28.56700777964554305 ) ) ;
#29766=CARTESIAN_POINT ( 'NONE',  ( -24.50000000000000355, 4.899999999999989697, -7.960532557706207157 ) ) ;
#29768=CARTESIAN_POINT ( 'NONE',  ( 20.75514604977248467, 16.42500000273118133, -28.56700777964554305 ) ) ;
#29769=CARTESIAN_POINT ( 'NONE',  ( -32.50000000000000000, 0.6000000054623972900, 10.55989012756946366 ) ) ;
#29771=CARTESIAN_POINT ( 'NONE',  ( 9.270509831248423538, 81.29999999999999716, -12.75976212528059861 ) ) ;
#29775=CARTESIAN_POINT ( 'NONE',  ( 1.555960095263670572E-15, 8.249999994537619230, -24.50000000000000000 ) ) ;
#29779=CARTESIAN_POINT ( 'NONE',  ( -20.75514604977248823, 42.82500000273119412, -28.56700777964554305 ) ) ;
#29782=CARTESIAN_POINT ( 'NONE',  ( 20.75514604977248467, 30.67500000273119909, -28.56700777964554305 ) ) ;
#29784=EDGE_CURVE ( 'NONE', #27962, #29096, #10249, .T. ) ;
#29790=CARTESIAN_POINT ( 'NONE',  ( 18.94512977948575738, 6.424999997268809437, 13.76444248337723408 ) ) ;
#29792=DIRECTION ( 'NONE',  ( -0.000000000000000000, 1.000000000000000000, -0.000000000000000000 ) ) ;
#29794=CARTESIAN_POINT ( 'NONE',  ( -15.00000000000000000, 76.15000000546235981, -4.873795443493594171 ) ) ;
#29795=CARTESIAN_POINT ( 'NONE',  ( -27.16883889988624290, 18.92500000273117422, -19.73931689729374028 ) ) ;
#29796=CARTESIAN_POINT ( 'NONE',  ( -7.236395654485763274, 6.524999997268826846, 22.27133577429736633 ) ) ;
#29797=VECTOR ( 'NONE', #22794, 1000.000000000000000 ) ;
#29800=ORIENTED_EDGE ( 'NONE', *, *, #4749, .F. ) ;
#29804=ORIENTED_EDGE ( 'NONE', *, *, #18195, .F. ) ;
#29807=CARTESIAN_POINT ( 'NONE',  ( -1.778240108872766143E-15, 39.50000000000000000, -32.49999999999999289 ) ) ;
#29808=CARTESIAN_POINT ( 'NONE',  ( -7.570916362186210335, 18.34999999453762598, -23.30088464923126779 ) ) ;
#29809=CARTESIAN_POINT ( 'NONE',  ( 23.41746825000000243, 2.724999997268822138, -7.608796670333727974 ) ) ;
#29810=CARTESIAN_POINT ( 'NONE',  ( 20.75514604977248467, 28.67500000273117777, -28.56700777964554305 ) ) ;
#29811=CARTESIAN_POINT ( 'NONE',  ( -2.092463501923844636E-15, 34.00000000546236123, -34.17252228774368916 ) ) ;
#29812=CARTESIAN_POINT ( 'NONE',  ( 26.29305231718579350, 74.80000000000001137, 19.10302069950537529 ) ) ;
#29813=CARTESIAN_POINT ( 'NONE',  ( -26.29305231718578995, 6.700000005462392494, 19.10302069950538595 ) ) ;
#29814=CARTESIAN_POINT ( 'NONE',  ( -24.50000000000000000, 10.90000000000000568, -7.960532557706207157 ) ) ;
#29816=CARTESIAN_POINT ( 'NONE',  ( -20.75514604977248823, 39.07500000273119412, -28.56700777964554305 ) ) ;
#29818=CARTESIAN_POINT ( 'NONE',  ( -23.41746825000000598, 10.22499999726881903, 7.608796670333726198 ) ) ;
#29819=CARTESIAN_POINT ( 'NONE',  ( 6.277390505771533514E-15, 16.50000000000000000, 34.17252228774368916 ) ) ;
#29823=CARTESIAN_POINT ( 'NONE',  ( 27.16883889988624290, 65.92500000273118133, 19.73931689729373673 ) ) ;
#29824=CARTESIAN_POINT ( 'NONE',  ( -10.37757302488624411, 46.97500000273119269, -31.93888565452638417 ) ) ;
#29827=CARTESIAN_POINT ( 'NONE',  ( 20.75514604977249178, 5.825000002731198556, 28.56700777964553950 ) ) ;
#29832=CARTESIAN_POINT ( 'NONE',  ( 0.000000000000000000, 80.00000000000001421, 0.000000000000000000 ) ) ;
#29839=CARTESIAN_POINT ( 'NONE',  ( 26.29305231718579350, 48.80000000000001137, 19.10302069950537529 ) ) ;
#29842=ORIENTED_EDGE ( 'NONE', *, *, #4845, .F. ) ;
#29847=FACE_OUTER_BOUND ( 'NONE', #27791, .T. ) ;
#29848=EDGE_LOOP ( 'NONE', ( #31045, #33352, #16677, #4193, #24930, #1305, #15782, #6894 ) ) ;
#29852=CARTESIAN_POINT ( 'NONE',  ( -27.16883889988624290, 47.17500000273119554, -19.73931689729374028 ) ) ;
#29853=CARTESIAN_POINT ( 'NONE',  ( 20.08610463437158344, 51.20000000546237828, 27.64615127144129403 ) ) ;
#29855=CARTESIAN_POINT ( 'NONE',  ( 33.58253175000000113, 36.12500000273119127, -4.112674001490185761E-15 ) ) ;
#29857=CARTESIAN_POINT ( 'NONE',  ( 33.58253175000000823, 64.27500000273118985, 10.91162601494192863 ) ) ;
#29858=( NAMED_UNIT ( * ) SI_UNIT ( $, .STERADIAN. ) SOLID_ANGLE_UNIT ( ) );
#29860=CARTESIAN_POINT ( 'NONE',  ( 26.29305231718579350, 30.79999999999999361, 19.10302069950537529 ) ) ;
#29862=CARTESIAN_POINT ( 'NONE',  ( -20.75514604977248823, 5.075000002731193227, -28.56700777964554305 ) ) ;
#29865=CARTESIAN_POINT ( 'NONE',  ( -33.58253175000000113, 69.37500000273119838, 0.000000000000000000 ) ) ;
#29866=CARTESIAN_POINT ( 'NONE',  ( -7.570916362186210335, 18.34999999453762598, -23.30088464923126779 ) ) ;
#29869=CARTESIAN_POINT ( 'NONE',  ( 7.570916362186207671, 3.349999994537639303, 23.30088464923126779 ) ) ;
#29870=STYLED_ITEM ( 'NONE', ( #11342 ), #11923 ) ;
#29882=CARTESIAN_POINT ( 'NONE',  ( -10.04305231718578462, 58.40000000000000568, 30.90933677959249337 ) ) ;
#29883=CARTESIAN_POINT ( 'NONE',  ( 5.779280353836490358E-15, 13.00000000546238077, 32.49999999999999289 ) ) ;
#29888=VERTEX_POINT ( 'NONE', #1821 ) ;
#29891=VERTEX_POINT ( 'NONE', #5263 ) ;
#29892=CARTESIAN_POINT ( 'NONE',  ( -32.50000000000000000, 55.99999999999999289, 0.000000000000000000 ) ) ;
#29893=CARTESIAN_POINT ( 'NONE',  ( 10.37757302488624056, 52.52500000273118985, -31.93888565452638417 ) ) ;
#29895=CARTESIAN_POINT ( 'NONE',  ( -26.29305231718578995, 10.70000000546239605, 19.10302069950538595 ) ) ;
#29897=CARTESIAN_POINT ( 'NONE',  ( 7.236395654485755280, 12.72499999726881015, 22.27133577429736988 ) ) ;
#29898=CARTESIAN_POINT ( 'NONE',  ( 26.29305231718579350, 58.80000000000001847, 19.10302069950537529 ) ) ;
#29899=CARTESIAN_POINT ( 'NONE',  ( -27.16883889988624290, 21.17500000273120264, -19.73931689729374028 ) ) ;
#29901=CARTESIAN_POINT ( 'NONE',  ( -32.50000000000000000, 24.40000000546237047, -10.55989012756945300 ) ) ;
#29903=CARTESIAN_POINT ( 'NONE',  ( -13.91746824999999532, 72.77500000273117564, -4.522059556121115875 ) ) ;
#29904=CARTESIAN_POINT ( 'NONE',  ( 7.890940483122900408E-14, 16.49999999999999645, -24.50000000000000000 ) ) ;
#29906=( BOUNDED_CURVE ( )  B_SPLINE_CURVE ( 2, ( #25272, #30929, #7422, #28188, #4676, #1745, #15155 ),
 .UNSPECIFIED., .F., .T. ) 
 B_SPLINE_CURVE_WITH_KNOTS ( ( 3, 2, 2, 3 ),
 ( 0.000000000000000000, 0.01111111111111111154, 0.02222222222222222307, 0.02777777777777777624 ),
 .UNSPECIFIED. ) 
 CURVE ( )  GEOMETRIC_REPRESENTATION_ITEM ( )  RATIONAL_B_SPLINE_CURVE ( ( 1.000000000000000000, 0.9510565162951535312, 1.000000000000000000, 0.9510565162951535312, 1.000000000000000000, 0.9755282581475768211, 0.9755282581475768211 ) ) 
 REPRESENTATION_ITEM ( '' )  );
#29908=EDGE_LOOP ( 'NONE', ( #932, #6676, #29717, #11512 ) ) ;
#29913=CARTESIAN_POINT ( 'NONE',  ( -27.16883889988623935, 17.32500000273118346, 19.73931689729374739 ) ) ;
#29917=CARTESIAN_POINT ( 'NONE',  ( 27.16883889988624290, 12.17500000273119554, 19.73931689729373673 ) ) ;
#29920=CARTESIAN_POINT ( 'NONE',  ( 20.08610463437158344, 3.200000005462373398, 27.64615127144129403 ) ) ;
#29921=CARTESIAN_POINT ( 'NONE',  ( 8.601468415847516980, 78.67500000273119554, -11.83890561707634603 ) ) ;
#29923=DIRECTION ( 'NONE',  ( 0.000000000000000000, 0.000000000000000000, 1.000000000000000000 ) ) ;
#29924=CARTESIAN_POINT ( 'NONE',  ( -27.16883889988623935, 49.32500000273118701, 19.73931689729374739 ) ) ;
#29928=CARTESIAN_POINT ( 'NONE',  ( 32.50000000000000000, 17.10000000000001208, -10.55989012756945833 ) ) ;
#29929=CARTESIAN_POINT ( 'NONE',  ( -4.523095164977116484E-15, 8.124999997268826490, 24.62258325217400312 ) ) ;
#29931=ORIENTED_EDGE ( 'NONE', *, *, #10511, .T. ) ;
#29934=ORIENTED_EDGE ( 'NONE', *, *, #2724, .T. ) ;
#29936=CARTESIAN_POINT ( 'NONE',  ( 20.75514604977249178, 58.07500000273117990, 28.56700777964553950 ) ) ;
#29938=CARTESIAN_POINT ( 'NONE',  ( -33.58253175000000113, 73.22500000273117848, 10.91162601494193929 ) ) ;
#29940=CARTESIAN_POINT ( 'NONE',  ( -15.14183272437242600, 3.300000000000012257, 20.84094480462497856 ) ) ;
#29941=CARTESIAN_POINT ( 'NONE',  ( -10.37757302488623701, 1.775000002731175197, 31.93888565452638417 ) ) ;
#29942=CARTESIAN_POINT ( 'NONE',  ( -27.16883889988623935, 17.32500000273118346, 19.73931689729374739 ) ) ;
#29943=CARTESIAN_POINT ( 'NONE',  ( -20.08610463437156923, 0.8000000054623617185, 27.64615127144130113 ) ) ;
#29945=CARTESIAN_POINT ( 'NONE',  ( -12.13525491562420910, 78.19999999999998863, 8.816778784387098611 ) ) ;
#29949=CARTESIAN_POINT ( 'NONE',  ( -5.147494310547430452, 38.05125428700922185, -32.49999999999999289 ) ) ;
#29951=CARTESIAN_POINT ( 'NONE',  ( 33.58253175000000113, 36.12500000273119127, -4.112674001490185761E-15 ) ) ;
#29954=CARTESIAN_POINT ( 'NONE',  ( -27.16883889988624290, 25.17500000273117777, -19.73931689729374028 ) ) ;
#29958=CARTESIAN_POINT ( 'NONE',  ( -8.891200544363830713E-16, 75.50000000000001421, -15.00000000000000000 ) ) ;
#29960=CARTESIAN_POINT ( 'NONE',  ( -23.41746825000000243, 13.72499999726882258, 7.608796670333725309 ) ) ;
#29962=CARTESIAN_POINT ( 'NONE',  ( 3.980102097228898626E-15, 80.00000000000001421, 32.50000000000000000 ) ) ;
#29965=CARTESIAN_POINT ( 'NONE',  ( -33.58253175000000113, 15.12500000273120371, 0.000000000000000000 ) ) ;
#29966=CARTESIAN_POINT ( 'NONE',  ( -23.41746824999999887, 4.124999997268813168, -2.867812753649727150E-15 ) ) ;
#29968=EDGE_LOOP ( 'NONE', ( #17073, #19814, #27707, #10113 ) ) ;
#29971=EDGE_CURVE ( 'NONE', #7495, #5936, #16604, .T. ) ;
#29972=EDGE_LOOP ( 'NONE', ( #13670, #31083, #6850, #12385 ) ) ;
#29975=CARTESIAN_POINT ( 'NONE',  ( -10.04305231718578462, 10.39999999999999325, 30.90933677959249337 ) ) ;
#29976=CARTESIAN_POINT ( 'NONE',  ( -4.732186688966233175E-15, 15.24999999453762811, 25.76082449383753925 ) ) ;
#29978=CARTESIAN_POINT ( 'NONE',  ( -7.236395654485763274, 4.024999997268824181, 22.27133577429736633 ) ) ;
#29979=CARTESIAN_POINT ( 'NONE',  ( -33.58253175000000113, 19.37500000273118062, 0.000000000000000000 ) ) ;
#29980=CARTESIAN_POINT ( 'NONE',  ( 6.277390505771533514E-15, 31.00000000546236834, 34.17252228774368916 ) ) ;
#29981=CARTESIAN_POINT ( 'NONE',  ( -10.04305231718579172, 69.59999999999999432, -30.90933677959248982 ) ) ;
#29984=CARTESIAN_POINT ( 'NONE',  ( 10.37757302488624056, 34.77500000273120406, -31.93888565452638417 ) ) ;
#29988=CARTESIAN_POINT ( 'NONE',  ( -14.47279130897152122, 8.424999997268816543, 19.92008829642072243 ) ) ;
#29989=CARTESIAN_POINT ( 'NONE',  ( -32.50000000000000000, 16.00000000000001421, 0.000000000000000000 ) ) ;
#29992=CARTESIAN_POINT ( 'NONE',  ( 27.16883889988624290, 53.92500000273120264, 19.73931689729373673 ) ) ;
#29993=CARTESIAN_POINT ( 'NONE',  ( 33.58253175000000823, 48.27500000273119696, 10.91162601494192685 ) ) ;
#29995=CARTESIAN_POINT ( 'NONE',  ( 10.04305231718579705, 67.10000000546237686, 30.90933677959248982 ) ) ;
#29996=CARTESIAN_POINT ( 'NONE',  ( -27.16883889988624290, 2.925000002731187543, -19.73931689729374028 ) ) ;
#30001=LINE ( 'NONE', #6506, #28635 ) ;
#30002=CARTESIAN_POINT ( 'NONE',  ( -32.50000000000000000, 58.50000000546237544, 0.000000000000000000 ) ) ;
#30003=CARTESIAN_POINT ( 'NONE',  ( -5.147494310547640062, 30.94874572391553258, 32.49999999999992895 ) ) ;
#30006=( BOUNDED_CURVE ( )  B_SPLINE_CURVE ( 2, ( #25026, #7004, #17486, #6831, #14906, #27948, #9398, #11644, #11982, #9231, #22451, #22623, #24688 ),
 .UNSPECIFIED., .F., .T. ) 
 B_SPLINE_CURVE_WITH_KNOTS ( ( 3, 2, 2, 2, 2, 2, 3 ),
 ( 0.1944444444444444475, 0.2000000000000000111, 0.2111111111111111105, 0.2222222222222222099, 0.2333333333333333370, 0.2444444444444444364, 0.2499999999999999722 ),
 .UNSPECIFIED. ) 
 CURVE ( )  GEOMETRIC_REPRESENTATION_ITEM ( )  RATIONAL_B_SPLINE_CURVE ( ( 0.9755282581475768211, 0.9755282581475768211, 1.000000000000000000, 0.9510565162951535312, 1.000000000000000000, 0.9510565162951535312, 1.000000000000000000, 0.9510565162951535312, 1.000000000000000000, 0.9510565162951535312, 1.000000000000000000, 0.9755282581475768211, 0.9755282581475768211 ) ) 
 REPRESENTATION_ITEM ( '' )  );
#30008=CARTESIAN_POINT ( 'NONE',  ( -10.37757302488623701, 31.52500000273117564, 31.93888565452638417 ) ) ;
#30013=EDGE_CURVE ( 'NONE', #18081, #16083, #20110, .T. ) ;
#30015=ORIENTED_EDGE ( 'NONE', *, *, #24524, .F. ) ;
#30019=CARTESIAN_POINT ( 'NONE',  ( 20.08610463437157279, 57.29999999999999005, -27.64615127144129758 ) ) ;
#30020=CARTESIAN_POINT ( 'NONE',  ( -20.75514604977248823, 41.07500000273119412, -28.56700777964554305 ) ) ;
#30021=CARTESIAN_POINT ( 'NONE',  ( -32.50000000000000000, 48.50000000546239676, 0.000000000000000000 ) ) ;
#30023=CARTESIAN_POINT ( 'NONE',  ( -10.37757302488623701, 29.52500000273117209, 31.93888565452638417 ) ) ;
#30025=CARTESIAN_POINT ( 'NONE',  ( -2.162160676586881955E-15, 56.87500000273117706, -35.31076352940723240 ) ) ;
#30027=CARTESIAN_POINT ( 'NONE',  ( -32.50000000000000000, 31.90000000000001279, -10.55989012756945478 ) ) ;
#30029=CARTESIAN_POINT ( 'NONE',  ( -33.58253175000000113, 1.475000002731190474, 10.91162601494193929 ) ) ;
#30030=DIRECTION ( 'NONE',  ( 0.000000000000000000, 0.000000000000000000, -1.000000000000000000 ) ) ;
#30032=CARTESIAN_POINT ( 'NONE',  ( 33.58253175000000823, 66.27500000273117564, 10.91162601494192685 ) ) ;
#30033=CARTESIAN_POINT ( 'NONE',  ( 3.880418787951150694, 4.198745712990782586, -24.49999999999999645 ) ) ;
#30035=CARTESIAN_POINT ( 'NONE',  ( 24.50000000000000355, 5.649999994537638237, 7.960532557706212486 ) ) ;
#30047=CARTESIAN_POINT ( 'NONE',  ( 5.779280353836490358E-15, 14.50000000000000178, 32.49999999999999289 ) ) ;
#30048=CARTESIAN_POINT ( 'NONE',  ( 20.08610463437158344, 58.70000000000000995, 27.64615127144129403 ) ) ;
#30049=ORIENTED_EDGE ( 'NONE', *, *, #11361, .T. ) ;
#30051=CARTESIAN_POINT ( 'NONE',  ( -15.00000000000000000, 81.12500000273121259, 0.000000000000000000 ) ) ;
#30056=CARTESIAN_POINT ( 'NONE',  ( -20.08610463437157989, 55.69999999999998863, -27.64615127144129758 ) ) ;
#30057=CARTESIAN_POINT ( 'NONE',  ( -20.75514604977248823, 50.82500000273116569, -28.56700777964554305 ) ) ;
#30059=CARTESIAN_POINT ( 'NONE',  ( 26.29305231718578995, 11.70000000546239605, -19.10302069950538240 ) ) ;
#30061=CARTESIAN_POINT ( 'NONE',  ( -23.41746824999999887, 12.12499999726882116, -2.867812753649727150E-15 ) ) ;
#30062=CARTESIAN_POINT ( 'NONE',  ( -32.50000000000000000, 55.90000000000000568, -10.55989012756945478 ) ) ;
#30063=CARTESIAN_POINT ( 'NONE',  ( 33.58253175000000113, 26.37500000273118417, -4.112674001490185761E-15 ) ) ;
#30066=CARTESIAN_POINT ( 'NONE',  ( 8.601468415847520532, 75.57500000273120122, 11.83890561707634781 ) ) ;
#30067=CARTESIAN_POINT ( 'NONE',  ( 4.635254915624209993, 75.65000000546237402, -14.26584774442730463 ) ) ;
#30068=CARTESIAN_POINT ( 'NONE',  ( -33.58253175000000113, 1.375000002731191495, 0.000000000000000000 ) ) ;
#30070=VERTEX_POINT ( 'NONE', #16251 ) ;
#30072=CARTESIAN_POINT ( 'NONE',  ( 20.08610463437158344, 71.20000000546237118, 27.64615127144129403 ) ) ;
#30077=CARTESIAN_POINT ( 'NONE',  ( 20.75514604977248467, 10.67500000273119021, -28.56700777964554305 ) ) ;
#30080=CARTESIAN_POINT ( 'NONE',  ( -13.91746824999999532, 77.47500000273120691, 4.522059556121122093 ) ) ;
#30083=CARTESIAN_POINT ( 'NONE',  ( -20.75514604977248112, 51.42500000273118133, 28.56700777964554661 ) ) ;
#30087=CARTESIAN_POINT ( 'NONE',  ( 0.000000000000000000, 80.00000000000001421, 0.000000000000000000 ) ) ;
#30088=CARTESIAN_POINT ( 'NONE',  ( -23.41746825000000243, 11.52499999726880553, -7.608796670333730638 ) ) ;
#30090=ORIENTED_EDGE ( 'NONE', *, *, #22577, .T. ) ;
#30092=DIRECTION ( 'NONE',  ( 0.000000000000000000, 0.000000000000000000, -1.000000000000000000 ) ) ;
#30095=CARTESIAN_POINT ( 'NONE',  ( -20.75514604977248112, 57.67500000273118133, 28.56700777964554661 ) ) ;
#30096=CARTESIAN_POINT ( 'NONE',  ( -32.50000000000000000, 36.50000000546238255, 0.000000000000000000 ) ) ;
#30097=CARTESIAN_POINT ( 'NONE',  ( -33.58253175000000113, 65.02500000273118985, -10.91162601494193218 ) ) ;
#30100=CARTESIAN_POINT ( 'NONE',  ( 24.50000000000000000, 8.000000000000007105, 0.000000000000000000 ) ) ;
#30101=DIRECTION ( 'NONE',  ( 0.000000000000000000, 0.000000000000000000, -1.000000000000000000 ) ) ;
#30102=CARTESIAN_POINT ( 'NONE',  ( 27.16883889988623935, 16.32500000273118346, -19.73931689729374384 ) ) ;
#30103=CARTESIAN_POINT ( 'NONE',  ( 8.601468415847520532, 73.57500000273117280, 11.83890561707634603 ) ) ;
#30105=CARTESIAN_POINT ( 'NONE',  ( -13.91746824999999887, 71.37500000273119838, 0.000000000000000000 ) ) ;
#30111=CARTESIAN_POINT ( 'NONE',  ( 4.635254915624209993, 79.65000000546237402, -14.26584774442730463 ) ) ;
#30113=CARTESIAN_POINT ( 'NONE',  ( -10.37757302488623701, 39.52500000273118275, 31.93888565452638417 ) ) ;
#30116=CARTESIAN_POINT ( 'NONE',  ( -33.58253175000000113, 27.37500000273118772, 0.000000000000000000 ) ) ;
#30117=CARTESIAN_POINT ( 'NONE',  ( -32.50000000000000000, 68.00000000000000000, 0.000000000000000000 ) ) ;
#30120=CARTESIAN_POINT ( 'NONE',  ( -20.08610463437156923, 18.30000000000000426, 27.64615127144130113 ) ) ;
#30123=CARTESIAN_POINT ( 'NONE',  ( -14.47279130897152299, 13.92499999726881654, 19.92008829642072243 ) ) ;
#30128=CARTESIAN_POINT ( 'NONE',  ( 33.58253175000000823, 16.02500000273119340, 10.91162601494192685 ) ) ;
#30129=CARTESIAN_POINT ( 'NONE',  ( 18.94512977948575738, 2.924999997268806773, 13.76444248337723408 ) ) ;
#30131=VERTEX_POINT ( 'NONE', #13056 ) ;
#30137=CARTESIAN_POINT ( 'NONE',  ( 5.779280353836490358E-15, 38.50000000000000000, 32.49999999999999289 ) ) ;
#30138=CARTESIAN_POINT ( 'NONE',  ( 15.14183272437241889, 17.44999999453764516, 20.84094480462498211 ) ) ;
#30139=CARTESIAN_POINT ( 'NONE',  ( 7.236395654485760609, 5.024999997268825069, -22.27133577429736633 ) ) ;
#30140=CARTESIAN_POINT ( 'NONE',  ( 33.58253175000000113, 20.37500000273118062, -4.112674001490185761E-15 ) ) ;
#30141=CARTESIAN_POINT ( 'NONE',  ( 20.08610463437157279, 25.80000000546239036, -27.64615127144129758 ) ) ;
#30142=CARTESIAN_POINT ( 'NONE',  ( -10.04305231718578462, 72.40000000000001990, 30.90933677959249337 ) ) ;
#30143=CARTESIAN_POINT ( 'NONE',  ( 10.04305231718579705, 33.10000000546236976, 30.90933677959248982 ) ) ;
#30146=CARTESIAN_POINT ( 'NONE',  ( -20.75514604977248112, 35.67500000273118843, 28.56700777964554661 ) ) ;
#30150=CARTESIAN_POINT ( 'NONE',  ( 14.47279130897151767, 9.424999997268814766, -19.92008829642072598 ) ) ;
#30151=CARTESIAN_POINT ( 'NONE',  ( -26.29305231718579350, 17.79999999999998295, -19.10302069950537884 ) ) ;
#30154=CARTESIAN_POINT ( 'NONE',  ( 33.58253175000000113, 58.22500000273116427, -10.91162601494193751 ) ) ;
#30155=CARTESIAN_POINT ( 'NONE',  ( 27.16883889988624290, 48.17500000273117422, 19.73931689729373673 ) ) ;
#30157=DIRECTION ( 'NONE',  ( 1.000000000000000000, 0.000000000000000000, -0.000000000000000000 ) ) ;
#30158=CARTESIAN_POINT ( 'NONE',  ( -5.147494310547430452, 5.551254281546842861, -32.49999999999999289 ) ) ;
#30166=CARTESIAN_POINT ( 'NONE',  ( 26.29305231718578995, 41.70000000546237118, -19.10302069950538240 ) ) ;
#30169=CARTESIAN_POINT ( 'NONE',  ( 32.50000000000000711, 34.89999999999999858, 10.55989012756945122 ) ) ;
#30170=CARTESIAN_POINT ( 'NONE',  ( -2.162160676586882350E-15, 32.62500000273119838, -35.31076352940722529 ) ) ;
#30173=EDGE_LOOP ( 'NONE', ( #29218, #16573, #29388, #18105 ) ) ;
#30181=CARTESIAN_POINT ( 'NONE',  ( -10.37757302488624411, 42.97500000273119269, -31.93888565452638417 ) ) ;
#30183=CARTESIAN_POINT ( 'NONE',  ( 26.29305231718578995, 41.70000000546237118, -19.10302069950538240 ) ) ;
#30185=CARTESIAN_POINT ( 'NONE',  ( -27.16883889988624290, 26.92500000273118133, -19.73931689729374028 ) ) ;
#30186=LINE ( 'NONE', #4286, #31305 ) ;
#30187=CARTESIAN_POINT ( 'NONE',  ( -10.37757302488623701, 53.77500000273119696, 31.93888565452638417 ) ) ;
#30190=CARTESIAN_POINT ( 'NONE',  ( 10.04305231718579705, 34.59999999999999432, 30.90933677959248982 ) ) ;
#30192=CARTESIAN_POINT ( 'NONE',  ( -20.75514604977248823, 72.82500000273118701, -28.56700777964554305 ) ) ;
#30193=CARTESIAN_POINT ( 'NONE',  ( 0.000000000000000000, 0.000000000000000000, 24.50000000000000000 ) ) ;
#30194=AXIS2_PLACEMENT_3D ( 'NONE', #2878, #31357, #7513 ) ;
#30197=CARTESIAN_POINT ( 'NONE',  ( -20.75514604977248112, 63.67500000273117422, 28.56700777964554661 ) ) ;
#30200=CARTESIAN_POINT ( 'NONE',  ( 7.570916362186213000, 6.149999994537635573, -23.30088464923126423 ) ) ;
#30203=CARTESIAN_POINT ( 'NONE',  ( 24.50000000000000000, 7.849999994537627757, -7.960532557706203605 ) ) ;
#30214=CARTESIAN_POINT ( 'NONE',  ( 0.000000000000000000, 0.000000000000000000, 0.000000000000000000 ) ) ;
#30215=CARTESIAN_POINT ( 'NONE',  ( 26.29305231718579350, 58.80000000000001847, 19.10302069950537529 ) ) ;
#30224=CARTESIAN_POINT ( 'NONE',  ( -5.147494310547418017, 74.05125428700922896, -32.50000000000000000 ) ) ;
#30225=CARTESIAN_POINT ( 'NONE',  ( -33.58253175000000113, 51.22500000273119269, 10.91162601494193929 ) ) ;
#30227=CARTESIAN_POINT ( 'NONE',  ( 10.04305231718578817, 11.90000000546237402, -30.90933677959249337 ) ) ;
#30228=CARTESIAN_POINT ( 'NONE',  ( 18.94512977948575738, 16.92499999726882010, 13.76444248337723408 ) ) ;
#30229=CARTESIAN_POINT ( 'NONE',  ( 32.50000000000000000, 52.99999999999999289, -3.980102097228898626E-15 ) ) ;
#30231=CARTESIAN_POINT ( 'NONE',  ( 33.58253175000000113, 14.37500000273117529, -4.112674001490185761E-15 ) ) ;
#30233=CARTESIAN_POINT ( 'NONE',  ( -11.25946833292375793, 76.67500000273119554, -8.180482586598733619 ) ) ;
#30237=ORIENTED_EDGE ( 'NONE', *, *, #337, .T. ) ;
#30244=CARTESIAN_POINT ( 'NONE',  ( 20.75514604977249178, 12.07500000273120477, 28.56700777964553950 ) ) ;
#30248=EDGE_CURVE ( 'NONE', #33045, #14454, #5160, .T. ) ;
#30249=CARTESIAN_POINT ( 'NONE',  ( 4.300734207923761154, 71.97500000273119269, 13.23629886949340495 ) ) ;
#30252=CARTESIAN_POINT ( 'NONE',  ( 33.58253175000000113, 54.22500000273117848, -10.91162601494193574 ) ) ;
#30256=CARTESIAN_POINT ( 'NONE',  ( 26.29305231718578995, 17.19999999999999218, -19.10302069950538240 ) ) ;
#30257=AXIS2_PLACEMENT_3D ( 'NONE', #8570, #16313, #19218 ) ;
#30258=VECTOR ( 'NONE', #22454, 1000.000000000000000 ) ;
#30259=CARTESIAN_POINT ( 'NONE',  ( -23.41746825000000243, 13.52499999726880198, -7.608796670333730638 ) ) ;
#30261=VERTEX_POINT ( 'NONE', #31239 ) ;
#30263=VECTOR ( 'NONE', #24960, 1000.000000000000000 ) ;
#30264=DIRECTION ( 'NONE',  ( -0.000000000000000000, 1.000000000000000000, -0.000000000000000000 ) ) ;
#30268=CARTESIAN_POINT ( 'NONE',  ( 27.16883889988623935, 60.57500000273119412, -19.73931689729374384 ) ) ;
#30269=CARTESIAN_POINT ( 'NONE',  ( 5.779280353836490358E-15, 37.00000000546237544, 32.49999999999999289 ) ) ;
#30270=CARTESIAN_POINT ( 'NONE',  ( 20.75514604977249178, 67.82500000273120122, 28.56700777964553950 ) ) ;
#30272=CARTESIAN_POINT ( 'NONE',  ( -19.82091636218621389, 15.19999999999999218, 14.40073868116558842 ) ) ;
#30273=CARTESIAN_POINT ( 'NONE',  ( 20.75514604977249178, 4.075000002731195892, 28.56700777964553950 ) ) ;
#30274=CARTESIAN_POINT ( 'NONE',  ( -33.58253175000000113, 7.125000002731196602, 0.000000000000000000 ) ) ;
#30275=CARTESIAN_POINT ( 'NONE',  ( -11.25946833292375793, 75.07500000273120122, 8.180482586598737171 ) ) ;
#30277=CARTESIAN_POINT ( 'NONE',  ( 15.00000000000000355, 76.89999999999999147, 4.873795443493592394 ) ) ;
#30279=CARTESIAN_POINT ( 'NONE',  ( 5.779280353836490358E-15, 67.00000000546236834, 32.49999999999999289 ) ) ;
#30281=CARTESIAN_POINT ( 'NONE',  ( -4.635254915624208216, 78.65000000546237402, 14.26584774442730463 ) ) ;
#30283=CARTESIAN_POINT ( 'NONE',  ( -33.58253175000000113, 39.02500000273118985, -10.91162601494193218 ) ) ;
#30284=VECTOR ( 'NONE', #5105, 1000.000000000000000 ) ;
#30287=CARTESIAN_POINT ( 'NONE',  ( 27.16883889988624290, 28.17500000273118133, 19.73931689729373673 ) ) ;
#30288=CARTESIAN_POINT ( 'NONE',  ( -32.50000000000000000, 67.89999999999997726, -10.55989012756945300 ) ) ;
#30290=CARTESIAN_POINT ( 'NONE',  ( 32.50000000000000711, 78.89999999999997726, 10.55989012756945122 ) ) ;
#30292=CARTESIAN_POINT ( 'NONE',  ( 23.41746824999999887, 10.72499999726880127, -7.608796670333727974 ) ) ;
#30296=CYLINDRICAL_SURFACE ( 'NONE', #28805, 32.50000000000000000 ) ;
#30297=CARTESIAN_POINT ( 'NONE',  ( 27.16883889988623935, 16.32500000273118346, -19.73931689729374384 ) ) ;
#30298=CARTESIAN_POINT ( 'NONE',  ( 18.94512977948575738, 10.92499999726881299, 13.76444248337723408 ) ) ;
#30300=ADVANCED_FACE ( 'NONE', ( #15470 ), #18727, .T. ) ;
#30303=EDGE_CURVE ( 'NONE', #10039, #7495, #15645, .T. ) ;
#30305=EDGE_LOOP ( 'NONE', ( #25338, #21355 ) ) ;
#30309=CARTESIAN_POINT ( 'NONE',  ( 15.14183272437241889, 15.44999999453761852, 20.84094480462498211 ) ) ;
#30310=AXIS2_PLACEMENT_3D ( 'NONE', #11243, #23955, #924 ) ;
#30311=EDGE_CURVE ( 'NONE', #8544, #3811, #1279, .T. ) ;
#30312=CARTESIAN_POINT ( 'NONE',  ( -18.94512977948575738, 11.42499999726881477, -13.76444248337723231 ) ) ;
#30313=CARTESIAN_POINT ( 'NONE',  ( -2.162160676586881955E-15, 22.87500000273118062, -35.31076352940723240 ) ) ;
#30314=CARTESIAN_POINT ( 'NONE',  ( 32.50000000000000711, 23.40000000546237047, 10.55989012756945122 ) ) ;
#30315=CARTESIAN_POINT ( 'NONE',  ( 10.04305231718579705, 72.59999999999999432, 30.90933677959248982 ) ) ;
#30316=CARTESIAN_POINT ( 'NONE',  ( -32.50000000000000000, 6.400000005462388231, -10.55989012756945300 ) ) ;
#30319=CARTESIAN_POINT ( 'NONE',  ( 33.58253175000000113, 34.37500000273119127, -4.112674001490185761E-15 ) ) ;
#30323=CARTESIAN_POINT ( 'NONE',  ( 7.236395654485760609, 11.52499999726880375, -22.27133577429736633 ) ) ;
#30324=CARTESIAN_POINT ( 'NONE',  ( -32.50000000000000000, 14.00000000000001243, 0.000000000000000000 ) ) ;
#30325=CARTESIAN_POINT ( 'NONE',  ( 26.29305231718578995, 9.700000005462394270, -19.10302069950538240 ) ) ;
#30327=CARTESIAN_POINT ( 'NONE',  ( 10.37757302488624056, 58.52500000273119696, -31.93888565452638417 ) ) ;
#30328=CARTESIAN_POINT ( 'NONE',  ( -20.75514604977248112, 49.67500000273118133, 28.56700777964554661 ) ) ;
#30330=DIRECTION ( 'NONE',  ( -0.000000000000000000, -1.000000000000000000, -0.000000000000000000 ) ) ;
#30331=CARTESIAN_POINT ( 'NONE',  ( -20.08610463437157989, 5.699999999999993960, -27.64615127144129758 ) ) ;
#30336=CARTESIAN_POINT ( 'NONE',  ( 3.735172737399427541E-15, 0.000000000000000000, 30.50000000000000000 ) ) ;
#30337=AXIS2_PLACEMENT_3D ( 'NONE', #18213, #13050, #26089 ) ;
#30339=CARTESIAN_POINT ( 'NONE',  ( 32.50000000000000711, 41.40000000546238823, 10.55989012756945122 ) ) ;
#30342=CARTESIAN_POINT ( 'NONE',  ( -10.37757302488624411, 30.72500000273117848, -31.93888565452638417 ) ) ;
#30344=ORIENTED_EDGE ( 'NONE', *, *, #8175, .F. ) ;
#30347=CARTESIAN_POINT ( 'NONE',  ( 0.000000000000000000, 0.000000000000000000, 0.000000000000000000 ) ) ;
#30348=ORIENTED_EDGE ( 'NONE', *, *, #31376, .T. ) ;
#30353=CARTESIAN_POINT ( 'NONE',  ( -32.50000000000000000, 64.40000000546238823, -10.55989012756945300 ) ) ;
#30354=CARTESIAN_POINT ( 'NONE',  ( -33.58253175000000113, 43.47500000273117138, 10.91162601494193929 ) ) ;
#30355=CARTESIAN_POINT ( 'NONE',  ( -32.50000000000000000, 42.40000000546238823, -10.55989012756945478 ) ) ;
#30357=CARTESIAN_POINT ( 'NONE',  ( 20.75514604977249178, 27.82500000273116925, 28.56700777964553950 ) ) ;
#30358=CARTESIAN_POINT ( 'NONE',  ( -26.29305231718579350, 23.79999999999998650, -19.10302069950537884 ) ) ;
#30359=CARTESIAN_POINT ( 'NONE',  ( -2.162160676586881955E-15, 54.87500000273119127, -35.31076352940723240 ) ) ;
#30362=CARTESIAN_POINT ( 'NONE',  ( -20.08610463437156923, 34.29999999999998295, 27.64615127144130113 ) ) ;
#30364=CARTESIAN_POINT ( 'NONE',  ( 20.75514604977248467, 78.42500000273116711, -28.56700777964554305 ) ) ;
#30367=CARTESIAN_POINT ( 'NONE',  ( -10.37757302488624411, 66.97500000273117848, -31.93888565452638417 ) ) ;
#30369=ORIENTED_EDGE ( 'NONE', *, *, #9396, .F. ) ;
#30370=CARTESIAN_POINT ( 'NONE',  ( -15.14183272437242600, 9.049999994537618164, 20.84094480462497856 ) ) ;
#30372=CARTESIAN_POINT ( 'NONE',  ( -10.04305231718579172, 25.60000000000001208, -30.90933677959248982 ) ) ;
#30382=CARTESIAN_POINT ( 'NONE',  ( -32.50000000000000000, 57.99999999999999289, 0.000000000000000000 ) ) ;
#30383=CARTESIAN_POINT ( 'NONE',  ( -2.092463501923844636E-15, 74.00000000546236834, -34.17252228774368916 ) ) ;
#30386=CARTESIAN_POINT ( 'NONE',  ( 5.779280353836490358E-15, 76.49999999999998579, 32.49999999999999289 ) ) ;
#30387=ORIENTED_EDGE ( 'NONE', *, *, #11880, .T. ) ;
#30389=ORIENTED_EDGE ( 'NONE', *, *, #6000, .T. ) ;
#30391=CARTESIAN_POINT ( 'NONE',  ( -10.04305231718579172, 62.10000000546239818, -30.90933677959248982 ) ) ;
#30394=CARTESIAN_POINT ( 'NONE',  ( 32.50000000000000000, 27.09999999999998721, -10.55989012756945833 ) ) ;
#30395=CARTESIAN_POINT ( 'NONE',  ( 10.37757302488624767, 45.72500000273119269, 31.93888565452638417 ) ) ;
#30396=CARTESIAN_POINT ( 'NONE',  ( 4.635254915624209993, 73.65000000546240244, -14.26584774442730463 ) ) ;
#30398=EDGE_CURVE ( 'NONE', #26987, #5934, #14589, .T. ) ;
#30399=CARTESIAN_POINT ( 'NONE',  ( 10.04305231718579705, 7.100000005462375974, 30.90933677959248982 ) ) ;
#30401=CARTESIAN_POINT ( 'NONE',  ( -18.94512977948576093, 12.32499999726882578, 13.76444248337722698 ) ) ;
#30403=CARTESIAN_POINT ( 'NONE',  ( -10.04305231718579172, 51.60000000000000853, -30.90933677959248982 ) ) ;
#30405=( BOUNDED_CURVE ( )  B_SPLINE_CURVE ( 2, ( #33477, #11905, #1085, #24944, #11733, #17883, #32493, #23191, #9316, #16898, #28166, #25761, #19803 ),
 .UNSPECIFIED., .F., .T. ) 
 B_SPLINE_CURVE_WITH_KNOTS ( ( 3, 2, 2, 2, 2, 2, 3 ),
 ( 0.02777777777777777624, 0.03333333333333333287, 0.04444444444444444614, 0.05555555555555555247, 0.06666666666666667962, 0.07777777777777777901, 0.08333333333333334259 ),
 .UNSPECIFIED. ) 
 CURVE ( )  GEOMETRIC_REPRESENTATION_ITEM ( )  RATIONAL_B_SPLINE_CURVE ( ( 0.9755282581475768211, 0.9755282581475768211, 1.000000000000000000, 0.9510565162951535312, 1.000000000000000000, 0.9510565162951535312, 1.000000000000000000, 0.9510565162951535312, 1.000000000000000000, 0.9510565162951535312, 1.000000000000000000, 0.9755282581475767101, 0.9755282581475768211 ) ) 
 REPRESENTATION_ITEM ( '' )  );
#30406=CARTESIAN_POINT ( 'NONE',  ( 33.58253175000000113, 18.37500000273117706, -4.112674001490185761E-15 ) ) ;
#30407=CARTESIAN_POINT ( 'NONE',  ( -5.147494310547423346, 74.44874571845315359, 32.50000000000000000 ) ) ;
#30409=CARTESIAN_POINT ( 'NONE',  ( 8.601468415847520532, 71.57500000273118701, 11.83890561707634781 ) ) ;
#30410=CARTESIAN_POINT ( 'NONE',  ( -5.147494310547423346, 44.44874571845313938, 32.50000000000000000 ) ) ;
#30414=CARTESIAN_POINT ( 'NONE',  ( 0.000000000000000000, 80.00000000000001421, -32.50000000000000000 ) ) ;
#30419=DIRECTION ( 'NONE',  ( 0.000000000000000000, 0.000000000000000000, -1.000000000000000000 ) ) ;
#30423=CARTESIAN_POINT ( 'NONE',  ( 20.08610463437157279, 69.29999999999999716, -27.64615127144129758 ) ) ;
#30425=CARTESIAN_POINT ( 'NONE',  ( 27.16883889988623935, 50.32500000273118701, -19.73931689729374384 ) ) ;
#30427=CARTESIAN_POINT ( 'NONE',  ( 26.29305231718578995, 21.70000000546237828, -19.10302069950538240 ) ) ;
#30428=VECTOR ( 'NONE', #13331, 1000.000000000000000 ) ;
#30429=ORIENTED_EDGE ( 'NONE', *, *, #15361, .F. ) ;
#30431=CARTESIAN_POINT ( 'NONE',  ( -32.50000000000000000, 2.000000000000001776, 0.000000000000000000 ) ) ;
#30432=CARTESIAN_POINT ( 'NONE',  ( -14.47279130897152122, 9.924999997268825425, 19.92008829642072243 ) ) ;
#30436=CARTESIAN_POINT ( 'NONE',  ( -32.50000000000000000, 34.40000000546237402, -10.55989012756945300 ) ) ;
#30438=VERTEX_POINT ( 'NONE', #32245 ) ;
#30442=CARTESIAN_POINT ( 'NONE',  ( -33.58253175000000113, 67.02500000273117564, -10.91162601494193218 ) ) ;
#30444=CARTESIAN_POINT ( 'NONE',  ( 19.82091636218621389, 12.19999999999998863, -14.40073868116559197 ) ) ;
#30445=CARTESIAN_POINT ( 'NONE',  ( 20.75514604977248467, 4.675000002731176885, -28.56700777964554305 ) ) ;
#30446=CARTESIAN_POINT ( 'NONE',  ( -2.162160676586881955E-15, 10.62500000273119127, -35.31076352940723240 ) ) ;
#30447=CARTESIAN_POINT ( 'NONE',  ( 2.688165632520823219E-15, 73.37500000273118417, 14.63369212191046209 ) ) ;
#30449=CARTESIAN_POINT ( 'NONE',  ( 12.13525491562420910, 77.19999999999998863, -8.816778784387098611 ) ) ;
#30452=CARTESIAN_POINT ( 'NONE',  ( 20.08610463437158344, 61.20000000546237118, 27.64615127144129403 ) ) ;
#30454=CARTESIAN_POINT ( 'NONE',  ( -4.635254915624208216, 74.65000000546240244, 14.26584774442730463 ) ) ;
#30456=CARTESIAN_POINT ( 'NONE',  ( -2.162160676586881955E-15, 36.62500000273119127, -35.31076352940723240 ) ) ;
#30459=CARTESIAN_POINT ( 'NONE',  ( -10.37757302488624411, 22.97500000273117138, -31.93888565452638417 ) ) ;
#30460=CARTESIAN_POINT ( 'NONE',  ( -20.08610463437157989, 12.20000000546237828, -27.64615127144129758 ) ) ;
#30462=CARTESIAN_POINT ( 'NONE',  ( 12.13525491562420910, 81.19999999999998863, -8.816778784387098611 ) ) ;
#30464=CARTESIAN_POINT ( 'NONE',  ( -7.236395654485763274, 8.024999997268800200, 22.27133577429736633 ) ) ;
#30469=CARTESIAN_POINT ( 'NONE',  ( 33.58253175000000113, 10.12500000273119838, -4.112674001490185761E-15 ) ) ;
#30470=CARTESIAN_POINT ( 'NONE',  ( 14.47279130897151767, 15.42499999726882898, -19.92008829642072598 ) ) ;
#30472=ORIENTED_EDGE ( 'NONE', *, *, #19118, .F. ) ;
#30479=CARTESIAN_POINT ( 'NONE',  ( 15.14183272437241889, 13.44999999453762385, 20.84094480462498211 ) ) ;
#30480=CARTESIAN_POINT ( 'NONE',  ( 23.41746824999999887, 10.62499999726881938, 0.000000000000000000 ) ) ;
#30481=CARTESIAN_POINT ( 'NONE',  ( 33.58253175000000113, 24.47500000273118914, -10.91162601494193751 ) ) ;
#30482=CARTESIAN_POINT ( 'NONE',  ( -26.29305231718578995, 22.70000000546237828, 19.10302069950538595 ) ) ;
#30483=CARTESIAN_POINT ( 'NONE',  ( -26.29305231718579350, 67.79999999999999716, -19.10302069950537884 ) ) ;
#30484=CARTESIAN_POINT ( 'NONE',  ( 5.147494310547434893, 47.05125428700922896, 32.49999999999999289 ) ) ;
#30487=CARTESIAN_POINT ( 'NONE',  ( -20.75514604977248823, 37.07500000273120122, -28.56700777964554305 ) ) ;
#30488=DIRECTION ( 'NONE',  ( -0.000000000000000000, -1.000000000000000000, -0.000000000000000000 ) ) ;
#30491=CARTESIAN_POINT ( 'NONE',  ( -23.41746825000000598, 16.22499999726880304, 7.608796670333726198 ) ) ;
#30492=CARTESIAN_POINT ( 'NONE',  ( -32.50000000000000000, 16.10000000000001563, 10.55989012756946366 ) ) ;
#30495=CARTESIAN_POINT ( 'NONE',  ( -20.75514604977248823, 54.82500000273118701, -28.56700777964554305 ) ) ;
#30497=CARTESIAN_POINT ( 'NONE',  ( 6.486482029760648627E-15, 45.87500000273118417, 35.31076352940722529 ) ) ;
#30499=CARTESIAN_POINT ( 'NONE',  ( 32.50000000000000000, 67.60000000546237686, -10.55989012756945833 ) ) ;
#30502=( BOUNDED_CURVE ( )  B_SPLINE_CURVE ( 2, ( #33070, #22446, #7518, #27770, #9392, #28448, #12144, #25021, #19876, #14901, #22617, #9576, #20053 ),
 .UNSPECIFIED., .F., .F. ) 
 B_SPLINE_CURVE_WITH_KNOTS ( ( 3, 2, 2, 2, 2, 2, 3 ),
 ( 0.4423076923076922906, 0.4435897435897435681, 0.4461538461538461786, 0.4487179487179487336, 0.4512820512820512886, 0.4538461538461538436, 0.4551282051282051211 ),
 .UNSPECIFIED. ) 
 CURVE ( )  GEOMETRIC_REPRESENTATION_ITEM ( )  RATIONAL_B_SPLINE_CURVE ( ( 0.9755282581475768211, 0.9755282581475768211, 1.000000000000000000, 0.9510565162951535312, 1.000000000000000000, 0.9510565162951535312, 1.000000000000000000, 0.9510565162951535312, 1.000000000000000000, 0.9510565162951535312, 1.000000000000000000, 0.9755282581475768211, 0.9755282581475768211 ) ) 
 REPRESENTATION_ITEM ( '' )  );
#30504=CARTESIAN_POINT ( 'NONE',  ( -32.50000000000000000, 42.00000000000000711, 0.000000000000000000 ) ) ;
#30506=CARTESIAN_POINT ( 'NONE',  ( 5.147494310547481966, 67.44874571845315359, -32.49999999999998579 ) ) ;
#30508=CARTESIAN_POINT ( 'NONE',  ( -32.50000000000000000, 78.50000000546236834, 0.000000000000000000 ) ) ;
#30511=LINE ( 'NONE', #7180, #5760 ) ;
#30512=CARTESIAN_POINT ( 'NONE',  ( 27.16883889988624290, 31.92500000273118488, 19.73931689729373673 ) ) ;
#30513=CARTESIAN_POINT ( 'NONE',  ( 33.58253175000000113, 64.47500000273120691, -10.91162601494193751 ) ) ;
#30519=ORIENTED_EDGE ( 'NONE', *, *, #23725, .T. ) ;
#30526=CARTESIAN_POINT ( 'NONE',  ( -33.58253175000000113, 39.27500000273118275, -10.91162601494193218 ) ) ;
#30527=CARTESIAN_POINT ( 'NONE',  ( -10.04305231718579172, 46.10000000546238397, -30.90933677959248982 ) ) ;
#30530=CARTESIAN_POINT ( 'NONE',  ( 33.58253175000000823, 28.02500000273119340, 10.91162601494192863 ) ) ;
#30531=CARTESIAN_POINT ( 'NONE',  ( 20.08610463437158344, 31.20000000546238894, 27.64615127144129403 ) ) ;
#30532=CARTESIAN_POINT ( 'NONE',  ( -33.58253175000000113, 57.47500000273119269, 10.91162601494193929 ) ) ;
#30533=EDGE_CURVE ( 'NONE', #22307, #17621, #8903, .T. ) ;
#30535=CARTESIAN_POINT ( 'NONE',  ( 26.29305231718578995, 35.20000000000000995, -19.10302069950538240 ) ) ;
#30537=CARTESIAN_POINT ( 'NONE',  ( -33.58253175000000113, 75.02500000273117564, -10.91162601494193218 ) ) ;
#30539=CARTESIAN_POINT ( 'NONE',  ( -32.50000000000000000, 20.40000000546238468, -10.55989012756945300 ) ) ;
#30540=CARTESIAN_POINT ( 'NONE',  ( 33.58253175000000113, 66.37500000273119838, -4.112674001490185761E-15 ) ) ;
#30543=VERTEX_POINT ( 'NONE', #5999 ) ;
#30544=CARTESIAN_POINT ( 'NONE',  ( 10.37757302488624767, 17.72500000273119625, 31.93888565452638417 ) ) ;
#30545=CARTESIAN_POINT ( 'NONE',  ( -24.50000000000000355, 10.64999999453762491, -7.960532557706207157 ) ) ;
#30547=CARTESIAN_POINT ( 'NONE',  ( -5.147494310547423346, 26.44874571845315714, 32.50000000000000000 ) ) ;
#30557=LINE ( 'NONE', #1555, #19262 ) ;
#30558=CARTESIAN_POINT ( 'NONE',  ( -32.50000000000000000, 74.50000000546236834, 0.000000000000000000 ) ) ;
#30562=VERTEX_POINT ( 'NONE', #24528 ) ;
#30563=CARTESIAN_POINT ( 'NONE',  ( 10.37757302488624767, 77.97500000273119269, 31.93888565452638417 ) ) ;
#30567=CARTESIAN_POINT ( 'NONE',  ( 20.08610463437157279, 63.80000000546237970, -27.64615127144129758 ) ) ;
#30568=ORIENTED_EDGE ( 'NONE', *, *, #27898, .T. ) ;
#30570=CARTESIAN_POINT ( 'NONE',  ( -20.75514604977248112, 51.42500000273118133, 28.56700777964554661 ) ) ;
#30571=CARTESIAN_POINT ( 'NONE',  ( -23.41746825000000243, 17.52499999726881796, -7.608796670333730638 ) ) ;
#30572=CARTESIAN_POINT ( 'NONE',  ( -26.29305231718579350, 8.300000005462383257, -19.10302069950537884 ) ) ;
#30573=CARTESIAN_POINT ( 'NONE',  ( -9.270509831248419985, 78.29999999999999716, 12.75976212528060039 ) ) ;
#30576=CARTESIAN_POINT ( 'NONE',  ( 10.04305231718579705, 50.60000000000000853, 30.90933677959248982 ) ) ;
#30577=DIRECTION ( 'NONE',  ( 0.000000000000000000, 0.000000000000000000, -1.000000000000000000 ) ) ;
#30578=CARTESIAN_POINT ( 'NONE',  ( 6.486482029760649416E-15, 17.87500000273119838, 35.31076352940723240 ) ) ;
#30581=CARTESIAN_POINT ( 'NONE',  ( 13.91746824999999887, 76.37500000273116996, -1.704398294459741270E-15 ) ) ;
#30585=VERTEX_POINT ( 'NONE', #13900 ) ;
#30587=CARTESIAN_POINT ( 'NONE',  ( 5.147494310547453544, 71.94874572391553613, -32.49999999999999289 ) ) ;
#30596=EDGE_CURVE ( 'NONE', #5893, #20206, #26723, .T. ) ;
#30597=LINE ( 'NONE', #7092, #33023 ) ;
#30599=CARTESIAN_POINT ( 'NONE',  ( 10.37757302488624767, 43.72500000273119269, 31.93888565452638417 ) ) ;
#30601=CARTESIAN_POINT ( 'NONE',  ( -8.891200544363830713E-16, 79.50000000000001421, -15.00000000000000000 ) ) ;
#30602=ORIENTED_EDGE ( 'NONE', *, *, #23499, .T. ) ;
#30604=CARTESIAN_POINT ( 'NONE',  ( -20.08610463437157989, 4.200000005462371178, -27.64615127144129758 ) ) ;
#30605=CARTESIAN_POINT ( 'NONE',  ( 23.41746824999999887, 12.62499999726882116, 0.000000000000000000 ) ) ;
#30609=CARTESIAN_POINT ( 'NONE',  ( -1.778240108872766143E-15, 70.00000000546238255, -32.49999999999999289 ) ) ;
#30610=VERTEX_POINT ( 'NONE', #19387 ) ;
#30612=CARTESIAN_POINT ( 'NONE',  ( 20.75514604977248467, 68.42500000273120975, -28.56700777964554305 ) ) ;
#30614=CARTESIAN_POINT ( 'NONE',  ( 15.14183272437242245, 12.29999999999999183, -20.84094480462497856 ) ) ;
#30615=CARTESIAN_POINT ( 'NONE',  ( 1.507698388325705758E-15, 1.624999997268798735, -24.62258325217400312 ) ) ;
#30616=CARTESIAN_POINT ( 'NONE',  ( 33.58253175000000113, 12.22500000273120158, -10.91162601494193751 ) ) ;
#30619=CARTESIAN_POINT ( 'NONE',  ( 9.270509831248423538, 75.30000000000001137, -12.75976212528059861 ) ) ;
#30622=CARTESIAN_POINT ( 'NONE',  ( -12.13525491562420910, 74.45000000546237118, 8.816778784387098611 ) ) ;
#30624=CARTESIAN_POINT ( 'NONE',  ( -4.635254915624211769, 75.85000000546237686, -14.26584774442730286 ) ) ;
#30626=CARTESIAN_POINT ( 'NONE',  ( -27.16883889988624290, 34.92500000273118843, -19.73931689729374028 ) ) ;
#30629=CARTESIAN_POINT ( 'NONE',  ( 20.75514604977249178, 22.07500000273117990, 28.56700777964553950 ) ) ;
#30631=CARTESIAN_POINT ( 'NONE',  ( 1.555960095263670572E-15, 14.24999999453762278, -24.50000000000000000 ) ) ;
#30633=CARTESIAN_POINT ( 'NONE',  ( 20.08610463437158344, 32.69999999999998863, 27.64615127144129403 ) ) ;
#30635=CARTESIAN_POINT ( 'NONE',  ( 18.94512977948576093, 10.82499999726882578, -13.76444248337722875 ) ) ;
#30636=CARTESIAN_POINT ( 'NONE',  ( 20.75514604977249178, 63.82500000273119412, 28.56700777964553950 ) ) ;
#30637=ADVANCED_FACE ( 'NONE', ( #27270 ), #29336, .T. ) ;
#30638=CARTESIAN_POINT ( 'NONE',  ( 2.667360163309149608E-15, 79.50000000000000000, -32.50000000000000000 ) ) ;
#30640=CARTESIAN_POINT ( 'NONE',  ( 33.58253175000000113, 12.22500000273119980, -10.91162601494193574 ) ) ;
#30641=CARTESIAN_POINT ( 'NONE',  ( 7.236395654485760609, 9.524999997268801977, -22.27133577429736633 ) ) ;
#30643=ORIENTED_EDGE ( 'NONE', *, *, #18179, .F. ) ;
#30651=CARTESIAN_POINT ( 'NONE',  ( -14.47279130897151589, 1.824999997268821339, -19.92008829642072598 ) ) ;
#30652=CARTESIAN_POINT ( 'NONE',  ( 14.47279130897151767, 10.92499999726882365, -19.92008829642072598 ) ) ;
#30653=CARTESIAN_POINT ( 'NONE',  ( 27.16883889988623935, 20.57500000273118701, -19.73931689729374384 ) ) ;
#30654=CARTESIAN_POINT ( 'NONE',  ( 20.08610463437157279, 23.80000000546235839, -27.64615127144129758 ) ) ;
#30655=CARTESIAN_POINT ( 'NONE',  ( -20.08610463437157989, 63.69999999999998863, -27.64615127144129758 ) ) ;
#30659=CARTESIAN_POINT ( 'NONE',  ( 10.37757302488624767, 27.97500000273117493, 31.93888565452638417 ) ) ;
#30660=CARTESIAN_POINT ( 'NONE',  ( -13.91746824999999532, 81.27500000273120406, -4.522059556121115875 ) ) ;
#30663=CARTESIAN_POINT ( 'NONE',  ( -3.880418787951136039, 0.5512542815468468582, -24.50000000000000000 ) ) ;
#30664=CARTESIAN_POINT ( 'NONE',  ( 20.08610463437157279, 11.29999999999999361, -27.64615127144129758 ) ) ;
#30665=CARTESIAN_POINT ( 'NONE',  ( 10.04305231718578817, 9.900000005462372243, -30.90933677959249337 ) ) ;
#30667=CARTESIAN_POINT ( 'NONE',  ( 27.16883889988624290, 57.92500000273120975, 19.73931689729373673 ) ) ;
#30669=CARTESIAN_POINT ( 'NONE',  ( 33.58253175000000113, 38.47500000273118559, -10.91162601494193574 ) ) ;
#30671=CARTESIAN_POINT ( 'NONE',  ( 20.08610463437157279, 67.80000000546236549, -27.64615127144129758 ) ) ;
#30672=CARTESIAN_POINT ( 'NONE',  ( -26.29305231718578995, 6.199999999999983302, 19.10302069950538595 ) ) ;
#30675=CARTESIAN_POINT ( 'NONE',  ( -5.147494310547423346, 28.44874571845315714, 32.50000000000000000 ) ) ;
#30677=CYLINDRICAL_SURFACE ( 'NONE', #5642, 32.50000000000000000 ) ;
#30679=DIRECTION ( 'NONE',  ( -0.000000000000000000, -1.000000000000000000, -0.000000000000000000 ) ) ;
#30682=CARTESIAN_POINT ( 'NONE',  ( 10.04305231718578817, 11.39999999999999325, -30.90933677959249337 ) ) ;
#30683=CARTESIAN_POINT ( 'NONE',  ( 20.75514604977249178, 29.82500000273119767, 28.56700777964553950 ) ) ;
#30684=CARTESIAN_POINT ( 'NONE',  ( -10.37757302488623701, 63.77500000273117564, 31.93888565452638417 ) ) ;
#30686=VERTEX_POINT ( 'NONE', #19555 ) ;
#30690=DIRECTION ( 'NONE',  ( -0.000000000000000000, 1.000000000000000000, -0.000000000000000000 ) ) ;
#30691=ORIENTED_EDGE ( 'NONE', *, *, #26853, .T. ) ;
#30695=EDGE_CURVE ( 'NONE', #30610, #13948, #2781, .T. ) ;
#30697=CARTESIAN_POINT ( 'NONE',  ( 0.000000000000000000, 80.00000000000001421, -32.50000000000000000 ) ) ;
#30698=CARTESIAN_POINT ( 'NONE',  ( -33.58253175000000113, 39.37500000273119838, 0.000000000000000000 ) ) ;
#30699=CARTESIAN_POINT ( 'NONE',  ( 32.50000000000000711, 41.40000000546238823, 10.55989012756945122 ) ) ;
#30702=CARTESIAN_POINT ( 'NONE',  ( -33.58253175000000113, 23.22500000273117138, 10.91162601494193929 ) ) ;
#30704=CARTESIAN_POINT ( 'NONE',  ( 10.37757302488624767, 55.97500000273119980, 31.93888565452638417 ) ) ;
#30707=CARTESIAN_POINT ( 'NONE',  ( 32.50000000000000000, 27.09999999999999076, -10.55989012756945833 ) ) ;
#30710=CARTESIAN_POINT ( 'NONE',  ( 20.75514604977248467, 76.42500000273118133, -28.56700777964554305 ) ) ;
#30711=CARTESIAN_POINT ( 'NONE',  ( -20.08610463437157989, 70.20000000546237118, -27.64615127144129758 ) ) ;
#30712=CARTESIAN_POINT ( 'NONE',  ( -15.14183272437242067, 14.70000000000000107, -20.84094480462497856 ) ) ;
#30713=CARTESIAN_POINT ( 'NONE',  ( -33.58253175000000113, 61.37500000273119127, 0.000000000000000000 ) ) ;
#30716=CARTESIAN_POINT ( 'NONE',  ( 33.58253175000000113, 18.22500000273118559, -10.91162601494193751 ) ) ;
#30717=CARTESIAN_POINT ( 'NONE',  ( 7.570916362186213000, 8.149999994537637349, -23.30088464923126423 ) ) ;
#30719=CARTESIAN_POINT ( 'NONE',  ( 5.147494310547426899, 47.44874571845313938, -32.50000000000000000 ) ) ;
#30729=CARTESIAN_POINT ( 'NONE',  ( -23.41746825000000243, 2.024999997268815299, -7.608796670333730638 ) ) ;
#30731=CARTESIAN_POINT ( 'NONE',  ( -33.58253175000000113, 1.225000002731198467, 10.91162601494193929 ) ) ;
#30735=EDGE_LOOP ( 'NONE', ( #18650, #32003, #6086, #29434 ) ) ;
#30736=CARTESIAN_POINT ( 'NONE',  ( -27.16883889988624290, 77.17500000273119554, -19.73931689729374028 ) ) ;
#30740=CARTESIAN_POINT ( 'NONE',  ( -26.29305231718579350, 62.30000000546237260, -19.10302069950537884 ) ) ;
#30741=VERTEX_POINT ( 'NONE', #17316 ) ;
#30742=CARTESIAN_POINT ( 'NONE',  ( -7.570916362186215665, 13.14999999453761426, 23.30088464923126423 ) ) ;
#30743=CARTESIAN_POINT ( 'NONE',  ( -33.58253175000000113, 49.12500000273117706, 0.000000000000000000 ) ) ;
#30744=CARTESIAN_POINT ( 'NONE',  ( -18.94512977948576093, 15.82499999726880091, 13.76444248337722698 ) ) ;
#30746=CARTESIAN_POINT ( 'NONE',  ( -32.50000000000000000, 4.500000005462356789, 0.000000000000000000 ) ) ;
#30748=CARTESIAN_POINT ( 'NONE',  ( 7.890940483122900408E-14, 12.24999999453763166, -24.50000000000000000 ) ) ;
#30750=CARTESIAN_POINT ( 'NONE',  ( -20.08610463437156923, 50.30000000000001137, 27.64615127144130113 ) ) ;
#30751=CARTESIAN_POINT ( 'NONE',  ( -32.50000000000000000, 14.00000000000001243, 0.000000000000000000 ) ) ;
#30752=CARTESIAN_POINT ( 'NONE',  ( -27.16883889988623935, 15.57500000273118168, 19.73931689729374739 ) ) ;
#30753=CARTESIAN_POINT ( 'NONE',  ( -1.778240108872766143E-15, 24.00000000546237899, -32.49999999999999289 ) ) ;
#30755=CARTESIAN_POINT ( 'NONE',  ( 13.91746824999999532, 76.47500000273117848, -4.522059556121118540 ) ) ;
#30756=CARTESIAN_POINT ( 'NONE',  ( 2.375766604868043252, 75.69874572391552192, -14.99999999999999822 ) ) ;
#30757=CARTESIAN_POINT ( 'NONE',  ( -20.08610463437156923, 44.29999999999999716, 27.64615127144130113 ) ) ;
#30759=ORIENTED_EDGE ( 'NONE', *, *, #9981, .T. ) ;
#30767=CARTESIAN_POINT ( 'NONE',  ( 10.37757302488624767, 3.975000002731182924, 31.93888565452638417 ) ) ;
#30771=CARTESIAN_POINT ( 'NONE',  ( -1.778240108872766143E-15, 3.500000000000004441, -32.49999999999999289 ) ) ;
#30773=CIRCLE ( 'NONE', #18726, 30.50000000000000000 ) ;
#30774=CARTESIAN_POINT ( 'NONE',  ( 33.58253175000000113, 42.22500000273118559, -10.91162601494193574 ) ) ;
#30779=CARTESIAN_POINT ( 'NONE',  ( -26.29305231718578995, 4.700000005462390718, 19.10302069950538595 ) ) ;
#30781=CARTESIAN_POINT ( 'NONE',  ( 33.58253175000000823, 78.27500000273116143, 10.91162601494192863 ) ) ;
#30786=CYLINDRICAL_SURFACE ( 'NONE', #11656, 24.50000000000000000 ) ;
#30787=CARTESIAN_POINT ( 'NONE',  ( -33.58253175000000113, 69.12500000273119838, 0.000000000000000000 ) ) ;
#30789=CARTESIAN_POINT ( 'NONE',  ( 15.14183272437241889, 9.700000000000013500, 20.84094480462498211 ) ) ;
#30790=CARTESIAN_POINT ( 'NONE',  ( 14.47279130897151944, 5.424999997268823648, -19.92008829642072598 ) ) ;
#30791=CARTESIAN_POINT ( 'NONE',  ( 6.486482029760649416E-15, 11.62500000273118950, 35.31076352940723240 ) ) ;
#30792=CARTESIAN_POINT ( 'NONE',  ( 32.50000000000000000, 28.99999999999999645, -3.980102097228898626E-15 ) ) ;
#30794=CARTESIAN_POINT ( 'NONE',  ( -15.00000000000000000, 72.00000000000001421, 0.000000000000000000 ) ) ;
#30796=CARTESIAN_POINT ( 'NONE',  ( 32.50000000000000711, 19.40000000546238468, 10.55989012756945122 ) ) ;
#30797=CARTESIAN_POINT ( 'NONE',  ( -1.778240108872766143E-15, 23.49999999999999645, -32.49999999999999289 ) ) ;
#30799=CARTESIAN_POINT ( 'NONE',  ( 9.270509831248423538, 77.55000000546236549, -12.75976212528059861 ) ) ;
#30801=CARTESIAN_POINT ( 'NONE',  ( -10.37757302488623701, 33.52500000273117564, 31.93888565452638417 ) ) ;
#30802=CARTESIAN_POINT ( 'NONE',  ( -8.891200544363830713E-16, 73.75000000546239676, -15.00000000000000000 ) ) ;
#30804=CARTESIAN_POINT ( 'NONE',  ( 33.58253175000000823, 22.27500000273117209, 10.91162601494192685 ) ) ;
#30805=CARTESIAN_POINT ( 'NONE',  ( 33.58253175000000823, 74.02500000273120406, 10.91162601494192685 ) ) ;
#30806=CARTESIAN_POINT ( 'NONE',  ( -32.50000000000000000, 26.50000000546237544, 0.000000000000000000 ) ) ;
#30808=VECTOR ( 'NONE', #21381, 1000.000000000000000 ) ;
#30809=CARTESIAN_POINT ( 'NONE',  ( 14.47279130897151944, 14.92499999726881477, -19.92008829642072598 ) ) ;
#30810=CARTESIAN_POINT ( 'NONE',  ( -33.58253175000000113, 67.02500000273117564, -10.91162601494193041 ) ) ;
#30811=( BOUNDED_CURVE ( )  B_SPLINE_CURVE ( 2, ( #9707, #25152, #1628, #4047, #22753, #7129, #14521, #24980, #12106, #1464, #32528, #20014, #17609 ),
 .UNSPECIFIED., .F., .T. ) 
 B_SPLINE_CURVE_WITH_KNOTS ( ( 3, 2, 2, 2, 2, 2, 3 ),
 ( 0.8910256410256410797, 0.8923076923076923572, 0.8948717948717949122, 0.8974358974358974672, 0.9000000000000000222, 0.9025641025641025772, 0.9038461538461538547 ),
 .UNSPECIFIED. ) 
 CURVE ( )  GEOMETRIC_REPRESENTATION_ITEM ( )  RATIONAL_B_SPLINE_CURVE ( ( 0.9755282581475768211, 0.9755282581475778203, 1.000000000000000000, 0.9510565162951535312, 1.000000000000000000, 0.9510565162951535312, 1.000000000000000000, 0.9510565162951535312, 1.000000000000000000, 0.9510565162951535312, 1.000000000000000000, 0.9755282581475768211, 0.9755282581475768211 ) ) 
 REPRESENTATION_ITEM ( '' )  );
#30815=( BOUNDED_CURVE ( )  B_SPLINE_CURVE ( 2, ( #9128, #27665, #25438, #14628, #24915, #30394, #9289, #22019, #19610, #24748, #22689, #1224, #19773 ),
 .UNSPECIFIED., .F., .T. ) 
 B_SPLINE_CURVE_WITH_KNOTS ( ( 3, 2, 2, 2, 2, 2, 3 ),
 ( 0.6730769230769231282, 0.6743589743589744057, 0.6769230769230769607, 0.6794871794871795156, 0.6820512820512820706, 0.6846153846153846256, 0.6858974358974359031 ),
 .UNSPECIFIED. ) 
 CURVE ( )  GEOMETRIC_REPRESENTATION_ITEM ( )  RATIONAL_B_SPLINE_CURVE ( ( 0.9755282581475768211, 0.9755282581475778203, 1.000000000000000000, 0.9510565162951535312, 1.000000000000000000, 0.9510565162951535312, 1.000000000000000000, 0.9510565162951535312, 1.000000000000000000, 0.9510565162951535312, 1.000000000000000000, 0.9755282581475768211, 0.9755282581475768211 ) ) 
 REPRESENTATION_ITEM ( '' )  );
#30816=CARTESIAN_POINT ( 'NONE',  ( 27.16883889988624290, 3.925000002731188431, 19.73931689729373673 ) ) ;
#30817=CARTESIAN_POINT ( 'NONE',  ( 1.507698388325705758E-15, 13.62499999726882827, -24.62258325217400312 ) ) ;
#30827=CARTESIAN_POINT ( 'NONE',  ( 18.94512977948575738, 6.924999997268810326, 13.76444248337723408 ) ) ;
#30828=CARTESIAN_POINT ( 'NONE',  ( 23.41746825000000243, 10.72499999726880127, -7.608796670333727974 ) ) ;
#30829=CARTESIAN_POINT ( 'NONE',  ( 27.16883889988624290, 16.17500000273119909, 19.73931689729373673 ) ) ;
#30830=CARTESIAN_POINT ( 'NONE',  ( 20.08610463437157279, 27.80000000546238326, -27.64615127144129758 ) ) ;
#30833=CARTESIAN_POINT ( 'NONE',  ( -10.04305231718579172, 65.59999999999999432, -30.90933677959248982 ) ) ;
#30834=CARTESIAN_POINT ( 'NONE',  ( 24.50000000000000000, 11.64999999453762314, 7.960532557706212486 ) ) ;
#30837=CARTESIAN_POINT ( 'NONE',  ( -10.37757302488623701, 31.77500000273120051, 31.93888565452638417 ) ) ;
#30838=CARTESIAN_POINT ( 'NONE',  ( -11.25946833292375793, 81.17500000273119554, -8.180482586598733619 ) ) ;
#30842=CARTESIAN_POINT ( 'NONE',  ( -4.523095164977116484E-15, 14.62499999726882649, 24.62258325217400312 ) ) ;
#30843=CARTESIAN_POINT ( 'NONE',  ( -32.50000000000000000, 6.000000000000005329, 0.000000000000000000 ) ) ;
#30846=CARTESIAN_POINT ( 'NONE',  ( 20.75514604977249178, 51.82500000273120122, 28.56700777964553950 ) ) ;
#30848=CARTESIAN_POINT ( 'NONE',  ( -20.75514604977248823, 41.07500000273119412, -28.56700777964554305 ) ) ;
#30850=DIRECTION ( 'NONE',  ( -0.000000000000000000, 1.000000000000000000, -0.000000000000000000 ) ) ;
#30851=CARTESIAN_POINT ( 'NONE',  ( -20.75514604977248112, 1.425000002731191984, 28.56700777964554661 ) ) ;
#30859=CARTESIAN_POINT ( 'NONE',  ( -5.147494310547423346, 60.94874572391552192, 32.50000000000000000 ) ) ;
#30860=CARTESIAN_POINT ( 'NONE',  ( -33.58253175000000113, 27.12500000273118772, 0.000000000000000000 ) ) ;
#30862=VECTOR ( 'NONE', #4712, 1000.000000000000000 ) ;
#30863=ORIENTED_EDGE ( 'NONE', *, *, #10848, .T. ) ;
#30867=ORIENTED_EDGE ( 'NONE', *, *, #223, .T. ) ;
#30873=CARTESIAN_POINT ( 'NONE',  ( -33.58253175000000113, 33.37500000273119127, 0.000000000000000000 ) ) ;
#30874=CARTESIAN_POINT ( 'NONE',  ( -10.04305231718578462, 40.90000000546237402, 30.90933677959249337 ) ) ;
#30876=CARTESIAN_POINT ( 'NONE',  ( 20.75514604977248467, 24.42500000273119554, -28.56700777964554305 ) ) ;
#30877=CARTESIAN_POINT ( 'NONE',  ( -32.50000000000000000, 23.90000000000000213, -10.55989012756945300 ) ) ;
#30878=CARTESIAN_POINT ( 'NONE',  ( -33.58253175000000113, 49.27500000273118985, -10.91162601494193218 ) ) ;
#30882=CARTESIAN_POINT ( 'NONE',  ( -20.08610463437156923, 30.30000000000000426, 27.64615127144130113 ) ) ;
#30884=CARTESIAN_POINT ( 'NONE',  ( -2.162160676586881955E-15, 68.62500000273119838, -35.31076352940723240 ) ) ;
#30886=CARTESIAN_POINT ( 'NONE',  ( 0.000000000000000000, 0.000000000000000000, -30.50000000000000000 ) ) ;
#30887=CARTESIAN_POINT ( 'NONE',  ( 27.16883889988624290, 58.17500000273118133, 19.73931689729373673 ) ) ;
#30890=CARTESIAN_POINT ( 'NONE',  ( -10.04305231718578462, 40.90000000546237402, 30.90933677959249337 ) ) ;
#30891=CARTESIAN_POINT ( 'NONE',  ( 33.58253175000000113, 20.22500000273117848, -10.91162601494193751 ) ) ;
#30892=CARTESIAN_POINT ( 'NONE',  ( 19.82091636218621034, 9.549999994537621717, 14.40073868116559730 ) ) ;
#30894=CARTESIAN_POINT ( 'NONE',  ( -1.778240108872766143E-15, 47.49999999999999289, -32.49999999999999289 ) ) ;
#30900=DIRECTION ( 'NONE',  ( 0.000000000000000000, 1.000000000000000000, 0.000000000000000000 ) ) ;
#30906=CARTESIAN_POINT ( 'NONE',  ( -14.47279130897152122, 2.424999997268802332, 19.92008829642072243 ) ) ;
#30907=CARTESIAN_POINT ( 'NONE',  ( -32.50000000000000000, 76.40000000546235981, -10.55989012756945478 ) ) ;
#30912=CARTESIAN_POINT ( 'NONE',  ( 6.486482029760649416E-15, 75.87500000273119838, 35.31076352940723240 ) ) ;
#30915=CARTESIAN_POINT ( 'NONE',  ( 27.16883889988624290, 60.17500000273118133, 19.73931689729373673 ) ) ;
#30916=CARTESIAN_POINT ( 'NONE',  ( -10.04305231718578462, 60.90000000546235981, 30.90933677959249337 ) ) ;
#30917=ORIENTED_EDGE ( 'NONE', *, *, #15759, .F. ) ;
#30918=( BOUNDED_CURVE ( )  B_SPLINE_CURVE ( 2, ( #17445, #25153, #27906, #1805, #6959, #27394, #14695, #30290, #16937, #33030, #22755, #17270, #4560 ),
 .UNSPECIFIED., .F., .T. ) 
 B_SPLINE_CURVE_WITH_KNOTS ( ( 3, 2, 2, 2, 2, 2, 3 ),
 ( 0.006410256410256410901, 0.007692307692307692735, 0.01025641025641025640, 0.01282051282051282007, 0.01538461538461538547, 0.01794871794871794740, 0.01923076923076923184 ),
 .UNSPECIFIED. ) 
 CURVE ( )  GEOMETRIC_REPRESENTATION_ITEM ( )  RATIONAL_B_SPLINE_CURVE ( ( 0.9755282581475768211, 0.9755282581475768211, 1.000000000000000000, 0.9510565162951535312, 1.000000000000000000, 0.9510565162951535312, 1.000000000000000000, 0.9510565162951535312, 1.000000000000000000, 0.9510565162951535312, 1.000000000000000000, 0.9755282581475767101, 0.9755282581475768211 ) ) 
 REPRESENTATION_ITEM ( '' )  );
#30920=CARTESIAN_POINT ( 'NONE',  ( 27.16883889988624290, 41.92500000273119554, 19.73931689729373673 ) ) ;
#30921=CARTESIAN_POINT ( 'NONE',  ( 23.41746824999999887, 16.62499999726882294, 0.000000000000000000 ) ) ;
#30922=CARTESIAN_POINT ( 'NONE',  ( 33.58253175000000113, 66.37500000273119838, -4.112674001490185761E-15 ) ) ;
#30923=CARTESIAN_POINT ( 'NONE',  ( 10.04305231718578817, 3.900000005462367358, -30.90933677959249337 ) ) ;
#30925=DIRECTION ( 'NONE',  ( -0.000000000000000000, -1.000000000000000000, -0.000000000000000000 ) ) ;
#30926=CARTESIAN_POINT ( 'NONE',  ( 32.50000000000000000, 47.10000000000000142, -10.55989012756945833 ) ) ;
#30927=CARTESIAN_POINT ( 'NONE',  ( 15.14183272437242422, 2.299999999999985612, -20.84094480462497856 ) ) ;
#30928=CARTESIAN_POINT ( 'NONE',  ( 6.486482029760649416E-15, 19.87500000273119483, 35.31076352940723240 ) ) ;
#30929=CARTESIAN_POINT ( 'NONE',  ( 24.50000000000000000, 0.09999999999999682754, -7.960532557706203605 ) ) ;
#30931=CARTESIAN_POINT ( 'NONE',  ( -13.91746824999999887, 79.37500000273118417, 0.000000000000000000 ) ) ;
#30932=CARTESIAN_POINT ( 'NONE',  ( -10.37757302488623701, 77.77500000273118985, 31.93888565452638417 ) ) ;
#30933=CARTESIAN_POINT ( 'NONE',  ( 32.50000000000000000, 53.50000000546237544, -3.980102097228898626E-15 ) ) ;
#30935=ORIENTED_EDGE ( 'NONE', *, *, #11534, .F. ) ;
#30946=CARTESIAN_POINT ( 'NONE',  ( -4.300734207923755825, 71.77500000273117564, 13.23629886949340673 ) ) ;
#30948=CARTESIAN_POINT ( 'NONE',  ( 27.16883889988623935, 48.32500000273117990, -19.73931689729374384 ) ) ;
#30950=CARTESIAN_POINT ( 'NONE',  ( 15.00000000000000000, 79.10000000000000853, -4.873795443493596835 ) ) ;
#30955=CARTESIAN_POINT ( 'NONE',  ( 33.58253175000000113, 74.37500000273116996, -4.112674001490185761E-15 ) ) ;
#30959=( BOUNDED_CURVE ( )  B_SPLINE_CURVE ( 2, ( #32567, #1502, #28112, #30671, #16972, #30499, #19547, #1670, #17144, #19877, #29995, #22447, #9577 ),
 .UNSPECIFIED., .F., .T. ) 
 B_SPLINE_CURVE_WITH_KNOTS ( ( 3, 2, 2, 2, 2, 2, 3 ),
 ( 0.1346153846153846090, 0.1358974358974358865, 0.1384615384615384692, 0.1410256410256410242, 0.1435897435897435792, 0.1461538461538461620, 0.1474358974358974395 ),
 .UNSPECIFIED. ) 
 CURVE ( )  GEOMETRIC_REPRESENTATION_ITEM ( )  RATIONAL_B_SPLINE_CURVE ( ( 0.9755282581475768211, 0.9755282581475768211, 1.000000000000000000, 0.9510565162951535312, 1.000000000000000000, 0.9510565162951535312, 1.000000000000000000, 0.9510565162951535312, 1.000000000000000000, 0.9510565162951535312, 1.000000000000000000, 0.9755282581475768211, 0.9755282581475768211 ) ) 
 REPRESENTATION_ITEM ( '' )  );
#30961=CARTESIAN_POINT ( 'NONE',  ( -5.147494310547213736, 14.05125428700922541, -32.50000000000007105 ) ) ;
#30962=CARTESIAN_POINT ( 'NONE',  ( 20.75514604977249178, 59.82500000273117280, 28.56700777964553950 ) ) ;
#30964=CARTESIAN_POINT ( 'NONE',  ( -19.82091636218621389, 11.19999999999998863, 14.40073868116558842 ) ) ;
#30965=CARTESIAN_POINT ( 'NONE',  ( -18.94512977948575738, 3.924999997268807661, -13.76444248337723231 ) ) ;
#30967=CARTESIAN_POINT ( 'NONE',  ( -10.37757302488623701, 11.52500000273118452, 31.93888565452638417 ) ) ;
#30969=CARTESIAN_POINT ( 'NONE',  ( 5.147494310547426899, 37.44874571845314648, -32.50000000000000000 ) ) ;
#30971=CARTESIAN_POINT ( 'NONE',  ( 10.04305231718578817, 19.90000000546238113, -30.90933677959249337 ) ) ;
#30974=CARTESIAN_POINT ( 'NONE',  ( 13.91746825000000065, 79.77500000273118985, 4.522059556121114987 ) ) ;
#30976=CARTESIAN_POINT ( 'NONE',  ( -10.37757302488624411, 32.72500000273117848, -31.93888565452638417 ) ) ;
#30980=CARTESIAN_POINT ( 'NONE',  ( -20.75514604977248823, 21.07500000273118346, -28.56700777964554305 ) ) ;
#30981=CARTESIAN_POINT ( 'NONE',  ( -15.00000000000000000, 80.10000000000000853, 4.873795443493597723 ) ) ;
#30982=CARTESIAN_POINT ( 'NONE',  ( 10.37757302488624767, 75.72500000273119269, 31.93888565452638417 ) ) ;
#30983=VECTOR ( 'NONE', #13247, 1000.000000000000000 ) ;
#30984=CARTESIAN_POINT ( 'NONE',  ( 7.570916362186213000, 8.399999999999991473, -23.30088464923126423 ) ) ;
#30986=CARTESIAN_POINT ( 'NONE',  ( -18.94512977948576093, 15.82499999726880091, 13.76444248337722698 ) ) ;
#30987=CARTESIAN_POINT ( 'NONE',  ( -20.75514604977248823, 62.82500000273119412, -28.56700777964554305 ) ) ;
#30990=CARTESIAN_POINT ( 'NONE',  ( 6.486482029760648627E-15, 5.625000002731175286, 35.31076352940722529 ) ) ;
#30992=CARTESIAN_POINT ( 'NONE',  ( -18.94512977948575738, 1.424999997268805441, -13.76444248337723231 ) ) ;
#30994=AXIS2_PLACEMENT_3D ( 'NONE', #13655, #24120, #13819 ) ;
#30999=CARTESIAN_POINT ( 'NONE',  ( -32.50000000000000000, 80.00000000000001421, 0.000000000000000000 ) ) ;
#31001=CARTESIAN_POINT ( 'NONE',  ( -32.50000000000000000, 72.60000000546236265, 10.55989012756946366 ) ) ;
#31002=CARTESIAN_POINT ( 'NONE',  ( -18.94512977948575738, 1.924999997268805885, -13.76444248337723231 ) ) ;
#31003=CARTESIAN_POINT ( 'NONE',  ( 18.94512977948576093, 12.82499999726882578, -13.76444248337722875 ) ) ;
#31004=CARTESIAN_POINT ( 'NONE',  ( 10.37757302488624056, 12.77500000273118452, -31.93888565452638417 ) ) ;
#31005=CARTESIAN_POINT ( 'NONE',  ( 10.04305231718579705, 15.10000000546238219, 30.90933677959248982 ) ) ;
#31006=CARTESIAN_POINT ( 'NONE',  ( 26.29305231718579350, 62.79999999999999716, 19.10302069950537529 ) ) ;
#31007=CARTESIAN_POINT ( 'NONE',  ( 15.14183272437242422, 12.04999999453763948, -20.84094480462497856 ) ) ;
#31008=FACE_OUTER_BOUND ( 'NONE', #25085, .T. ) ;
#31010=CARTESIAN_POINT ( 'NONE',  ( 33.58253175000000823, 30.27500000273118630, 10.91162601494192863 ) ) ;
#31011=CARTESIAN_POINT ( 'NONE',  ( -20.08610463437157989, 32.20000000546238539, -27.64615127144129758 ) ) ;
#31013=CARTESIAN_POINT ( 'NONE',  ( -7.236395654485763274, 16.52499999726880731, 22.27133577429736633 ) ) ;
#31014=CARTESIAN_POINT ( 'NONE',  ( -2.092463501923844636E-15, 7.499999999999995559, -34.17252228774368916 ) ) ;
#31015=CARTESIAN_POINT ( 'NONE',  ( -9.270509831248419985, 74.30000000000001137, 12.75976212528060039 ) ) ;
#31017=CARTESIAN_POINT ( 'NONE',  ( -20.75514604977248112, 51.42500000273118133, 28.56700777964554661 ) ) ;
#31018=VECTOR ( 'NONE', #25062, 1000.000000000000000 ) ;
#31020=CARTESIAN_POINT ( 'NONE',  ( -33.58253175000000113, 41.47500000273117138, 10.91162601494193929 ) ) ;
#31021=( BOUNDED_CURVE ( )  B_SPLINE_CURVE ( 2, ( #23511, #29478, #27081, #26417, #21780, #5482, #13714, #14047, #487, #5982, #8383, #21283, #11302 ),
 .UNSPECIFIED., .F., .T. ) 
 B_SPLINE_CURVE_WITH_KNOTS ( ( 3, 2, 2, 2, 2, 2, 3 ),
 ( 0.3397435897435897578, 0.3410256410256410353, 0.3435897435897435903, 0.3461538461538461453, 0.3487179487179487003, 0.3512820512820512553, 0.3525641025641025883 ),
 .UNSPECIFIED. ) 
 CURVE ( )  GEOMETRIC_REPRESENTATION_ITEM ( )  RATIONAL_B_SPLINE_CURVE ( ( 0.9755282581475768211, 0.9755282581475768211, 1.000000000000000000, 0.9510565162951535312, 1.000000000000000000, 0.9510565162951535312, 1.000000000000000000, 0.9510565162951535312, 1.000000000000000000, 0.9510565162951535312, 1.000000000000000000, 0.9755282581475762660, 0.9755282581475768211 ) ) 
 REPRESENTATION_ITEM ( '' )  );
#31022=CARTESIAN_POINT ( 'NONE',  ( 0.000000000000000000, 70.00000000000000000, 26.50000000000000355 ) ) ;
#31023=CARTESIAN_POINT ( 'NONE',  ( 20.08610463437157279, 15.80000000546237970, -27.64615127144129758 ) ) ;
#31024=DIRECTION ( 'NONE',  ( 0.000000000000000000, 0.000000000000000000, -1.000000000000000000 ) ) ;
#31029=CARTESIAN_POINT ( 'NONE',  ( 0.000000000000000000, 0.000000000000000000, 0.000000000000000000 ) ) ;
#31030=CARTESIAN_POINT ( 'NONE',  ( -26.29305231718579350, 39.80000000000000426, -19.10302069950537884 ) ) ;
#31035=CARTESIAN_POINT ( 'NONE',  ( 27.16883889988623935, 24.32500000273119056, -19.73931689729374384 ) ) ;
#31038=ORIENTED_EDGE ( 'NONE', *, *, #19026, .F. ) ;
#31045=ORIENTED_EDGE ( 'NONE', *, *, #6084, .F. ) ;
#31050=CARTESIAN_POINT ( 'NONE',  ( -10.37757302488624411, 34.97500000273118559, -31.93888565452638417 ) ) ;
#31051=CARTESIAN_POINT ( 'NONE',  ( -32.50000000000000000, 34.50000000546238255, 0.000000000000000000 ) ) ;
#31054=CARTESIAN_POINT ( 'NONE',  ( -33.58253175000000113, 23.02500000273117919, -10.91162601494193218 ) ) ;
#31055=CARTESIAN_POINT ( 'NONE',  ( 5.147494310547217289, 31.05125428700920764, 32.50000000000007105 ) ) ;
#31056=CARTESIAN_POINT ( 'NONE',  ( 20.75514604977249178, 48.07500000273120122, 28.56700777964553950 ) ) ;
#31058=CARTESIAN_POINT ( 'NONE',  ( -10.04305231718578462, 24.40000000000000568, 30.90933677959249337 ) ) ;
#31060=CARTESIAN_POINT ( 'NONE',  ( 20.75514604977248467, 66.42500000273120975, -28.56700777964554305 ) ) ;
#31062=CARTESIAN_POINT ( 'NONE',  ( 33.58253175000000113, 62.47500000273118559, -10.91162601494193574 ) ) ;
#31063=CARTESIAN_POINT ( 'NONE',  ( -27.16883889988624290, 8.925000002731191984, -19.73931689729374028 ) ) ;
#31064=CARTESIAN_POINT ( 'NONE',  ( -7.570916362186210335, 12.34999999453761887, -23.30088464923126779 ) ) ;
#31074=ADVANCED_FACE ( 'NONE', ( #6507, #16980 ), #20919, .T. ) ;
#31079=CARTESIAN_POINT ( 'NONE',  ( 32.50000000000000000, 73.60000000546240528, -10.55989012756945833 ) ) ;
#31083=ORIENTED_EDGE ( 'NONE', *, *, #14693, .T. ) ;
#31084=CARTESIAN_POINT ( 'NONE',  ( 20.75514604977249178, 74.07500000273120122, 28.56700777964553950 ) ) ;
#31088=CARTESIAN_POINT ( 'NONE',  ( -33.58253175000000113, 51.27500000273118275, -10.91162601494193218 ) ) ;
#31089=CARTESIAN_POINT ( 'NONE',  ( 26.29305231718578995, 63.70000000546238539, -19.10302069950538240 ) ) ;
#31091=CARTESIAN_POINT ( 'NONE',  ( -10.37757302488624411, 42.72500000273119269, -31.93888565452638417 ) ) ;
#31092=CARTESIAN_POINT ( 'NONE',  ( 5.147494310547535257, 55.94874572391552903, -32.49999999999996447 ) ) ;
#31093=CARTESIAN_POINT ( 'NONE',  ( -2.162160676586881955E-15, 70.87500000273118417, -35.31076352940723240 ) ) ;
#31094=CARTESIAN_POINT ( 'NONE',  ( 26.29305231718578995, 3.700000005462389385, -19.10302069950538240 ) ) ;
#31096=CARTESIAN_POINT ( 'NONE',  ( 0.000000000000000000, 80.00000000000001421, -32.50000000000000000 ) ) ;
#31097=CARTESIAN_POINT ( 'NONE',  ( -20.08610463437157989, 47.70000000000000995, -27.64615127144129758 ) ) ;
#31099=CARTESIAN_POINT ( 'NONE',  ( 10.37757302488624767, 11.97500000273118914, 31.93888565452638417 ) ) ;
#31102=CARTESIAN_POINT ( 'NONE',  ( 4.300734207923761154, 77.97500000273119269, 13.23629886949340495 ) ) ;
#31103=CARTESIAN_POINT ( 'NONE',  ( -33.58253175000000113, 77.27500000273118985, -10.91162601494193041 ) ) ;
#31105=VECTOR ( 'NONE', #31426, 1000.000000000000000 ) ;
#31119=CARTESIAN_POINT ( 'NONE',  ( -5.147494310547322094, 56.05125428700922896, -32.50000000000003553 ) ) ;
#31121=CARTESIAN_POINT ( 'NONE',  ( 27.16883889988623935, 44.32500000273117990, -19.73931689729374384 ) ) ;
#31123=CARTESIAN_POINT ( 'NONE',  ( 5.779280353836490358E-15, 33.00000000546238965, 32.49999999999999289 ) ) ;
#31124=ORIENTED_EDGE ( 'NONE', *, *, #33712, .F. ) ;
#31127=CARTESIAN_POINT ( 'NONE',  ( -20.08610463437156923, 4.800000005462380592, 27.64615127144130113 ) ) ;
#31129=CARTESIAN_POINT ( 'NONE',  ( 10.37757302488624767, 77.97500000273119269, 31.93888565452638417 ) ) ;
#31130=ORIENTED_EDGE ( 'NONE', *, *, #3857, .F. ) ;
#31135=CARTESIAN_POINT ( 'NONE',  ( -1.778240108872766143E-15, 30.00000000546237189, -32.49999999999999289 ) ) ;
#31136=CARTESIAN_POINT ( 'NONE',  ( 6.486482029760649416E-15, 61.62500000273118417, 35.31076352940723240 ) ) ;
#31138=CARTESIAN_POINT ( 'NONE',  ( -4.732186688966233175E-15, 17.50000000000000000, 25.76082449383753925 ) ) ;
#31139=CARTESIAN_POINT ( 'NONE',  ( -14.47279130897152299, 2.424999997268802332, 19.92008829642072243 ) ) ;
#31140=CARTESIAN_POINT ( 'NONE',  ( 10.37757302488624056, 6.525000002731207616, -31.93888565452638417 ) ) ;
#31141=CARTESIAN_POINT ( 'NONE',  ( 2.067204126564591252E-14, 6.249999994537623671, -24.50000000000000000 ) ) ;
#31143=CARTESIAN_POINT ( 'NONE',  ( 33.58253175000000113, 78.47500000273116427, -10.91162601494193751 ) ) ;
#31145=CARTESIAN_POINT ( 'NONE',  ( 32.50000000000000000, 19.60000000546238041, -10.55989012756945833 ) ) ;
#31149=CARTESIAN_POINT ( 'NONE',  ( -4.635254915624208216, 70.65000000546240244, 14.26584774442730463 ) ) ;
#31151=CARTESIAN_POINT ( 'NONE',  ( -33.58253175000000113, 29.02500000273119340, -10.91162601494193218 ) ) ;
#31154=CARTESIAN_POINT ( 'NONE',  ( 33.58253175000000113, 22.47500000273119269, -10.91162601494193574 ) ) ;
#31156=CARTESIAN_POINT ( 'NONE',  ( 33.58253175000000113, 76.12500000273119838, -4.112674001490185761E-15 ) ) ;
#31157=CARTESIAN_POINT ( 'NONE',  ( -26.29305231718578995, 26.70000000546238184, 19.10302069950538595 ) ) ;
#31159=CARTESIAN_POINT ( 'NONE',  ( -14.47279130897151767, 15.32499999726880269, -19.92008829642072598 ) ) ;
#31160=CARTESIAN_POINT ( 'NONE',  ( -2.162160676586882350E-15, 66.62500000273119838, -35.31076352940722529 ) ) ;
#31163=CARTESIAN_POINT ( 'NONE',  ( 20.75514604977249178, 9.825000002731188786, 28.56700777964553950 ) ) ;
#31164=CARTESIAN_POINT ( 'NONE',  ( -4.523095164977116484E-15, 16.62499999726881583, 24.62258325217400312 ) ) ;
#31166=ADVANCED_FACE ( 'NONE', ( #10104 ), #31202, .T. ) ;
#31172=CARTESIAN_POINT ( 'NONE',  ( 33.58253175000000823, 78.02500000273118985, 10.91162601494192863 ) ) ;
#31173=CARTESIAN_POINT ( 'NONE',  ( -4.523095164977116484E-15, 4.624999997268820273, 24.62258325217400312 ) ) ;
#31176=CARTESIAN_POINT ( 'NONE',  ( -23.41746824999999887, 17.62499999726882649, -2.867812753649727150E-15 ) ) ;
#31177=CARTESIAN_POINT ( 'NONE',  ( 33.58253175000000113, 18.37500000273117706, -4.112674001490185761E-15 ) ) ;
#31178=CARTESIAN_POINT ( 'NONE',  ( 32.50000000000000000, 17.50000000546236834, -3.980102097228898626E-15 ) ) ;
#31179=CARTESIAN_POINT ( 'NONE',  ( 10.04305231718578817, 65.40000000000001990, -30.90933677959249337 ) ) ;
#31187=LINE ( 'NONE', #10769, #4195 ) ;
#31188=CARTESIAN_POINT ( 'NONE',  ( -18.94512977948576093, 18.32499999726880446, 13.76444248337722698 ) ) ;
#31189=CARTESIAN_POINT ( 'NONE',  ( -20.08610463437157989, 5.699999999999993960, -27.64615127144129758 ) ) ;
#31190=CARTESIAN_POINT ( 'NONE',  ( 32.50000000000000000, 17.50000000546236834, -3.980102097228898626E-15 ) ) ;
#31192=CARTESIAN_POINT ( 'NONE',  ( 6.486482029760649416E-15, 49.62500000273117706, 35.31076352940723240 ) ) ;
#31194=CARTESIAN_POINT ( 'NONE',  ( -33.58253175000000113, 43.37500000273119838, 0.000000000000000000 ) ) ;
#31195=CARTESIAN_POINT ( 'NONE',  ( 5.147494310547426899, 23.94874572391553968, -32.50000000000000000 ) ) ;
#31197=LINE ( 'NONE', #2370, #21831 ) ;
#31198=CARTESIAN_POINT ( 'NONE',  ( -32.50000000000000000, 22.40000000546237757, -10.55989012756945300 ) ) ;
#31202=PLANE ( 'NONE',  #4580 ) ;
#31203=FACE_OUTER_BOUND ( 'NONE', #32624, .T. ) ;
#31206=CARTESIAN_POINT ( 'NONE',  ( -24.50000000000000000, 10.64999999453762669, -7.960532557706207157 ) ) ;
#31207=CARTESIAN_POINT ( 'NONE',  ( -20.75514604977248823, 28.82500000273117280, -28.56700777964554305 ) ) ;
#31212=ORIENTED_EDGE ( 'NONE', *, *, #27607, .F. ) ;
#31217=CARTESIAN_POINT ( 'NONE',  ( -20.75514604977248823, 37.07500000273120122, -28.56700777964554305 ) ) ;
#31218=CARTESIAN_POINT ( 'NONE',  ( -32.50000000000000000, 38.60000000546239818, 10.55989012756946366 ) ) ;
#31220=CARTESIAN_POINT ( 'NONE',  ( -10.04305231718579172, 47.60000000000000142, -30.90933677959248982 ) ) ;
#31221=CARTESIAN_POINT ( 'NONE',  ( 33.58253175000000823, 22.02500000273117919, 10.91162601494192863 ) ) ;
#31223=CARTESIAN_POINT ( 'NONE',  ( 10.37757302488624056, 50.77500000273118985, -31.93888565452638417 ) ) ;
#31224=( BOUNDED_CURVE ( )  B_SPLINE_CURVE ( 2, ( #19236, #29674, #6179, #16661, #27118, #24542, #11496, #21975, #19403, #6352, #16831, #9947, #10295 ),
 .UNSPECIFIED., .F., .T. ) 
 B_SPLINE_CURVE_WITH_KNOTS ( ( 3, 2, 2, 2, 2, 2, 3 ),
 ( 0.4038461538461538547, 0.4051282051282051322, 0.4076923076923076872, 0.4102564102564102422, 0.4128205128205127972, 0.4153846153846154077, 0.4166666666666666852 ),
 .UNSPECIFIED. ) 
 CURVE ( )  GEOMETRIC_REPRESENTATION_ITEM ( )  RATIONAL_B_SPLINE_CURVE ( ( 0.9755282581475768211, 0.9755282581475768211, 1.000000000000000000, 0.9510565162951535312, 1.000000000000000000, 0.9510565162951535312, 1.000000000000000000, 0.9510565162951535312, 1.000000000000000000, 0.9510565162951535312, 1.000000000000000000, 0.9755282581475768211, 0.9755282581475768211 ) ) 
 REPRESENTATION_ITEM ( '' )  );
#31226=CARTESIAN_POINT ( 'NONE',  ( 26.29305231718578995, 25.19999999999999929, -19.10302069950538240 ) ) ;
#31228=EDGE_CURVE ( 'NONE', #11992, #16018, #2196, .T. ) ;
#31229=CARTESIAN_POINT ( 'NONE',  ( -27.16883889988623935, 71.32500000273117280, 19.73931689729374739 ) ) ;
#31231=CARTESIAN_POINT ( 'NONE',  ( 5.779280353836490358E-15, 38.50000000000000000, 32.49999999999999289 ) ) ;
#31232=CARTESIAN_POINT ( 'NONE',  ( -10.37757302488623701, 57.77500000273119696, 31.93888565452638417 ) ) ;
#31233=CYLINDRICAL_SURFACE ( 'NONE', #30337, 32.50000000000000000 ) ;
#31234=CARTESIAN_POINT ( 'NONE',  ( 27.16883889988623935, 12.32500000273117990, -19.73931689729374384 ) ) ;
#31236=FACE_OUTER_BOUND ( 'NONE', #29203, .T. ) ;
#31238=CARTESIAN_POINT ( 'NONE',  ( -1.778240108872766143E-15, 46.00000000546238255, -32.49999999999999289 ) ) ;
#31239=CARTESIAN_POINT ( 'NONE',  ( -1.778240108872766143E-15, 3.500000000000004441, -32.49999999999999289 ) ) ;
#31244=CARTESIAN_POINT ( 'NONE',  ( 32.50000000000000000, 61.00000000000000000, -3.980102097228898626E-15 ) ) ;
#31246=CARTESIAN_POINT ( 'NONE',  ( -32.50000000000000000, 54.10000000000000853, 10.55989012756946366 ) ) ;
#31247=CARTESIAN_POINT ( 'NONE',  ( -26.29305231718579350, 66.30000000546237970, -19.10302069950537884 ) ) ;
#31251=ORIENTED_EDGE ( 'NONE', *, *, #5665, .F. ) ;
#31252=CARTESIAN_POINT ( 'NONE',  ( 27.16883889988624290, 74.17500000273119554, 19.73931689729373673 ) ) ;
#31256=CARTESIAN_POINT ( 'NONE',  ( -27.16883889988624290, 51.17500000273117422, -19.73931689729374028 ) ) ;
#31257=CARTESIAN_POINT ( 'NONE',  ( -10.04305231718578462, 56.90000000546238823, 30.90933677959249337 ) ) ;
#31259=CARTESIAN_POINT ( 'NONE',  ( -20.75514604977248112, 43.42500000273117422, 28.56700777964554661 ) ) ;
#31261=CARTESIAN_POINT ( 'NONE',  ( 33.58253175000000113, 70.37500000273119838, -4.112674001490185761E-15 ) ) ;
#31262=CARTESIAN_POINT ( 'NONE',  ( -10.04305231718579172, 2.100000005462371533, -30.90933677959248982 ) ) ;
#31265=CARTESIAN_POINT ( 'NONE',  ( 10.04305231718579705, 44.60000000000000142, 30.90933677959248982 ) ) ;
#31268=CARTESIAN_POINT ( 'NONE',  ( 20.75514604977249178, 10.07500000273118168, 28.56700777964553950 ) ) ;
#31269=DIRECTION ( 'NONE',  ( -0.000000000000000000, 1.000000000000000000, -0.000000000000000000 ) ) ;
#31271=CARTESIAN_POINT ( 'NONE',  ( -8.960552108402742093E-16, 76.87500000273115575, -14.63369212191046387 ) ) ;
#31272=CARTESIAN_POINT ( 'NONE',  ( -27.16883889988624290, 77.17500000273119554, -19.73931689729374028 ) ) ;
#31273=DIRECTION ( 'NONE',  ( 0.000000000000000000, 0.000000000000000000, -1.000000000000000000 ) ) ;
#31274=EDGE_CURVE ( 'NONE', #26581, #17842, #28794, .T. ) ;
#31276=ORIENTED_EDGE ( 'NONE', *, *, #3708, .F. ) ;
#31287=CARTESIAN_POINT ( 'NONE',  ( -33.58253175000000113, 47.02500000273117564, -10.91162601494193041 ) ) ;
#31289=CARTESIAN_POINT ( 'NONE',  ( -5.147494310547423346, 2.948745723915526806, 32.50000000000000000 ) ) ;
#31295=CARTESIAN_POINT ( 'NONE',  ( 33.58253175000000113, 78.37500000273116996, -4.112674001490185761E-15 ) ) ;
#31296=ORIENTED_EDGE ( 'NONE', *, *, #4186, .T. ) ;
#31299=ORIENTED_EDGE ( 'NONE', *, *, #32725, .F. ) ;
#31300=CARTESIAN_POINT ( 'NONE',  ( -32.50000000000000000, 14.40000000546236869, -10.55989012756945300 ) ) ;
#31301=CARTESIAN_POINT ( 'NONE',  ( 10.37757302488624767, 63.72500000273117848, 31.93888565452638417 ) ) ;
#31303=CARTESIAN_POINT ( 'NONE',  ( 24.50000000000000000, 16.00000000000001421, 0.000000000000000000 ) ) ;
#31304=CARTESIAN_POINT ( 'NONE',  ( -23.41746825000000243, 2.224999997268808816, 7.608796670333725309 ) ) ;
#31305=VECTOR ( 'NONE', #14760, 1000.000000000000000 ) ;
#31306=CARTESIAN_POINT ( 'NONE',  ( 33.58253175000000113, 2.225000002731166937, -10.91162601494193751 ) ) ;
#31308=CARTESIAN_POINT ( 'NONE',  ( -2.375766604868044141, 79.80125428700920054, -14.99999999999999822 ) ) ;
#31313=ADVANCED_FACE ( 'NONE', ( #4776 ), #12671, .F. ) ;
#31314=EDGE_CURVE ( 'NONE', #21689, #30261, #28456, .T. ) ;
#31316=CARTESIAN_POINT ( 'NONE',  ( 9.270509831248425314, 70.95000000546234276, 12.75976212528059683 ) ) ;
#31318=CARTESIAN_POINT ( 'NONE',  ( 10.37757302488624767, 33.72500000273117848, 31.93888565452638417 ) ) ;
#31322=CARTESIAN_POINT ( 'NONE',  ( 20.75514604977249178, 16.07500000273119767, 28.56700777964553950 ) ) ;
#31323=CARTESIAN_POINT ( 'NONE',  ( -15.00000000000000000, 79.90000000000000568, -4.873795443493594171 ) ) ;
#31325=CARTESIAN_POINT ( 'NONE',  ( -27.16883889988624290, 78.92500000273116711, -19.73931689729374028 ) ) ;
#31326=CARTESIAN_POINT ( 'NONE',  ( -20.08610463437157989, 65.69999999999998863, -27.64615127144129758 ) ) ;
#31327=( BOUNDED_CURVE ( )  B_SPLINE_CURVE ( 2, ( #31238, #7731, #5330, #10481, #18555, #18220, #23528, #8069, #28664, #5159, #15644, #28999, #5499 ),
 .UNSPECIFIED., .F., .T. ) 
 B_SPLINE_CURVE_WITH_KNOTS ( ( 3, 2, 2, 2, 2, 2, 3 ),
 ( 0.4166666666666666852, 0.4179487179487179627, 0.4205128205128205177, 0.4230769230769230727, 0.4256410256410256276, 0.4282051282051281826, 0.4294871794871795156 ),
 .UNSPECIFIED. ) 
 CURVE ( )  GEOMETRIC_REPRESENTATION_ITEM ( )  RATIONAL_B_SPLINE_CURVE ( ( 0.9755282581475768211, 0.9755282581475768211, 1.000000000000000000, 0.9510565162951535312, 1.000000000000000000, 0.9510565162951535312, 1.000000000000000000, 0.9510565162951535312, 1.000000000000000000, 0.9510565162951535312, 1.000000000000000000, 0.9755282581475762660, 0.9755282581475768211 ) ) 
 REPRESENTATION_ITEM ( '' )  );
#31329=DIRECTION ( 'NONE',  ( -0.000000000000000000, -1.000000000000000000, -0.000000000000000000 ) ) ;
#31330=CARTESIAN_POINT ( 'NONE',  ( 6.486482029760648627E-15, 61.62500000273118417, 35.31076352940722529 ) ) ;
#31333=CARTESIAN_POINT ( 'NONE',  ( 10.37757302488624767, 7.725000002731185589, 31.93888565452638417 ) ) ;
#31334=CARTESIAN_POINT ( 'NONE',  ( 23.41746825000000243, 0.7249999972688272454, -7.608796670333727974 ) ) ;
#31336=VERTEX_POINT ( 'NONE', #18178 ) ;
#31338=VERTEX_POINT ( 'NONE', #23832 ) ;
#31340=CARTESIAN_POINT ( 'NONE',  ( -32.50000000000000000, 79.90000000000000568, -10.55989012756945300 ) ) ;
#31342=CARTESIAN_POINT ( 'NONE',  ( -26.29305231718579350, 71.79999999999999716, -19.10302069950537884 ) ) ;
#31344=CARTESIAN_POINT ( 'NONE',  ( 23.41746825000000243, 16.72499999726881725, -7.608796670333727974 ) ) ;
#31345=CARTESIAN_POINT ( 'NONE',  ( -27.16883889988623935, 15.57500000273118168, 19.73931689729374739 ) ) ;
#31346=CARTESIAN_POINT ( 'NONE',  ( 10.04305231718578817, 59.40000000000000568, -30.90933677959249337 ) ) ;
#31348=CARTESIAN_POINT ( 'NONE',  ( 20.08610463437157279, 73.80000000546236549, -27.64615127144129758 ) ) ;
#31350=CARTESIAN_POINT ( 'NONE',  ( 2.688165632520823219E-15, 77.87500000273118417, 14.63369212191046387 ) ) ;
#31355=CARTESIAN_POINT ( 'NONE',  ( 24.50000000000000000, 16.09999999999998721, -7.960532557706203605 ) ) ;
#31356=CARTESIAN_POINT ( 'NONE',  ( -26.29305231718578995, 6.199999999999983302, 19.10302069950538595 ) ) ;
#31357=DIRECTION ( 'NONE',  ( -0.000000000000000000, -1.000000000000000000, -0.000000000000000000 ) ) ;
#31359=CARTESIAN_POINT ( 'NONE',  ( -33.58253175000000113, 53.12500000273118417, 0.000000000000000000 ) ) ;
#31361=CARTESIAN_POINT ( 'NONE',  ( -2.162160676586882350E-15, 42.87500000273119127, -35.31076352940722529 ) ) ;
#31362=CARTESIAN_POINT ( 'NONE',  ( -14.45873412499999944, 81.68750000136559208, 0.000000000000000000 ) ) ;
#31363=CARTESIAN_POINT ( 'NONE',  ( 0.000000000000000000, 0.000000000000000000, 24.50000000000000000 ) ) ;
#31364=CARTESIAN_POINT ( 'NONE',  ( -3.880418787951118276, 8.551254281546841085, -24.50000000000000355 ) ) ;
#31368=CARTESIAN_POINT ( 'NONE',  ( 10.04305231718579705, 6.599999999999994316, 30.90933677959248982 ) ) ;
#31369=DIRECTION ( 'NONE',  ( 0.000000000000000000, 0.000000000000000000, -1.000000000000000000 ) ) ;
#31370=CARTESIAN_POINT ( 'NONE',  ( 0.000000000000000000, 80.00000000000001421, 0.000000000000000000 ) ) ;
#31373=CARTESIAN_POINT ( 'NONE',  ( 24.50000000000000000, 17.64999999453763735, 7.960532557706212486 ) ) ;
#31374=CARTESIAN_POINT ( 'NONE',  ( -20.75514604977248823, 26.82500000273117280, -28.56700777964554305 ) ) ;
#31376=EDGE_CURVE ( 'NONE', #9001, #24073, #14190, .T. ) ;
#31383=ORIENTED_EDGE ( 'NONE', *, *, #18882, .F. ) ;
#31386=CARTESIAN_POINT ( 'NONE',  ( 14.47279130897151767, 0.9249999972688209837, -19.92008829642072598 ) ) ;
#31387=CARTESIAN_POINT ( 'NONE',  ( -27.16883889988623935, 35.57500000273120122, 19.73931689729374739 ) ) ;
#31388=CARTESIAN_POINT ( 'NONE',  ( -10.04305231718579172, 38.10000000546237686, -30.90933677959248982 ) ) ;
#31391=CARTESIAN_POINT ( 'NONE',  ( -20.75514604977248112, 23.42500000273119909, 28.56700777964554661 ) ) ;
#31393=CARTESIAN_POINT ( 'NONE',  ( -27.16883889988623935, 51.57500000273118701, 19.73931689729374739 ) ) ;
#31396=CARTESIAN_POINT ( 'NONE',  ( -10.04305231718578462, 26.40000000000000568, 30.90933677959249337 ) ) ;
#31398=CARTESIAN_POINT ( 'NONE',  ( 27.16883889988624290, 69.92500000273119554, 19.73931689729373673 ) ) ;
#31400=CARTESIAN_POINT ( 'NONE',  ( 5.779280353836490358E-15, 1.000000005462375885, 32.49999999999999289 ) ) ;
#31401=CARTESIAN_POINT ( 'NONE',  ( -33.58253175000000113, 57.37500000273118417, 0.000000000000000000 ) ) ;
#31402=CARTESIAN_POINT ( 'NONE',  ( 5.147494310547434893, 7.051254287009218302, 32.49999999999999289 ) ) ;
#31403=CARTESIAN_POINT ( 'NONE',  ( -2.162160676586881955E-15, 12.62500000273118772, -35.31076352940723240 ) ) ;
#31406=CARTESIAN_POINT ( 'NONE',  ( -33.58253175000000113, 3.475000002731185589, 10.91162601494193929 ) ) ;
#31410=CIRCLE ( 'NONE', #1802, 24.50000000000000000 ) ;
#31417=CARTESIAN_POINT ( 'NONE',  ( 14.47279130897151767, 1.424999997268804997, -19.92008829642072598 ) ) ;
#31418=CARTESIAN_POINT ( 'NONE',  ( 32.50000000000000000, 69.50000000546238255, -3.980102097228898626E-15 ) ) ;
#31426=DIRECTION ( 'NONE',  ( -0.000000000000000000, -1.000000000000000000, -0.000000000000000000 ) ) ;
#31427=CARTESIAN_POINT ( 'NONE',  ( 33.58253175000000823, 56.27500000273116854, 10.91162601494192863 ) ) ;
#31428=CARTESIAN_POINT ( 'NONE',  ( -20.08610463437156923, 56.80000000546240102, 27.64615127144130113 ) ) ;
#31430=CARTESIAN_POINT ( 'NONE',  ( 10.37757302488624056, 42.52500000273118275, -31.93888565452638417 ) ) ;
#31431=CARTESIAN_POINT ( 'NONE',  ( 15.00000000000000355, 73.15000000546240244, 4.873795443493592394 ) ) ;
#31432=CARTESIAN_POINT ( 'NONE',  ( -27.16883889988623935, 69.57500000273120122, 19.73931689729374739 ) ) ;
#31434=AXIS2_PLACEMENT_3D ( 'NONE', #13183, #7526, #15775 ) ;
#31437=CARTESIAN_POINT ( 'NONE',  ( -32.50000000000000000, 47.99999999999998579, 0.000000000000000000 ) ) ;
#31439=CARTESIAN_POINT ( 'NONE',  ( -20.75514604977248112, 9.675000002731193760, 28.56700777964554661 ) ) ;
#31442=CARTESIAN_POINT ( 'NONE',  ( -13.91746824999999532, 73.27500000273118985, -4.522059556121115875 ) ) ;
#31443=DIRECTION ( 'NONE',  ( 0.000000000000000000, 0.000000000000000000, -1.000000000000000000 ) ) ;
#31444=DIRECTION ( 'NONE',  ( -0.000000000000000000, -1.000000000000000000, -0.000000000000000000 ) ) ;
#31446=ORIENTED_EDGE ( 'NONE', *, *, #18618, .F. ) ;
#31447=CARTESIAN_POINT ( 'NONE',  ( -1.778240108872766143E-15, 20.00000000546237544, -32.49999999999999289 ) ) ;
#31457=AXIS2_PLACEMENT_3D ( 'NONE', #20912, #26393, #26053 ) ;
#31458=CARTESIAN_POINT ( 'NONE',  ( -27.16883889988623935, 41.32500000273120122, 19.73931689729374739 ) ) ;
#31463=ADVANCED_FACE ( 'NONE', ( #5077 ), #4730, .T. ) ;
#31467=CARTESIAN_POINT ( 'NONE',  ( -33.58253175000000113, 75.37500000273116996, 0.000000000000000000 ) ) ;
#31468=EDGE_CURVE ( 'NONE', #9001, #32300, #28920, .T. ) ;
#31469=VERTEX_POINT ( 'NONE', #15900 ) ;
#31474=CARTESIAN_POINT ( 'NONE',  ( 27.16883889988623935, 58.32500000273119412, -19.73931689729374384 ) ) ;
#31477=CARTESIAN_POINT ( 'NONE',  ( -7.236395654485763274, 6.524999997268826846, 22.27133577429736633 ) ) ;
#31479=CARTESIAN_POINT ( 'NONE',  ( -10.37757302488624411, 4.725000002731183812, -31.93888565452638417 ) ) ;
#31482=CARTESIAN_POINT ( 'NONE',  ( -4.635254915624211769, 79.85000000546239107, -14.26584774442730286 ) ) ;
#31484=CARTESIAN_POINT ( 'NONE',  ( 32.50000000000000711, 8.900000000000011013, 10.55989012756945122 ) ) ;
#31488=CARTESIAN_POINT ( 'NONE',  ( -13.91746824999999532, 80.77500000273118985, -4.522059556121115875 ) ) ;
#31490=CARTESIAN_POINT ( 'NONE',  ( 27.16883889988623935, 26.32500000273119056, -19.73931689729374384 ) ) ;
#31493=CARTESIAN_POINT ( 'NONE',  ( -2.162160676586882350E-15, 14.87500000273120371, -35.31076352940722529 ) ) ;
#31496=CARTESIAN_POINT ( 'NONE',  ( 27.16883889988623935, 78.32500000273118701, -19.73931689729374384 ) ) ;
#31497=CARTESIAN_POINT ( 'NONE',  ( -32.50000000000000000, 66.00000000000000000, 0.000000000000000000 ) ) ;
#31499=CARTESIAN_POINT ( 'NONE',  ( 1.507698388325705758E-15, 15.12499999726880873, -24.62258325217400312 ) ) ;
#31500=CARTESIAN_POINT ( 'NONE',  ( 33.58253175000000113, 56.12500000273118417, -4.112674001490185761E-15 ) ) ;
#31502=EDGE_CURVE ( 'NONE', #22348, #15702, #23450, .T. ) ;
#31503=VERTEX_POINT ( 'NONE', #23098 ) ;
#31505=CARTESIAN_POINT ( 'NONE',  ( -2.162160676586882350E-15, 4.625000002731207260, -35.31076352940722529 ) ) ;
#31506=CARTESIAN_POINT ( 'NONE',  ( -4.523095164977116484E-15, 18.62499999726881583, 24.62258325217400312 ) ) ;
#31510=ORIENTED_EDGE ( 'NONE', *, *, #9342, .T. ) ;
#31512=CARTESIAN_POINT ( 'NONE',  ( 32.50000000000000000, 5.000000000000004441, -3.980102097228898626E-15 ) ) ;
#31516=CARTESIAN_POINT ( 'NONE',  ( -23.41746825000000598, 15.72499999726882081, 7.608796670333726198 ) ) ;
#31517=CARTESIAN_POINT ( 'NONE',  ( -27.16883889988624290, 15.17500000273119909, -19.73931689729374028 ) ) ;
#31518=CARTESIAN_POINT ( 'NONE',  ( 32.50000000000000000, 61.00000000000000000, -3.980102097228898626E-15 ) ) ;
#31519=CARTESIAN_POINT ( 'NONE',  ( -13.91746824999999532, 78.97500000273117848, 4.522059556121122093 ) ) ;
#31520=CARTESIAN_POINT ( 'NONE',  ( 2.489536152421872915E-14, 74.00000000546238255, -32.49999999999999289 ) ) ;
#31522=CARTESIAN_POINT ( 'NONE',  ( -13.91746824999999887, 77.37500000273116996, 0.000000000000000000 ) ) ;
#31525=CARTESIAN_POINT ( 'NONE',  ( -19.82091636218621389, 13.19999999999998863, 14.40073868116558842 ) ) ;
#31526=CARTESIAN_POINT ( 'NONE',  ( -10.04305231718579172, 3.599999999999992095, -30.90933677959248982 ) ) ;
#31527=CARTESIAN_POINT ( 'NONE',  ( 26.29305231718579350, 17.30000000546239036, 19.10302069950537529 ) ) ;
#31530=CARTESIAN_POINT ( 'NONE',  ( -20.75514604977248823, 50.82500000273116569, -28.56700777964554305 ) ) ;
#31533=CARTESIAN_POINT ( 'NONE',  ( 33.58253175000000823, 32.27500000273117564, 10.91162601494192685 ) ) ;
#31534=CARTESIAN_POINT ( 'NONE',  ( 32.50000000000000711, 24.89999999999999858, 10.55989012756945122 ) ) ;
#31536=CARTESIAN_POINT ( 'NONE',  ( -1.778240108872766143E-15, 16.00000000546237899, -32.49999999999999289 ) ) ;
#31542=CARTESIAN_POINT ( 'NONE',  ( -20.75514604977248112, 23.42500000273119554, 28.56700777964554661 ) ) ;
#31546=ORIENTED_EDGE ( 'NONE', *, *, #32629, .F. ) ;
#31550=CARTESIAN_POINT ( 'NONE',  ( 14.47279130897151589, 2.324999997268805796, 19.92008829642072953 ) ) ;
#31551=CARTESIAN_POINT ( 'NONE',  ( -20.75514604977248823, 33.07500000273117990, -28.56700777964554305 ) ) ;
#31552=CARTESIAN_POINT ( 'NONE',  ( -10.04305231718578462, 36.90000000546236691, 30.90933677959249337 ) ) ;
#31554=CARTESIAN_POINT ( 'NONE',  ( -32.50000000000000000, 78.00000000000001421, 0.000000000000000000 ) ) ;
#31555=CARTESIAN_POINT ( 'NONE',  ( -20.08610463437157989, 47.70000000000000284, -27.64615127144129758 ) ) ;
#31556=CARTESIAN_POINT ( 'NONE',  ( 20.08610463437157279, 77.30000000000001137, -27.64615127144129758 ) ) ;
#31557=CARTESIAN_POINT ( 'NONE',  ( 33.58253175000000823, 48.27500000273119696, 10.91162601494192863 ) ) ;
#31559=CARTESIAN_POINT ( 'NONE',  ( 20.08610463437157279, 21.29999999999999716, -27.64615127144129758 ) ) ;
#31561=CARTESIAN_POINT ( 'NONE',  ( -33.58253175000000113, 67.02500000273117564, -10.91162601494193218 ) ) ;
#31564=CARTESIAN_POINT ( 'NONE',  ( -10.37757302488623701, 51.77500000273118985, 31.93888565452638417 ) ) ;
#31565=CARTESIAN_POINT ( 'NONE',  ( -32.50000000000000000, 40.60000000546238397, 10.55989012756946366 ) ) ;
#31566=CARTESIAN_POINT ( 'NONE',  ( 6.486482029760649416E-15, 11.62500000273118950, 35.31076352940723240 ) ) ;
#31568=CARTESIAN_POINT ( 'NONE',  ( 3.778760231354629433E-15, 2.249999994537632553, -24.50000000000000355 ) ) ;
#31577=CARTESIAN_POINT ( 'NONE',  ( 5.147494310547434893, 60.55125428154682510, 32.49999999999999289 ) ) ;
#31579=CARTESIAN_POINT ( 'NONE',  ( -7.236395654485757944, 5.724999997268803931, -22.27133577429736988 ) ) ;
#31580=CARTESIAN_POINT ( 'NONE',  ( -10.04305231718578462, 68.90000000546237402, 30.90933677959249337 ) ) ;
#31589=CARTESIAN_POINT ( 'NONE',  ( 26.29305231718578995, 75.19999999999998863, -19.10302069950538240 ) ) ;
#31590=CARTESIAN_POINT ( 'NONE',  ( -10.37757302488624411, 54.97500000273119980, -31.93888565452638417 ) ) ;
#31591=CARTESIAN_POINT ( 'NONE',  ( -26.29305231718579350, 56.30000000546237260, -19.10302069950537884 ) ) ;
#31592=CARTESIAN_POINT ( 'NONE',  ( -27.16883889988623935, 39.32500000273120122, 19.73931689729374739 ) ) ;
#31593=CYLINDRICAL_SURFACE ( 'NONE', #4451, 32.50000000000000000 ) ;
#31594=CARTESIAN_POINT ( 'NONE',  ( 20.75514604977248467, 68.67500000273119554, -28.56700777964554305 ) ) ;
#31595=CARTESIAN_POINT ( 'NONE',  ( -10.04305231718578462, 0.9000000054623646939, 30.90933677959249337 ) ) ;
#31598=EDGE_CURVE ( 'NONE', #4188, #7938, #21218, .T. ) ;
#31600=CARTESIAN_POINT ( 'NONE',  ( -10.04305231718579172, 43.60000000000000142, -30.90933677959248982 ) ) ;
#31602=CARTESIAN_POINT ( 'NONE',  ( 27.16883889988623935, 12.57500000273120655, -19.73931689729374384 ) ) ;
#31603=DIRECTION ( 'NONE',  ( -0.000000000000000000, -1.000000000000000000, -0.000000000000000000 ) ) ;
#31605=CARTESIAN_POINT ( 'NONE',  ( 0.000000000000000000, 82.00000000000001421, 0.000000000000000000 ) ) ;
#31606=CARTESIAN_POINT ( 'NONE',  ( -33.58253175000000113, 77.37500000273116996, 0.000000000000000000 ) ) ;
#31607=CARTESIAN_POINT ( 'NONE',  ( 3.980102097228898626E-15, 82.00000000000001421, 32.50000000000000000 ) ) ;
#31609=ORIENTED_EDGE ( 'NONE', *, *, #5047, .T. ) ;
#31611=CYLINDRICAL_SURFACE ( 'NONE', #24454, 32.50000000000000000 ) ;
#31620=CARTESIAN_POINT ( 'NONE',  ( 5.779280353836490358E-15, 57.00000000546238965, 32.49999999999999289 ) ) ;
#31621=CARTESIAN_POINT ( 'NONE',  ( 20.75514604977249178, 37.82500000273117280, 28.56700777964553950 ) ) ;
#31624=CARTESIAN_POINT ( 'NONE',  ( 0.000000000000000000, 80.00000000000001421, 0.000000000000000000 ) ) ;
#31629=CARTESIAN_POINT ( 'NONE',  ( 33.58253175000000113, 70.37500000273119838, -4.112674001490185761E-15 ) ) ;
#31634=CARTESIAN_POINT ( 'NONE',  ( 5.779280353836490358E-15, 49.00000000546238255, 32.49999999999999289 ) ) ;
#31635=CARTESIAN_POINT ( 'NONE',  ( 10.37757302488624056, 60.52500000273119696, -31.93888565452638417 ) ) ;
#31638=CARTESIAN_POINT ( 'NONE',  ( -20.08610463437156923, 66.80000000546236549, 27.64615127144130113 ) ) ;
#31639=CARTESIAN_POINT ( 'NONE',  ( -14.47279130897152299, 6.424999997268821872, 19.92008829642072243 ) ) ;
#31640=CARTESIAN_POINT ( 'NONE',  ( -33.58253175000000113, 5.125000002731194826, 0.000000000000000000 ) ) ;
#31641=CARTESIAN_POINT ( 'NONE',  ( 33.58253175000000113, 28.37500000273118772, -4.112674001490185761E-15 ) ) ;
#31642=CARTESIAN_POINT ( 'NONE',  ( -4.223320258572821363E-15, 78.75000000546238255, 15.00000000000000355 ) ) ;
#31644=CARTESIAN_POINT ( 'NONE',  ( -27.16883889988624290, 79.17500000273119554, -19.73931689729374028 ) ) ;
#31646=CARTESIAN_POINT ( 'NONE',  ( -32.50000000000000000, 4.000000000000003553, 0.000000000000000000 ) ) ;
#31650=CARTESIAN_POINT ( 'NONE',  ( -15.00000000000000000, 70.35000000546237686, 4.873795443493597723 ) ) ;
#31652=EDGE_CURVE ( 'NONE', #10540, #22185, #27112, .T. ) ;
#31653=CARTESIAN_POINT ( 'NONE',  ( -2.162160676586881955E-15, 22.62500000273119127, -35.31076352940723240 ) ) ;
#31656=CARTESIAN_POINT ( 'NONE',  ( 20.75514604977249178, 18.07500000273119056, 28.56700777964553950 ) ) ;
#31659=CARTESIAN_POINT ( 'NONE',  ( -2.162160676586882350E-15, 68.62500000273119838, -35.31076352940722529 ) ) ;
#31662=CARTESIAN_POINT ( 'NONE',  ( -15.00000000000000000, 72.35000000546236265, 4.873795443493597723 ) ) ;
#31663=CARTESIAN_POINT ( 'NONE',  ( -20.75514604977248823, 60.82500000273120122, -28.56700777964554305 ) ) ;
#31666=VERTEX_POINT ( 'NONE', #16402 ) ;
#31669=CARTESIAN_POINT ( 'NONE',  ( 1.507698388325705758E-15, 1.124999997268814722, -24.62258325217400312 ) ) ;
#31673=LINE ( 'NONE', #24621, #15434 ) ;
#31678=CARTESIAN_POINT ( 'NONE',  ( 5.779280353836490358E-15, 27.00000000546237544, 32.49999999999999289 ) ) ;
#31680=CARTESIAN_POINT ( 'NONE',  ( 24.50000000000000355, 2.099999999999991651, -7.960532557706203605 ) ) ;
#31681=CARTESIAN_POINT ( 'NONE',  ( 33.58253175000000823, 10.27500000273117564, 10.91162601494192863 ) ) ;
#31682=CARTESIAN_POINT ( 'NONE',  ( -10.04305231718578462, 60.40000000000000568, 30.90933677959249337 ) ) ;
#31683=CARTESIAN_POINT ( 'NONE',  ( -8.601468415847518756, 76.57500000273117280, -11.83890561707634603 ) ) ;
#31686=CARTESIAN_POINT ( 'NONE',  ( -13.91746824999999532, 75.27500000273121827, -4.522059556121115875 ) ) ;
#31689=DIRECTION ( 'NONE',  ( 0.000000000000000000, 0.000000000000000000, -1.000000000000000000 ) ) ;
#31690=CARTESIAN_POINT ( 'NONE',  ( 7.313012447739250820E-14, 15.50000000000000178, 24.50000000000000000 ) ) ;
#31691=CARTESIAN_POINT ( 'NONE',  ( -10.04305231718578462, 4.400000000000014566, 30.90933677959249337 ) ) ;
#31695=CARTESIAN_POINT ( 'NONE',  ( -33.58253175000000113, 41.02500000273118985, -10.91162601494193218 ) ) ;
#31698=CARTESIAN_POINT ( 'NONE',  ( -10.37757302488623701, 33.77500000273120406, 31.93888565452638417 ) ) ;
#31702=CARTESIAN_POINT ( 'NONE',  ( 1.093617666956751375E-13, 61.50000000000000000, -32.50000000000000711 ) ) ;
#31703=CARTESIAN_POINT ( 'NONE',  ( -5.147494310547423346, 22.94874572391553968, 32.50000000000000000 ) ) ;
#31706=CARTESIAN_POINT ( 'NONE',  ( -23.41746824999999887, 7.624999997268816720, -2.867812753649727150E-15 ) ) ;
#31707=CARTESIAN_POINT ( 'NONE',  ( -20.08610463437157989, 39.69999999999999574, -27.64615127144129758 ) ) ;
#31711=CARTESIAN_POINT ( 'NONE',  ( 6.486482029760648627E-15, 19.62500000273116996, 35.31076352940722529 ) ) ;
#31715=ORIENTED_EDGE ( 'NONE', *, *, #13138, .F. ) ;
#31719=ORIENTED_EDGE ( 'NONE', *, *, #25524, .F. ) ;
#31720=FACE_OUTER_BOUND ( 'NONE', #15571, .T. ) ;
#31721=CARTESIAN_POINT ( 'NONE',  ( -20.75514604977248112, 27.67500000273118133, 28.56700777964554661 ) ) ;
#31722=CARTESIAN_POINT ( 'NONE',  ( 32.50000000000000000, 39.60000000546234844, -10.55989012756945833 ) ) ;
#31724=CARTESIAN_POINT ( 'NONE',  ( -20.08610463437157989, 79.70000000000000284, -27.64615127144129758 ) ) ;
#31726=CARTESIAN_POINT ( 'NONE',  ( 6.486482029760649416E-15, 39.87500000273119127, 35.31076352940723240 ) ) ;
#31728=CARTESIAN_POINT ( 'NONE',  ( 6.277390505771533514E-15, 22.49999999999998934, 34.17252228774368916 ) ) ;
#31730=CARTESIAN_POINT ( 'NONE',  ( -33.58253175000000113, 65.12500000273119838, 0.000000000000000000 ) ) ;
#31733=CARTESIAN_POINT ( 'NONE',  ( -33.58253175000000113, 53.27500000273118275, -10.91162601494193041 ) ) ;
#31736=CARTESIAN_POINT ( 'NONE',  ( 33.58253175000000113, 12.12500000273120193, -4.112674001490185761E-15 ) ) ;
#31741=CARTESIAN_POINT ( 'NONE',  ( -26.29305231718579350, 18.30000000546239036, -19.10302069950537884 ) ) ;
#31748=CARTESIAN_POINT ( 'NONE',  ( 26.29305231718578995, 69.70000000546238539, -19.10302069950538240 ) ) ;
#31750=ADVANCED_FACE ( 'NONE', ( #24291 ), #425, .T. ) ;
#31757=CARTESIAN_POINT ( 'NONE',  ( 5.147494310547440222, 75.44874571845313938, -32.50000000000000000 ) ) ;
#31758=CARTESIAN_POINT ( 'NONE',  ( 10.37757302488624056, 48.77500000273118985, -31.93888565452638417 ) ) ;
#31759=CARTESIAN_POINT ( 'NONE',  ( -10.04305231718578462, 54.90000000546238823, 30.90933677959249337 ) ) ;
#31761=CARTESIAN_POINT ( 'NONE',  ( -33.58253175000000113, 37.22500000273119980, 10.91162601494193929 ) ) ;
#31762=CARTESIAN_POINT ( 'NONE',  ( -33.58253175000000113, 63.47500000273117138, 10.91162601494193929 ) ) ;
#31763=CARTESIAN_POINT ( 'NONE',  ( -2.092463501923844636E-15, 2.000000005462382102, -34.17252228774368916 ) ) ;
#31766=CARTESIAN_POINT ( 'NONE',  ( 26.29305231718579350, 42.80000000000000426, 19.10302069950537529 ) ) ;
#31768=CARTESIAN_POINT ( 'NONE',  ( -20.75514604977248823, 11.07500000273117813, -28.56700777964554305 ) ) ;
#31769=DIRECTION ( 'NONE',  ( -0.000000000000000000, -1.000000000000000000, -0.000000000000000000 ) ) ;
#31772=CARTESIAN_POINT ( 'NONE',  ( 10.37757302488624767, 69.97500000273119269, 31.93888565452638417 ) ) ;
#31773=FACE_OUTER_BOUND ( 'NONE', #9200, .T. ) ;
#31776=LINE ( 'NONE', #18760, #11300 ) ;
#31786=CARTESIAN_POINT ( 'NONE',  ( -32.50000000000000000, 56.50000000546237544, 0.000000000000000000 ) ) ;
#31787=CARTESIAN_POINT ( 'NONE',  ( 27.16883889988623935, 36.32500000273120122, -19.73931689729374384 ) ) ;
#31791=CARTESIAN_POINT ( 'NONE',  ( -32.50000000000000000, 2.600000005462363095, 10.55989012756946366 ) ) ;
#31794=CARTESIAN_POINT ( 'NONE',  ( -1.778240108872766143E-15, 50.00000000546237544, -32.49999999999999289 ) ) ;
#31796=CARTESIAN_POINT ( 'NONE',  ( 33.58253175000000823, 66.27500000273118985, 10.91162601494192863 ) ) ;
#31799=EDGE_CURVE ( 'NONE', #21272, #33751, #23422, .T. ) ;
#31801=ORIENTED_EDGE ( 'NONE', *, *, #8939, .T. ) ;
#31802=CYLINDRICAL_SURFACE ( 'NONE', #5644, 32.50000000000000000 ) ;
#31803=CARTESIAN_POINT ( 'NONE',  ( 33.58253175000000823, 52.02500000273118985, 10.91162601494192863 ) ) ;
#31805=CARTESIAN_POINT ( 'NONE',  ( 32.50000000000000711, 19.40000000546238468, 10.55989012756945122 ) ) ;
#31807=CARTESIAN_POINT ( 'NONE',  ( -7.236395654485763274, 10.52499999726880198, 22.27133577429736633 ) ) ;
#31808=CARTESIAN_POINT ( 'NONE',  ( -33.58253175000000113, 29.27500000273118630, -10.91162601494193218 ) ) ;
#31809=CARTESIAN_POINT ( 'NONE',  ( -2.375766604868045029, 77.80125428700922896, -14.99999999999999822 ) ) ;
#31811=CARTESIAN_POINT ( 'NONE',  ( 20.75514604977248467, 78.67500000273116711, -28.56700777964554305 ) ) ;
#31813=CARTESIAN_POINT ( 'NONE',  ( -26.29305231718579350, 3.799999999999998046, -19.10302069950537884 ) ) ;
#31817=CARTESIAN_POINT ( 'NONE',  ( -13.91746824999999532, 72.77500000273117564, -4.522059556121115875 ) ) ;
#31820=CARTESIAN_POINT ( 'NONE',  ( 33.58253175000000113, 26.22500000273119625, -10.91162601494193751 ) ) ;
#31823=CARTESIAN_POINT ( 'NONE',  ( 33.58253175000000823, 16.27500000273118985, 10.91162601494192685 ) ) ;
#31825=CARTESIAN_POINT ( 'NONE',  ( -20.75514604977248823, 70.82500000273117280, -28.56700777964554305 ) ) ;
#31826=CARTESIAN_POINT ( 'NONE',  ( 32.50000000000000711, 3.400000005462366914, 10.55989012756945122 ) ) ;
#31828=CARTESIAN_POINT ( 'NONE',  ( -4.223320258572821363E-15, 78.75000000546238255, 15.00000000000000355 ) ) ;
#31829=CARTESIAN_POINT ( 'NONE',  ( -27.16883889988624290, 60.92500000273118133, -19.73931689729374028 ) ) ;
#31831=EDGE_LOOP ( 'NONE', ( #17028, #24907, #22544, #32993 ) ) ;
#31833=CARTESIAN_POINT ( 'NONE',  ( 10.37757302488624767, 1.725000002731180704, 31.93888565452638417 ) ) ;
#31834=CARTESIAN_POINT ( 'NONE',  ( 23.41746825000000243, 8.524999997268812635, 7.608796670333735079 ) ) ;
#31839=AXIS2_PLACEMENT_3D ( 'NONE', #10444, #23661, #26060 ) ;
#31840=ORIENTED_EDGE ( 'NONE', *, *, #26437, .F. ) ;
#31844=CARTESIAN_POINT ( 'NONE',  ( -5.147494310547450880, 72.44874571845318201, 32.49999999999999289 ) ) ;
#31846=CARTESIAN_POINT ( 'NONE',  ( 19.82091636218621034, 1.799999999999996048, 14.40073868116559730 ) ) ;
#31847=CARTESIAN_POINT ( 'NONE',  ( -10.37757302488623701, 7.775000002731180970, 31.93888565452638417 ) ) ;
#31848=CARTESIAN_POINT ( 'NONE',  ( -10.04305231718579172, 61.59999999999998721, -30.90933677959248982 ) ) ;
#31849=CARTESIAN_POINT ( 'NONE',  ( 4.300734207923757602, 76.27500000273118985, -13.23629886949340673 ) ) ;
#31850=LINE ( 'NONE', #8343, #12677 ) ;
#31852=VECTOR ( 'NONE', #2911, 1000.000000000000000 ) ;
#31853=CARTESIAN_POINT ( 'NONE',  ( 8.601468415847516980, 74.67500000273118133, -11.83890561707634781 ) ) ;
#31855=DIRECTION ( 'NONE',  ( 0.000000000000000000, 0.000000000000000000, -1.000000000000000000 ) ) ;
#31856=CARTESIAN_POINT ( 'NONE',  ( 10.04305231718579705, 49.10000000546238397, 30.90933677959248982 ) ) ;
#31858=CARTESIAN_POINT ( 'NONE',  ( -33.58253175000000113, 41.22500000273118559, 10.91162601494193929 ) ) ;
#31861=CARTESIAN_POINT ( 'NONE',  ( -33.58253175000000113, 35.27500000273119696, -10.91162601494193041 ) ) ;
#31868=CARTESIAN_POINT ( 'NONE',  ( 1.507698388325705758E-15, 7.124999997268799845, -24.62258325217400312 ) ) ;
#31871=CARTESIAN_POINT ( 'NONE',  ( 27.16883889988623935, 20.32500000273118701, -19.73931689729374384 ) ) ;
#31874=EDGE_LOOP ( 'NONE', ( #4488, #4021, #3028, #31276 ) ) ;
#31877=ORIENTED_EDGE ( 'NONE', *, *, #5392, .T. ) ;
#31881=EDGE_CURVE ( 'NONE', #28042, #8956, #30405, .T. ) ;
#31882=VERTEX_POINT ( 'NONE', #15302 ) ;
#31883=DIRECTION ( 'NONE',  ( -0.000000000000000000, 1.000000000000000000, -0.000000000000000000 ) ) ;
#31884=CARTESIAN_POINT ( 'NONE',  ( -33.58253175000000113, 25.37500000273118417, 0.000000000000000000 ) ) ;
#31885=CARTESIAN_POINT ( 'NONE',  ( -32.50000000000000000, 32.40000000546238113, -10.55989012756945478 ) ) ;
#31886=CARTESIAN_POINT ( 'NONE',  ( 26.29305231718578995, 79.19999999999998863, -19.10302069950538240 ) ) ;
#31887=CARTESIAN_POINT ( 'NONE',  ( 32.50000000000000711, 33.40000000546238113, 10.55989012756945122 ) ) ;
#31888=CARTESIAN_POINT ( 'NONE',  ( 10.04305231718579705, 37.10000000546237686, 30.90933677959248982 ) ) ;
#31889=CARTESIAN_POINT ( 'NONE',  ( -33.58253175000000113, 43.47500000273117138, 10.91162601494193929 ) ) ;
#31891=CARTESIAN_POINT ( 'NONE',  ( -32.50000000000000000, 21.90000000000000924, -10.55989012756945478 ) ) ;
#31893=CARTESIAN_POINT ( 'NONE',  ( -20.75514604977248823, 60.82500000273121543, -28.56700777964554305 ) ) ;
#31894=CARTESIAN_POINT ( 'NONE',  ( -5.147494310547418017, 77.55125428154686062, -32.50000000000000000 ) ) ;
#31896=CARTESIAN_POINT ( 'NONE',  ( 10.37757302488624056, 54.77500000273119696, -31.93888565452638417 ) ) ;
#31899=CARTESIAN_POINT ( 'NONE',  ( 27.16883889988624290, 3.925000002731188431, 19.73931689729373673 ) ) ;
#31911=DIRECTION ( 'NONE',  ( 0.000000000000000000, 0.000000000000000000, -1.000000000000000000 ) ) ;
#31914=( BOUNDED_CURVE ( )  B_SPLINE_CURVE ( 2, ( #31642, #26675, #5230, #18289, #21030, #26169, #2662, #23937, #13640, #32144, #29065, #31809, #23597 ),
 .UNSPECIFIED., .F., .T. ) 
 B_SPLINE_CURVE_WITH_KNOTS ( ( 3, 2, 2, 2, 2, 2, 3 ),
 ( 0.1500000000000000222, 0.1600000000000000033, 0.1799999999999999933, 0.2000000000000000111, 0.2200000000000000011, 0.2399999999999999911, 0.2500000000000000000 ),
 .UNSPECIFIED. ) 
 CURVE ( )  GEOMETRIC_REPRESENTATION_ITEM ( )  RATIONAL_B_SPLINE_CURVE ( ( 0.9755282581475768211, 0.9755282581475768211, 1.000000000000000000, 0.9510565162951535312, 1.000000000000000000, 0.9510565162951535312, 1.000000000000000000, 0.9510565162951535312, 1.000000000000000000, 0.9510565162951535312, 1.000000000000000000, 0.9755282581475768211, 0.9755282581475768211 ) ) 
 REPRESENTATION_ITEM ( '' )  );
#31916=CARTESIAN_POINT ( 'NONE',  ( 20.08610463437158344, 71.20000000546237118, 27.64615127144129403 ) ) ;
#31925=CARTESIAN_POINT ( 'NONE',  ( 27.16883889988624290, 46.17500000273119554, 19.73931689729373673 ) ) ;
#31926=CARTESIAN_POINT ( 'NONE',  ( -32.50000000000000000, 58.50000000546237544, 0.000000000000000000 ) ) ;
#31928=CARTESIAN_POINT ( 'NONE',  ( -20.75514604977248112, 35.42500000273119554, 28.56700777964554661 ) ) ;
#31930=CARTESIAN_POINT ( 'NONE',  ( 10.37757302488624056, 64.77500000273117564, -31.93888565452638417 ) ) ;
#31934=CARTESIAN_POINT ( 'NONE',  ( 20.08610463437157279, 41.30000000000001137, -27.64615127144129758 ) ) ;
#31936=CARTESIAN_POINT ( 'NONE',  ( -33.58253175000000113, 5.375000002731167292, 0.000000000000000000 ) ) ;
#31937=CYLINDRICAL_SURFACE ( 'NONE', #21698, 32.50000000000000000 ) ;
#31938=FACE_OUTER_BOUND ( 'NONE', #304, .T. ) ;
#31939=CARTESIAN_POINT ( 'NONE',  ( 10.37757302488624767, 73.97500000273119269, 31.93888565452638417 ) ) ;
#31940=FACE_OUTER_BOUND ( 'NONE', #14473, .T. ) ;
#31944=DIRECTION ( 'NONE',  ( 0.000000000000000000, 0.000000000000000000, -1.000000000000000000 ) ) ;
#31955=CARTESIAN_POINT ( 'NONE',  ( -20.75514604977248112, 37.42500000273118843, 28.56700777964554661 ) ) ;
#31958=FACE_OUTER_BOUND ( 'NONE', #5428, .T. ) ;
#31961=CARTESIAN_POINT ( 'NONE',  ( 20.08610463437158344, 50.69999999999999574, 27.64615127144129403 ) ) ;
#31964=CARTESIAN_POINT ( 'NONE',  ( -33.58253175000000113, 69.47500000273116427, 10.91162601494193929 ) ) ;
#31965=ORIENTED_EDGE ( 'NONE', *, *, #19915, .F. ) ;
#31967=AXIS2_PLACEMENT_3D ( 'NONE', #26096, #20627, #29164 ) ;
#31969=ORIENTED_EDGE ( 'NONE', *, *, #27745, .T. ) ;
#31970=CARTESIAN_POINT ( 'NONE',  ( 27.16883889988624290, 55.92500000273120975, 19.73931689729373673 ) ) ;
#31972=CARTESIAN_POINT ( 'NONE',  ( -26.29305231718579350, 16.30000000546239036, -19.10302069950537884 ) ) ;
#31974=CARTESIAN_POINT ( 'NONE',  ( 1.507698388325705758E-15, 9.624999997268808727, -24.62258325217400312 ) ) ;
#31975=CARTESIAN_POINT ( 'NONE',  ( -33.58253175000000113, 21.47500000273119980, 10.91162601494193929 ) ) ;
#31978=CARTESIAN_POINT ( 'NONE',  ( 11.25946833292375793, 79.67500000273119554, 8.180482586598731842 ) ) ;
#31979=CARTESIAN_POINT ( 'NONE',  ( -10.04305231718578462, 4.400000000000014566, 30.90933677959249337 ) ) ;
#31981=EDGE_LOOP ( 'NONE', ( #30237, #4660, #33620, #20592 ) ) ;
#31983=CARTESIAN_POINT ( 'NONE',  ( 4.300734207923761154, 77.47500000273119269, 13.23629886949340495 ) ) ;
#31985=CARTESIAN_POINT ( 'NONE',  ( 33.58253175000000823, 24.02500000273117564, 10.91162601494192863 ) ) ;
#31988=VECTOR ( 'NONE', #12324, 1000.000000000000000 ) ;
#31989=CARTESIAN_POINT ( 'NONE',  ( 33.58253175000000113, 18.47500000273117848, -10.91162601494193574 ) ) ;
#31991=CARTESIAN_POINT ( 'NONE',  ( 33.58253175000000823, 70.02500000273120406, 10.91162601494192685 ) ) ;
#31992=DIRECTION ( 'NONE',  ( -0.000000000000000000, -1.000000000000000000, -0.000000000000000000 ) ) ;
#31993=CARTESIAN_POINT ( 'NONE',  ( -4.300734207923759378, 80.97500000273119269, -13.23629886949340495 ) ) ;
#31995=CARTESIAN_POINT ( 'NONE',  ( -2.375766604868045029, 71.80125428700922896, -14.99999999999999822 ) ) ;
#31996=CARTESIAN_POINT ( 'NONE',  ( -2.162160676586882350E-15, 58.62500000273118417, -35.31076352940722529 ) ) ;
#31998=ORIENTED_EDGE ( 'NONE', *, *, #31274, .T. ) ;
#32001=CARTESIAN_POINT ( 'NONE',  ( 1.507698388325705758E-15, 5.124999997268805174, -24.62258325217400312 ) ) ;
#32003=ORIENTED_EDGE ( 'NONE', *, *, #27471, .T. ) ;
#32006=EDGE_CURVE ( 'NONE', #31666, #14496, #24506, .T. ) ;
#32007=VERTEX_POINT ( 'NONE', #20632 ) ;
#32010=CARTESIAN_POINT ( 'NONE',  ( -24.50000000000000711, 3.099999999999989431, 7.960532557706201828 ) ) ;
#32011=CARTESIAN_POINT ( 'NONE',  ( 10.37757302488624056, 72.52500000273120406, -31.93888565452638417 ) ) ;
#32013=CARTESIAN_POINT ( 'NONE',  ( 19.82091636218621034, 7.800000000000001599, 14.40073868116559730 ) ) ;
#32014=CARTESIAN_POINT ( 'NONE',  ( 10.37757302488624767, 9.975000002731187365, 31.93888565452638417 ) ) ;
#32015=CARTESIAN_POINT ( 'NONE',  ( 6.486482029760649416E-15, 17.62500000273117351, 35.31076352940723240 ) ) ;
#32016=( BOUNDED_CURVE ( )  B_SPLINE_CURVE ( 2, ( #29462, #8536, #21764, #16941, #803, #16279, #26737, #19350, #27061, #24329, #8700, #24490, #13699 ),
 .UNSPECIFIED., .F., .T. ) 
 B_SPLINE_CURVE_WITH_KNOTS ( ( 3, 2, 2, 2, 2, 2, 3 ),
 ( 0.3269230769230769273, 0.3282051282051282048, 0.3307692307692307598, 0.3333333333333333148, 0.3358974358974358698, 0.3384615384615384803, 0.3397435897435897578 ),
 .UNSPECIFIED. ) 
 CURVE ( )  GEOMETRIC_REPRESENTATION_ITEM ( )  RATIONAL_B_SPLINE_CURVE ( ( 0.9755282581475768211, 0.9755282581475768211, 1.000000000000000000, 0.9510565162951535312, 1.000000000000000000, 0.9510565162951535312, 1.000000000000000000, 0.9510565162951535312, 1.000000000000000000, 0.9510565162951535312, 1.000000000000000000, 0.9755282581475768211, 0.9755282581475768211 ) ) 
 REPRESENTATION_ITEM ( '' )  );
#32017=CARTESIAN_POINT ( 'NONE',  ( -4.300734207923759378, 80.47500000273119269, -13.23629886949340495 ) ) ;
#32020=CARTESIAN_POINT ( 'NONE',  ( -4.300734207923755825, 77.77500000273118985, 13.23629886949340673 ) ) ;
#32024=DIRECTION ( 'NONE',  ( -0.000000000000000000, 1.000000000000000000, -0.000000000000000000 ) ) ;
#32026=CARTESIAN_POINT ( 'NONE',  ( -20.75514604977248112, 43.42500000273117422, 28.56700777964554661 ) ) ;
#32029=CARTESIAN_POINT ( 'NONE',  ( -10.37757302488623701, 37.77500000273118275, 31.93888565452638417 ) ) ;
#32036=CARTESIAN_POINT ( 'NONE',  ( -4.523095164977117273E-15, 2.124999997268811835, 24.62258325217400312 ) ) ;
#32037=DIRECTION ( 'NONE',  ( -0.000000000000000000, -1.000000000000000000, -0.000000000000000000 ) ) ;
#32039=CARTESIAN_POINT ( 'NONE',  ( -20.08610463437156923, 60.29999999999997584, 27.64615127144130113 ) ) ;
#32040=CARTESIAN_POINT ( 'NONE',  ( -10.37757302488623701, 21.52500000273119340, 31.93888565452638417 ) ) ;
#32048=EDGE_LOOP ( 'NONE', ( #18145, #28892, #4153, #4962 ) ) ;
#32049=CARTESIAN_POINT ( 'NONE',  ( -14.47279130897152122, 1.924999997268818541, 19.92008829642072243 ) ) ;
#32050=CARTESIAN_POINT ( 'NONE',  ( -2.162160676586881955E-15, 26.87500000273116996, -35.31076352940723240 ) ) ;
#32051=( BOUNDED_CURVE ( )  B_SPLINE_CURVE ( 2, ( #18441, #31289, #15862, #21349, #2644, #31791, #7783, #18269, #28717, #13107, #23581, #46, #2807 ),
 .UNSPECIFIED., .F., .F. ) 
 B_SPLINE_CURVE_WITH_KNOTS ( ( 3, 2, 2, 2, 2, 2, 3 ),
 ( 0.9679487179487179516, 0.9692307692307692291, 0.9717948717948717841, 0.9743589743589743390, 0.9769230769230768940, 0.9794871794871794490, 0.9807692307692307265 ),
 .UNSPECIFIED. ) 
 CURVE ( )  GEOMETRIC_REPRESENTATION_ITEM ( )  RATIONAL_B_SPLINE_CURVE ( ( 0.9755282581475768211, 0.9755282581475768211, 1.000000000000000000, 0.9510565162951535312, 1.000000000000000000, 0.9510565162951535312, 1.000000000000000000, 0.9510565162951535312, 1.000000000000000000, 0.9510565162951535312, 1.000000000000000000, 0.9755282581475768211, 0.9755282581475768211 ) ) 
 REPRESENTATION_ITEM ( '' )  );
#32052=MECHANICAL_DESIGN_GEOMETRIC_PRESENTATION_REPRESENTATION('',(#12317),#16710);
#32053=CARTESIAN_POINT ( 'NONE',  ( 6.277390505771533514E-15, 29.00000000546237189, 34.17252228774368916 ) ) ;
#32054=CARTESIAN_POINT ( 'NONE',  ( 32.50000000000000000, 77.00000000000001421, -3.980102097228898626E-15 ) ) ;
#32055=CARTESIAN_POINT ( 'NONE',  ( -20.08610463437156923, 54.80000000546236549, 27.64615127144130113 ) ) ;
#32057=CARTESIAN_POINT ( 'NONE',  ( -10.37757302488623701, 41.77500000273118275, 31.93888565452638417 ) ) ;
#32060=CARTESIAN_POINT ( 'NONE',  ( 20.08610463437158344, 22.70000000000000995, 27.64615127144129403 ) ) ;
#32062=CARTESIAN_POINT ( 'NONE',  ( 33.58253175000000113, 66.12500000273119838, -4.112674001490185761E-15 ) ) ;
#32063=CARTESIAN_POINT ( 'NONE',  ( 10.37757302488624056, 52.77500000273118985, -31.93888565452638417 ) ) ;
#32066=CARTESIAN_POINT ( 'NONE',  ( -10.37757302488624411, 2.725000002731181592, -31.93888565452638417 ) ) ;
#32068=EDGE_CURVE ( 'NONE', #28845, #2126, #15069, .T. ) ;
#32071=FACE_OUTER_BOUND ( 'NONE', #4872, .T. ) ;
#32075=EDGE_CURVE ( 'NONE', #21334, #9459, #18621, .T. ) ;
#32076=CARTESIAN_POINT ( 'NONE',  ( 5.147494310547434893, 1.051254287009222965, 32.49999999999999289 ) ) ;
#32087=ORIENTED_EDGE ( 'NONE', *, *, #23790, .T. ) ;
#32091=CARTESIAN_POINT ( 'NONE',  ( -32.50000000000000000, 36.09999999999999432, 10.55989012756946366 ) ) ;
#32092=CARTESIAN_POINT ( 'NONE',  ( 33.58253175000000113, 48.47500000273118559, -10.91162601494193751 ) ) ;
#32093=CARTESIAN_POINT ( 'NONE',  ( 20.08610463437158344, 53.20000000546237118, 27.64615127144129403 ) ) ;
#32096=CARTESIAN_POINT ( 'NONE',  ( -10.37757302488624411, 38.72500000273118559, -31.93888565452638417 ) ) ;
#32097=CARTESIAN_POINT ( 'NONE',  ( 27.16883889988623935, 62.57500000273119412, -19.73931689729374384 ) ) ;
#32098=CARTESIAN_POINT ( 'NONE',  ( -10.04305231718578462, 42.39999999999999147, 30.90933677959249337 ) ) ;
#32100=CARTESIAN_POINT ( 'NONE',  ( 10.37757302488624767, 1.975000002731180926, 31.93888565452638417 ) ) ;
#32101=DIRECTION ( 'NONE',  ( 0.000000000000000000, 0.000000000000000000, -1.000000000000000000 ) ) ;
#32102=CARTESIAN_POINT ( 'NONE',  ( -13.91746824999999887, 75.37500000273116996, 0.000000000000000000 ) ) ;
#32103=CARTESIAN_POINT ( 'NONE',  ( -10.37757302488624411, 70.97500000273119269, -31.93888565452638417 ) ) ;
#32116=( BOUNDED_CURVE ( )  B_SPLINE_CURVE ( 2, ( #19808, #16903, #16738, #14662, #6431, #32995, #30431 ),
 .UNSPECIFIED., .F., .T. ) 
 B_SPLINE_CURVE_WITH_KNOTS ( ( 3, 2, 2, 3 ),
 ( 0.9935897435897436125, 0.9948717948717948900, 0.9974358974358974450, 1.000000000000000000 ),
 .UNSPECIFIED. ) 
 CURVE ( )  GEOMETRIC_REPRESENTATION_ITEM ( )  RATIONAL_B_SPLINE_CURVE ( ( 0.9755282581475768211, 0.9755282581475768211, 1.000000000000000000, 0.9510565162951535312, 1.000000000000000000, 0.9510565162951535312, 1.000000000000000000 ) ) 
 REPRESENTATION_ITEM ( '' )  );
#32118=EDGE_CURVE ( 'NONE', #13788, #4296, #167, .T. ) ;
#32125=CARTESIAN_POINT ( 'NONE',  ( 10.04305231718578817, 59.40000000000000568, -30.90933677959249337 ) ) ;
#32126=ORIENTED_EDGE ( 'NONE', *, *, #6421, .T. ) ;
#32128=CARTESIAN_POINT ( 'NONE',  ( -10.04305231718578462, 50.90000000546238113, 30.90933677959249337 ) ) ;
#32131=CARTESIAN_POINT ( 'NONE',  ( -33.58253175000000113, 67.37500000273119838, 0.000000000000000000 ) ) ;
#32132=ORIENTED_EDGE ( 'NONE', *, *, #13841, .T. ) ;
#32136=DIRECTION ( 'NONE',  ( 0.000000000000000000, 0.000000000000000000, -1.000000000000000000 ) ) ;
#32137=CARTESIAN_POINT ( 'NONE',  ( -10.37757302488623701, 55.52500000273119696, 31.93888565452638417 ) ) ;
#32139=CARTESIAN_POINT ( 'NONE',  ( -2.092463501923844636E-15, 16.00000000546237544, -34.17252228774368916 ) ) ;
#32140=DIRECTION ( 'NONE',  ( -0.000000000000000000, 1.000000000000000000, -0.000000000000000000 ) ) ;
#32141=AXIS2_PLACEMENT_3D ( 'NONE', #14346, #19499, #13849 ) ;
#32142=CARTESIAN_POINT ( 'NONE',  ( 14.47279130897151944, 11.42499999726880944, -19.92008829642072598 ) ) ;
#32143=CARTESIAN_POINT ( 'NONE',  ( -27.16883889988623935, 21.57500000273118701, 19.73931689729374739 ) ) ;
#32144=CARTESIAN_POINT ( 'NONE',  ( -9.270509831248423538, 77.95000000546237118, -12.75976212528059861 ) ) ;
#32150=EDGE_LOOP ( 'NONE', ( #21599, #5724, #10353, #16568 ) ) ;
#32152=CARTESIAN_POINT ( 'NONE',  ( -4.300734207923759378, 74.47500000273119269, -13.23629886949340495 ) ) ;
#32154=CARTESIAN_POINT ( 'NONE',  ( 27.16883889988624290, 27.92500000273118133, 19.73931689729373673 ) ) ;
#32158=CARTESIAN_POINT ( 'NONE',  ( -27.16883889988624290, 7.175000002731191096, -19.73931689729374028 ) ) ;
#32160=CARTESIAN_POINT ( 'NONE',  ( -33.58253175000000113, 71.02500000273117564, -10.91162601494193041 ) ) ;
#32163=CARTESIAN_POINT ( 'NONE',  ( 13.91746825000000065, 76.27500000273118985, 4.522059556121115875 ) ) ;
#32166=CARTESIAN_POINT ( 'NONE',  ( 10.37757302488624767, 59.72500000273117848, 31.93888565452638417 ) ) ;
#32168=VECTOR ( 'NONE', #21545, 1000.000000000000000 ) ;
#32169=ORIENTED_EDGE ( 'NONE', *, *, #3894, .T. ) ;
#32172=CARTESIAN_POINT ( 'NONE',  ( 23.41746824999999887, 4.624999997268814056, 0.000000000000000000 ) ) ;
#32174=VERTEX_POINT ( 'NONE', #8238 ) ;
#32176=CARTESIAN_POINT ( 'NONE',  ( -20.08610463437157989, 42.20000000546238539, -27.64615127144129758 ) ) ;
#32177=ORIENTED_EDGE ( 'NONE', *, *, #1170, .T. ) ;
#32181=CARTESIAN_POINT ( 'NONE',  ( 20.75514604977248467, 76.42500000273118133, -28.56700777964554305 ) ) ;
#32183=CARTESIAN_POINT ( 'NONE',  ( -24.50000000000000355, 6.899999999999985256, -7.960532557706207157 ) ) ;
#32184=CARTESIAN_POINT ( 'NONE',  ( 33.58253175000000113, 8.475000002731173154, -10.91162601494193751 ) ) ;
#32185=CARTESIAN_POINT ( 'NONE',  ( 33.58253175000000113, 18.22500000273118559, -10.91162601494193751 ) ) ;
#32187=CARTESIAN_POINT ( 'NONE',  ( -8.960552108402744065E-16, 78.37500000273116996, -14.63369212191046209 ) ) ;
#32188=DIRECTION ( 'NONE',  ( -0.000000000000000000, 1.000000000000000000, -0.000000000000000000 ) ) ;
#32190=CARTESIAN_POINT ( 'NONE',  ( 4.300734207923761154, 71.97500000273119269, 13.23629886949340495 ) ) ;
#32193=CARTESIAN_POINT ( 'NONE',  ( 32.50000000000000711, 70.90000000000000568, 10.55989012756945122 ) ) ;
#32195=CARTESIAN_POINT ( 'NONE',  ( 27.16883889988623935, 42.32500000273120833, -19.73931689729374384 ) ) ;
#32198=CARTESIAN_POINT ( 'NONE',  ( -33.58253175000000113, 33.27500000273120406, -10.91162601494193041 ) ) ;
#32205=CARTESIAN_POINT ( 'NONE',  ( -23.41746824999999887, 5.624999997268814944, -2.867812753649727150E-15 ) ) ;
#32207=DIRECTION ( 'NONE',  ( -0.000000000000000000, -1.000000000000000000, -0.000000000000000000 ) ) ;
#32209=DIRECTION ( 'NONE',  ( 0.000000000000000000, 0.000000000000000000, -1.000000000000000000 ) ) ;
#32210=CARTESIAN_POINT ( 'NONE',  ( 10.37757302488624056, 18.52500000273118985, -31.93888565452638417 ) ) ;
#32211=CARTESIAN_POINT ( 'NONE',  ( 18.94512977948575738, 8.924999997268812990, 13.76444248337723408 ) ) ;
#32214=ORIENTED_EDGE ( 'NONE', *, *, #22423, .F. ) ;
#32218=ORIENTED_EDGE ( 'NONE', *, *, #2527, .F. ) ;
#32223=CARTESIAN_POINT ( 'NONE',  ( -14.47279130897152122, 7.924999997268803220, 19.92008829642072243 ) ) ;
#32224=CARTESIAN_POINT ( 'NONE',  ( 10.37757302488624767, 27.97500000273117493, 31.93888565452638417 ) ) ;
#32225=CARTESIAN_POINT ( 'NONE',  ( 32.50000000000000000, 29.50000000546237899, -3.980102097228898626E-15 ) ) ;
#32226=CARTESIAN_POINT ( 'NONE',  ( 26.29305231718578995, 69.19999999999998863, -19.10302069950538240 ) ) ;
#32228=CARTESIAN_POINT ( 'NONE',  ( -19.82091636218621389, 11.19999999999998863, 14.40073868116558842 ) ) ;
#32230=CARTESIAN_POINT ( 'NONE',  ( -10.37757302488623701, 45.77500000273118985, 31.93888565452638417 ) ) ;
#32231=CARTESIAN_POINT ( 'NONE',  ( 18.94512977948576093, 13.32499999726882756, -13.76444248337722875 ) ) ;
#32232=CARTESIAN_POINT ( 'NONE',  ( 6.277390505771533514E-15, 18.49999999999999645, 34.17252228774368916 ) ) ;
#32234=CARTESIAN_POINT ( 'NONE',  ( 33.58253175000000823, 62.02500000273116143, 10.91162601494192863 ) ) ;
#32235=CARTESIAN_POINT ( 'NONE',  ( 20.75514604977249178, 52.07500000273119412, 28.56700777964553950 ) ) ;
#32237=LINE ( 'NONE', #10981, #16141 ) ;
#32238=CARTESIAN_POINT ( 'NONE',  ( 27.16883889988623935, 6.325000002731173687, -19.73931689729374384 ) ) ;
#32241=MANIFOLD_SOLID_BREP ( 'Thread3', #17772 ) ;
#32242=CARTESIAN_POINT ( 'NONE',  ( -5.147494310547430452, 19.55125428154684641, -32.49999999999999289 ) ) ;
#32244=LINE ( 'NONE', #3592, #1223 ) ;
#32245=CARTESIAN_POINT ( 'NONE',  ( 3.735172737399427541E-15, 70.00000000000000000, 30.50000000000000000 ) ) ;
#32247=CARTESIAN_POINT ( 'NONE',  ( -10.04305231718578462, 30.90000000546239178, 30.90933677959249337 ) ) ;
#32254=LINE ( 'NONE', #4107, #908 ) ;
#32255=ORIENTED_EDGE ( 'NONE', *, *, #14071, .F. ) ;
#32259=CARTESIAN_POINT ( 'NONE',  ( 32.50000000000000711, 56.90000000000000568, 10.55989012756945122 ) ) ;
#32260=CARTESIAN_POINT ( 'NONE',  ( -33.58253175000000113, 47.47500000273119269, 10.91162601494193929 ) ) ;
#32261=CARTESIAN_POINT ( 'NONE',  ( 32.50000000000000000, 49.50000000546239676, -3.980102097228898626E-15 ) ) ;
#32262=ADVANCED_FACE ( 'NONE', ( #6005 ), #1342, .F. ) ;
#32264=CARTESIAN_POINT ( 'NONE',  ( 10.37757302488624767, 33.72500000273117848, 31.93888565452638417 ) ) ;
#32266=CARTESIAN_POINT ( 'NONE',  ( -10.37757302488624411, 62.97500000273120691, -31.93888565452638417 ) ) ;
#32267=CARTESIAN_POINT ( 'NONE',  ( 32.50000000000000000, 39.00000000000000711, -3.980102097228898626E-15 ) ) ;
#32269=CARTESIAN_POINT ( 'NONE',  ( -33.58253175000000113, 3.275000002731191628, -10.91162601494193218 ) ) ;
#32270=DIRECTION ( 'NONE',  ( -0.000000000000000000, 1.000000000000000000, -0.000000000000000000 ) ) ;
#32272=CARTESIAN_POINT ( 'NONE',  ( -27.16883889988623935, 73.57500000273120122, 19.73931689729374739 ) ) ;
#32273=CARTESIAN_POINT ( 'NONE',  ( -24.50000000000000711, 18.84999999453762953, 7.960532557706201828 ) ) ;
#32276=CARTESIAN_POINT ( 'NONE',  ( -7.570916362186210335, 6.349999994537613546, -23.30088464923126779 ) ) ;
#32289=CARTESIAN_POINT ( 'NONE',  ( 32.50000000000000711, 13.40000000546237047, 10.55989012756945122 ) ) ;
#32292=CARTESIAN_POINT ( 'NONE',  ( 0.000000000000000000, 80.00000000000001421, 0.000000000000000000 ) ) ;
#32294=CARTESIAN_POINT ( 'NONE',  ( 27.16883889988623935, 66.57500000273120122, -19.73931689729374384 ) ) ;
#32295=ORIENTED_EDGE ( 'NONE', *, *, #7702, .T. ) ;
#32298=EDGE_CURVE ( 'NONE', #21770, #16286, #18894, .T. ) ;
#32300=VERTEX_POINT ( 'NONE', #8578 ) ;
#32302=CARTESIAN_POINT ( 'NONE',  ( 27.16883889988623935, 54.32500000273118701, -19.73931689729374384 ) ) ;
#32305=CARTESIAN_POINT ( 'NONE',  ( 26.29305231718578995, 9.700000005462394270, -19.10302069950538240 ) ) ;
#32307=CARTESIAN_POINT ( 'NONE',  ( -14.47279130897152299, 12.42499999726880588, 19.92008829642072243 ) ) ;
#32308=CARTESIAN_POINT ( 'NONE',  ( -27.16883889988624290, 25.17500000273117777, -19.73931689729374028 ) ) ;
#32309=CARTESIAN_POINT ( 'NONE',  ( 4.635254915624209993, 77.39999999999999147, -14.26584774442730463 ) ) ;
#32313=CARTESIAN_POINT ( 'NONE',  ( -32.50000000000000000, 34.10000000000000142, 10.55989012756946366 ) ) ;
#32314=( BOUNDED_CURVE ( )  B_SPLINE_CURVE ( 2, ( #10716, #59, #21195, #31638, #8136, #29061, #16047, #27163, #14132, #901, #6057, #13799, #21858 ),
 .UNSPECIFIED., .F., .T. ) 
 B_SPLINE_CURVE_WITH_KNOTS ( ( 3, 2, 2, 2, 2, 2, 3 ),
 ( 0.1474358974358974395, 0.1487179487179487170, 0.1512820512820512719, 0.1538461538461538547, 0.1564102564102564097, 0.1589743589743589647, 0.1602564102564102699 ),
 .UNSPECIFIED. ) 
 CURVE ( )  GEOMETRIC_REPRESENTATION_ITEM ( )  RATIONAL_B_SPLINE_CURVE ( ( 0.9755282581475768211, 0.9755282581475768211, 1.000000000000000000, 0.9510565162951535312, 1.000000000000000000, 0.9510565162951535312, 1.000000000000000000, 0.9510565162951535312, 1.000000000000000000, 0.9510565162951535312, 1.000000000000000000, 0.9755282581475764880, 0.9755282581475768211 ) ) 
 REPRESENTATION_ITEM ( '' )  );
#32318=CARTESIAN_POINT ( 'NONE',  ( 13.91746825000000065, 77.77500000273117564, 4.522059556121114987 ) ) ;
#32320=CARTESIAN_POINT ( 'NONE',  ( 6.486482029760649416E-15, 17.62500000273117351, 35.31076352940723240 ) ) ;
#32324=CARTESIAN_POINT ( 'NONE',  ( -10.37757302488624411, 6.975000002731185589, -31.93888565452638417 ) ) ;
#32327=CARTESIAN_POINT ( 'NONE',  ( 5.147494310547434893, 59.05125428700924317, 32.49999999999999289 ) ) ;
#32328=CARTESIAN_POINT ( 'NONE',  ( -13.91746824999999532, 75.27500000273123248, -4.522059556121115875 ) ) ;
#32331=CARTESIAN_POINT ( 'NONE',  ( 33.58253175000000823, 50.02500000273119696, 10.91162601494192685 ) ) ;
#32333=VERTEX_POINT ( 'NONE', #12157 ) ;
#32336=CARTESIAN_POINT ( 'NONE',  ( 23.41746824999999887, 6.624999997268815832, 0.000000000000000000 ) ) ;
#32338=ORIENTED_EDGE ( 'NONE', *, *, #9999, .T. ) ;
#32343=CARTESIAN_POINT ( 'NONE',  ( -27.16883889988624290, 61.17500000273118133, -19.73931689729374028 ) ) ;
#32345=CARTESIAN_POINT ( 'NONE',  ( 33.58253175000000113, 74.12500000273119838, -4.112674001490185761E-15 ) ) ;
#32347=CARTESIAN_POINT ( 'NONE',  ( 19.82091636218621034, 5.799999999999999822, 14.40073868116559730 ) ) ;
#32350=EDGE_CURVE ( 'NONE', #19359, #3811, #30511, .T. ) ;
#32351=CARTESIAN_POINT ( 'NONE',  ( -10.37757302488624411, 14.72500000273119269, -31.93888565452638417 ) ) ;
#32352=CARTESIAN_POINT ( 'NONE',  ( 13.91746824999999532, 73.97500000273120691, -4.522059556121118540 ) ) ;
#32354=CARTESIAN_POINT ( 'NONE',  ( 15.00000000000000355, 78.89999999999999147, 4.873795443493592394 ) ) ;
#32357=CARTESIAN_POINT ( 'NONE',  ( 32.50000000000000000, 71.00000000000001421, -3.980102097228898626E-15 ) ) ;
#32359=CARTESIAN_POINT ( 'NONE',  ( 27.16883889988623935, 44.32500000273117990, -19.73931689729374384 ) ) ;
#32362=CARTESIAN_POINT ( 'NONE',  ( 20.75514604977249178, 26.07500000273119767, 28.56700777964553950 ) ) ;
#32363=LINE ( 'NONE', #8857, #23488 ) ;
#32366=CARTESIAN_POINT ( 'NONE',  ( -2.165007332552593587E-13, 45.00000000546237544, 32.50000000000000000 ) ) ;
#32369=CARTESIAN_POINT ( 'NONE',  ( -18.94512977948575738, 3.424999997268807217, -13.76444248337723231 ) ) ;
#32372=CARTESIAN_POINT ( 'NONE',  ( -1.089172066684569321E-14, 76.75000000546238255, 15.00000000000000000 ) ) ;
#32373=CARTESIAN_POINT ( 'NONE',  ( 10.37757302488624056, 16.52500000273118985, -31.93888565452638417 ) ) ;
#32374=CARTESIAN_POINT ( 'NONE',  ( 1.507698388325705758E-15, 3.624999997268822938, -24.62258325217400312 ) ) ;
#32376=ORIENTED_EDGE ( 'NONE', *, *, #32118, .T. ) ;
#32379=ORIENTED_EDGE ( 'NONE', *, *, #6700, .T. ) ;
#32382=AXIS2_PLACEMENT_3D ( 'NONE', #11466, #16627, #24509 ) ;
#32383=CARTESIAN_POINT ( 'NONE',  ( -32.50000000000000000, 10.00000000000000888, 0.000000000000000000 ) ) ;
#32384=CARTESIAN_POINT ( 'NONE',  ( 7.570916362186213000, 16.14999999453761603, -23.30088464923126423 ) ) ;
#32385=CARTESIAN_POINT ( 'NONE',  ( -18.94512977948575738, 7.424999997268811214, -13.76444248337723231 ) ) ;
#32386=CARTESIAN_POINT ( 'NONE',  ( -2.162160676586881955E-15, 28.87500000273119838, -35.31076352940723240 ) ) ;
#32387=CARTESIAN_POINT ( 'NONE',  ( 10.04305231718578817, 27.90000000546238823, -30.90933677959249337 ) ) ;
#32388=CARTESIAN_POINT ( 'NONE',  ( -2.092463501923844636E-15, 73.49999999999998579, -34.17252228774368916 ) ) ;
#32389=CARTESIAN_POINT ( 'NONE',  ( 26.29305231718578995, 47.70000000546237118, -19.10302069950538240 ) ) ;
#32390=CARTESIAN_POINT ( 'NONE',  ( 4.635254915624209993, 73.40000000000001990, -14.26584774442730463 ) ) ;
#32392=CARTESIAN_POINT ( 'NONE',  ( 33.58253175000000113, 40.47500000273118559, -10.91162601494193751 ) ) ;
#32393=CARTESIAN_POINT ( 'NONE',  ( -18.94512977948576093, 8.324999997268822227, 13.76444248337722698 ) ) ;
#32394=CARTESIAN_POINT ( 'NONE',  ( 26.29305231718579350, 14.79999999999997939, 19.10302069950537529 ) ) ;
#32398=CARTESIAN_POINT ( 'NONE',  ( -33.58253175000000113, 63.02500000273118985, -10.91162601494193218 ) ) ;
#32399=CARTESIAN_POINT ( 'NONE',  ( -33.58253175000000113, 49.47500000273118559, 10.91162601494193929 ) ) ;
#32401=CARTESIAN_POINT ( 'NONE',  ( -33.58253175000000113, 7.225000002731182924, 10.91162601494193929 ) ) ;
#32404=CARTESIAN_POINT ( 'NONE',  ( -26.29305231718579350, 19.79999999999998295, -19.10302069950537884 ) ) ;
#32406=AXIS2_PLACEMENT_3D ( 'NONE', #18838, #32024, #28064 ) ;
#32407=LINE ( 'NONE', #11317, #23183 ) ;
#32409=CARTESIAN_POINT ( 'NONE',  ( -10.04305231718579172, 58.10000000546239107, -30.90933677959248982 ) ) ;
#32412=CARTESIAN_POINT ( 'NONE',  ( 32.50000000000000000, 49.09999999999999432, -10.55989012756945833 ) ) ;
#32413=( BOUNDED_CURVE ( )  B_SPLINE_CURVE ( 2, ( #22536, #6918, #17400, #27864, #21956, #667, #8734, #18884, #32404, #24197, #11155, #32242, #3425 ),
 .UNSPECIFIED., .F., .T. ) 
 B_SPLINE_CURVE_WITH_KNOTS ( ( 3, 2, 2, 2, 2, 2, 3 ),
 ( 0.7628205128205127750, 0.7641025641025640525, 0.7666666666666667185, 0.7692307692307692735, 0.7717948717948718285, 0.7743589743589743835, 0.7756410256410256610 ),
 .UNSPECIFIED. ) 
 CURVE ( )  GEOMETRIC_REPRESENTATION_ITEM ( )  RATIONAL_B_SPLINE_CURVE ( ( 0.9755282581475768211, 0.9755282581475768211, 1.000000000000000000, 0.9510565162951535312, 1.000000000000000000, 0.9510565162951535312, 1.000000000000000000, 0.9510565162951535312, 1.000000000000000000, 0.9510565162951535312, 1.000000000000000000, 0.9755282581475768211, 0.9755282581475768211 ) ) 
 REPRESENTATION_ITEM ( '' )  );
#32414=FILL_AREA_STYLE_COLOUR ( '', #26584 ) ;
#32418=DIRECTION ( 'NONE',  ( 0.000000000000000000, 0.000000000000000000, -1.000000000000000000 ) ) ;
#32423=CARTESIAN_POINT ( 'NONE',  ( -32.50000000000000000, 64.60000000546239107, 10.55989012756946366 ) ) ;
#32424=CARTESIAN_POINT ( 'NONE',  ( -27.16883889988623935, 49.57500000273118701, 19.73931689729374739 ) ) ;
#32425=CARTESIAN_POINT ( 'NONE',  ( 32.50000000000000711, 51.40000000546238823, 10.55989012756945122 ) ) ;
#32426=EDGE_CURVE ( 'NONE', #1865, #19851, #26910, .T. ) ;
#32428=CARTESIAN_POINT ( 'NONE',  ( -27.16883889988624290, 32.92500000273118843, -19.73931689729374028 ) ) ;
#32429=CARTESIAN_POINT ( 'NONE',  ( 5.147494310547428675, 77.05125428700924317, 32.50000000000000000 ) ) ;
#32430=CARTESIAN_POINT ( 'NONE',  ( -33.58253175000000113, 61.37500000273119127, 0.000000000000000000 ) ) ;
#32432=CARTESIAN_POINT ( 'NONE',  ( 10.04305231718579705, 38.59999999999999432, 30.90933677959248982 ) ) ;
#32434=CARTESIAN_POINT ( 'NONE',  ( 10.37757302488624767, 3.975000002731182924, 31.93888565452638417 ) ) ;
#32437=CARTESIAN_POINT ( 'NONE',  ( -33.58253175000000113, 71.37500000273119838, 0.000000000000000000 ) ) ;
#32438=CARTESIAN_POINT ( 'NONE',  ( 24.50000000000000000, 3.849999994537637082, -7.960532557706203605 ) ) ;
#32441=CARTESIAN_POINT ( 'NONE',  ( -7.570916362186210335, 4.349999994537640191, -23.30088464923126779 ) ) ;
#32453=CARTESIAN_POINT ( 'NONE',  ( -32.50000000000000000, 58.10000000000000142, 10.55989012756946366 ) ) ;
#32454=CARTESIAN_POINT ( 'NONE',  ( -4.223320258572819786E-15, 17.50000000000000000, 24.50000000000000000 ) ) ;
#32455=ORIENTED_EDGE ( 'NONE', *, *, #14537, .F. ) ;
#32457=CARTESIAN_POINT ( 'NONE',  ( 2.489536152421872915E-14, 75.50000000000001421, -32.49999999999999289 ) ) ;
#32463=CARTESIAN_POINT ( 'NONE',  ( -7.570916362186210335, 12.34999999453761887, -23.30088464923126779 ) ) ;
#32464=CARTESIAN_POINT ( 'NONE',  ( -33.58253175000000113, 55.12500000273118417, 0.000000000000000000 ) ) ;
#32466=CARTESIAN_POINT ( 'NONE',  ( -2.092463501923844636E-15, 12.00000000546238610, -34.17252228774368916 ) ) ;
#32467=CARTESIAN_POINT ( 'NONE',  ( 7.313012447739250820E-14, 11.49999999999999112, 24.50000000000000000 ) ) ;
#32468=CARTESIAN_POINT ( 'NONE',  ( -23.41746824999999887, 18.02499999726880731, -7.608796670333730638 ) ) ;
#32469=CARTESIAN_POINT ( 'NONE',  ( 32.50000000000000711, 56.90000000000001279, 10.55989012756945122 ) ) ;
#32470=CARTESIAN_POINT ( 'NONE',  ( 10.37757302488624767, 25.97500000273117493, 31.93888565452638417 ) ) ;
#32471=CARTESIAN_POINT ( 'NONE',  ( -8.891200544363830713E-16, 77.50000000000001421, -15.00000000000000000 ) ) ;
#32473=CARTESIAN_POINT ( 'NONE',  ( 4.300734207923757602, 74.27500000273118985, -13.23629886949340673 ) ) ;
#32474=CARTESIAN_POINT ( 'NONE',  ( 32.50000000000000711, 64.89999999999999147, 10.55989012756945122 ) ) ;
#32477=ORIENTED_EDGE ( 'NONE', *, *, #6000, .F. ) ;
#32479=CARTESIAN_POINT ( 'NONE',  ( -13.91746824999999532, 76.97500000273119269, 4.522059556121122093 ) ) ;
#32481=CARTESIAN_POINT ( 'NONE',  ( 20.75514604977248467, 20.42500000273120619, -28.56700777964554305 ) ) ;
#32485=CARTESIAN_POINT ( 'NONE',  ( 27.16883889988623935, 6.575000002731201221, -19.73931689729374384 ) ) ;
#32489=EDGE_CURVE ( 'NONE', #22185, #13788, #33941, .T. ) ;
#32490=CARTESIAN_POINT ( 'NONE',  ( 11.25946833292375793, 78.57500000273121543, -8.180482586598735395 ) ) ;
#32491=VECTOR ( 'NONE', #3639, 1000.000000000000000 ) ;
#32493=CARTESIAN_POINT ( 'NONE',  ( -24.50000000000000000, 2.749999994537621895, -3.000384657911015469E-15 ) ) ;
#32494=CARTESIAN_POINT ( 'NONE',  ( -10.37757302488623701, 53.52500000273118985, 31.93888565452638417 ) ) ;
#32497=ORIENTED_EDGE ( 'NONE', *, *, #29282, .F. ) ;
#32499=CARTESIAN_POINT ( 'NONE',  ( -7.236395654485763274, 8.024999997268800200, 22.27133577429736633 ) ) ;
#32501=EDGE_LOOP ( 'NONE', ( #8549, #9760, #29396, #19848 ) ) ;
#32503=CARTESIAN_POINT ( 'NONE',  ( 3.880418787951140036, 6.448745718453147369, -24.49999999999999645 ) ) ;
#32504=ORIENTED_EDGE ( 'NONE', *, *, #3708, .T. ) ;
#32506=CARTESIAN_POINT ( 'NONE',  ( -33.58253175000000113, 63.37500000273119127, 0.000000000000000000 ) ) ;
#32508=CARTESIAN_POINT ( 'NONE',  ( 33.58253175000000113, 72.12500000273119838, -4.112674001490185761E-15 ) ) ;
#32510=CARTESIAN_POINT ( 'NONE',  ( -19.82091636218621034, 4.799999999999998934, -14.40073868116559552 ) ) ;
#32511=CARTESIAN_POINT ( 'NONE',  ( -20.75514604977248112, 3.675000002731179549, 28.56700777964554661 ) ) ;
#32512=CARTESIAN_POINT ( 'NONE',  ( 20.75514604977248467, 18.42500000273117422, -28.56700777964554305 ) ) ;
#32513=CARTESIAN_POINT ( 'NONE',  ( 4.300734207923761154, 75.47500000273119269, 13.23629886949340495 ) ) ;
#32515=CARTESIAN_POINT ( 'NONE',  ( 4.300734207923757602, 72.77500000273118985, -13.23629886949340673 ) ) ;
#32518=CARTESIAN_POINT ( 'NONE',  ( 4.445600272181915325E-13, 27.50000000000000355, -32.50000000000000000 ) ) ;
#32520=CARTESIAN_POINT ( 'NONE',  ( 20.08610463437157279, 49.80000000546238681, -27.64615127144129758 ) ) ;
#32522=CARTESIAN_POINT ( 'NONE',  ( 27.16883889988624290, 39.92500000273119554, 19.73931689729373673 ) ) ;
#32525=CARTESIAN_POINT ( 'NONE',  ( -20.75514604977248823, 29.07500000273119056, -28.56700777964554305 ) ) ;
#32528=CARTESIAN_POINT ( 'NONE',  ( -10.04305231718579172, 8.100000005462376862, -30.90933677959248982 ) ) ;
#32529=EDGE_CURVE ( 'NONE', #4234, #6801, #141, .T. ) ;
#32530=CARTESIAN_POINT ( 'NONE',  ( -32.50000000000000000, 44.60000000546237686, 10.55989012756946366 ) ) ;
#32533=CARTESIAN_POINT ( 'NONE',  ( -7.236395654485757944, 13.22499999726881015, -22.27133577429736988 ) ) ;
#32535=CARTESIAN_POINT ( 'NONE',  ( 5.779280353836490358E-15, 23.00000000546237899, 32.49999999999999289 ) ) ;
#32538=CARTESIAN_POINT ( 'NONE',  ( 27.16883889988623935, 12.32500000273117990, -19.73931689729374384 ) ) ;
#32539=CARTESIAN_POINT ( 'NONE',  ( 14.47279130897151767, 7.424999997268820096, -19.92008829642072598 ) ) ;
#32542=ORIENTED_EDGE ( 'NONE', *, *, #23533, .T. ) ;
#32545=ORIENTED_EDGE ( 'NONE', *, *, #3089, .F. ) ;
#32548=CARTESIAN_POINT ( 'NONE',  ( -32.50000000000000000, 10.10000000000000142, 10.55989012756946366 ) ) ;
#32549=CARTESIAN_POINT ( 'NONE',  ( -19.82091636218621389, 18.94999999453761319, 14.40073868116558842 ) ) ;
#32550=CARTESIAN_POINT ( 'NONE',  ( -18.94512977948576093, 3.824999997268818674, 13.76444248337722698 ) ) ;
#32551=CARTESIAN_POINT ( 'NONE',  ( -33.58253175000000113, 23.27500000273116854, -10.91162601494193218 ) ) ;
#32552=CARTESIAN_POINT ( 'NONE',  ( 20.08610463437157279, 31.80000000546237260, -27.64615127144129758 ) ) ;
#32553=CARTESIAN_POINT ( 'NONE',  ( 26.29305231718579350, 70.79999999999999716, 19.10302069950537529 ) ) ;
#32554=CARTESIAN_POINT ( 'NONE',  ( -32.50000000000000000, 6.500000005462358565, 0.000000000000000000 ) ) ;
#32555=DIRECTION ( 'NONE',  ( -0.000000000000000000, -1.000000000000000000, -0.000000000000000000 ) ) ;
#32557=CARTESIAN_POINT ( 'NONE',  ( -27.16883889988623935, 35.57500000273120122, 19.73931689729374739 ) ) ;
#32560=CARTESIAN_POINT ( 'NONE',  ( 14.47279130897151767, 13.42499999726880411, -19.92008829642072598 ) ) ;
#32561=CARTESIAN_POINT ( 'NONE',  ( -32.50000000000000000, 11.90000000000000391, -10.55989012756945478 ) ) ;
#32564=CARTESIAN_POINT ( 'NONE',  ( 20.75514604977249178, 59.82500000273117280, 28.56700777964553950 ) ) ;
#32565=CARTESIAN_POINT ( 'NONE',  ( -10.37757302488624411, 48.97500000273119269, -31.93888565452638417 ) ) ;
#32567=CARTESIAN_POINT ( 'NONE',  ( -1.778240108872766143E-15, 68.00000000546238255, -32.49999999999999289 ) ) ;
#32568=CARTESIAN_POINT ( 'NONE',  ( -10.37757302488624411, 4.725000002731183812, -31.93888565452638417 ) ) ;
#32570=CARTESIAN_POINT ( 'NONE',  ( 32.50000000000000711, 25.40000000546237047, 10.55989012756945122 ) ) ;
#32576=CARTESIAN_POINT ( 'NONE',  ( -32.50000000000000000, 30.60000000546238041, 10.55989012756946366 ) ) ;
#32579=CARTESIAN_POINT ( 'NONE',  ( -33.58253175000000113, 39.12500000273119838, 0.000000000000000000 ) ) ;
#32584=VECTOR ( 'NONE', #21635, 1000.000000000000000 ) ;
#32585=DIRECTION ( 'NONE',  ( 0.000000000000000000, -0.000000000000000000, -1.000000000000000000 ) ) ;
#32590=CARTESIAN_POINT ( 'NONE',  ( 32.50000000000000000, 20.99999999999998934, -3.980102097228898626E-15 ) ) ;
#32591=CARTESIAN_POINT ( 'NONE',  ( -33.58253175000000113, 43.27500000273117564, -10.91162601494193218 ) ) ;
#32592=CARTESIAN_POINT ( 'NONE',  ( 26.29305231718579350, 51.30000000546236549, 19.10302069950537529 ) ) ;
#32594=CARTESIAN_POINT ( 'NONE',  ( 27.16883889988624290, 31.92500000273118488, 19.73931689729373673 ) ) ;
#32595=CARTESIAN_POINT ( 'NONE',  ( 10.04305231718578817, 77.90000000546237402, -30.90933677959249337 ) ) ;
#32596=CARTESIAN_POINT ( 'NONE',  ( 33.58253175000000823, 56.27500000273116854, 10.91162601494192863 ) ) ;
#32598=CARTESIAN_POINT ( 'NONE',  ( -2.092463501923844636E-15, 33.50000000000001421, -34.17252228774368916 ) ) ;
#32600=CARTESIAN_POINT ( 'NONE',  ( -33.58253175000000113, 7.275000002731181858, -10.91162601494193218 ) ) ;
#32602=CARTESIAN_POINT ( 'NONE',  ( -4.934616302121927505E-14, 71.00000000546238255, 32.50000000000000000 ) ) ;
#32604=CARTESIAN_POINT ( 'NONE',  ( 27.16883889988623935, 64.57500000273120122, -19.73931689729374384 ) ) ;
#32605=CARTESIAN_POINT ( 'NONE',  ( -19.82091636218621034, 4.799999999999998934, -14.40073868116559552 ) ) ;
#32606=ORIENTED_EDGE ( 'NONE', *, *, #33839, .T. ) ;
#32607=CARTESIAN_POINT ( 'NONE',  ( -15.14183272437241889, 2.449999994537622960, -20.84094480462497856 ) ) ;
#32610=( BOUNDED_SURFACE ( )  B_SPLINE_SURFACE ( 1, 2, ( 
 ( #28936, #23463, #2696, #2861, #12818, #23291, #33759, #10251, #8171, #29100, #20732, #31172, #7664, #28769, #33925, #10415, #18323, #98, #24464, #3697, #3530, #21895, #19655, #32675, #605, #9171, #5939, #32181, #18994, #29438, #16748, #26872, #16420, #11420, #3367, #27374, #13837, #5773, #16253, #940, #11260, #14170, #11583, #19158, #11097, #21736, #26709, #3206, #13674, #24791, #32345, #3863, #16913, #14335, #9009, #24627, #1270, #24304, #19489, #29938, #21566, #11750, #8839, #29597, #1100, #19322, #32011, #29764, #6442, #22064, #32508, #6099, #22230, #24138, #8506, #778, #16580, #8676, #27035, #14002, #6271, #27206, #1444, #25132, #9332, #22735, #17763, #12258, #9513, #4709, #4540, #1609, #4200, #2132, #9688, #15013, #20169, #27884, #4367, #22555, #30787, #14503, #27711, #14672, #12607, #6940, #23076, #30612, #33008, #25653, #7108, #19818, #12087, #30270, #17251, #24961, #19994, #11921, #17423, #7280, #22392, #30442, #28222, #14842, #32841, #15189, #28052, #6770, #25308, #33185, #17590, #1780, #25484, #1963, #20337, #12437, #22907, #33364, #33537, #9860, #10040, #30097, #6604, #17081, #27541, #4028, #26499, #23424, #29059, #20694, #23761, #18452, #2308, #5564, #31301, #8134, #13464, #23592, #23254, #15873, #33885, #15537, #5397, #10377, #2656, #15364, #26330, #2483, #2818, #25818, #7627, #20855, #226, #28894, #18623, #31136, #10714, #21193, #12781, #16044, #13118, #7794, #13286, #15707, #33717, #57, #31635, #2992, #23931, #18284, #399, #20516, #10214, #30962, #28729, #7460, #17943, #18107, #28393, #28556, #5053, #25989, #12951, #10545, #4882, #21024, #5225, #26163, #31474, #7966, #18953, #16870, #24421, #29720, #898, #8632, #19116, #3326, #11537, #29229, #8464, #29398, #27332, #21691, #3819, #11380, #13796, #6394, #21855, #566, #5898, #11057, #31970, #5734, #24264, #16214, #32137, #22020, #26667, #16377, #32464, #11217, #3163, #8965, #8795, #13634, #29554, #26990, #32302, #26830, #732, #6054, #1057, #19278, #16538, #3489, #19447, #6226, #13958, #16705, #27160, #14129, #3652, #24098, #14292, #24585, #29893, #21522, #24749, #10885, #21360, #31803, #8294, #18785, #28180, #4324, #3986, #30570, #14629, #30225, #20126, #25087, #17377, #30057, #7067, #17207, #17550, #6562, #22350, #1566, #17037, #27666, #22188, #32635, #1225, #20295, #6896, #22862, #12392, #33320, #30743, #28009, #4495, #11877, #1915, #32797, #11705, #6725, #12042, #27497, #9129, #9290, #32964, #19775, #25439, #14459, #25263, #22513, #1737, #9818, #22690, #7234, #4156, #19611, #27840, #24916, #9467, #14798, #17722, #4667, #1401, #15147, #14971, #19949, #30395, #33140, #12217, #9644, #12737, #17899, #20981, #5184, #10339, #23551, #23381, #7753, #5522, #18579, #20468, #29020, #25777, #18065, #4838, #15319, #2614, #23208, #2263, #31259, #33670, #13243, #10167, #25611, #2091, #20815, #31091, #14, #31430, #5008, #20651, #18240, #28352, #15833, #30920, #7588, #33844, #183, #7923, #28686, #28513, #23717, #15491, #15667, #10672, #26117, #12565, #18408, #25945, #28854, #2439, #10502, #33494, #12907, #13077, #5352, #26289, #23036, #2778, #21151, #31592, #8092, #9995, #7413, #8756, #8252, #32096, #8924, #24221, #19240, #26457, #21320, #13919, #24056, #2948, #26949, #18745, #13420, #692, #10842, #3449, #31761, #29187, #16665, #859, #1017, #26791, #27122, #11011, #5692, #3615, #524, #29855, #16001, #11178, #21481, #24386, #21815, #29356, #31928, #21649, #16170, #6183, #26626, #3121, #8591, #24546, #11339, #19076, #8420, #14089, #13592, #29515, #11500, #6019, #19407, #32264, #18910, #29678, #5857, #21979, #23887, #16335, #16495, #32428, #358, #3283, #13751, #19908, #27971, #17000, #22316, #25222, #33101, #32594, #22476, #33280, #14591, #9604, #16835, #11669, #4285, #14423, #27290, #17338, #9093, #3782, #25050, #1187, #27801, #22150, #19575, #7027, #1700, #25397, #17172, #17510, #1359, #30023, #1874, #12177, #22648, #27457, #4454, #3948, #6356, #11838, #6688, #6527, #14253, #24877, #4117, #32761, #30530, #9255, #30357, #27629, #6859, #14931, #14759, #12352, #19740, #24710, #32924, #30185, #1531, #12005, #22821, #9776, #9423, #20258, #20086, #23512, #16257, #28643, #28141, #10127, #17857, #22994, #26079, #10300, #15450, #5140, #28477, #12867, #11101, #24142, #25571, #610, #30876, #23166, #9952, #20427, #7714, #28309, #7373, #2399, #4797, #15276, #31391, #25737, #30702, #2217, #31054, #2051, #7198, #12696, #4973, #33628, #20942, #33453, #20777, #7546, #31221, #5777, #18201, #18371, #20609, #15106, #23345, #18031, #25905, #33806, #3210, #26714, #4627, #28816, #33970, #10464, #13678, #15628, #12526, #2575, #13041, #7881, #17679, #1104, #6276, #19494, #19326, #3702, #1448, #14507, #16424, #24966, #21740, #14006, #782, #11264, #32512, #8680, #32185, #27210, #19164, #9175, #29601, #21570, #32015, #16752, #27040, #29942, #27378, #944, #6103, #14174, #24308, #11754, #26876, #16584, #29768, #30102, #16918, #24631, #24469, #19659, #3534, #11589, #6608, #22068, #8511, #3867, #11424, #14339, #21899, #6446, #29442, #32351, #9013, #24796, #1274, #18998, #22235, #32680, #17085, #8843, #27545, #4032, #5945, #13842, #3371, #4886, #20173, #15194, #22396, #17255, #9864, #19998, #32845, #22912, #4204, #9337, #30616, #6774, #33368, #27716, #14676, #12611, #30791, #30967, #22739, #23080, #6944, #25137, #7465, #17768, #28227, #20341, #30446, #4372, #9517, #2136, #1967, #17427, #12262, #10044, #7284, #33189, #27888, #12442, #25657, #17594, #1613, #17948, #14846, #20521, #12091, #33541, #4713, #22560, #28397, #9692, #15368, #25823, #15018, #33012, #11927, #25312, #1785, #19822, #7112, #28056, #4544, #30274, #25488, #26334, #20698, #25993, #18288, #31140, #10381, #12785, #23258, #2312, #26504, #21029, #29063, #5568, #16050, #21197, #2823, #2997, #12955, #31640, #8138, #28561, #13470, #31479, #5229, #23765, #10548, #15541, #7970, #18627, #232, #10718, #15712, #33721, #10219, #2487, #7631, #23596, #18112, #5057, #28733, #23430, #26168, #2661, #18456, #13121, #33889, #20859, #31306, #13291, #7799, #61, #28899, #5401, #15877, #12554, #17887, #23025, #30731, #7224 ),
 ( #12894, #25932, #27828, #2426, #33127, #25426, #12205, #22676, #9982, #28340, #9807, #4484, #33480, #2249, #4656, #1725, #4996, #1904, #7574, #9631, #12723, #30907, #14786, #18054, #20283, #20636, #32952, #2079, #20113, #4825, #12381, #27997, #15305, #22850, #15136, #4311, #25764, #14960, #23194, #25250, #30558, #33308, #7054, #17710, #19936, #30383, #9454, #28499, #25600, #31079, #10154, #15479, #33656, #7401, #6884, #17537, #17365, #28168, #20456, #10999, #15989, #2765, #18733, #18565, #15654, #26445, #26612, #29175, #5680, #13229, #3110, #8240, #18228, #31916, #23704, #24044, #513, #28674, #29344, #26104, #5169, #18395, #2602, #2936, #21470, #5508, #170, #8409, #31748, #28841, #31418, #5845, #13406, #16158, #23875, #21139, #31580, #15821, #18897, #7739, #20967, #7911, #16324, #10660, #26780, #345, #26275, #3271, #10829, #13063, #5339, #23539, #10490, #33989, #8080, #29008, #21308, #23369, #13582, #33830, #10327, #20803, #31247, #1912, #12214, #7410, #14795, #1734, #25259, #20292, #22687, #2260, #33137, #28509, #14626, #33316, #20123, #20648, #28177, #33490, #4664, #12389, #22858, #7064, #15315, #32961, #9640, #30567, #31089, #25436, #7586, #15144, #17547, #10164, #25608, #4321, #28006, #4492, #14968, #9463, #9815, #19946, #30740, #25774, #30391, #7232, #12734, #17718, #6893, #23205, #25084, #2087, #23033, #12562, #9992, #20465, #30916, #17896, #4835, #28349, #33667, #18064, #1563, #12039, #22509, #17374, #27837, #8250, #10670, #7749, #11009, #7921, #13590, #5182, #18743, #2946, #20813, #24054, #15831, #26623, #31926, #8090, #18238, #356, #18406, #11, #23885, #28851, #21149, #33842, #10840, #20978, #21317, #10337, #26114, #5350, #31257, #31428, #25943, #2437, #5006, #522, #31591, #3119, #16168, #21479, #29185, #13417, #8418, #15665, #5690, #18907, #28684, #15489, #18577, #26287, #31759, #180, #2612, #29018, #12904, #23379, #13075, #2776, #23549, #10500, #13240, #23714, #5520, #15999, #26455, #690, #1357, #32093, #11176, #24384, #8589, #21977, #16997, #11498, #8754, #3946, #3780, #857, #3447, #11337, #11666, #6017, #14251, #3281, #13917, #32425, #32592, #29853, #26789, #1185, #8922, #27455, #16492, #21813, #24708, #22148, #21647, #19405, #22314, #3613, #9091, #5854, #19073, #27288, #32261, #16333, #6354, #29513, #13748, #14086, #24219, #16833, #26947, #19238, #30021, #19573, #14421, #6181, #6525, #29676, #16663, #24874, #11836, #32759, #27120, #9253, #24544, #29354, #1015, #20084, #14588, #19738, #27799, #17507, #6857, #9949, #22474, #9773, #30527, #20256, #28307, #7196, #7370, #4283, #4114, #12350, #32922, #9602, #25395, #25735, #4795, #17170, #17854, #12524, #22992, #15274, #17677, #27627, #33099, #17335, #12003, #15104, #33278, #4452, #28139, #27969, #1872, #33625, #12693, #25048, #23162, #19906, #7025, #14757, #33451, #30355, #25220, #1698, #22819, #12174, #2214, #22646, #30183, #6686, #14929, #30699, #4625, #25569, #2049, #20425, #30874, #9421, #1529, #4969, #10297, #18368, #18706, #5480, #5310, #2570, #8213, #33804, #2736, #31722, #15791, #3080, #15959, #23676, #13038, #5648, #21109, #20774, #5137, #31218, #7711, #15447, #23509, #28474, #31388, #21281, #25902, #18198, #29144, #10461, #2395, #16130, #24013, #28641, #18536, #15624, #31552, #26075, #33967, #20939, #313, #140, #7878, #28812, #26585, #28981, #26248, #13199, #10631, #13377, #8050, #12864, #13550, #26415, #10124, #2909, #23849, #10801, #23341, #20605, #31051, #7543, #18028, #3573, #3244, #29811, #13880, #29476, #19368, #24347, #16624, #29313, #6313, #16457, #16790, #5816, #21608, #819, #16293, #26909, #21441, #31885, #485, #19530, #6139, #22107, #11624, #32552, #3741, #8882, #9051, #649, #14212, #24668, #26751, #29980, #27078, #11299, #27248, #29636, #13712, #14044, #1142, #6485, #16957, #21778, #27416, #3906, #24178, #14375, #32225, #10967, #8381, #11139, #18866, #32053, #8552, #5980, #19037, #24505, #3408, #979, #8714, #19197, #11463, #21937, #32387, #30830, #4409, #9728, #14886, #22600, #33054, #17291, #25527, #9212, #22432, #32879, #7324, #1653, #17808, #17125, #6983, #28266, #9559, #28094, #1312, #30141, #22777, #9378, #11795, #1827, #27582, #22273, #20037, #19695, #12305, #6645, #4071, #2004, #20214, #9904, #12128, #12479, #19859, #14546, #20381, #30654, #7151, #1487, #22949, #30314, #24834, #6811, #25174, #25005, #32715, #27753, #30482, #11961, #15060, #4241, #25347, #17466, #33229, #33407, #17633, #4752, #14715, #27926, #4583, #28434, #5096, #21362, #21693, #24266, #12646, #13798, #8467, #18955, #734, #13636, #23117, #28597, #2349, #7502, #11059, #29231, #402, #24100, #13467, #31805, #29556, #8635, #10079, #19119, #15404, #2994, #12824, #29400, #25860, #23295, #33763, #8296, #10255, #3328, #20736, #15229, #25692, #10888, #31178, #568, #21524, #16046, #7668, #18787, #17986, #5902, #20560, #18155, #23933, #11219, #31972, #5736, #26501, #32139, #4924, #16216, #2173, #26670, #33580, #16379, #3166, #26832, #31005, #24918, #13960, #14131, #22190, #9292, #6565, #3491, #11879, #19613, #27669, #16707, #22022, #1403, #32799, #6727, #1059, #900, #25090, #22352, #19777, #27162, #17211, #3654, #6056, #11540, #6396, #11382, #16540, #24587, #3821, #32466, #30227, #8797, #30059, #16872, #17039, #14632, #27499, #4159, #8967, #24423, #32637, #19280, #29895, #11707, #12046, #1569, #21857, #22516, #32967, #9470, #19952, #3989, #32305, #19449, #27335, #29722, #26992, #14462, #24752, #6228, #14294, #9131, #1227, #23385, #25266, #33847, #30572, #17724, #28011, #23211, #7069, #17552, #4497, #2094, #14973, #18068, #25442, #10342, #30399, #15149, #1917, #4841, #2267, #9820, #12394, #25613, #33142, #20654, #1739, #22865, #4669, #5012, #25779, #12567, #33322, #28517, #20128, #23038, #15494, #33496, #6899, #12740, #20297, #33673, #30746, #15323, #4327, #7236, #9998, #10171, #30923, #27844, #31094, #20471, #25948, #28182, #7416, #7591, #2442, #22692, #17902, #17380, #28355, #12910, #14801, #12218, #9648, #28857, #31262, #31763, #13080, #7757, #5525, #15670, #8256, #2617, #26120, #21484, #5695, #5860, #31595, #8423, #2951, #186, #29359 ) ),
 .UNSPECIFIED., .F., .F., .T. ) 
 B_SPLINE_SURFACE_WITH_KNOTS ( ( 2, 2 ),
 ( 3, 2, 2, 2, 2, 2, 2, 2, 2, 2, 2, 2, 2, 2, 2, 2, 2, 2, 2, 2, 2, 2, 2, 2, 2, 2, 2, 2, 2, 2, 2, 2, 2, 2, 2, 2, 2, 2, 2, 2, 2, 2, 2, 2, 2, 2, 2, 2, 2, 2, 2, 2, 2, 2, 2, 2, 2, 2, 2, 2, 2, 2, 2, 2, 2, 2, 2, 2, 2, 2, 2, 2, 2, 2, 2, 2, 2, 2, 2, 2, 2, 2, 2, 2, 2, 2, 2, 2, 2, 2, 2, 2, 2, 2, 2, 2, 2, 2, 2, 2, 2, 2, 2, 2, 2, 2, 2, 2, 2, 2, 2, 2, 2, 2, 2, 2, 2, 2, 2, 2, 2, 2, 2, 2, 2, 2, 2, 2, 2, 2, 2, 2, 2, 2, 2, 2, 2, 2, 2, 2, 2, 2, 2, 2, 2, 2, 2, 2, 2, 2, 2, 2, 2, 2, 2, 2, 2, 2, 2, 2, 2, 2, 2, 2, 2, 2, 2, 2, 2, 2, 2, 2, 2, 2, 2, 2, 2, 2, 2, 2, 2, 2, 2, 2, 2, 2, 2, 2, 2, 2, 2, 2, 2, 2, 2, 2, 2, 2, 2, 2, 2, 2, 2, 2, 2, 2, 2, 2, 2, 2, 2, 2, 2, 2, 2, 2, 2, 2, 2, 2, 2, 2, 2, 2, 2, 2, 2, 2, 2, 2, 2, 2, 2, 2, 2, 2, 2, 2, 2, 2, 2, 2, 2, 2, 2, 2, 2, 2, 2, 2, 2, 2, 2, 2, 2, 2, 2, 2, 2, 2, 2, 2, 2, 2, 2, 2, 2, 2, 2, 2, 2, 2, 2, 2, 2, 2, 2, 2, 2, 2, 2, 2, 2, 2, 2, 2, 2, 2, 2, 2, 2, 2, 2, 2, 2, 2, 2, 2, 2, 2, 2, 2, 2, 2, 2, 2, 2, 2, 2, 2, 2, 2, 2, 2, 2, 2, 2, 2, 2, 2, 2, 2, 2, 2, 2, 2, 2, 2, 2, 2, 2, 2, 2, 2, 2, 2, 2, 2, 2, 2, 2, 2, 2, 2, 2, 2, 2, 2, 2, 2, 2, 2, 2, 2, 2, 2, 2, 2, 2, 2, 2, 2, 2, 2, 2, 2, 2, 2, 2, 2, 2, 2, 2, 2, 2, 2, 2, 2, 2, 2, 2, 2, 2, 2, 2, 2, 2, 2, 2, 2, 3 ),
 ( 0.000000000000000000, 1.000000000000000000 ),
 ( 0.000000000000000000, 0.002564102564102564100, 0.005128205128205128201, 0.007692307692307692735, 0.01025641025641025640, 0.01282051282051282007, 0.01538461538461538547, 0.01794871794871794740, 0.02051282051282051280, 0.02307692307692307820, 0.02564102564102564014, 0.02820512820512820554, 0.03076923076923077094, 0.03333333333333333287, 0.03589743589743589480, 0.03846153846153846367, 0.04102564102564102561, 0.04358974358974358754, 0.04615384615384615641, 0.04871794871794871834, 0.05128205128205128027, 0.05384615384615384914, 0.05641025641025641107, 0.05897435897435897301, 0.06153846153846154188, 0.06410256410256409687, 0.06666666666666666574, 0.06923076923076923461, 0.07179487179487178961, 0.07435897435897435848, 0.07692307692307692735, 0.07948717948717948234, 0.08205128205128205121, 0.08461538461538462008, 0.08717948717948717507, 0.08974358974358974395, 0.09230769230769231282, 0.09487179487179486781, 0.09743589743589743668, 0.1000000000000000056, 0.1025641025641025605, 0.1051282051282051294, 0.1076923076923076983, 0.1102564102564102533, 0.1128205128205128221, 0.1153846153846153910, 0.1179487179487179460, 0.1205128205128205149, 0.1230769230769230838, 0.1256410256410256387, 0.1282051282051281937, 0.1307692307692307765, 0.1333333333333333315, 0.1358974358974358865, 0.1384615384615384692, 0.1410256410256410242, 0.1435897435897435792, 0.1461538461538461620, 0.1487179487179487170, 0.1512820512820512719, 0.1538461538461538547, 0.1564102564102564097, 0.1589743589743589647, 0.1615384615384615474, 0.1641025641025641024, 0.1666666666666666574, 0.1692307692307692402, 0.1717948717948717952, 0.1743589743589743501, 0.1769230769230769329, 0.1794871794871794879, 0.1820512820512820429, 0.1846153846153846256, 0.1871794871794871806, 0.1897435897435897356, 0.1923076923076923184, 0.1948717948717948734, 0.1974358974358974284, 0.2000000000000000111, 0.2025641025641025661, 0.2051282051282051211, 0.2076923076923077038, 0.2102564102564102588, 0.2128205128205128138, 0.2153846153846153966, 0.2179487179487179516, 0.2205128205128205066, 0.2230769230769230893, 0.2256410256410256443, 0.2282051282051281993, 0.2307692307692307820, 0.2333333333333333370, 0.2358974358974358920, 0.2384615384615384748, 0.2410256410256410298, 0.2435897435897435848, 0.2461538461538461675, 0.2487179487179487225, 0.2512820512820512775, 0.2538461538461538325, 0.2564102564102563875, 0.2589743589743589980, 0.2615384615384615530, 0.2641025641025641080, 0.2666666666666666630, 0.2692307692307692180, 0.2717948717948717730, 0.2743589743589743835, 0.2769230769230769384, 0.2794871794871794934, 0.2820512820512820484, 0.2846153846153846034, 0.2871794871794871584, 0.2897435897435897689, 0.2923076923076923239, 0.2948717948717948789, 0.2974358974358974339, 0.2999999999999999889, 0.3025641025641025439, 0.3051282051282051544, 0.3076923076923077094, 0.3102564102564102644, 0.3128205128205128194, 0.3153846153846153744, 0.3179487179487179294, 0.3205128205128205399, 0.3230769230769230949, 0.3256410256410256499, 0.3282051282051282048, 0.3307692307692307598, 0.3333333333333333148, 0.3358974358974358698, 0.3384615384615384803, 0.3410256410256410353, 0.3435897435897435903, 0.3461538461538461453, 0.3487179487179487003, 0.3512820512820512553, 0.3538461538461538658, 0.3564102564102564208, 0.3589743589743589758, 0.3615384615384615308, 0.3641025641025640858, 0.3666666666666666408, 0.3692307692307692513, 0.3717948717948718063, 0.3743589743589743613, 0.3769230769230769162, 0.3794871794871794712, 0.3820512820512820262, 0.3846153846153846367, 0.3871794871794871917, 0.3897435897435897467, 0.3923076923076923017, 0.3948717948717948567, 0.3974358974358974117, 0.4000000000000000222, 0.4025641025641025772, 0.4051282051282051322, 0.4076923076923076872, 0.4102564102564102422, 0.4128205128205127972, 0.4153846153846154077, 0.4179487179487179627, 0.4205128205128205177, 0.4230769230769230727, 0.4256410256410256276, 0.4282051282051281826, 0.4307692307692307931, 0.4333333333333333481, 0.4358974358974359031, 0.4384615384615384581, 0.4410256410256410131, 0.4435897435897435681, 0.4461538461538461786, 0.4487179487179487336, 0.4512820512820512886, 0.4538461538461538436, 0.4564102564102563986, 0.4589743589743589536, 0.4615384615384615641, 0.4641025641025641191, 0.4666666666666666741, 0.4692307692307692291, 0.4717948717948717841, 0.4743589743589743390, 0.4769230769230769496, 0.4794871794871795045, 0.4820512820512820595, 0.4846153846153846145, 0.4871794871794871695, 0.4897435897435897245, 0.4923076923076923350, 0.4948717948717948900, 0.4974358974358974450, 0.5000000000000000000, 0.5025641025641025550, 0.5051282051282051100, 0.5076923076923076650, 0.5102564102564102200, 0.5128205128205127750, 0.5153846153846153300, 0.5179487179487179960, 0.5205128205128205510, 0.5230769230769231060, 0.5256410256410256610, 0.5282051282051282159, 0.5307692307692307709, 0.5333333333333333259, 0.5358974358974358809, 0.5384615384615384359, 0.5410256410256409909, 0.5435897435897435459, 0.5461538461538461009, 0.5487179487179487669, 0.5512820512820513219, 0.5538461538461538769, 0.5564102564102564319, 0.5589743589743589869, 0.5615384615384615419, 0.5641025641025640969, 0.5666666666666666519, 0.5692307692307692069, 0.5717948717948717618, 0.5743589743589743168, 0.5769230769230768718, 0.5794871794871795379, 0.5820512820512820928, 0.5846153846153846478, 0.5871794871794872028, 0.5897435897435897578, 0.5923076923076923128, 0.5948717948717948678, 0.5974358974358974228, 0.5999999999999999778, 0.6025641025641025328, 0.6051282051282050878, 0.6076923076923076428, 0.6102564102564103088, 0.6128205128205128638, 0.6153846153846154188, 0.6179487179487179738, 0.6205128205128205288, 0.6230769230769230838, 0.6256410256410256387, 0.6282051282051281937, 0.6307692307692307487, 0.6333333333333333037, 0.6358974358974358587, 0.6384615384615384137, 0.6410256410256410797, 0.6435897435897436347, 0.6461538461538461897, 0.6487179487179487447, 0.6512820512820512997, 0.6538461538461538547, 0.6564102564102564097, 0.6589743589743589647, 0.6615384615384615197, 0.6641025641025640747, 0.6666666666666666297, 0.6692307692307691847, 0.6717948717948717396, 0.6743589743589744057, 0.6769230769230769607, 0.6794871794871795156, 0.6820512820512820706, 0.6846153846153846256, 0.6871794871794871806, 0.6897435897435897356, 0.6923076923076922906, 0.6948717948717948456, 0.6974358974358974006, 0.6999999999999999556, 0.7025641025641025106, 0.7051282051282051766, 0.7076923076923077316, 0.7102564102564102866, 0.7128205128205128416, 0.7153846153846153966, 0.7179487179487179516, 0.7205128205128205066, 0.7230769230769230616, 0.7256410256410256165, 0.7282051282051281715, 0.7307692307692307265, 0.7333333333333332815, 0.7358974358974359475, 0.7384615384615385025, 0.7410256410256410575, 0.7435897435897436125, 0.7461538461538461675, 0.7487179487179487225, 0.7512820512820512775, 0.7538461538461538325, 0.7564102564102563875, 0.7589743589743589425, 0.7615384615384614975, 0.7641025641025640525, 0.7666666666666667185, 0.7692307692307692735, 0.7717948717948718285, 0.7743589743589743835, 0.7769230769230769384, 0.7794871794871794934, 0.7820512820512820484, 0.7846153846153846034, 0.7871794871794871584, 0.7897435897435897134, 0.7923076923076922684, 0.7948717948717948234, 0.7974358974358974894, 0.8000000000000000444, 0.8025641025641025994, 0.8051282051282051544, 0.8076923076923077094, 0.8102564102564102644, 0.8128205128205128194, 0.8153846153846153744, 0.8179487179487179294, 0.8205128205128204844, 0.8230769230769230393, 0.8256410256410255943, 0.8282051282051282604, 0.8307692307692308153, 0.8333333333333333703, 0.8358974358974359253, 0.8384615384615384803, 0.8410256410256410353, 0.8435897435897435903, 0.8461538461538461453, 0.8487179487179487003, 0.8512820512820512553, 0.8538461538461538103, 0.8564102564102563653, 0.8589743589743589203, 0.8615384615384615863, 0.8641025641025641413, 0.8666666666666666963, 0.8692307692307692513, 0.8717948717948718063, 0.8743589743589743613, 0.8769230769230769162, 0.8794871794871794712, 0.8820512820512820262, 0.8846153846153845812, 0.8871794871794871362, 0.8897435897435896912, 0.8923076923076923572, 0.8948717948717949122, 0.8974358974358974672, 0.9000000000000000222, 0.9025641025641025772, 0.9051282051282051322, 0.9076923076923076872, 0.9102564102564102422, 0.9128205128205127972, 0.9153846153846153522, 0.9179487179487179072, 0.9205128205128204621, 0.9230769230769231282, 0.9256410256410256832, 0.9282051282051282382, 0.9307692307692307931, 0.9333333333333333481, 0.9358974358974359031, 0.9384615384615384581, 0.9410256410256410131, 0.9435897435897435681, 0.9461538461538461231, 0.9487179487179486781, 0.9512820512820512331, 0.9538461538461538991, 0.9564102564102564541, 0.9589743589743590091, 0.9615384615384615641, 0.9641025641025641191, 0.9666666666666666741, 0.9692307692307692291, 0.9717948717948717841, 0.9743589743589743390, 0.9769230769230768940, 0.9794871794871794490, 0.9820512820512820040, 0.9846153846153846700, 0.9871794871794872250, 0.9897435897435897800, 0.9923076923076923350, 0.9948717948717948900, 0.9974358974358974450, 1.000000000000000000 ),
 .UNSPECIFIED. ) 
 GEOMETRIC_REPRESENTATION_ITEM ( )  RATIONAL_B_SPLINE_SURFACE ( (
 ( 1.000000000000000000, 0.9510565162951535312, 1.000000000000000000, 0.9510565162951535312, 1.000000000000000000, 0.9510565162951535312, 1.000000000000000000, 0.9510565162951535312, 1.000000000000000000, 0.9510565162951535312, 1.000000000000000000, 0.9510565162951535312, 1.000000000000000000, 0.9510565162951535312, 1.000000000000000000, 0.9510565162951535312, 1.000000000000000000, 0.9510565162951535312, 1.000000000000000000, 0.9510565162951535312, 1.000000000000000000, 0.9510565162951535312, 1.000000000000000000, 0.9510565162951535312, 1.000000000000000000, 0.9510565162951535312, 1.000000000000000000, 0.9510565162951535312, 1.000000000000000000, 0.9510565162951535312, 1.000000000000000000, 0.9510565162951535312, 1.000000000000000000, 0.9510565162951535312, 1.000000000000000000, 0.9510565162951535312, 1.000000000000000000, 0.9510565162951535312, 1.000000000000000000, 0.9510565162951535312, 1.000000000000000000, 0.9510565162951535312, 1.000000000000000000, 0.9510565162951535312, 1.000000000000000000, 0.9510565162951535312, 1.000000000000000000, 0.9510565162951535312, 1.000000000000000000, 0.9510565162951535312, 1.000000000000000000, 0.9510565162951535312, 1.000000000000000000, 0.9510565162951535312, 1.000000000000000000, 0.9510565162951535312, 1.000000000000000000, 0.9510565162951535312, 1.000000000000000000, 0.9510565162951535312, 1.000000000000000000, 0.9510565162951535312, 1.000000000000000000, 0.9510565162951535312, 1.000000000000000000, 0.9510565162951535312, 1.000000000000000000, 0.9510565162951535312, 1.000000000000000000, 0.9510565162951535312, 1.000000000000000000, 0.9510565162951535312, 1.000000000000000000, 0.9510565162951535312, 1.000000000000000000, 0.9510565162951535312, 1.000000000000000000, 0.9510565162951535312, 1.000000000000000000, 0.9510565162951535312, 1.000000000000000000, 0.9510565162951535312, 1.000000000000000000, 0.9510565162951535312, 1.000000000000000000, 0.9510565162951535312, 1.000000000000000000, 0.9510565162951535312, 1.000000000000000000, 0.9510565162951535312, 1.000000000000000000, 0.9510565162951535312, 1.000000000000000000, 0.9510565162951535312, 1.000000000000000000, 0.9510565162951535312, 1.000000000000000000, 0.9510565162951535312, 1.000000000000000000, 0.9510565162951535312, 1.000000000000000000, 0.9510565162951535312, 1.000000000000000000, 0.9510565162951535312, 1.000000000000000000, 0.9510565162951535312, 1.000000000000000000, 0.9510565162951535312, 1.000000000000000000, 0.9510565162951535312, 1.000000000000000000, 0.9510565162951535312, 1.000000000000000000, 0.9510565162951535312, 1.000000000000000000, 0.9510565162951535312, 1.000000000000000000, 0.9510565162951535312, 1.000000000000000000, 0.9510565162951535312, 1.000000000000000000, 0.9510565162951535312, 1.000000000000000000, 0.9510565162951535312, 1.000000000000000000, 0.9510565162951535312, 1.000000000000000000, 0.9510565162951535312, 1.000000000000000000, 0.9510565162951535312, 1.000000000000000000, 0.9510565162951535312, 1.000000000000000000, 0.9510565162951535312, 1.000000000000000000, 0.9510565162951535312, 1.000000000000000000, 0.9510565162951535312, 1.000000000000000000, 0.9510565162951535312, 1.000000000000000000, 0.9510565162951535312, 1.000000000000000000, 0.9510565162951535312, 1.000000000000000000, 0.9510565162951535312, 1.000000000000000000, 0.9510565162951535312, 1.000000000000000000, 0.9510565162951535312, 1.000000000000000000, 0.9510565162951535312, 1.000000000000000000, 0.9510565162951535312, 1.000000000000000000, 0.9510565162951535312, 1.000000000000000000, 0.9510565162951535312, 1.000000000000000000, 0.9510565162951535312, 1.000000000000000000, 0.9510565162951535312, 1.000000000000000000, 0.9510565162951535312, 1.000000000000000000, 0.9510565162951535312, 1.000000000000000000, 0.9510565162951535312, 1.000000000000000000, 0.9510565162951535312, 1.000000000000000000, 0.9510565162951535312, 1.000000000000000000, 0.9510565162951535312, 1.000000000000000000, 0.9510565162951535312, 1.000000000000000000, 0.9510565162951535312, 1.000000000000000000, 0.9510565162951535312, 1.000000000000000000, 0.9510565162951535312, 1.000000000000000000, 0.9510565162951535312, 1.000000000000000000, 0.9510565162951535312, 1.000000000000000000, 0.9510565162951535312, 1.000000000000000000, 0.9510565162951535312, 1.000000000000000000, 0.9510565162951535312, 1.000000000000000000, 0.9510565162951535312, 1.000000000000000000, 0.9510565162951535312, 1.000000000000000000, 0.9510565162951535312, 1.000000000000000000, 0.9510565162951535312, 1.000000000000000000, 0.9510565162951535312, 1.000000000000000000, 0.9510565162951535312, 1.000000000000000000, 0.9510565162951535312, 1.000000000000000000, 0.9510565162951535312, 1.000000000000000000, 0.9510565162951535312, 1.000000000000000000, 0.9510565162951535312, 1.000000000000000000, 0.9510565162951535312, 1.000000000000000000, 0.9510565162951535312, 1.000000000000000000, 0.9510565162951535312, 1.000000000000000000, 0.9510565162951535312, 1.000000000000000000, 0.9510565162951535312, 1.000000000000000000, 0.9510565162951535312, 1.000000000000000000, 0.9510565162951535312, 1.000000000000000000, 0.9510565162951535312, 1.000000000000000000, 0.9510565162951535312, 1.000000000000000000, 0.9510565162951535312, 1.000000000000000000, 0.9510565162951535312, 1.000000000000000000, 0.9510565162951535312, 1.000000000000000000, 0.9510565162951535312, 1.000000000000000000, 0.9510565162951535312, 1.000000000000000000, 0.9510565162951535312, 1.000000000000000000, 0.9510565162951535312, 1.000000000000000000, 0.9510565162951535312, 1.000000000000000000, 0.9510565162951535312, 1.000000000000000000, 0.9510565162951535312, 1.000000000000000000, 0.9510565162951535312, 1.000000000000000000, 0.9510565162951535312, 1.000000000000000000, 0.9510565162951535312, 1.000000000000000000, 0.9510565162951535312, 1.000000000000000000, 0.9510565162951535312, 1.000000000000000000, 0.9510565162951535312, 1.000000000000000000, 0.9510565162951535312, 1.000000000000000000, 0.9510565162951535312, 1.000000000000000000, 0.9510565162951535312, 1.000000000000000000, 0.9510565162951535312, 1.000000000000000000, 0.9510565162951535312, 1.000000000000000000, 0.9510565162951535312, 1.000000000000000000, 0.9510565162951535312, 1.000000000000000000, 0.9510565162951535312, 1.000000000000000000, 0.9510565162951535312, 1.000000000000000000, 0.9510565162951535312, 1.000000000000000000, 0.9510565162951535312, 1.000000000000000000, 0.9510565162951535312, 1.000000000000000000, 0.9510565162951535312, 1.000000000000000000, 0.9510565162951535312, 1.000000000000000000, 0.9510565162951535312, 1.000000000000000000, 0.9510565162951535312, 1.000000000000000000, 0.9510565162951535312, 1.000000000000000000, 0.9510565162951535312, 1.000000000000000000, 0.9510565162951535312, 1.000000000000000000, 0.9510565162951535312, 1.000000000000000000, 0.9510565162951535312, 1.000000000000000000, 0.9510565162951535312, 1.000000000000000000, 0.9510565162951535312, 1.000000000000000000, 0.9510565162951535312, 1.000000000000000000, 0.9510565162951535312, 1.000000000000000000, 0.9510565162951535312, 1.000000000000000000, 0.9510565162951535312, 1.000000000000000000, 0.9510565162951535312, 1.000000000000000000, 0.9510565162951535312, 1.000000000000000000, 0.9510565162951535312, 1.000000000000000000, 0.9510565162951535312, 1.000000000000000000, 0.9510565162951535312, 1.000000000000000000, 0.9510565162951535312, 1.000000000000000000, 0.9510565162951535312, 1.000000000000000000, 0.9510565162951535312, 1.000000000000000000, 0.9510565162951535312, 1.000000000000000000, 0.9510565162951535312, 1.000000000000000000, 0.9510565162951535312, 1.000000000000000000, 0.9510565162951535312, 1.000000000000000000, 0.9510565162951535312, 1.000000000000000000, 0.9510565162951535312, 1.000000000000000000, 0.9510565162951535312, 1.000000000000000000, 0.9510565162951535312, 1.000000000000000000, 0.9510565162951535312, 1.000000000000000000, 0.9510565162951535312, 1.000000000000000000, 0.9510565162951535312, 1.000000000000000000, 0.9510565162951535312, 1.000000000000000000, 0.9510565162951535312, 1.000000000000000000, 0.9510565162951535312, 1.000000000000000000, 0.9510565162951535312, 1.000000000000000000, 0.9510565162951535312, 1.000000000000000000, 0.9510565162951535312, 1.000000000000000000, 0.9510565162951535312, 1.000000000000000000, 0.9510565162951535312, 1.000000000000000000, 0.9510565162951535312, 1.000000000000000000, 0.9510565162951535312, 1.000000000000000000, 0.9510565162951535312, 1.000000000000000000, 0.9510565162951535312, 1.000000000000000000, 0.9510565162951535312, 1.000000000000000000, 0.9510565162951535312, 1.000000000000000000, 0.9510565162951535312, 1.000000000000000000, 0.9510565162951535312, 1.000000000000000000, 0.9510565162951535312, 1.000000000000000000, 0.9510565162951535312, 1.000000000000000000, 0.9510565162951535312, 1.000000000000000000, 0.9510565162951535312, 1.000000000000000000, 0.9510565162951535312, 1.000000000000000000, 0.9510565162951535312, 1.000000000000000000, 0.9510565162951535312, 1.000000000000000000, 0.9510565162951535312, 1.000000000000000000, 0.9510565162951535312, 1.000000000000000000, 0.9510565162951535312, 1.000000000000000000, 0.9510565162951535312, 1.000000000000000000, 0.9510565162951535312, 1.000000000000000000, 0.9510565162951535312, 1.000000000000000000, 0.9510565162951535312, 1.000000000000000000, 0.9510565162951535312, 1.000000000000000000, 0.9510565162951535312, 1.000000000000000000, 0.9510565162951535312, 1.000000000000000000, 0.9510565162951535312, 1.000000000000000000, 0.9510565162951535312, 1.000000000000000000, 0.9510565162951535312, 1.000000000000000000, 0.9510565162951535312, 1.000000000000000000, 0.9510565162951535312, 1.000000000000000000, 0.9510565162951535312, 1.000000000000000000, 0.9510565162951535312, 1.000000000000000000, 0.9510565162951535312, 1.000000000000000000, 0.9510565162951535312, 1.000000000000000000, 0.9510565162951535312, 1.000000000000000000, 0.9510565162951535312, 1.000000000000000000, 0.9510565162951535312, 1.000000000000000000, 0.9510565162951535312, 1.000000000000000000, 0.9510565162951535312, 1.000000000000000000, 0.9510565162951535312, 1.000000000000000000, 0.9510565162951535312, 1.000000000000000000, 0.9510565162951535312, 1.000000000000000000, 0.9510565162951535312, 1.000000000000000000, 0.9510565162951535312, 1.000000000000000000, 0.9510565162951535312, 1.000000000000000000, 0.9510565162951535312, 1.000000000000000000, 0.9510565162951535312, 1.000000000000000000, 0.9510565162951535312, 1.000000000000000000, 0.9510565162951535312, 1.000000000000000000, 0.9510565162951535312, 1.000000000000000000, 0.9510565162951535312, 1.000000000000000000, 0.9510565162951535312, 1.000000000000000000, 0.9510565162951535312, 1.000000000000000000, 0.9510565162951535312, 1.000000000000000000, 0.9510565162951535312, 1.000000000000000000, 0.9510565162951535312, 1.000000000000000000, 0.9510565162951535312, 1.000000000000000000, 0.9510565162951535312, 1.000000000000000000, 0.9510565162951535312, 1.000000000000000000, 0.9510565162951535312, 1.000000000000000000, 0.9510565162951535312, 1.000000000000000000, 0.9510565162951535312, 1.000000000000000000, 0.9510565162951535312, 1.000000000000000000, 0.9510565162951535312, 1.000000000000000000, 0.9510565162951535312, 1.000000000000000000, 0.9510565162951535312, 1.000000000000000000, 0.9510565162951535312, 1.000000000000000000, 0.9510565162951535312, 1.000000000000000000, 0.9510565162951535312, 1.000000000000000000, 0.9510565162951535312, 1.000000000000000000, 0.9510565162951535312, 1.000000000000000000, 0.9510565162951535312, 1.000000000000000000, 0.9510565162951535312, 1.000000000000000000, 0.9510565162951535312, 1.000000000000000000, 0.9510565162951535312, 1.000000000000000000, 0.9510565162951535312, 1.000000000000000000, 0.9510565162951535312, 1.000000000000000000, 0.9510565162951535312, 1.000000000000000000, 0.9510565162951535312, 1.000000000000000000, 0.9510565162951535312, 1.000000000000000000, 0.9510565162951535312, 1.000000000000000000, 0.9510565162951535312, 1.000000000000000000, 0.9510565162951535312, 1.000000000000000000, 0.9510565162951535312, 1.000000000000000000, 0.9510565162951535312, 1.000000000000000000, 0.9510565162951535312, 1.000000000000000000, 0.9510565162951535312, 1.000000000000000000, 0.9510565162951535312, 1.000000000000000000, 0.9510565162951535312, 1.000000000000000000, 0.9510565162951535312, 1.000000000000000000, 0.9510565162951535312, 1.000000000000000000, 0.9510565162951535312, 1.000000000000000000, 0.9510565162951535312, 1.000000000000000000, 0.9510565162951535312, 1.000000000000000000, 0.9510565162951535312, 1.000000000000000000, 0.9510565162951535312, 1.000000000000000000, 0.9510565162951535312, 1.000000000000000000, 0.9510565162951535312, 1.000000000000000000, 0.9510565162951535312, 1.000000000000000000, 0.9510565162951535312, 1.000000000000000000, 0.9510565162951535312, 1.000000000000000000, 0.9510565162951535312, 1.000000000000000000, 0.9510565162951535312, 1.000000000000000000, 0.9510565162951535312, 1.000000000000000000, 0.9510565162951535312, 1.000000000000000000, 0.9510565162951535312, 1.000000000000000000, 0.9510565162951535312, 1.000000000000000000, 0.9510565162951535312, 1.000000000000000000, 0.9510565162951535312, 1.000000000000000000, 0.9510565162951535312, 1.000000000000000000, 0.9510565162951535312, 1.000000000000000000, 0.9510565162951535312, 1.000000000000000000, 0.9510565162951535312, 1.000000000000000000, 0.9510565162951535312, 1.000000000000000000, 0.9510565162951535312, 1.000000000000000000, 0.9510565162951535312, 1.000000000000000000, 0.9510565162951535312, 1.000000000000000000, 0.9510565162951535312, 1.000000000000000000, 0.9510565162951535312, 1.000000000000000000, 0.9510565162951535312, 1.000000000000000000, 0.9510565162951535312, 1.000000000000000000, 0.9510565162951535312, 1.000000000000000000, 0.9510565162951535312, 1.000000000000000000, 0.9510565162951535312, 1.000000000000000000, 0.9510565162951535312, 1.000000000000000000, 0.9510565162951535312, 1.000000000000000000, 0.9510565162951535312, 1.000000000000000000, 0.9510565162951535312, 1.000000000000000000, 0.9510565162951535312, 1.000000000000000000, 0.9510565162951535312, 1.000000000000000000, 0.9510565162951535312, 1.000000000000000000, 0.9510565162951535312, 1.000000000000000000, 0.9510565162951535312, 1.000000000000000000, 0.9510565162951535312, 1.000000000000000000, 0.9510565162951535312, 1.000000000000000000, 0.9510565162951535312, 1.000000000000000000, 0.9510565162951535312, 1.000000000000000000, 0.9510565162951535312, 1.000000000000000000, 0.9510565162951535312, 1.000000000000000000, 0.9510565162951535312, 1.000000000000000000, 0.9510565162951535312, 1.000000000000000000, 0.9510565162951535312, 1.000000000000000000, 0.9510565162951535312, 1.000000000000000000, 0.9510565162951535312, 1.000000000000000000, 0.9510565162951535312, 1.000000000000000000, 0.9510565162951535312, 1.000000000000000000, 0.9510565162951535312, 1.000000000000000000, 0.9510565162951535312, 1.000000000000000000, 0.9510565162951535312, 1.000000000000000000, 0.9510565162951535312, 1.000000000000000000, 0.9510565162951535312, 1.000000000000000000, 0.9510565162951535312, 1.000000000000000000, 0.9510565162951535312, 1.000000000000000000, 0.9510565162951535312, 1.000000000000000000, 0.9510565162951535312, 1.000000000000000000, 0.9510565162951535312, 1.000000000000000000, 0.9510565162951535312, 1.000000000000000000, 0.9510565162951535312, 1.000000000000000000, 0.9510565162951535312, 1.000000000000000000, 0.9510565162951535312, 1.000000000000000000, 0.9510565162951535312, 1.000000000000000000, 0.9510565162951535312, 1.000000000000000000, 0.9510565162951535312, 1.000000000000000000, 0.9510565162951535312, 1.000000000000000000, 0.9510565162951535312, 1.000000000000000000, 0.9510565162951535312, 1.000000000000000000, 0.9510565162951535312, 1.000000000000000000, 0.9510565162951535312, 1.000000000000000000, 0.9510565162951535312, 1.000000000000000000, 0.9510565162951535312, 1.000000000000000000, 0.9510565162951535312, 1.000000000000000000, 0.9510565162951535312, 1.000000000000000000, 0.9510565162951535312, 1.000000000000000000, 0.9510565162951535312, 1.000000000000000000, 0.9510565162951535312, 1.000000000000000000, 0.9510565162951535312, 1.000000000000000000, 0.9510565162951535312, 1.000000000000000000, 0.9510565162951535312, 1.000000000000000000, 0.9510565162951535312, 1.000000000000000000, 0.9510565162951535312, 1.000000000000000000, 0.9510565162951535312, 1.000000000000000000, 0.9510565162951535312, 1.000000000000000000, 0.9510565162951535312, 1.000000000000000000, 0.9510565162951535312, 1.000000000000000000, 0.9510565162951535312, 1.000000000000000000, 0.9510565162951535312, 1.000000000000000000, 0.9510565162951535312, 1.000000000000000000, 0.9510565162951535312, 1.000000000000000000, 0.9510565162951535312, 1.000000000000000000, 0.9510565162951535312, 1.000000000000000000, 0.9510565162951535312, 1.000000000000000000, 0.9510565162951535312, 1.000000000000000000, 0.9510565162951535312, 1.000000000000000000, 0.9510565162951535312, 1.000000000000000000, 0.9510565162951535312, 1.000000000000000000, 0.9510565162951535312, 1.000000000000000000, 0.9510565162951535312, 1.000000000000000000, 0.9510565162951535312, 1.000000000000000000, 0.9510565162951535312, 1.000000000000000000, 0.9510565162951535312, 1.000000000000000000, 0.9510565162951535312, 1.000000000000000000, 0.9510565162951535312, 1.000000000000000000, 0.9510565162951535312, 1.000000000000000000, 0.9510565162951535312, 1.000000000000000000, 0.9510565162951535312, 1.000000000000000000),
 ( 1.000000000000000000, 0.9510565162951535312, 1.000000000000000000, 0.9510565162951535312, 1.000000000000000000, 0.9510565162951535312, 1.000000000000000000, 0.9510565162951535312, 1.000000000000000000, 0.9510565162951535312, 1.000000000000000000, 0.9510565162951535312, 1.000000000000000000, 0.9510565162951535312, 1.000000000000000000, 0.9510565162951535312, 1.000000000000000000, 0.9510565162951535312, 1.000000000000000000, 0.9510565162951535312, 1.000000000000000000, 0.9510565162951535312, 1.000000000000000000, 0.9510565162951535312, 1.000000000000000000, 0.9510565162951535312, 1.000000000000000000, 0.9510565162951535312, 1.000000000000000000, 0.9510565162951535312, 1.000000000000000000, 0.9510565162951535312, 1.000000000000000000, 0.9510565162951535312, 1.000000000000000000, 0.9510565162951535312, 1.000000000000000000, 0.9510565162951535312, 1.000000000000000000, 0.9510565162951535312, 1.000000000000000000, 0.9510565162951535312, 1.000000000000000000, 0.9510565162951535312, 1.000000000000000000, 0.9510565162951535312, 1.000000000000000000, 0.9510565162951535312, 1.000000000000000000, 0.9510565162951535312, 1.000000000000000000, 0.9510565162951535312, 1.000000000000000000, 0.9510565162951535312, 1.000000000000000000, 0.9510565162951535312, 1.000000000000000000, 0.9510565162951535312, 1.000000000000000000, 0.9510565162951535312, 1.000000000000000000, 0.9510565162951535312, 1.000000000000000000, 0.9510565162951535312, 1.000000000000000000, 0.9510565162951535312, 1.000000000000000000, 0.9510565162951535312, 1.000000000000000000, 0.9510565162951535312, 1.000000000000000000, 0.9510565162951535312, 1.000000000000000000, 0.9510565162951535312, 1.000000000000000000, 0.9510565162951535312, 1.000000000000000000, 0.9510565162951535312, 1.000000000000000000, 0.9510565162951535312, 1.000000000000000000, 0.9510565162951535312, 1.000000000000000000, 0.9510565162951535312, 1.000000000000000000, 0.9510565162951535312, 1.000000000000000000, 0.9510565162951535312, 1.000000000000000000, 0.9510565162951535312, 1.000000000000000000, 0.9510565162951535312, 1.000000000000000000, 0.9510565162951535312, 1.000000000000000000, 0.9510565162951535312, 1.000000000000000000, 0.9510565162951535312, 1.000000000000000000, 0.9510565162951535312, 1.000000000000000000, 0.9510565162951535312, 1.000000000000000000, 0.9510565162951535312, 1.000000000000000000, 0.9510565162951535312, 1.000000000000000000, 0.9510565162951535312, 1.000000000000000000, 0.9510565162951535312, 1.000000000000000000, 0.9510565162951535312, 1.000000000000000000, 0.9510565162951535312, 1.000000000000000000, 0.9510565162951535312, 1.000000000000000000, 0.9510565162951535312, 1.000000000000000000, 0.9510565162951535312, 1.000000000000000000, 0.9510565162951535312, 1.000000000000000000, 0.9510565162951535312, 1.000000000000000000, 0.9510565162951535312, 1.000000000000000000, 0.9510565162951535312, 1.000000000000000000, 0.9510565162951535312, 1.000000000000000000, 0.9510565162951535312, 1.000000000000000000, 0.9510565162951535312, 1.000000000000000000, 0.9510565162951535312, 1.000000000000000000, 0.9510565162951535312, 1.000000000000000000, 0.9510565162951535312, 1.000000000000000000, 0.9510565162951535312, 1.000000000000000000, 0.9510565162951535312, 1.000000000000000000, 0.9510565162951535312, 1.000000000000000000, 0.9510565162951535312, 1.000000000000000000, 0.9510565162951535312, 1.000000000000000000, 0.9510565162951535312, 1.000000000000000000, 0.9510565162951535312, 1.000000000000000000, 0.9510565162951535312, 1.000000000000000000, 0.9510565162951535312, 1.000000000000000000, 0.9510565162951535312, 1.000000000000000000, 0.9510565162951535312, 1.000000000000000000, 0.9510565162951535312, 1.000000000000000000, 0.9510565162951535312, 1.000000000000000000, 0.9510565162951535312, 1.000000000000000000, 0.9510565162951535312, 1.000000000000000000, 0.9510565162951535312, 1.000000000000000000, 0.9510565162951535312, 1.000000000000000000, 0.9510565162951535312, 1.000000000000000000, 0.9510565162951535312, 1.000000000000000000, 0.9510565162951535312, 1.000000000000000000, 0.9510565162951535312, 1.000000000000000000, 0.9510565162951535312, 1.000000000000000000, 0.9510565162951535312, 1.000000000000000000, 0.9510565162951535312, 1.000000000000000000, 0.9510565162951535312, 1.000000000000000000, 0.9510565162951535312, 1.000000000000000000, 0.9510565162951535312, 1.000000000000000000, 0.9510565162951535312, 1.000000000000000000, 0.9510565162951535312, 1.000000000000000000, 0.9510565162951535312, 1.000000000000000000, 0.9510565162951535312, 1.000000000000000000, 0.9510565162951535312, 1.000000000000000000, 0.9510565162951535312, 1.000000000000000000, 0.9510565162951535312, 1.000000000000000000, 0.9510565162951535312, 1.000000000000000000, 0.9510565162951535312, 1.000000000000000000, 0.9510565162951535312, 1.000000000000000000, 0.9510565162951535312, 1.000000000000000000, 0.9510565162951535312, 1.000000000000000000, 0.9510565162951535312, 1.000000000000000000, 0.9510565162951535312, 1.000000000000000000, 0.9510565162951535312, 1.000000000000000000, 0.9510565162951535312, 1.000000000000000000, 0.9510565162951535312, 1.000000000000000000, 0.9510565162951535312, 1.000000000000000000, 0.9510565162951535312, 1.000000000000000000, 0.9510565162951535312, 1.000000000000000000, 0.9510565162951535312, 1.000000000000000000, 0.9510565162951535312, 1.000000000000000000, 0.9510565162951535312, 1.000000000000000000, 0.9510565162951535312, 1.000000000000000000, 0.9510565162951535312, 1.000000000000000000, 0.9510565162951535312, 1.000000000000000000, 0.9510565162951535312, 1.000000000000000000, 0.9510565162951535312, 1.000000000000000000, 0.9510565162951535312, 1.000000000000000000, 0.9510565162951535312, 1.000000000000000000, 0.9510565162951535312, 1.000000000000000000, 0.9510565162951535312, 1.000000000000000000, 0.9510565162951535312, 1.000000000000000000, 0.9510565162951535312, 1.000000000000000000, 0.9510565162951535312, 1.000000000000000000, 0.9510565162951535312, 1.000000000000000000, 0.9510565162951535312, 1.000000000000000000, 0.9510565162951535312, 1.000000000000000000, 0.9510565162951535312, 1.000000000000000000, 0.9510565162951535312, 1.000000000000000000, 0.9510565162951535312, 1.000000000000000000, 0.9510565162951535312, 1.000000000000000000, 0.9510565162951535312, 1.000000000000000000, 0.9510565162951535312, 1.000000000000000000, 0.9510565162951535312, 1.000000000000000000, 0.9510565162951535312, 1.000000000000000000, 0.9510565162951535312, 1.000000000000000000, 0.9510565162951535312, 1.000000000000000000, 0.9510565162951535312, 1.000000000000000000, 0.9510565162951535312, 1.000000000000000000, 0.9510565162951535312, 1.000000000000000000, 0.9510565162951535312, 1.000000000000000000, 0.9510565162951535312, 1.000000000000000000, 0.9510565162951535312, 1.000000000000000000, 0.9510565162951535312, 1.000000000000000000, 0.9510565162951535312, 1.000000000000000000, 0.9510565162951535312, 1.000000000000000000, 0.9510565162951535312, 1.000000000000000000, 0.9510565162951535312, 1.000000000000000000, 0.9510565162951535312, 1.000000000000000000, 0.9510565162951535312, 1.000000000000000000, 0.9510565162951535312, 1.000000000000000000, 0.9510565162951535312, 1.000000000000000000, 0.9510565162951535312, 1.000000000000000000, 0.9510565162951535312, 1.000000000000000000, 0.9510565162951535312, 1.000000000000000000, 0.9510565162951535312, 1.000000000000000000, 0.9510565162951535312, 1.000000000000000000, 0.9510565162951535312, 1.000000000000000000, 0.9510565162951535312, 1.000000000000000000, 0.9510565162951535312, 1.000000000000000000, 0.9510565162951535312, 1.000000000000000000, 0.9510565162951535312, 1.000000000000000000, 0.9510565162951535312, 1.000000000000000000, 0.9510565162951535312, 1.000000000000000000, 0.9510565162951535312, 1.000000000000000000, 0.9510565162951535312, 1.000000000000000000, 0.9510565162951535312, 1.000000000000000000, 0.9510565162951535312, 1.000000000000000000, 0.9510565162951535312, 1.000000000000000000, 0.9510565162951535312, 1.000000000000000000, 0.9510565162951535312, 1.000000000000000000, 0.9510565162951535312, 1.000000000000000000, 0.9510565162951535312, 1.000000000000000000, 0.9510565162951535312, 1.000000000000000000, 0.9510565162951535312, 1.000000000000000000, 0.9510565162951535312, 1.000000000000000000, 0.9510565162951535312, 1.000000000000000000, 0.9510565162951535312, 1.000000000000000000, 0.9510565162951535312, 1.000000000000000000, 0.9510565162951535312, 1.000000000000000000, 0.9510565162951535312, 1.000000000000000000, 0.9510565162951535312, 1.000000000000000000, 0.9510565162951535312, 1.000000000000000000, 0.9510565162951535312, 1.000000000000000000, 0.9510565162951535312, 1.000000000000000000, 0.9510565162951535312, 1.000000000000000000, 0.9510565162951535312, 1.000000000000000000, 0.9510565162951535312, 1.000000000000000000, 0.9510565162951535312, 1.000000000000000000, 0.9510565162951535312, 1.000000000000000000, 0.9510565162951535312, 1.000000000000000000, 0.9510565162951535312, 1.000000000000000000, 0.9510565162951535312, 1.000000000000000000, 0.9510565162951535312, 1.000000000000000000, 0.9510565162951535312, 1.000000000000000000, 0.9510565162951535312, 1.000000000000000000, 0.9510565162951535312, 1.000000000000000000, 0.9510565162951535312, 1.000000000000000000, 0.9510565162951535312, 1.000000000000000000, 0.9510565162951535312, 1.000000000000000000, 0.9510565162951535312, 1.000000000000000000, 0.9510565162951535312, 1.000000000000000000, 0.9510565162951535312, 1.000000000000000000, 0.9510565162951535312, 1.000000000000000000, 0.9510565162951535312, 1.000000000000000000, 0.9510565162951535312, 1.000000000000000000, 0.9510565162951535312, 1.000000000000000000, 0.9510565162951535312, 1.000000000000000000, 0.9510565162951535312, 1.000000000000000000, 0.9510565162951535312, 1.000000000000000000, 0.9510565162951535312, 1.000000000000000000, 0.9510565162951535312, 1.000000000000000000, 0.9510565162951535312, 1.000000000000000000, 0.9510565162951535312, 1.000000000000000000, 0.9510565162951535312, 1.000000000000000000, 0.9510565162951535312, 1.000000000000000000, 0.9510565162951535312, 1.000000000000000000, 0.9510565162951535312, 1.000000000000000000, 0.9510565162951535312, 1.000000000000000000, 0.9510565162951535312, 1.000000000000000000, 0.9510565162951535312, 1.000000000000000000, 0.9510565162951535312, 1.000000000000000000, 0.9510565162951535312, 1.000000000000000000, 0.9510565162951535312, 1.000000000000000000, 0.9510565162951535312, 1.000000000000000000, 0.9510565162951535312, 1.000000000000000000, 0.9510565162951535312, 1.000000000000000000, 0.9510565162951535312, 1.000000000000000000, 0.9510565162951535312, 1.000000000000000000, 0.9510565162951535312, 1.000000000000000000, 0.9510565162951535312, 1.000000000000000000, 0.9510565162951535312, 1.000000000000000000, 0.9510565162951535312, 1.000000000000000000, 0.9510565162951535312, 1.000000000000000000, 0.9510565162951535312, 1.000000000000000000, 0.9510565162951535312, 1.000000000000000000, 0.9510565162951535312, 1.000000000000000000, 0.9510565162951535312, 1.000000000000000000, 0.9510565162951535312, 1.000000000000000000, 0.9510565162951535312, 1.000000000000000000, 0.9510565162951535312, 1.000000000000000000, 0.9510565162951535312, 1.000000000000000000, 0.9510565162951535312, 1.000000000000000000, 0.9510565162951535312, 1.000000000000000000, 0.9510565162951535312, 1.000000000000000000, 0.9510565162951535312, 1.000000000000000000, 0.9510565162951535312, 1.000000000000000000, 0.9510565162951535312, 1.000000000000000000, 0.9510565162951535312, 1.000000000000000000, 0.9510565162951535312, 1.000000000000000000, 0.9510565162951535312, 1.000000000000000000, 0.9510565162951535312, 1.000000000000000000, 0.9510565162951535312, 1.000000000000000000, 0.9510565162951535312, 1.000000000000000000, 0.9510565162951535312, 1.000000000000000000, 0.9510565162951535312, 1.000000000000000000, 0.9510565162951535312, 1.000000000000000000, 0.9510565162951535312, 1.000000000000000000, 0.9510565162951535312, 1.000000000000000000, 0.9510565162951535312, 1.000000000000000000, 0.9510565162951535312, 1.000000000000000000, 0.9510565162951535312, 1.000000000000000000, 0.9510565162951535312, 1.000000000000000000, 0.9510565162951535312, 1.000000000000000000, 0.9510565162951535312, 1.000000000000000000, 0.9510565162951535312, 1.000000000000000000, 0.9510565162951535312, 1.000000000000000000, 0.9510565162951535312, 1.000000000000000000, 0.9510565162951535312, 1.000000000000000000, 0.9510565162951535312, 1.000000000000000000, 0.9510565162951535312, 1.000000000000000000, 0.9510565162951535312, 1.000000000000000000, 0.9510565162951535312, 1.000000000000000000, 0.9510565162951535312, 1.000000000000000000, 0.9510565162951535312, 1.000000000000000000, 0.9510565162951535312, 1.000000000000000000, 0.9510565162951535312, 1.000000000000000000, 0.9510565162951535312, 1.000000000000000000, 0.9510565162951535312, 1.000000000000000000, 0.9510565162951535312, 1.000000000000000000, 0.9510565162951535312, 1.000000000000000000, 0.9510565162951535312, 1.000000000000000000, 0.9510565162951535312, 1.000000000000000000, 0.9510565162951535312, 1.000000000000000000, 0.9510565162951535312, 1.000000000000000000, 0.9510565162951535312, 1.000000000000000000, 0.9510565162951535312, 1.000000000000000000, 0.9510565162951535312, 1.000000000000000000, 0.9510565162951535312, 1.000000000000000000, 0.9510565162951535312, 1.000000000000000000, 0.9510565162951535312, 1.000000000000000000, 0.9510565162951535312, 1.000000000000000000, 0.9510565162951535312, 1.000000000000000000, 0.9510565162951535312, 1.000000000000000000, 0.9510565162951535312, 1.000000000000000000, 0.9510565162951535312, 1.000000000000000000, 0.9510565162951535312, 1.000000000000000000, 0.9510565162951535312, 1.000000000000000000, 0.9510565162951535312, 1.000000000000000000, 0.9510565162951535312, 1.000000000000000000, 0.9510565162951535312, 1.000000000000000000, 0.9510565162951535312, 1.000000000000000000, 0.9510565162951535312, 1.000000000000000000, 0.9510565162951535312, 1.000000000000000000, 0.9510565162951535312, 1.000000000000000000, 0.9510565162951535312, 1.000000000000000000, 0.9510565162951535312, 1.000000000000000000, 0.9510565162951535312, 1.000000000000000000, 0.9510565162951535312, 1.000000000000000000, 0.9510565162951535312, 1.000000000000000000, 0.9510565162951535312, 1.000000000000000000, 0.9510565162951535312, 1.000000000000000000, 0.9510565162951535312, 1.000000000000000000, 0.9510565162951535312, 1.000000000000000000, 0.9510565162951535312, 1.000000000000000000, 0.9510565162951535312, 1.000000000000000000, 0.9510565162951535312, 1.000000000000000000, 0.9510565162951535312, 1.000000000000000000, 0.9510565162951535312, 1.000000000000000000, 0.9510565162951535312, 1.000000000000000000, 0.9510565162951535312, 1.000000000000000000, 0.9510565162951535312, 1.000000000000000000, 0.9510565162951535312, 1.000000000000000000, 0.9510565162951535312, 1.000000000000000000, 0.9510565162951535312, 1.000000000000000000, 0.9510565162951535312, 1.000000000000000000, 0.9510565162951535312, 1.000000000000000000, 0.9510565162951535312, 1.000000000000000000, 0.9510565162951535312, 1.000000000000000000, 0.9510565162951535312, 1.000000000000000000, 0.9510565162951535312, 1.000000000000000000, 0.9510565162951535312, 1.000000000000000000, 0.9510565162951535312, 1.000000000000000000, 0.9510565162951535312, 1.000000000000000000, 0.9510565162951535312, 1.000000000000000000, 0.9510565162951535312, 1.000000000000000000, 0.9510565162951535312, 1.000000000000000000, 0.9510565162951535312, 1.000000000000000000, 0.9510565162951535312, 1.000000000000000000, 0.9510565162951535312, 1.000000000000000000, 0.9510565162951535312, 1.000000000000000000, 0.9510565162951535312, 1.000000000000000000, 0.9510565162951535312, 1.000000000000000000, 0.9510565162951535312, 1.000000000000000000, 0.9510565162951535312, 1.000000000000000000, 0.9510565162951535312, 1.000000000000000000, 0.9510565162951535312, 1.000000000000000000, 0.9510565162951535312, 1.000000000000000000, 0.9510565162951535312, 1.000000000000000000, 0.9510565162951535312, 1.000000000000000000, 0.9510565162951535312, 1.000000000000000000, 0.9510565162951535312, 1.000000000000000000, 0.9510565162951535312, 1.000000000000000000, 0.9510565162951535312, 1.000000000000000000, 0.9510565162951535312, 1.000000000000000000, 0.9510565162951535312, 1.000000000000000000, 0.9510565162951535312, 1.000000000000000000, 0.9510565162951535312, 1.000000000000000000, 0.9510565162951535312, 1.000000000000000000, 0.9510565162951535312, 1.000000000000000000, 0.9510565162951535312, 1.000000000000000000, 0.9510565162951535312, 1.000000000000000000, 0.9510565162951535312, 1.000000000000000000, 0.9510565162951535312, 1.000000000000000000, 0.9510565162951535312, 1.000000000000000000, 0.9510565162951535312, 1.000000000000000000, 0.9510565162951535312, 1.000000000000000000, 0.9510565162951535312, 1.000000000000000000, 0.9510565162951535312, 1.000000000000000000, 0.9510565162951535312, 1.000000000000000000, 0.9510565162951535312, 1.000000000000000000, 0.9510565162951535312, 1.000000000000000000, 0.9510565162951535312, 1.000000000000000000, 0.9510565162951535312, 1.000000000000000000, 0.9510565162951535312, 1.000000000000000000, 0.9510565162951535312, 1.000000000000000000, 0.9510565162951535312, 1.000000000000000000, 0.9510565162951535312, 1.000000000000000000, 0.9510565162951535312, 1.000000000000000000, 0.9510565162951535312, 1.000000000000000000, 0.9510565162951535312, 1.000000000000000000, 0.9510565162951535312, 1.000000000000000000) ) ) 
 REPRESENTATION_ITEM ( '' )  SURFACE ( )  );
#32619=PLANE ( 'NONE',  #21014 ) ;
#32623=CARTESIAN_POINT ( 'NONE',  ( -3.880418787951142701, 5.198745712990781698, 24.49999999999999645 ) ) ;
#32624=EDGE_LOOP ( 'NONE', ( #538, #22941, #22364, #9850 ) ) ;
#32628=ORIENTED_EDGE ( 'NONE', *, *, #15361, .T. ) ;
#32629=EDGE_CURVE ( 'NONE', #5219, #1686, #25817, .T. ) ;
#32630=EDGE_CURVE ( 'NONE', #28636, #22217, #2363, .T. ) ;
#32633=ORIENTED_EDGE ( 'NONE', *, *, #5798, .T. ) ;
#32635=CARTESIAN_POINT ( 'NONE',  ( 20.75514604977249178, 49.82500000273117990, 28.56700777964553950 ) ) ;
#32637=CARTESIAN_POINT ( 'NONE',  ( -10.04305231718578462, 10.90000000546237402, 30.90933677959249337 ) ) ;
#32639=CARTESIAN_POINT ( 'NONE',  ( 23.41746824999999887, 15.22499999726880482, -7.608796670333727974 ) ) ;
#32640=CARTESIAN_POINT ( 'NONE',  ( -10.04305231718579172, 55.59999999999998010, -30.90933677959248982 ) ) ;
#32641=CARTESIAN_POINT ( 'NONE',  ( -27.16883889988623935, 23.57500000273119056, 19.73931689729374739 ) ) ;
#32644=CARTESIAN_POINT ( 'NONE',  ( 4.300734207923757602, 72.27500000273117564, -13.23629886949340673 ) ) ;
#32645=CARTESIAN_POINT ( 'NONE',  ( -8.891200544363830713E-16, 77.75000000546236834, -15.00000000000000000 ) ) ;
#32648=EDGE_LOOP ( 'NONE', ( #22465, #32542, #18658, #24784 ) ) ;
#32655=CARTESIAN_POINT ( 'NONE',  ( 20.75514604977248467, 8.675000002731195536, -28.56700777964554305 ) ) ;
#32659=CARTESIAN_POINT ( 'NONE',  ( -8.601468415847518756, 79.07500000273121543, -11.83890561707634603 ) ) ;
#32662=CARTESIAN_POINT ( 'NONE',  ( 10.37757302488624056, 50.52500000273118985, -31.93888565452638417 ) ) ;
#32664=ORIENTED_EDGE ( 'NONE', *, *, #21544, .T. ) ;
#32666=LINE ( 'NONE', #4190, #33829 ) ;
#32667=CARTESIAN_POINT ( 'NONE',  ( 18.94512977948576093, 14.82499999726882933, -13.76444248337722875 ) ) ;
#32669=EDGE_LOOP ( 'NONE', ( #17799, #24762, #10245, #14873 ) ) ;
#32673=CARTESIAN_POINT ( 'NONE',  ( -10.37757302488624411, 62.97500000273120691, -31.93888565452638417 ) ) ;
#32675=CARTESIAN_POINT ( 'NONE',  ( -20.75514604977248823, 76.82500000273120122, -28.56700777964554305 ) ) ;
#32677=CARTESIAN_POINT ( 'NONE',  ( 15.14183272437242245, 4.300000000000009592, -20.84094480462497856 ) ) ;
#32678=FACE_OUTER_BOUND ( 'NONE', #31981, .T. ) ;
#32679=ADVANCED_FACE ( 'NONE', ( #5297 ), #7697, .T. ) ;
#32680=CARTESIAN_POINT ( 'NONE',  ( 33.58253175000000113, 14.12500000273120193, -4.112674001490185761E-15 ) ) ;
#32681=CARTESIAN_POINT ( 'NONE',  ( 8.601468415847520532, 71.57500000273118701, 11.83890561707634603 ) ) ;
#32683=CARTESIAN_POINT ( 'NONE',  ( -4.635254915624211769, 79.60000000000000853, -14.26584774442730286 ) ) ;
#32685=CARTESIAN_POINT ( 'NONE',  ( -15.14183272437242067, 8.449999994537638059, -20.84094480462497856 ) ) ;
#32687=CARTESIAN_POINT ( 'NONE',  ( -4.635254915624208216, 76.65000000546237402, 14.26584774442730463 ) ) ;
#32689=CARTESIAN_POINT ( 'NONE',  ( 10.37757302488624767, 35.72500000273118559, 31.93888565452638417 ) ) ;
#32692=CARTESIAN_POINT ( 'NONE',  ( -10.37757302488623701, 27.77500000273119696, 31.93888565452638417 ) ) ;
#32695=CARTESIAN_POINT ( 'NONE',  ( -26.29305231718578995, 18.19999999999999574, 19.10302069950538595 ) ) ;
#32698=CARTESIAN_POINT ( 'NONE',  ( 18.94512977948575738, 8.424999997268811214, 13.76444248337723408 ) ) ;
#32702=CARTESIAN_POINT ( 'NONE',  ( -20.75514604977248823, 12.82500000273118168, -28.56700777964554305 ) ) ;
#32703=CARTESIAN_POINT ( 'NONE',  ( -23.41746824999999887, 6.124999997268814944, -2.867812753649727150E-15 ) ) ;
#32705=ORIENTED_EDGE ( 'NONE', *, *, #19118, .T. ) ;
#32711=CARTESIAN_POINT ( 'NONE',  ( -5.147494310547423346, 72.94874572391552192, 32.50000000000000000 ) ) ;
#32712=CARTESIAN_POINT ( 'NONE',  ( 24.50000000000000355, 17.84999999453763309, -7.960532557706203605 ) ) ;
#32713=CARTESIAN_POINT ( 'NONE',  ( 18.94512977948576093, 4.824999997268819563, -13.76444248337722875 ) ) ;
#32714=CARTESIAN_POINT ( 'NONE',  ( -33.58253175000000113, 23.37500000273118417, 0.000000000000000000 ) ) ;
#32715=CARTESIAN_POINT ( 'NONE',  ( -10.04305231718578462, 22.90000000546238468, 30.90933677959249337 ) ) ;
#32716=EDGE_CURVE ( 'NONE', #29542, #3689, #17707, .T. ) ;
#32717=CARTESIAN_POINT ( 'NONE',  ( 20.08610463437157279, 75.30000000000001137, -27.64615127144129758 ) ) ;
#32718=CARTESIAN_POINT ( 'NONE',  ( -1.778240108872766143E-15, 48.00000000546238255, -32.49999999999999289 ) ) ;
#32721=CARTESIAN_POINT ( 'NONE',  ( -33.58253175000000113, 37.37500000273119838, 0.000000000000000000 ) ) ;
#32725=EDGE_CURVE ( 'NONE', #32333, #5219, #5677, .T. ) ;
#32726=VECTOR ( 'NONE', #20603, 1000.000000000000000 ) ;
#32727=CARTESIAN_POINT ( 'NONE',  ( 14.47279130897151767, 11.42499999726880944, -19.92008829642072598 ) ) ;
#32728=CARTESIAN_POINT ( 'NONE',  ( -20.08610463437157989, 15.69999999999999929, -27.64615127144129758 ) ) ;
#32731=CARTESIAN_POINT ( 'NONE',  ( -33.58253175000000113, 57.02500000273118275, -10.91162601494193218 ) ) ;
#32732=CARTESIAN_POINT ( 'NONE',  ( -33.58253175000000113, 49.37500000273120548, 0.000000000000000000 ) ) ;
#32734=CARTESIAN_POINT ( 'NONE',  ( 0.000000000000000000, 80.00000000000001421, -32.50000000000000000 ) ) ;
#32735=CARTESIAN_POINT ( 'NONE',  ( -32.50000000000000000, 6.099999999999980993, 10.55989012756946366 ) ) ;
#32738=DIRECTION ( 'NONE',  ( 0.000000000000000000, 0.000000000000000000, -1.000000000000000000 ) ) ;
#32740=DIRECTION ( 'NONE',  ( 0.000000000000000000, 0.000000000000000000, -1.000000000000000000 ) ) ;
#32742=CARTESIAN_POINT ( 'NONE',  ( -4.223320258572819786E-15, 13.50000000000000355, 24.50000000000000000 ) ) ;
#32745=CARTESIAN_POINT ( 'NONE',  ( 32.50000000000000000, 11.09999999999999787, -10.55989012756945833 ) ) ;
#32746=CARTESIAN_POINT ( 'NONE',  ( -27.16883889988623935, 35.32500000273120122, 19.73931689729374739 ) ) ;
#32748=EDGE_LOOP ( 'NONE', ( #30519, #19982, #8671, #3363 ) ) ;
#32753=EDGE_LOOP ( 'NONE', ( #14790, #4108 ) ) ;
#32757=CARTESIAN_POINT ( 'NONE',  ( 5.779280353836490358E-15, 20.49999999999999645, 32.49999999999999289 ) ) ;
#32758=CARTESIAN_POINT ( 'NONE',  ( 33.58253175000000113, 40.37500000273119838, -4.112674001490185761E-15 ) ) ;
#32759=CARTESIAN_POINT ( 'NONE',  ( 32.50000000000000000, 47.60000000546239818, -10.55989012756945833 ) ) ;
#32761=CARTESIAN_POINT ( 'NONE',  ( 33.58253175000000113, 28.12500000273118772, -4.112674001490185761E-15 ) ) ;
#32762=CARTESIAN_POINT ( 'NONE',  ( -33.58253175000000113, 57.27500000273120406, -10.91162601494193218 ) ) ;
#32763=SURFACE_SIDE_STYLE ('',( #16498 ) ) ;
#32764=EDGE_CURVE ( 'NONE', #19947, #33131, #5634, .T. ) ;
#32766=CARTESIAN_POINT ( 'NONE',  ( -20.08610463437157989, 33.70000000000001705, -27.64615127144129758 ) ) ;
#32768=CARTESIAN_POINT ( 'NONE',  ( -33.58253175000000113, 77.02500000273118985, -10.91162601494193218 ) ) ;
#32771=CARTESIAN_POINT ( 'NONE',  ( -27.16883889988624290, 65.17500000273118133, -19.73931689729374028 ) ) ;
#32773=LINE ( 'NONE', #12364, #2978 ) ;
#32774=CARTESIAN_POINT ( 'NONE',  ( 19.82091636218621034, 3.549999994537617276, 14.40073868116559730 ) ) ;
#32788=CARTESIAN_POINT ( 'NONE',  ( -7.570916362186210335, 4.349999994537640191, -23.30088464923126779 ) ) ;
#32789=ORIENTED_EDGE ( 'NONE', *, *, #4651, .T. ) ;
#32796=CARTESIAN_POINT ( 'NONE',  ( -26.29305231718579350, 74.30000000546237970, -19.10302069950537884 ) ) ;
#32797=CARTESIAN_POINT ( 'NONE',  ( -2.162160676586881955E-15, 48.62500000273118417, -35.31076352940723240 ) ) ;
#32799=CARTESIAN_POINT ( 'NONE',  ( 26.29305231718578995, 13.70000000546239782, -19.10302069950538240 ) ) ;
#32801=CARTESIAN_POINT ( 'NONE',  ( -14.47279130897152299, 16.42499999726882720, 19.92008829642072243 ) ) ;
#32802=CARTESIAN_POINT ( 'NONE',  ( 20.08610463437158344, 54.69999999999998863, 27.64615127144129403 ) ) ;
#32803=LINE ( 'NONE', #9296, #32909 ) ;
#32804=CARTESIAN_POINT ( 'NONE',  ( 10.37757302488624767, 17.97500000273119625, 31.93888565452638417 ) ) ;
#32805=CARTESIAN_POINT ( 'NONE',  ( 5.779280353836490358E-15, 5.000000005462372776, 32.49999999999999289 ) ) ;
#32807=CARTESIAN_POINT ( 'NONE',  ( 13.91746824999999532, 71.97500000273120691, -4.522059556121118540 ) ) ;
#32808=CARTESIAN_POINT ( 'NONE',  ( 15.00000000000000000, 75.25000000546239676, -1.836970198721029589E-15 ) ) ;
#32811=ORIENTED_EDGE ( 'NONE', *, *, #24665, .T. ) ;
#32813=CARTESIAN_POINT ( 'NONE',  ( -1.778240108872766143E-15, 40.00000000546237544, -32.49999999999999289 ) ) ;
#32819=CARTESIAN_POINT ( 'NONE',  ( -20.75514604977248112, 9.675000002731193760, 28.56700777964554661 ) ) ;
#32823=CARTESIAN_POINT ( 'NONE',  ( 5.147494310547426899, 3.448745718453164244, -32.50000000000000000 ) ) ;
#32826=CARTESIAN_POINT ( 'NONE',  ( 6.486482029760648627E-15, 51.62500000273120548, 35.31076352940722529 ) ) ;
#32828=EDGE_CURVE ( 'NONE', #9459, #29733, #11572, .T. ) ;
#32831=CARTESIAN_POINT ( 'NONE',  ( 5.779280353836490358E-15, 18.50000000000000000, 32.49999999999999289 ) ) ;
#32832=CARTESIAN_POINT ( 'NONE',  ( 23.41746825000000243, 14.72499999726881903, -7.608796670333727974 ) ) ;
#32837=ORIENTED_EDGE ( 'NONE', *, *, #25382, .T. ) ;
#32839=CARTESIAN_POINT ( 'NONE',  ( -33.58253175000000113, 57.47500000273119269, 10.91162601494193929 ) ) ;
#32841=CARTESIAN_POINT ( 'NONE',  ( -10.37757302488624411, 66.72500000273117848, -31.93888565452638417 ) ) ;
#32843=CARTESIAN_POINT ( 'NONE',  ( 24.50000000000000355, 9.900000000000007461, 7.960532557706212486 ) ) ;
#32844=CARTESIAN_POINT ( 'NONE',  ( -10.37757302488624411, 4.975000002731183812, -31.93888565452638417 ) ) ;
#32845=CARTESIAN_POINT ( 'NONE',  ( -2.162160676586881955E-15, 12.62500000273118772, -35.31076352940723240 ) ) ;
#32846=CARTESIAN_POINT ( 'NONE',  ( -8.960552108402744065E-16, 74.37500000273118417, -14.63369212191046209 ) ) ;
#32848=CARTESIAN_POINT ( 'NONE',  ( -15.00000000000000000, 80.00000000000001421, 0.000000000000000000 ) ) ;
#32851=CARTESIAN_POINT ( 'NONE',  ( -15.00000000000000000, 76.15000000546235981, -4.873795443493594171 ) ) ;
#32853=CARTESIAN_POINT ( 'NONE',  ( 6.486482029760649416E-15, 37.62500000273118417, 35.31076352940723240 ) ) ;
#32856=CARTESIAN_POINT ( 'NONE',  ( 6.486482029760648627E-15, 27.87500000273120193, 35.31076352940722529 ) ) ;
#32857=CARTESIAN_POINT ( 'NONE',  ( -32.50000000000000000, 12.50000000546236478, 0.000000000000000000 ) ) ;
#32859=CARTESIAN_POINT ( 'NONE',  ( 32.50000000000000000, 33.10000000000000142, -10.55989012756945833 ) ) ;
#32861=CARTESIAN_POINT ( 'NONE',  ( 14.47279130897151944, 12.92499999726881832, -19.92008829642072598 ) ) ;
#32865=DIRECTION ( 'NONE',  ( 0.000000000000000000, 0.000000000000000000, -1.000000000000000000 ) ) ;
#32866=CARTESIAN_POINT ( 'NONE',  ( -27.16883889988623935, 15.32500000273118168, 19.73931689729374739 ) ) ;
#32867=CARTESIAN_POINT ( 'NONE',  ( -7.236395654485757944, 11.72499999726880837, -22.27133577429736988 ) ) ;
#32869=ORIENTED_EDGE ( 'NONE', *, *, #28667, .T. ) ;
#32876=CARTESIAN_POINT ( 'NONE',  ( -7.570916362186215665, 17.14999999453761959, 23.30088464923126423 ) ) ;
#32877=CARTESIAN_POINT ( 'NONE',  ( 7.236395654485760609, 7.024999997268799312, -22.27133577429736633 ) ) ;
#32878=CARTESIAN_POINT ( 'NONE',  ( 20.75514604977248467, 20.67500000273119909, -28.56700777964554305 ) ) ;
#32879=CARTESIAN_POINT ( 'NONE',  ( -20.08610463437156923, 26.80000000546238681, 27.64615127144130113 ) ) ;
#32880=CARTESIAN_POINT ( 'NONE',  ( 10.04305231718579705, 70.59999999999999432, 30.90933677959248982 ) ) ;
#32884=CARTESIAN_POINT ( 'NONE',  ( -20.75514604977248112, 39.67500000273118133, 28.56700777964554661 ) ) ;
#32887=CARTESIAN_POINT ( 'NONE',  ( -14.47279130897151589, 11.82499999726882578, -19.92008829642072598 ) ) ;
#32888=CARTESIAN_POINT ( 'NONE',  ( -2.092463501923844636E-15, 15.50000000000000533, -34.17252228774368916 ) ) ;
#32889=CARTESIAN_POINT ( 'NONE',  ( -1.778240108872766143E-15, 10.00000000546236834, -32.49999999999999289 ) ) ;
#32891=CARTESIAN_POINT ( 'NONE',  ( -20.75514604977248112, 55.42500000273119554, 28.56700777964554661 ) ) ;
#32892=CARTESIAN_POINT ( 'NONE',  ( 33.58253175000000113, 46.37500000273120548, -4.112674001490185761E-15 ) ) ;
#32893=DIRECTION ( 'NONE',  ( -0.000000000000000000, -1.000000000000000000, -0.000000000000000000 ) ) ;
#32894=DIRECTION ( 'NONE',  ( -0.000000000000000000, 1.000000000000000000, -0.000000000000000000 ) ) ;
#32897=( BOUNDED_CURVE ( )  B_SPLINE_CURVE ( 2, ( #30508, #12332, #17490, #14570, #4096, #1855, #17151 ),
 .UNSPECIFIED., .F., .T. ) 
 B_SPLINE_CURVE_WITH_KNOTS ( ( 3, 2, 2, 3 ),
 ( 0.000000000000000000, 0.002564102564102564100, 0.005128205128205128201, 0.006410256410256410901 ),
 .UNSPECIFIED. ) 
 CURVE ( )  GEOMETRIC_REPRESENTATION_ITEM ( )  RATIONAL_B_SPLINE_CURVE ( ( 1.000000000000000000, 0.9510565162951535312, 1.000000000000000000, 0.9510565162951535312, 1.000000000000000000, 0.9755282581475768211, 0.9755282581475768211 ) ) 
 REPRESENTATION_ITEM ( '' )  );
#32899=FACE_OUTER_BOUND ( 'NONE', #26903, .T. ) ;
#32903=LINE ( 'NONE', #15083, #11036 ) ;
#32906=EDGE_CURVE ( 'NONE', #11992, #564, #12684, .T. ) ;
#32907=CARTESIAN_POINT ( 'NONE',  ( 5.147494310547426899, 11.44874571845314293, -32.50000000000000000 ) ) ;
#32908=CARTESIAN_POINT ( 'NONE',  ( 33.58253175000000823, 34.02500000273118275, 10.91162601494192685 ) ) ;
#32909=VECTOR ( 'NONE', #6733, 1000.000000000000000 ) ;
#32911=EDGE_CURVE ( 'NONE', #21391, #1603, #7396, .T. ) ;
#32914=DIRECTION ( 'NONE',  ( -0.000000000000000000, -1.000000000000000000, -0.000000000000000000 ) ) ;
#32915=VERTEX_POINT ( 'NONE', #22093 ) ;
#32921=CARTESIAN_POINT ( 'NONE',  ( -20.75514604977248112, 41.67500000273117422, 28.56700777964554661 ) ) ;
#32922=CARTESIAN_POINT ( 'NONE',  ( 26.29305231718579350, 45.30000000546238681, 19.10302069950537529 ) ) ;
#32924=CARTESIAN_POINT ( 'NONE',  ( -33.58253175000000113, 27.02500000273119696, -10.91162601494193218 ) ) ;
#32925=CARTESIAN_POINT ( 'NONE',  ( 26.29305231718579350, 31.30000000546237615, 19.10302069950537529 ) ) ;
#32926=CARTESIAN_POINT ( 'NONE',  ( 6.486482029760649416E-15, 57.87500000273117706, 35.31076352940723240 ) ) ;
#32929=CARTESIAN_POINT ( 'NONE',  ( 20.08610463437158344, 34.70000000000001705, 27.64615127144129403 ) ) ;
#32931=CARTESIAN_POINT ( 'NONE',  ( -33.58253175000000113, 75.22500000273119269, 10.91162601494193929 ) ) ;
#32936=CARTESIAN_POINT ( 'NONE',  ( -20.75514604977248112, 67.67500000273116711, 28.56700777964554661 ) ) ;
#32938=LINE ( 'NONE', #27472, #24334 ) ;
#32939=CARTESIAN_POINT ( 'NONE',  ( -19.82091636218621034, 6.549999994537619941, -14.40073868116559552 ) ) ;
#32941=CARTESIAN_POINT ( 'NONE',  ( 3.880418787951140036, 8.198745712990779921, -24.49999999999999645 ) ) ;
#32952=CARTESIAN_POINT ( 'NONE',  ( 10.04305231718578817, 75.90000000546237402, -30.90933677959249337 ) ) ;
#32959=ORIENTED_EDGE ( 'NONE', *, *, #2231, .F. ) ;
#32961=CARTESIAN_POINT ( 'NONE',  ( -2.092463501923844636E-15, 64.00000000546236834, -34.17252228774368916 ) ) ;
#32963=CARTESIAN_POINT ( 'NONE',  ( -32.50000000000000000, 55.90000000000000568, -10.55989012756945300 ) ) ;
#32964=CARTESIAN_POINT ( 'NONE',  ( 27.16883889988624290, 47.92500000273120264, 19.73931689729373673 ) ) ;
#32965=CARTESIAN_POINT ( 'NONE',  ( 10.04305231718579705, 55.10000000546239107, 30.90933677959248982 ) ) ;
#32967=CARTESIAN_POINT ( 'NONE',  ( -10.04305231718579172, 10.10000000546237864, -30.90933677959248982 ) ) ;
#32968=CARTESIAN_POINT ( 'NONE',  ( -1.089172066684569321E-14, 78.49999999999998579, 15.00000000000000000 ) ) ;
#32969=CARTESIAN_POINT ( 'NONE',  ( -7.236395654485757944, 15.72499999726881192, -22.27133577429736988 ) ) ;
#32970=CARTESIAN_POINT ( 'NONE',  ( 26.29305231718578995, 55.19999999999999574, -19.10302069950538240 ) ) ;
#32972=CARTESIAN_POINT ( 'NONE',  ( -33.58253175000000113, 17.47500000273117848, 10.91162601494193929 ) ) ;
#32973=CARTESIAN_POINT ( 'NONE',  ( -19.82091636218621034, 6.800000000000000711, -14.40073868116559552 ) ) ;
#32975=CARTESIAN_POINT ( 'NONE',  ( -8.601468415847515203, 75.17500000273118133, 11.83890561707634959 ) ) ;
#32977=CARTESIAN_POINT ( 'NONE',  ( -32.50000000000000000, 21.90000000000000568, -10.55989012756945300 ) ) ;
#32986=CARTESIAN_POINT ( 'NONE',  ( 27.16883889988623935, 2.575000002731198112, -19.73931689729374384 ) ) ;
#32990=CARTESIAN_POINT ( 'NONE',  ( 33.58253175000000113, 52.22500000273118559, -10.91162601494193574 ) ) ;
#32993=ORIENTED_EDGE ( 'NONE', *, *, #1170, .F. ) ;
#32995=CARTESIAN_POINT ( 'NONE',  ( -32.50000000000000000, 2.099999999999991651, 10.55989012756946366 ) ) ;
#32997=CARTESIAN_POINT ( 'NONE',  ( -7.236395654485757944, 11.22499999726880837, -22.27133577429736988 ) ) ;
#33002=CARTESIAN_POINT ( 'NONE',  ( 24.50000000000000000, 5.899999999999987921, 7.960532557706212486 ) ) ;
#33006=CARTESIAN_POINT ( 'NONE',  ( -27.16883889988623935, 57.57500000273119412, 19.73931689729374739 ) ) ;
#33007=CARTESIAN_POINT ( 'NONE',  ( -26.29305231718579350, 36.30000000546237970, -19.10302069950537884 ) ) ;
#33008=CARTESIAN_POINT ( 'NONE',  ( 27.16883889988623935, 68.32500000273117280, -19.73931689729374384 ) ) ;
#33010=CARTESIAN_POINT ( 'NONE',  ( 24.50000000000000355, 12.09999999999999787, -7.960532557706203605 ) ) ;
#33012=CARTESIAN_POINT ( 'NONE',  ( 27.16883889988624290, 7.925000002731191984, 19.73931689729373673 ) ) ;
#33015=CARTESIAN_POINT ( 'NONE',  ( -4.635254915624208216, 72.40000000000001990, 14.26584774442730463 ) ) ;
#33018=CARTESIAN_POINT ( 'NONE',  ( 5.147494310547426899, 23.44874571845314648, -32.50000000000000000 ) ) ;
#33020=CARTESIAN_POINT ( 'NONE',  ( -9.270509831248421762, 76.55000000546237970, 12.75976212528060039 ) ) ;
#33022=CARTESIAN_POINT ( 'NONE',  ( 20.75514604977248467, 38.42500000273118133, -28.56700777964554305 ) ) ;
#33023=VECTOR ( 'NONE', #18093, 1000.000000000000000 ) ;
#33026=CARTESIAN_POINT ( 'NONE',  ( 6.486482029760648627E-15, 25.87500000273117351, 35.31076352940722529 ) ) ;
#33027=CARTESIAN_POINT ( 'NONE',  ( -15.14183272437242778, 17.04999999453762527, 20.84094480462497856 ) ) ;
#33030=CARTESIAN_POINT ( 'NONE',  ( 20.08610463437158344, 78.69999999999998863, 27.64615127144129403 ) ) ;
#33032=CARTESIAN_POINT ( 'NONE',  ( -7.236395654485757944, 11.22499999726880837, -22.27133577429736988 ) ) ;
#33036=ADVANCED_FACE ( 'NONE', ( #11287 ), #14198, .T. ) ;
#33037=CARTESIAN_POINT ( 'NONE',  ( -1.778240108872766143E-15, 30.00000000546237189, -32.49999999999999289 ) ) ;
#33038=CARTESIAN_POINT ( 'NONE',  ( 10.37757302488624767, 13.72500000273119092, 31.93888565452638417 ) ) ;
#33039=CARTESIAN_POINT ( 'NONE',  ( 23.41746825000000243, 15.22499999726880482, -7.608796670333727974 ) ) ;
#33042=ORIENTED_EDGE ( 'NONE', *, *, #6322, .F. ) ;
#33045=VERTEX_POINT ( 'NONE', #29301 ) ;
#33048=CARTESIAN_POINT ( 'NONE',  ( -26.29305231718578995, 72.70000000546239960, 19.10302069950538595 ) ) ;
#33049=CARTESIAN_POINT ( 'NONE',  ( -24.50000000000000000, 18.74999999453763522, -3.000384657911015469E-15 ) ) ;
#33052=CARTESIAN_POINT ( 'NONE',  ( -23.41746825000000243, 13.52499999726880198, -7.608796670333730638 ) ) ;
#33053=CARTESIAN_POINT ( 'NONE',  ( 33.58253175000000113, 24.37500000273118417, -4.112674001490185761E-15 ) ) ;
#33054=CARTESIAN_POINT ( 'NONE',  ( 26.29305231718579350, 27.30000000546237260, 19.10302069950537529 ) ) ;
#33055=CARTESIAN_POINT ( 'NONE',  ( 32.50000000000000000, 67.00000000000000000, -3.980102097228898626E-15 ) ) ;
#33056=CARTESIAN_POINT ( 'NONE',  ( 20.08610463437158344, 47.20000000546237828, 27.64615127144129403 ) ) ;
#33059=CARTESIAN_POINT ( 'NONE',  ( 33.58253175000000113, 38.47500000273118559, -10.91162601494193751 ) ) ;
#33060=CARTESIAN_POINT ( 'NONE',  ( 5.779280353836490358E-15, 43.00000000546236834, 32.49999999999999289 ) ) ;
#33064=CARTESIAN_POINT ( 'NONE',  ( -10.04305231718578462, 16.39999999999999858, 30.90933677959249337 ) ) ;
#33067=CARTESIAN_POINT ( 'NONE',  ( -20.75514604977248112, 59.42500000273118843, 28.56700777964554661 ) ) ;
#33069=CARTESIAN_POINT ( 'NONE',  ( 10.37757302488624767, 45.97500000273119269, 31.93888565452638417 ) ) ;
#33070=CARTESIAN_POINT ( 'NONE',  ( -1.778240108872766143E-15, 45.49999999999999289, -32.49999999999999289 ) ) ;
#33071=LINE ( 'NONE', #11813, #20526 ) ;
#33072=CARTESIAN_POINT ( 'NONE',  ( -20.08610463437156923, 50.30000000000001137, 27.64615127144130113 ) ) ;
#33075=CARTESIAN_POINT ( 'NONE',  ( -1.778240108872766143E-15, 71.50000000000001421, -32.49999999999999289 ) ) ;
#33077=CARTESIAN_POINT ( 'NONE',  ( 32.50000000000000000, 67.00000000000000000, -3.980102097228898626E-15 ) ) ;
#33081=DIRECTION ( 'NONE',  ( -0.000000000000000000, -1.000000000000000000, -0.000000000000000000 ) ) ;
#33084=CARTESIAN_POINT ( 'NONE',  ( 1.093617666956751375E-13, 60.00000000546237544, -32.50000000000000711 ) ) ;
#33085=CARTESIAN_POINT ( 'NONE',  ( -20.75514604977248112, 33.42500000273120264, 28.56700777964554661 ) ) ;
#33088=ORIENTED_EDGE ( 'NONE', *, *, #21276, .T. ) ;
#33092=EDGE_LOOP ( 'NONE', ( #19727, #13632, #21167, #30049, #24460, #32379, #7018, #32338, #4272, #4787, #25208, #22057, #22680, #16703, #32132, #7314, #30387, #22900, #25105, #4528, #28974, #26988, #15099, #14123, #22730, #30568, #4149, #24998, #9286, #28803, #32126, #4698, #33957, #6766, #5041, #29934, #4783, #3940, #30389, #6557, #14289, #33919, #33113, #5468, #31296, #8793, #4, #32837, #2857, #8789, #28588, #26408, #11191, #3073, #3113, #9288, #14605, #17223, #21866, #6238, #4739, #20373, #28424, #23286, #27133, #8962, #24558, #9509, #30863, #2854, #3023, #18857, #5761, #32169, #13451, #28870, #6347, #8708, #15909, #24003, #31212, #5477 ) ) ;
#33097=CARTESIAN_POINT ( 'NONE',  ( 5.779280353836490358E-15, 43.00000000546236834, 32.49999999999999289 ) ) ;
#33098=CARTESIAN_POINT ( 'NONE',  ( 10.37757302488624056, 42.77500000273118275, -31.93888565452638417 ) ) ;
#33099=CARTESIAN_POINT ( 'NONE',  ( -10.04305231718579172, 44.10000000546238397, -30.90933677959248982 ) ) ;
#33101=CARTESIAN_POINT ( 'NONE',  ( 33.58253175000000823, 32.02500000273118275, 10.91162601494192863 ) ) ;
#33102=CARTESIAN_POINT ( 'NONE',  ( 20.75514604977248467, 52.67500000273116711, -28.56700777964554305 ) ) ;
#33104=CARTESIAN_POINT ( 'NONE',  ( -32.50000000000000000, 32.00000000000000000, 0.000000000000000000 ) ) ;
#33107=( BOUNDED_CURVE ( )  B_SPLINE_CURVE ( 2, ( #10785, #8199, #124, #10279, #23833, #21262, #18352, #298, #31030, #31707, #18690, #23492, #18520 ),
 .UNSPECIFIED., .F., .T. ) 
 B_SPLINE_CURVE_WITH_KNOTS ( ( 3, 2, 2, 2, 2, 2, 3 ),
 ( 0.5064102564102563875, 0.5076923076923076650, 0.5102564102564102200, 0.5128205128205127750, 0.5153846153846153300, 0.5179487179487179960, 0.5192307692307692735 ),
 .UNSPECIFIED. ) 
 CURVE ( )  GEOMETRIC_REPRESENTATION_ITEM ( )  RATIONAL_B_SPLINE_CURVE ( ( 0.9755282581475768211, 0.9755282581475768211, 1.000000000000000000, 0.9510565162951535312, 1.000000000000000000, 0.9510565162951535312, 1.000000000000000000, 0.9510565162951535312, 1.000000000000000000, 0.9510565162951535312, 1.000000000000000000, 0.9755282581475768211, 0.9755282581475768211 ) ) 
 REPRESENTATION_ITEM ( '' )  );
#33108=CARTESIAN_POINT ( 'NONE',  ( 20.75514604977249178, 77.82500000273120122, 28.56700777964553950 ) ) ;
#33111=CARTESIAN_POINT ( 'NONE',  ( 33.58253175000000823, 68.27500000273120406, 10.91162601494192685 ) ) ;
#33113=ORIENTED_EDGE ( 'NONE', *, *, #33267, .T. ) ;
#33114=CARTESIAN_POINT ( 'NONE',  ( -2.162160676586881955E-15, 16.62500000273120548, -35.31076352940723240 ) ) ;
#33115=CARTESIAN_POINT ( 'NONE',  ( -7.570916362186210335, 10.34999999453761710, -23.30088464923126779 ) ) ;
#33126=DIRECTION ( 'NONE',  ( 0.000000000000000000, 0.000000000000000000, 1.000000000000000000 ) ) ;
#33127=CARTESIAN_POINT ( 'NONE',  ( -10.04305231718579172, 78.10000000546237686, -30.90933677959248982 ) ) ;
#33131=VERTEX_POINT ( 'NONE', #7136 ) ;
#33132=CARTESIAN_POINT ( 'NONE',  ( 6.486482029760649416E-15, 71.87500000273116996, 35.31076352940723240 ) ) ;
#33135=ORIENTED_EDGE ( 'NONE', *, *, #9342, .F. ) ;
#33137=CARTESIAN_POINT ( 'NONE',  ( 26.29305231718579350, 65.30000000546237970, 19.10302069950537529 ) ) ;
#33138=VERTEX_POINT ( 'NONE', #33037 ) ;
#33139=CARTESIAN_POINT ( 'NONE',  ( -10.04305231718578462, 74.90000000546237402, 30.90933677959249337 ) ) ;
#33140=CARTESIAN_POINT ( 'NONE',  ( 6.486482029760649416E-15, 45.62500000273118417, 35.31076352940723240 ) ) ;
#33141=CARTESIAN_POINT ( 'NONE',  ( 2.205017735002230837E-13, 56.00000000546238255, -32.50000000000000000 ) ) ;
#33142=CARTESIAN_POINT ( 'NONE',  ( -26.29305231718579350, 6.300000005462380592, -19.10302069950537884 ) ) ;
#33144=CARTESIAN_POINT ( 'NONE',  ( 14.47279130897151767, 18.82499999726880802, 19.92008829642072953 ) ) ;
#33146=CARTESIAN_POINT ( 'NONE',  ( 26.29305231718578995, 53.19999999999999574, -19.10302069950538240 ) ) ;
#33147=ADVANCED_FACE ( 'NONE', ( #33390 ), #30296, .T. ) ;
#33148=CARTESIAN_POINT ( 'NONE',  ( 5.779280353836490358E-15, 14.50000000000000178, 32.49999999999999289 ) ) ;
#33149=CARTESIAN_POINT ( 'NONE',  ( -2.162160676586881955E-15, 18.87500000273119483, -35.31076352940723240 ) ) ;
#33152=CARTESIAN_POINT ( 'NONE',  ( -13.91746824999999532, 74.77500000273117564, -4.522059556121115875 ) ) ;
#33164=CARTESIAN_POINT ( 'NONE',  ( 33.58253175000000113, 2.375000002731192161, -4.112674001490185761E-15 ) ) ;
#33168=CARTESIAN_POINT ( 'NONE',  ( -13.91746824999999532, 73.47500000273119269, 4.522059556121122093 ) ) ;
#33170=CARTESIAN_POINT ( 'NONE',  ( -27.16883889988623935, 43.32500000273120833, 19.73931689729374739 ) ) ;
#33172=CARTESIAN_POINT ( 'NONE',  ( 26.29305231718579350, 21.30000000546239391, 19.10302069950537529 ) ) ;
#33174=VERTEX_POINT ( 'NONE', #8878 ) ;
#33176=FACE_OUTER_BOUND ( 'NONE', #19436, .T. ) ;
#33177=CARTESIAN_POINT ( 'NONE',  ( 7.236395654485760609, 13.02499999726880375, -22.27133577429736633 ) ) ;
#33179=ORIENTED_EDGE ( 'NONE', *, *, #8518, .F. ) ;
#33181=CARTESIAN_POINT ( 'NONE',  ( -20.08610463437156923, 34.80000000546238681, 27.64615127144130113 ) ) ;
#33185=CARTESIAN_POINT ( 'NONE',  ( 33.58253175000000113, 66.22500000273120691, -10.91162601494193751 ) ) ;
#33187=CARTESIAN_POINT ( 'NONE',  ( 24.50000000000000355, 13.89999999999999858, 7.960532557706212486 ) ) ;
#33188=CARTESIAN_POINT ( 'NONE',  ( -7.236395654485757944, 1.724999997268800156, -22.27133577429736988 ) ) ;
#33189=CARTESIAN_POINT ( 'NONE',  ( 10.37757302488624767, 9.725000002731187365, 31.93888565452638417 ) ) ;
#33190=CARTESIAN_POINT ( 'NONE',  ( 10.04305231718578817, 29.40000000000000924, -30.90933677959249337 ) ) ;
#33192=CARTESIAN_POINT ( 'NONE',  ( 26.29305231718579350, 36.79999999999999716, 19.10302069950537529 ) ) ;
#33194=CARTESIAN_POINT ( 'NONE',  ( 0.000000000000000000, 80.00000000000001421, 0.000000000000000000 ) ) ;
#33195=CARTESIAN_POINT ( 'NONE',  ( 2.445080149700053643E-15, 74.75000000546236834, 15.00000000000000000 ) ) ;
#33197=CARTESIAN_POINT ( 'NONE',  ( -12.13525491562420910, 74.45000000546237118, 8.816778784387098611 ) ) ;
#33199=CARTESIAN_POINT ( 'NONE',  ( 20.75514604977249178, 39.82500000273116569, 28.56700777964553950 ) ) ;
#33202=CARTESIAN_POINT ( 'NONE',  ( -20.75514604977248823, 19.07500000273118701, -28.56700777964554305 ) ) ;
#33205=CARTESIAN_POINT ( 'NONE',  ( 5.779280353836490358E-15, 13.00000000546238077, 32.49999999999999289 ) ) ;
#33207=CARTESIAN_POINT ( 'NONE',  ( 23.41746824999999887, 12.62499999726882116, 0.000000000000000000 ) ) ;
#33208=CARTESIAN_POINT ( 'NONE',  ( -20.75514604977248112, 61.42500000273118133, 28.56700777964554661 ) ) ;
#33209=( BOUNDED_CURVE ( )  B_SPLINE_CURVE ( 2, ( #19153, #773, #599, #11254, #8834, #8670, #29095, #29759, #3030, #8332, #29592, #16575, #27030 ),
 .UNSPECIFIED., .F., .T. ) 
 B_SPLINE_CURVE_WITH_KNOTS ( ( 3, 2, 2, 2, 2, 2, 3 ),
 ( 0.1217948717948718063, 0.1230769230769230838, 0.1256410256410256387, 0.1282051282051281937, 0.1307692307692307765, 0.1333333333333333315, 0.1346153846153846090 ),
 .UNSPECIFIED. ) 
 CURVE ( )  GEOMETRIC_REPRESENTATION_ITEM ( )  RATIONAL_B_SPLINE_CURVE ( ( 0.9755282581475767101, 0.9755282581475768211, 1.000000000000000000, 0.9510565162951535312, 1.000000000000000000, 0.9510565162951535312, 1.000000000000000000, 0.9510565162951535312, 1.000000000000000000, 0.9510565162951535312, 1.000000000000000000, 0.9755282581475768211, 0.9755282581475768211 ) ) 
 REPRESENTATION_ITEM ( '' )  );
#33212=EDGE_CURVE ( 'NONE', #1686, #3077, #16212, .T. ) ;
#33214=( BOUNDED_CURVE ( )  B_SPLINE_CURVE ( 2, ( #4557, #15036, #15207, #7298, #25671, #9353, #30117, #30288, #28411, #25838, #28576, #10396, #10233 ),
 .UNSPECIFIED., .F., .F. ) 
 B_SPLINE_CURVE_WITH_KNOTS ( ( 3, 2, 2, 2, 2, 2, 3 ),
 ( 0.1474358974358974395, 0.1487179487179487170, 0.1512820512820512719, 0.1538461538461538547, 0.1564102564102564097, 0.1589743589743589647, 0.1602564102564102699 ),
 .UNSPECIFIED. ) 
 CURVE ( )  GEOMETRIC_REPRESENTATION_ITEM ( )  RATIONAL_B_SPLINE_CURVE ( ( 0.9755282581475768211, 0.9755282581475768211, 1.000000000000000000, 0.9510565162951535312, 1.000000000000000000, 0.9510565162951535312, 1.000000000000000000, 0.9510565162951535312, 1.000000000000000000, 0.9510565162951535312, 1.000000000000000000, 0.9755282581475764880, 0.9755282581475768211 ) ) 
 REPRESENTATION_ITEM ( '' )  );
#33215=CARTESIAN_POINT ( 'NONE',  ( -27.16883889988624290, 10.92500000273119376, -19.73931689729374028 ) ) ;
#33216=CARTESIAN_POINT ( 'NONE',  ( 23.41746824999999887, 11.12499999726881938, 0.000000000000000000 ) ) ;
#33221=ORIENTED_EDGE ( 'NONE', *, *, #9334, .T. ) ;
#33225=CARTESIAN_POINT ( 'NONE',  ( -10.04305231718579172, 72.10000000546237686, -30.90933677959248982 ) ) ;
#33226=CARTESIAN_POINT ( 'NONE',  ( -18.94512977948575738, 5.924999997268809437, -13.76444248337723231 ) ) ;
#33227=CARTESIAN_POINT ( 'NONE',  ( 7.236395654485760609, 9.024999997268800200, -22.27133577429736633 ) ) ;
#33228=CARTESIAN_POINT ( 'NONE',  ( 20.75514604977249178, 22.07500000273117990, 28.56700777964553950 ) ) ;
#33229=CARTESIAN_POINT ( 'NONE',  ( -10.04305231718579172, 22.10000000546236265, -30.90933677959248982 ) ) ;
#33230=CARTESIAN_POINT ( 'NONE',  ( -26.29305231718578995, 64.20000000000000284, 19.10302069950538595 ) ) ;
#33234=CARTESIAN_POINT ( 'NONE',  ( -10.37757302488623701, 35.77500000273120406, 31.93888565452638417 ) ) ;
#33235=CARTESIAN_POINT ( 'NONE',  ( -20.08610463437156923, 32.80000000546237260, 27.64615127144130113 ) ) ;
#33238=AXIS2_PLACEMENT_3D ( 'NONE', #21246, #25868, #13003 ) ;
#33239=CARTESIAN_POINT ( 'NONE',  ( -14.47279130897151589, 13.82499999726882045, -19.92008829642072598 ) ) ;
#33240=CARTESIAN_POINT ( 'NONE',  ( 32.50000000000000000, 11.00000000000001066, -3.980102097228898626E-15 ) ) ;
#33241=CARTESIAN_POINT ( 'NONE',  ( 10.04305231718579705, 9.100000005462376862, 30.90933677959248982 ) ) ;
#33243=CARTESIAN_POINT ( 'NONE',  ( 10.37757302488624767, 57.72500000273117848, 31.93888565452638417 ) ) ;
#33245=CARTESIAN_POINT ( 'NONE',  ( 27.16883889988624290, 44.17500000273119554, 19.73931689729373673 ) ) ;
#33249=LINE ( 'NONE', #9745, #9521 ) ;
#33253=FACE_OUTER_BOUND ( 'NONE', #23968, .T. ) ;
#33255=CARTESIAN_POINT ( 'NONE',  ( 20.08610463437157279, 67.29999999999998295, -27.64615127144129758 ) ) ;
#33262=CARTESIAN_POINT ( 'NONE',  ( -20.08610463437156923, 60.80000000546238681, 27.64615127144130113 ) ) ;
#33263=CARTESIAN_POINT ( 'NONE',  ( 33.58253175000000113, 30.12500000273118772, -4.112674001490185761E-15 ) ) ;
#33264=CARTESIAN_POINT ( 'NONE',  ( 10.37757302488624056, 64.77500000273117564, -31.93888565452638417 ) ) ;
#33266=ORIENTED_EDGE ( 'NONE', *, *, #2764, .T. ) ;
#33267=EDGE_CURVE ( 'NONE', #30543, #29467, #28220, .T. ) ;
#33277=CARTESIAN_POINT ( 'NONE',  ( 27.16883889988624290, 38.17500000273118843, 19.73931689729373673 ) ) ;
#33278=CARTESIAN_POINT ( 'NONE',  ( 26.29305231718578995, 43.70000000546237118, -19.10302069950538240 ) ) ;
#33280=CARTESIAN_POINT ( 'NONE',  ( 10.37757302488624767, 31.72500000273117848, 31.93888565452638417 ) ) ;
#33282=CARTESIAN_POINT ( 'NONE',  ( -2.162160676586881955E-15, 52.87500000273119838, -35.31076352940723240 ) ) ;
#33285=CARTESIAN_POINT ( 'NONE',  ( 32.50000000000000711, 26.89999999999999147, 10.55989012756945122 ) ) ;
#33287=CARTESIAN_POINT ( 'NONE',  ( 33.58253175000000113, 74.12500000273119838, -4.112674001490185761E-15 ) ) ;
#33290=CARTESIAN_POINT ( 'NONE',  ( 10.37757302488624767, 61.97500000273120691, 31.93888565452638417 ) ) ;
#33292=DIRECTION ( 'NONE',  ( -0.000000000000000000, -1.000000000000000000, -0.000000000000000000 ) ) ;
#33293=CARTESIAN_POINT ( 'NONE',  ( 6.486482029760649416E-15, 19.62500000273116996, 35.31076352940723240 ) ) ;
#33294=CARTESIAN_POINT ( 'NONE',  ( -15.14183272437241889, 12.44999999453762918, -20.84094480462497856 ) ) ;
#33296=CARTESIAN_POINT ( 'NONE',  ( -26.29305231718578995, 26.20000000000000284, 19.10302069950538595 ) ) ;
#33307=CARTESIAN_POINT ( 'NONE',  ( -14.47279130897151589, 1.824999997268821339, -19.92008829642072598 ) ) ;
#33308=CARTESIAN_POINT ( 'NONE',  ( -32.50000000000000000, 74.40000000546234560, -10.55989012756945478 ) ) ;
#33313=CARTESIAN_POINT ( 'NONE',  ( -27.16883889988623935, 77.57500000273121543, 19.73931689729374739 ) ) ;
#33316=CARTESIAN_POINT ( 'NONE',  ( 6.277390505771533514E-15, 65.00000000546236834, 34.17252228774368916 ) ) ;
#33317=ORIENTED_EDGE ( 'NONE', *, *, #20647, .T. ) ;
#33318=( BOUNDED_CURVE ( )  B_SPLINE_CURVE ( 2, ( #31690, #19457, #8975, #7847, #2707, #3663, #8184, #31355, #6235, #14138, #13168, #18335, #29904 ),
 .UNSPECIFIED., .F., .T. ) 
 B_SPLINE_CURVE_WITH_KNOTS ( ( 3, 2, 2, 2, 2, 2, 3 ),
 ( 0.8611111111111111605, 0.8666666666666666963, 0.8777777777777777679, 0.8888888888888888395, 0.9000000000000000222, 0.9111111111111110938, 0.9166666666666666297 ),
 .UNSPECIFIED. ) 
 CURVE ( )  GEOMETRIC_REPRESENTATION_ITEM ( )  RATIONAL_B_SPLINE_CURVE ( ( 0.9755282581475768211, 0.9755282581475770431, 1.000000000000000000, 0.9510565162951535312, 1.000000000000000000, 0.9510565162951535312, 1.000000000000000000, 0.9510565162951535312, 1.000000000000000000, 0.9510565162951535312, 1.000000000000000000, 0.9755282581475770431, 0.9755282581475768211 ) ) 
 REPRESENTATION_ITEM ( '' )  );
#33319=CARTESIAN_POINT ( 'NONE',  ( 5.779280353836490358E-15, 73.00000000546236834, 32.49999999999999289 ) ) ;
#33320=CARTESIAN_POINT ( 'NONE',  ( -33.58253175000000113, 49.22500000273119269, 10.91162601494193929 ) ) ;
#33321=CARTESIAN_POINT ( 'NONE',  ( -18.94512977948576093, 17.82499999726880446, 13.76444248337722698 ) ) ;
#33322=CARTESIAN_POINT ( 'NONE',  ( 32.50000000000000000, 5.500000005462357677, -3.980102097228898626E-15 ) ) ;
#33323=CARTESIAN_POINT ( 'NONE',  ( -32.50000000000000000, 7.900000000000012790, -10.55989012756945300 ) ) ;
#33326=CARTESIAN_POINT ( 'NONE',  ( 10.04305231718578817, 55.40000000000000568, -30.90933677959249337 ) ) ;
#33328=CARTESIAN_POINT ( 'NONE',  ( -10.37757302488623701, 19.77500000273118985, 31.93888565452638417 ) ) ;
#33331=CARTESIAN_POINT ( 'NONE',  ( 11.25946833292375793, 76.57500000273120122, -8.180482586598735395 ) ) ;
#33333=CARTESIAN_POINT ( 'NONE',  ( 5.779280353836490358E-15, 53.00000000546238255, 32.49999999999999289 ) ) ;
#33343=CARTESIAN_POINT ( 'NONE',  ( -20.75514604977248112, 3.675000002731179105, 28.56700777964554661 ) ) ;
#33347=CARTESIAN_POINT ( 'NONE',  ( 5.779280353836490358E-15, 2.500000000000005329, 32.49999999999999289 ) ) ;
#33349=CARTESIAN_POINT ( 'NONE',  ( 20.75514604977248467, 42.42500000273117422, -28.56700777964554305 ) ) ;
#33352=ORIENTED_EDGE ( 'NONE', *, *, #32630, .F. ) ;
#33357=CARTESIAN_POINT ( 'NONE',  ( -10.37757302488624411, 74.97500000273119269, -31.93888565452638417 ) ) ;
#33358=EDGE_CURVE ( 'NONE', #27962, #14241, #6960, .T. ) ;
#33363=CARTESIAN_POINT ( 'NONE',  ( 23.41746824999999887, 1.124999997268810725, 0.000000000000000000 ) ) ;
#33364=CARTESIAN_POINT ( 'NONE',  ( -20.75514604977248112, 65.42500000273118133, 28.56700777964554661 ) ) ;
#33366=CARTESIAN_POINT ( 'NONE',  ( 19.82091636218621389, 14.19999999999999041, -14.40073868116559197 ) ) ;
#33367=CARTESIAN_POINT ( 'NONE',  ( 18.94512977948576093, 5.324999997268820451, -13.76444248337722875 ) ) ;
#33368=CARTESIAN_POINT ( 'NONE',  ( 33.58253175000000823, 12.02500000273117742, 10.91162601494192863 ) ) ;
#33371=CARTESIAN_POINT ( 'NONE',  ( 4.635254915624212657, 72.59999999999999432, 14.26584774442730286 ) ) ;
#33374=CARTESIAN_POINT ( 'NONE',  ( 26.29305231718578995, 23.19999999999999929, -19.10302069950538240 ) ) ;
#33376=CARTESIAN_POINT ( 'NONE',  ( -9.270509831248421762, 78.55000000546236549, 12.75976212528060039 ) ) ;
#33378=CARTESIAN_POINT ( 'NONE',  ( 10.37757302488624056, 28.52500000273120051, -31.93888565452638417 ) ) ;
#33381=CARTESIAN_POINT ( 'NONE',  ( 27.16883889988624290, 20.17500000273120264, 19.73931689729373673 ) ) ;
#33382=DIRECTION ( 'NONE',  ( -0.000000000000000000, -1.000000000000000000, -0.000000000000000000 ) ) ;
#33383=CARTESIAN_POINT ( 'NONE',  ( 20.75514604977248467, 74.42500000273119554, -28.56700777964554305 ) ) ;
#33384=CARTESIAN_POINT ( 'NONE',  ( -26.29305231718578995, 66.19999999999997442, 19.10302069950538595 ) ) ;
#33386=CARTESIAN_POINT ( 'NONE',  ( -14.47279130897152299, 15.92499999726881121, 19.92008829642072243 ) ) ;
#33387=CARTESIAN_POINT ( 'NONE',  ( -33.58253175000000113, 63.12500000273119127, 0.000000000000000000 ) ) ;
#33390=FACE_OUTER_BOUND ( 'NONE', #11702, .T. ) ;
#33391=CARTESIAN_POINT ( 'NONE',  ( 33.58253175000000113, 4.125000002731193938, -4.112674001490185761E-15 ) ) ;
#33392=CARTESIAN_POINT ( 'NONE',  ( 18.94512977948576093, 11.32499999726882578, -13.76444248337722875 ) ) ;
#33398=ADVANCED_FACE ( 'NONE', ( #22427 ), #20210, .F. ) ;
#33399=ORIENTED_EDGE ( 'NONE', *, *, #4186, .F. ) ;
#33404=CARTESIAN_POINT ( 'NONE',  ( 23.41746824999999887, 7.124999997268815832, 0.000000000000000000 ) ) ;
#33405=CARTESIAN_POINT ( 'NONE',  ( -14.47279130897151589, 9.324999997268816898, -19.92008829642072598 ) ) ;
#33406=CARTESIAN_POINT ( 'NONE',  ( -33.58253175000000113, 17.47500000273117848, 10.91162601494193929 ) ) ;
#33407=CARTESIAN_POINT ( 'NONE',  ( -2.092463501923844636E-15, 22.00000000546238965, -34.17252228774368916 ) ) ;
#33408=CARTESIAN_POINT ( 'NONE',  ( -10.04305231718578462, 68.40000000000001990, 30.90933677959249337 ) ) ;
#33412=CARTESIAN_POINT ( 'NONE',  ( 6.486482029760649416E-15, 31.87500000273119127, 35.31076352940723240 ) ) ;
#33413=CARTESIAN_POINT ( 'NONE',  ( 32.50000000000000711, 43.40000000546238113, 10.55989012756945122 ) ) ;
#33416=CARTESIAN_POINT ( 'NONE',  ( 1.507698388325705758E-15, 15.62499999726882116, -24.62258325217400312 ) ) ;
#33417=CARTESIAN_POINT ( 'NONE',  ( -32.50000000000000000, 10.10000000000000142, 10.55989012756946366 ) ) ;
#33420=CARTESIAN_POINT ( 'NONE',  ( 10.37757302488624767, 47.72500000273119269, 31.93888565452638417 ) ) ;
#33422=CARTESIAN_POINT ( 'NONE',  ( 33.58253175000000823, 40.27500000273118985, 10.91162601494192685 ) ) ;
#33423=( BOUNDED_CURVE ( )  B_SPLINE_CURVE ( 2, ( #29028, #24067, #23727, #26298, #3293, #3129, #13602, #367, #16343, #8101, #533, #28696, #11020 ),
 .UNSPECIFIED., .F., .F. ) 
 B_SPLINE_CURVE_WITH_KNOTS ( ( 3, 2, 2, 2, 2, 2, 3 ),
 ( 0.5448717948717948234, 0.5461538461538461009, 0.5487179487179487669, 0.5512820512820513219, 0.5538461538461538769, 0.5564102564102564319, 0.5576923076923077094 ),
 .UNSPECIFIED. ) 
 CURVE ( )  GEOMETRIC_REPRESENTATION_ITEM ( )  RATIONAL_B_SPLINE_CURVE ( ( 0.9755282581475768211, 0.9755282581475768211, 1.000000000000000000, 0.9510565162951535312, 1.000000000000000000, 0.9510565162951535312, 1.000000000000000000, 0.9510565162951535312, 1.000000000000000000, 0.9510565162951535312, 1.000000000000000000, 0.9755282581475768211, 0.9755282581475768211 ) ) 
 REPRESENTATION_ITEM ( '' )  );
#33426=CARTESIAN_POINT ( 'NONE',  ( 6.486482029760649416E-15, 1.625000002731185944, 35.31076352940723240 ) ) ;
#33430=CARTESIAN_POINT ( 'NONE',  ( -10.04305231718579172, 62.10000000546239818, -30.90933677959248982 ) ) ;
#33432=CYLINDRICAL_SURFACE ( 'NONE', #27530, 32.50000000000000000 ) ;
#33436=CARTESIAN_POINT ( 'NONE',  ( -10.37757302488623701, 33.52500000273117564, 31.93888565452638417 ) ) ;
#33437=CARTESIAN_POINT ( 'NONE',  ( -10.37757302488623701, 65.77500000273117564, 31.93888565452638417 ) ) ;
#33450=CARTESIAN_POINT ( 'NONE',  ( -20.75514604977248823, 35.07500000273120833, -28.56700777964554305 ) ) ;
#33451=CARTESIAN_POINT ( 'NONE',  ( -32.50000000000000000, 42.50000000546238965, 0.000000000000000000 ) ) ;
#33453=CARTESIAN_POINT ( 'NONE',  ( 27.16883889988623935, 22.32500000273118701, -19.73931689729374384 ) ) ;
#33454=CARTESIAN_POINT ( 'NONE',  ( 5.147494310547426899, 31.94874572391553258, -32.50000000000000000 ) ) ;
#33455=CARTESIAN_POINT ( 'NONE',  ( 20.75514604977248467, 48.67500000273117422, -28.56700777964554305 ) ) ;
#33457=CARTESIAN_POINT ( 'NONE',  ( 32.50000000000000000, 28.99999999999999645, -3.980102097228898626E-15 ) ) ;
#33459=CARTESIAN_POINT ( 'NONE',  ( 10.37757302488624056, 74.52500000273118985, -31.93888565452638417 ) ) ;
#33461=CARTESIAN_POINT ( 'NONE',  ( 7.313012447739250820E-14, 15.50000000000000178, 24.50000000000000000 ) ) ;
#33462=CARTESIAN_POINT ( 'NONE',  ( 33.58253175000000823, 58.27500000273116854, 10.91162601494192685 ) ) ;
#33465=CARTESIAN_POINT ( 'NONE',  ( -10.37757302488623701, 21.52500000273119340, 31.93888565452638417 ) ) ;
#33466=CARTESIAN_POINT ( 'NONE',  ( -7.570916362186215665, 11.14999999453764090, 23.30088464923126423 ) ) ;
#33468=CARTESIAN_POINT ( 'NONE',  ( -20.08610463437156923, 26.29999999999998295, 27.64615127144130113 ) ) ;
#33477=CARTESIAN_POINT ( 'NONE',  ( 3.778760231354629433E-15, 2.249999994537632553, -24.50000000000000355 ) ) ;
#33479=CARTESIAN_POINT ( 'NONE',  ( 32.50000000000000000, 63.50000000546238255, -3.980102097228898626E-15 ) ) ;
#33480=CARTESIAN_POINT ( 'NONE',  ( 26.29305231718579350, 77.30000000546239391, 19.10302069950537529 ) ) ;
#33483=EDGE_CURVE ( 'NONE', #2126, #15317, #27922, .T. ) ;
#33487=CARTESIAN_POINT ( 'NONE',  ( -33.58253175000000113, 75.27500000273118985, -10.91162601494193218 ) ) ;
#33490=CARTESIAN_POINT ( 'NONE',  ( -32.50000000000000000, 64.60000000546237686, 10.55989012756946366 ) ) ;
#33491=ORIENTED_EDGE ( 'NONE', *, *, #7267, .F. ) ;
#33492=CARTESIAN_POINT ( 'NONE',  ( -32.50000000000000000, 10.60000000546237153, 10.55989012756946366 ) ) ;
#33493=AXIS2_PLACEMENT_3D ( 'NONE', #14215, #21940, #19200 ) ;
#33494=CARTESIAN_POINT ( 'NONE',  ( 33.58253175000000113, 40.12500000273119838, -4.112674001490185761E-15 ) ) ;
#33495=CARTESIAN_POINT ( 'NONE',  ( 32.50000000000000000, 55.60000000546237686, -10.55989012756945833 ) ) ;
#33496=CARTESIAN_POINT ( 'NONE',  ( 6.277390505771533514E-15, 5.000000005462374553, 34.17252228774368916 ) ) ;
#33499=CARTESIAN_POINT ( 'NONE',  ( -32.50000000000000000, 49.89999999999999147, -10.55989012756945478 ) ) ;
#33500=CARTESIAN_POINT ( 'NONE',  ( -26.29305231718578995, 14.19999999999999041, 19.10302069950538595 ) ) ;
#33501=CARTESIAN_POINT ( 'NONE',  ( 27.16883889988623935, 16.57500000273118346, -19.73931689729374384 ) ) ;
#33502=CARTESIAN_POINT ( 'NONE',  ( -10.04305231718578462, 74.40000000000001990, 30.90933677959249337 ) ) ;
#33504=CARTESIAN_POINT ( 'NONE',  ( 2.688165632520823219E-15, 77.87500000273118417, 14.63369212191046387 ) ) ;
#33505=CARTESIAN_POINT ( 'NONE',  ( 10.37757302488624056, 78.77500000273118985, -31.93888565452638417 ) ) ;
#33506=CARTESIAN_POINT ( 'NONE',  ( 10.04305231718578817, 53.90000000546238113, -30.90933677959249337 ) ) ;
#33520=CARTESIAN_POINT ( 'NONE',  ( 2.688165632520823219E-15, 71.87500000273121259, 14.63369212191046209 ) ) ;
#33522=CIRCLE ( 'NONE', #2294, 30.50000000000000000 ) ;
#33523=CARTESIAN_POINT ( 'NONE',  ( 33.58253175000000113, 46.12500000273117706, -4.112674001490185761E-15 ) ) ;
#33525=CARTESIAN_POINT ( 'NONE',  ( 5.147494310547434893, 21.05125428700922185, 32.49999999999999289 ) ) ;
#33526=VERTEX_POINT ( 'NONE', #7147 ) ;
#33528=( BOUNDED_CURVE ( )  B_SPLINE_CURVE ( 2, ( #26604, #16814, #13731, #2927, #23868, #10821, #3102, #21301, #31741, #26772, #5998, #8232, #29335 ),
 .UNSPECIFIED., .F., .T. ) 
 B_SPLINE_CURVE_WITH_KNOTS ( ( 3, 2, 2, 2, 2, 2, 3 ),
 ( 0.7628205128205127750, 0.7641025641025640525, 0.7666666666666667185, 0.7692307692307692735, 0.7717948717948718285, 0.7743589743589743835, 0.7756410256410256610 ),
 .UNSPECIFIED. ) 
 CURVE ( )  GEOMETRIC_REPRESENTATION_ITEM ( )  RATIONAL_B_SPLINE_CURVE ( ( 0.9755282581475768211, 0.9755282581475768211, 1.000000000000000000, 0.9510565162951535312, 1.000000000000000000, 0.9510565162951535312, 1.000000000000000000, 0.9510565162951535312, 1.000000000000000000, 0.9510565162951535312, 1.000000000000000000, 0.9755282581475768211, 0.9755282581475768211 ) ) 
 REPRESENTATION_ITEM ( '' )  );
#33531=CARTESIAN_POINT ( 'NONE',  ( 27.16883889988623935, 74.57500000273120122, -19.73931689729374384 ) ) ;
#33535=ORIENTED_EDGE ( 'NONE', *, *, #7163, .T. ) ;
#33536=DIRECTION ( 'NONE',  ( 0.000000000000000000, 0.000000000000000000, -1.000000000000000000 ) ) ;
#33537=CARTESIAN_POINT ( 'NONE',  ( -27.16883889988623935, 65.32500000273117280, 19.73931689729374739 ) ) ;
#33539=CARTESIAN_POINT ( 'NONE',  ( -7.570916362186210335, 14.60000000000000142, -23.30088464923126779 ) ) ;
#33541=CARTESIAN_POINT ( 'NONE',  ( -10.37757302488624411, 8.725000002731187365, -31.93888565452638417 ) ) ;
#33544=CARTESIAN_POINT ( 'NONE',  ( 15.00000000000000000, 75.09999999999999432, -4.873795443493596835 ) ) ;
#33549=CARTESIAN_POINT ( 'NONE',  ( 9.270509831248423538, 71.55000000546239391, -12.75976212528059861 ) ) ;
#33552=CARTESIAN_POINT ( 'NONE',  ( 33.58253175000000823, 28.02500000273119340, 10.91162601494192863 ) ) ;
#33555=CARTESIAN_POINT ( 'NONE',  ( -20.75514604977248823, 25.07500000273120122, -28.56700777964554305 ) ) ;
#33556=CARTESIAN_POINT ( 'NONE',  ( -3.880418787951104953, 17.19874571299077104, 24.50000000000000711 ) ) ;
#33558=CARTESIAN_POINT ( 'NONE',  ( 10.37757302488624056, 78.52500000273118985, -31.93888565452638417 ) ) ;
#33559=CARTESIAN_POINT ( 'NONE',  ( 1.093617666956751375E-13, 60.00000000546237544, -32.50000000000000711 ) ) ;
#33561=VECTOR ( 'NONE', #27779, 1000.000000000000000 ) ;
#33562=CARTESIAN_POINT ( 'NONE',  ( 23.41746824999999887, 16.52499999726882152, 7.608796670333735079 ) ) ;
#33563=CARTESIAN_POINT ( 'NONE',  ( -10.37757302488624411, 66.72500000273117848, -31.93888565452638417 ) ) ;
#33564=VECTOR ( 'NONE', #2963, 1000.000000000000000 ) ;
#33567=CARTESIAN_POINT ( 'NONE',  ( -33.58253175000000113, 9.025000002731184523, -10.91162601494193041 ) ) ;
#33568=CARTESIAN_POINT ( 'NONE',  ( 18.94512977948576093, 13.32499999726882756, -13.76444248337722875 ) ) ;
#33570=VERTEX_POINT ( 'NONE', #12300 ) ;
#33572=VERTEX_POINT ( 'NONE', #10074 ) ;
#33577=CARTESIAN_POINT ( 'NONE',  ( 24.50000000000000000, 19.74999999453763877, 0.000000000000000000 ) ) ;
#33578=CARTESIAN_POINT ( 'NONE',  ( 23.41746825000000243, 14.52499999726880020, 7.608796670333735079 ) ) ;
#33579=CARTESIAN_POINT ( 'NONE',  ( 33.58253175000000113, 16.37500000273117706, -4.112674001490185761E-15 ) ) ;
#33580=CARTESIAN_POINT ( 'NONE',  ( 32.50000000000000000, 15.50000000546236656, -3.980102097228898626E-15 ) ) ;
#33582=CARTESIAN_POINT ( 'NONE',  ( 32.50000000000000000, 69.00000000000000000, -3.980102097228898626E-15 ) ) ;
#33583=CARTESIAN_POINT ( 'NONE',  ( 10.04305231718578817, 57.90000000546238823, -30.90933677959249337 ) ) ;
#33585=CARTESIAN_POINT ( 'NONE',  ( -33.58253175000000113, 33.27500000273120406, -10.91162601494193218 ) ) ;
#33586=FACE_OUTER_BOUND ( 'NONE', #7228, .T. ) ;
#33590=CARTESIAN_POINT ( 'NONE',  ( 18.94512977948576093, 15.32499999726882933, -13.76444248337722875 ) ) ;
#33591=CARTESIAN_POINT ( 'NONE',  ( 10.04305231718579705, 10.59999999999999787, 30.90933677959248982 ) ) ;
#33592=CARTESIAN_POINT ( 'NONE',  ( 10.04305231718578817, 17.90000000546238113, -30.90933677959249337 ) ) ;
#33595=CARTESIAN_POINT ( 'NONE',  ( -20.75514604977248823, 52.82500000273116569, -28.56700777964554305 ) ) ;
#33597=CARTESIAN_POINT ( 'NONE',  ( 20.75514604977249178, 40.07500000273118701, 28.56700777964553950 ) ) ;
#33600=AXIS2_PLACEMENT_3D ( 'NONE', #28959, #10270, #7854 ) ;
#33601=CARTESIAN_POINT ( 'NONE',  ( -10.04305231718579172, 61.59999999999998721, -30.90933677959248982 ) ) ;
#33602=CYLINDRICAL_SURFACE ( 'NONE', #1390, 30.50000000000000000 ) ;
#33605=CARTESIAN_POINT ( 'NONE',  ( 26.29305231718578995, 7.199999999999984190, -19.10302069950538240 ) ) ;
#33606=LINE ( 'NONE', #19885, #24262 ) ;
#33609=CARTESIAN_POINT ( 'NONE',  ( 19.82091636218621034, 17.54999999453762882, 14.40073868116559730 ) ) ;
#33610=CARTESIAN_POINT ( 'NONE',  ( 20.75514604977249178, 25.82500000273117990, 28.56700777964553950 ) ) ;
#33616=CARTESIAN_POINT ( 'NONE',  ( 5.779280353836490358E-15, 17.00000000546237899, 32.49999999999999289 ) ) ;
#33620=ORIENTED_EDGE ( 'NONE', *, *, #14403, .F. ) ;
#33624=CARTESIAN_POINT ( 'NONE',  ( 10.37757302488624767, 33.97500000273117848, 31.93888565452638417 ) ) ;
#33625=CARTESIAN_POINT ( 'NONE',  ( 20.08610463437158344, 43.20000000546235697, 27.64615127144129403 ) ) ;
#33628=CARTESIAN_POINT ( 'NONE',  ( 10.37757302488624056, 22.52500000273119340, -31.93888565452638417 ) ) ;
#33630=CARTESIAN_POINT ( 'NONE',  ( -2.162160676586881955E-15, 50.87500000273119838, -35.31076352940723240 ) ) ;
#33631=( BOUNDED_CURVE ( )  B_SPLINE_CURVE ( 2, ( #30601, #18096, #23243, #7097, #33704, #30950, #10203, #28041, #25642, #15525, #1597, #17752, #12424 ),
 .UNSPECIFIED., .F., .T. ) 
 B_SPLINE_CURVE_WITH_KNOTS ( ( 3, 2, 2, 2, 2, 2, 3 ),
 ( 0.2500000000000000000, 0.2600000000000000089, 0.2800000000000000266, 0.2999999999999999889, 0.3200000000000000067, 0.3400000000000000244, 0.3500000000000000333 ),
 .UNSPECIFIED. ) 
 CURVE ( )  GEOMETRIC_REPRESENTATION_ITEM ( )  RATIONAL_B_SPLINE_CURVE ( ( 0.9755282581475768211, 0.9755282581475768211, 1.000000000000000000, 0.9510565162951535312, 1.000000000000000000, 0.9510565162951535312, 1.000000000000000000, 0.9510565162951535312, 1.000000000000000000, 0.9510565162951535312, 1.000000000000000000, 0.9755282581475767101, 0.9755282581475768211 ) ) 
 REPRESENTATION_ITEM ( '' )  );
#33633=CARTESIAN_POINT ( 'NONE',  ( 32.50000000000000000, 24.99999999999999289, -3.980102097228898626E-15 ) ) ;
#33635=CARTESIAN_POINT ( 'NONE',  ( 27.16883889988623935, 70.32500000273117280, -19.73931689729374384 ) ) ;
#33638=CARTESIAN_POINT ( 'NONE',  ( -27.16883889988623935, 59.57500000273119412, 19.73931689729374739 ) ) ;
#33640=AXIS2_PLACEMENT_3D ( 'NONE', #5670, #2239, #15981 ) ;
#33641=CARTESIAN_POINT ( 'NONE',  ( 32.50000000000000000, 73.00000000000001421, -3.980102097228898626E-15 ) ) ;
#33642=CARTESIAN_POINT ( 'NONE',  ( 27.16883889988624290, 13.92500000273116889, 19.73931689729373673 ) ) ;
#33643=CARTESIAN_POINT ( 'NONE',  ( 1.577395562988744260E-15, 12.24999999453763522, -25.76082449383753925 ) ) ;
#33653=CARTESIAN_POINT ( 'NONE',  ( 5.147494310547426899, 63.44874571845315359, -32.50000000000000000 ) ) ;
#33655=CARTESIAN_POINT ( 'NONE',  ( -1.778240108872766143E-15, 64.00000000546238255, -32.49999999999999289 ) ) ;
#33656=CARTESIAN_POINT ( 'NONE',  ( 26.29305231718579350, 73.30000000546237970, 19.10302069950537529 ) ) ;
#33660=ORIENTED_EDGE ( 'NONE', *, *, #27184, .T. ) ;
#33661=CARTESIAN_POINT ( 'NONE',  ( 20.75514604977249178, 76.07500000273118701, 28.56700777964553950 ) ) ;
#33666=CARTESIAN_POINT ( 'NONE',  ( -10.37757302488623701, 51.77500000273118985, 31.93888565452638417 ) ) ;
#33667=CARTESIAN_POINT ( 'NONE',  ( -32.50000000000000000, 60.50000000546237544, 0.000000000000000000 ) ) ;
#33669=CARTESIAN_POINT ( 'NONE',  ( -10.04305231718578462, 10.90000000546237402, 30.90933677959249337 ) ) ;
#33670=CARTESIAN_POINT ( 'NONE',  ( -27.16883889988623935, 43.32500000273120833, 19.73931689729374739 ) ) ;
#33671=CARTESIAN_POINT ( 'NONE',  ( -7.236395654485757944, 17.22499999726881370, -22.27133577429736988 ) ) ;
#33672=CARTESIAN_POINT ( 'NONE',  ( -20.75514604977248112, 65.67500000273118133, 28.56700777964554661 ) ) ;
#33673=CARTESIAN_POINT ( 'NONE',  ( -32.50000000000000000, 4.600000005462387520, 10.55989012756946366 ) ) ;
#33676=CARTESIAN_POINT ( 'NONE',  ( 20.08610463437157279, 47.29999999999999005, -27.64615127144129758 ) ) ;
#33678=CARTESIAN_POINT ( 'NONE',  ( -33.58253175000000113, 11.37500000273117351, 0.000000000000000000 ) ) ;
#33679=CARTESIAN_POINT ( 'NONE',  ( 0.000000000000000000, 82.00000000000001421, -15.00000000000000000 ) ) ;
#33681=CARTESIAN_POINT ( 'NONE',  ( 13.91746824999999532, 80.47500000273119269, -4.522059556121118540 ) ) ;
#33682=CARTESIAN_POINT ( 'NONE',  ( -2.162160676586882350E-15, 76.87500000273115575, -35.31076352940722529 ) ) ;
#33683=FACE_OUTER_BOUND ( 'NONE', #15871, .T. ) ;
#33685=ORIENTED_EDGE ( 'NONE', *, *, #11771, .T. ) ;
#33695=EDGE_CURVE ( 'NONE', #33138, #27031, #12475, .T. ) ;
#33700=CARTESIAN_POINT ( 'NONE',  ( -20.75514604977248112, 45.42500000273118843, 28.56700777964554661 ) ) ;
#33704=CARTESIAN_POINT ( 'NONE',  ( 12.13525491562420910, 79.19999999999998863, -8.816778784387098611 ) ) ;
#33709=CARTESIAN_POINT ( 'NONE',  ( -10.37757302488623701, 75.77500000273118985, 31.93888565452638417 ) ) ;
#33710=VERTEX_POINT ( 'NONE', #21235 ) ;
#33712=EDGE_CURVE ( 'NONE', #3815, #22014, #25856, .T. ) ;
#33717=CARTESIAN_POINT ( 'NONE',  ( -10.37757302488624411, 60.72500000273117848, -31.93888565452638417 ) ) ;
#33720=CARTESIAN_POINT ( 'NONE',  ( 18.94512977948576093, 3.324999997268818230, -13.76444248337722875 ) ) ;
#33721=CARTESIAN_POINT ( 'NONE',  ( 10.37757302488624767, 3.725000002731182480, 31.93888565452638417 ) ) ;
#33722=CARTESIAN_POINT ( 'NONE',  ( -15.14183272437242778, 7.049999994537622605, 20.84094480462497856 ) ) ;
#33724=CARTESIAN_POINT ( 'NONE',  ( -15.00000000000000000, 74.00000000000001421, 0.000000000000000000 ) ) ;
#33725=DIRECTION ( 'NONE',  ( -0.000000000000000000, -1.000000000000000000, -0.000000000000000000 ) ) ;
#33729=CARTESIAN_POINT ( 'NONE',  ( 11.25946833292375793, 80.07500000273121543, -8.180482586598735395 ) ) ;
#33731=CARTESIAN_POINT ( 'NONE',  ( 6.486482029760649416E-15, 33.62500000273119127, 35.31076352940723240 ) ) ;
#33732=AXIS2_PLACEMENT_3D ( 'NONE', #31362, #18513, #29291 ) ;
#33735=CARTESIAN_POINT ( 'NONE',  ( 20.75514604977249178, 24.07500000273120477, 28.56700777964553950 ) ) ;
#33736=CARTESIAN_POINT ( 'NONE',  ( -26.29305231718578995, 64.20000000000000284, 19.10302069950538595 ) ) ;
#33737=CARTESIAN_POINT ( 'NONE',  ( -2.162160676586882350E-15, 78.62500000273116996, -35.31076352940722529 ) ) ;
#33739=DIRECTION ( 'NONE',  ( -0.000000000000000000, -1.000000000000000000, -0.000000000000000000 ) ) ;
#33742=CARTESIAN_POINT ( 'NONE',  ( 7.236395654485755280, 18.22499999726881370, 22.27133577429736988 ) ) ;
#33743=CARTESIAN_POINT ( 'NONE',  ( 20.75514604977249178, 61.82500000273117280, 28.56700777964553950 ) ) ;
#33746=CARTESIAN_POINT ( 'NONE',  ( -27.16883889988623935, 7.325000002731174575, 19.73931689729374739 ) ) ;
#33748=CARTESIAN_POINT ( 'NONE',  ( 7.236395654485755280, 16.72499999726881370, 22.27133577429736988 ) ) ;
#33751=VERTEX_POINT ( 'NONE', #10924 ) ;
#33753=EDGE_LOOP ( 'NONE', ( #30015, #12468, #19440, #7871, #10833, #17521, #8244, #7210, #12605, #10208, #28765, #7792, #3151, #33135 ) ) ;
#33755=VERTEX_POINT ( 'NONE', #23971 ) ;
#33759=CARTESIAN_POINT ( 'NONE',  ( 10.37757302488624056, 78.52500000273118985, -31.93888565452638417 ) ) ;
#33760=CARTESIAN_POINT ( 'NONE',  ( -4.523095164977116484E-15, 2.624999997268825158, 24.62258325217400312 ) ) ;
#33761=CARTESIAN_POINT ( 'NONE',  ( 19.82091636218621389, 2.200000000000007283, -14.40073868116559197 ) ) ;
#33762=CARTESIAN_POINT ( 'NONE',  ( 33.58253175000000113, 18.47500000273117848, -10.91162601494193751 ) ) ;
#33763=CARTESIAN_POINT ( 'NONE',  ( -26.29305231718579350, 18.30000000546239036, -19.10302069950537884 ) ) ;
#33764=CARTESIAN_POINT ( 'NONE',  ( 32.50000000000000000, 63.00000000000000000, -3.980102097228898626E-15 ) ) ;
#33766=CARTESIAN_POINT ( 'NONE',  ( 0.000000000000000000, 0.000000000000000000, 0.000000000000000000 ) ) ;
#33768=CARTESIAN_POINT ( 'NONE',  ( 4.300734207923757602, 80.77500000273118985, -13.23629886949340673 ) ) ;
#33771=DIRECTION ( 'NONE',  ( 0.000000000000000000, 0.000000000000000000, -1.000000000000000000 ) ) ;
#33772=CARTESIAN_POINT ( 'NONE',  ( -7.236395654485763274, 18.52499999726881086, 22.27133577429736633 ) ) ;
#33773=CARTESIAN_POINT ( 'NONE',  ( -32.50000000000000000, 5.899999999999987921, -10.55989012756945478 ) ) ;
#33776=CARTESIAN_POINT ( 'NONE',  ( 10.37757302488624056, 52.52500000273118985, -31.93888565452638417 ) ) ;
#33778=CARTESIAN_POINT ( 'NONE',  ( 20.75514604977249178, 42.07500000273118701, 28.56700777964553950 ) ) ;
#33779=PLANE ( 'NONE',  #33732 ) ;
#33785=CARTESIAN_POINT ( 'NONE',  ( -32.50000000000000000, 62.40000000546236691, -10.55989012756945300 ) ) ;
#33790=CARTESIAN_POINT ( 'NONE',  ( -5.147494310547430452, 11.55125428154683753, -32.49999999999999289 ) ) ;
#33791=CARTESIAN_POINT ( 'NONE',  ( 27.16883889988624290, 27.92500000273118133, 19.73931689729373673 ) ) ;
#33793=ORIENTED_EDGE ( 'NONE', *, *, #20502, .T. ) ;
#33800=EDGE_CURVE ( 'NONE', #25557, #29691, #8337, .T. ) ;
#33803=CARTESIAN_POINT ( 'NONE',  ( -2.162160676586881955E-15, 34.87500000273117706, -35.31076352940723240 ) ) ;
#33804=CARTESIAN_POINT ( 'NONE',  ( 20.08610463437157279, 39.80000000546238681, -27.64615127144129758 ) ) ;
#33806=CARTESIAN_POINT ( 'NONE',  ( -33.58253175000000113, 21.12500000273118062, 0.000000000000000000 ) ) ;
#33808=CARTESIAN_POINT ( 'NONE',  ( -27.16883889988624290, 51.17500000273117422, -19.73931689729374028 ) ) ;
#33811=CARTESIAN_POINT ( 'NONE',  ( 20.08610463437158344, 26.70000000000000284, 27.64615127144129403 ) ) ;
#33813=CARTESIAN_POINT ( 'NONE',  ( 10.37757302488624767, 69.72500000273117848, 31.93888565452638417 ) ) ;
#33815=CARTESIAN_POINT ( 'NONE',  ( 1.555960095263670572E-15, 14.50000000000000178, -24.50000000000000000 ) ) ;
#33816=CARTESIAN_POINT ( 'NONE',  ( 20.75514604977248467, 60.67500000273118133, -28.56700777964554305 ) ) ;
#33817=CARTESIAN_POINT ( 'NONE',  ( -33.58253175000000113, 11.12500000273120015, 0.000000000000000000 ) ) ;
#33828=FACE_OUTER_BOUND ( 'NONE', #17915, .T. ) ;
#33829=VECTOR ( 'NONE', #17413, 1000.000000000000000 ) ;
#33830=CARTESIAN_POINT ( 'NONE',  ( -32.50000000000000000, 66.60000000546236265, 10.55989012756946366 ) ) ;
#33834=ORIENTED_EDGE ( 'NONE', *, *, #8918, .F. ) ;
#33835=CARTESIAN_POINT ( 'NONE',  ( -20.75514604977248823, 75.07500000273118701, -28.56700777964554305 ) ) ;
#33839=EDGE_CURVE ( 'NONE', #25478, #20831, #19897, .T. ) ;
#33840=CARTESIAN_POINT ( 'NONE',  ( 33.58253175000000823, 54.27500000273118275, 10.91162601494192863 ) ) ;
#33841=EDGE_CURVE ( 'NONE', #29096, #12812, #4561, .T. ) ;
#33842=CARTESIAN_POINT ( 'NONE',  ( 32.50000000000000000, 57.60000000546237686, -10.55989012756945833 ) ) ;
#33844=CARTESIAN_POINT ( 'NONE',  ( 10.37757302488624767, 41.72500000273118559, 31.93888565452638417 ) ) ;
#33845=CARTESIAN_POINT ( 'NONE',  ( -15.00000000000000000, 72.09999999999999432, 4.873795443493597723 ) ) ;
#33846=CARTESIAN_POINT ( 'NONE',  ( 27.16883889988623935, 66.57500000273120122, -19.73931689729374384 ) ) ;
#33847=CARTESIAN_POINT ( 'NONE',  ( -32.50000000000000000, 8.400000005462384678, -10.55989012756945478 ) ) ;
#33850=CARTESIAN_POINT ( 'NONE',  ( 10.04305231718578817, 47.39999999999999858, -30.90933677959249337 ) ) ;
#33852=CARTESIAN_POINT ( 'NONE',  ( 33.58253175000000113, 12.37500000273117351, -4.112674001490185761E-15 ) ) ;
#33853=FACE_OUTER_BOUND ( 'NONE', #22051, .T. ) ;
#33855=CARTESIAN_POINT ( 'NONE',  ( -11.25946833292375793, 77.17500000273119554, -8.180482586598733619 ) ) ;
#33856=FACE_OUTER_BOUND ( 'NONE', #22420, .T. ) ;
#33859=ORIENTED_EDGE ( 'NONE', *, *, #741, .T. ) ;
#33862=ADVANCED_FACE ( 'NONE', ( #5265 ), #32610, .F. ) ;
#33870=CARTESIAN_POINT ( 'NONE',  ( 0.000000000000000000, 80.00000000000001421, 0.000000000000000000 ) ) ;
#33871=CARTESIAN_POINT ( 'NONE',  ( 10.37757302488624767, 45.72500000273119269, 31.93888565452638417 ) ) ;
#33878=CARTESIAN_POINT ( 'NONE',  ( -2.162160676586881955E-15, 76.87500000273115575, -35.31076352940723240 ) ) ;
#33879=VERTEX_POINT ( 'NONE', #18243 ) ;
#33884=CARTESIAN_POINT ( 'NONE',  ( -32.50000000000000000, 14.60000000546239107, 10.55989012756946366 ) ) ;
#33885=CARTESIAN_POINT ( 'NONE',  ( -33.58253175000000113, 63.12500000273119127, 0.000000000000000000 ) ) ;
#33887=CARTESIAN_POINT ( 'NONE',  ( 24.50000000000000000, 18.00000000000001421, 0.000000000000000000 ) ) ;
#33888=CARTESIAN_POINT ( 'NONE',  ( -23.41746824999999887, 2.124999997268811391, -2.867812753649727150E-15 ) ) ;
#33889=CARTESIAN_POINT ( 'NONE',  ( 20.75514604977248467, 2.425000002731189763, -28.56700777964554305 ) ) ;
#33892=CARTESIAN_POINT ( 'NONE',  ( 27.16883889988623935, 78.57500000273121543, -19.73931689729374384 ) ) ;
#33894=CARTESIAN_POINT ( 'NONE',  ( 5.147494310547434893, 8.551254281546841085, 32.49999999999999289 ) ) ;
#33899=CARTESIAN_POINT ( 'NONE',  ( -13.91746824999999887, 80.87500000273118417, 0.000000000000000000 ) ) ;
#33901=CARTESIAN_POINT ( 'NONE',  ( -33.58253175000000113, 31.22500000273118559, 10.91162601494193929 ) ) ;
#33904=CARTESIAN_POINT ( 'NONE',  ( -33.58253175000000113, 13.47500000273118914, 10.91162601494193929 ) ) ;
#33908=CARTESIAN_POINT ( 'NONE',  ( -33.58253175000000113, 75.12500000273119838, 0.000000000000000000 ) ) ;
#33909=CARTESIAN_POINT ( 'NONE',  ( -10.04305231718578462, 66.40000000000001990, 30.90933677959249337 ) ) ;
#33911=CARTESIAN_POINT ( 'NONE',  ( 3.980102097228898626E-15, 80.00000000000001421, 32.50000000000000000 ) ) ;
#33912=CARTESIAN_POINT ( 'NONE',  ( 10.37757302488624767, 61.72500000273117848, 31.93888565452638417 ) ) ;
#33916=CARTESIAN_POINT ( 'NONE',  ( -33.58253175000000113, 5.125000002731194826, 0.000000000000000000 ) ) ;
#33917=CARTESIAN_POINT ( 'NONE',  ( 23.41746824999999887, 2.624999997268812280, 0.000000000000000000 ) ) ;
#33919=ORIENTED_EDGE ( 'NONE', *, *, #19161, .T. ) ;
#33925=CARTESIAN_POINT ( 'NONE',  ( 10.37757302488624767, 77.72500000273119269, 31.93888565452638417 ) ) ;
#33926=CARTESIAN_POINT ( 'NONE',  ( 1.507698388325705758E-15, 5.624999997268818497, -24.62258325217400312 ) ) ;
#33927=CARTESIAN_POINT ( 'NONE',  ( -14.47279130897152122, 15.92499999726881121, 19.92008829642072243 ) ) ;
#33928=CARTESIAN_POINT ( 'NONE',  ( -27.16883889988624290, 13.17500000273119554, -19.73931689729374028 ) ) ;
#33929=CARTESIAN_POINT ( 'NONE',  ( 32.50000000000000000, 61.09999999999998721, -10.55989012756945833 ) ) ;
#33930=CARTESIAN_POINT ( 'NONE',  ( 9.270509831248425314, 76.95000000546239960, 12.75976212528059683 ) ) ;
#33931=CARTESIAN_POINT ( 'NONE',  ( -26.29305231718579350, 29.79999999999999361, -19.10302069950537884 ) ) ;
#33933=CARTESIAN_POINT ( 'NONE',  ( -4.300734207923755825, 75.77500000273118985, 13.23629886949340673 ) ) ;
#33936=FACE_OUTER_BOUND ( 'NONE', #28978, .T. ) ;
#33937=CARTESIAN_POINT ( 'NONE',  ( 10.04305231718579705, 64.59999999999999432, 30.90933677959248982 ) ) ;
#33938=CARTESIAN_POINT ( 'NONE',  ( 26.29305231718579350, 10.80000000000000426, 19.10302069950537529 ) ) ;
#33939=CARTESIAN_POINT ( 'NONE',  ( -9.270509831248423538, 73.70000000000000284, -12.75976212528059861 ) ) ;
#33941=( BOUNDED_CURVE ( )  B_SPLINE_CURVE ( 2, ( #6673, #7010, #27782, #22976, #4099, #28292, #25033, #14573, #14742, #1513, #12335, #9932, #4437 ),
 .UNSPECIFIED., .F., .T. ) 
 B_SPLINE_CURVE_WITH_KNOTS ( ( 3, 2, 2, 2, 2, 2, 3 ),
 ( 0.8499999999999999778, 0.8599999999999999867, 0.8800000000000000044, 0.9000000000000000222, 0.9200000000000000400, 0.9399999999999999467, 0.9499999999999999556 ),
 .UNSPECIFIED. ) 
 CURVE ( )  GEOMETRIC_REPRESENTATION_ITEM ( )  RATIONAL_B_SPLINE_CURVE ( ( 0.9755282581475768211, 0.9755282581475768211, 1.000000000000000000, 0.9510565162951535312, 1.000000000000000000, 0.9510565162951535312, 1.000000000000000000, 0.9510565162951535312, 1.000000000000000000, 0.9510565162951535312, 1.000000000000000000, 0.9755282581475768211, 0.9755282581475768211 ) ) 
 REPRESENTATION_ITEM ( '' )  );
#33942=CARTESIAN_POINT ( 'NONE',  ( 20.75514604977248467, 52.42500000273118133, -28.56700777964554305 ) ) ;
#33944=CARTESIAN_POINT ( 'NONE',  ( 10.37757302488624767, 43.97500000273119269, 31.93888565452638417 ) ) ;
#33946=CARTESIAN_POINT ( 'NONE',  ( -1.778240108872766143E-15, 5.500000000000003553, -32.49999999999999289 ) ) ;
#33951=DIRECTION ( 'NONE',  ( 0.000000000000000000, 0.000000000000000000, -1.000000000000000000 ) ) ;
#33954=CARTESIAN_POINT ( 'NONE',  ( -15.14183272437242778, 11.04999999453761284, 20.84094480462497856 ) ) ;
#33955=CARTESIAN_POINT ( 'NONE',  ( -33.58253175000000113, 25.02500000273117564, -10.91162601494193041 ) ) ;
#33957=ORIENTED_EDGE ( 'NONE', *, *, #14925, .T. ) ;
#33960=VERTEX_POINT ( 'NONE', #695 ) ;
#33965=DIRECTION ( 'NONE',  ( 0.000000000000000000, 0.000000000000000000, -1.000000000000000000 ) ) ;
#33966=CARTESIAN_POINT ( 'NONE',  ( -33.58253175000000113, 35.47500000273118559, 10.91162601494193929 ) ) ;
#33967=CARTESIAN_POINT ( 'NONE',  ( -26.29305231718578995, 36.70000000546236407, 19.10302069950538595 ) ) ;
#33970=CARTESIAN_POINT ( 'NONE',  ( -2.162160676586881955E-15, 20.62500000273119483, -35.31076352940723240 ) ) ;
#33972=CARTESIAN_POINT ( 'NONE',  ( -20.75514604977248112, 47.67500000273118843, 28.56700777964554661 ) ) ;
#33975=CARTESIAN_POINT ( 'NONE',  ( -26.29305231718579350, 25.79999999999999005, -19.10302069950537884 ) ) ;
#33977=CARTESIAN_POINT ( 'NONE',  ( 10.37757302488624056, 70.52500000273120406, -31.93888565452638417 ) ) ;
#33980=CARTESIAN_POINT ( 'NONE',  ( -20.75514604977248112, 59.67500000273118133, 28.56700777964554661 ) ) ;
#33982=CARTESIAN_POINT ( 'NONE',  ( -27.16883889988623935, 11.32500000273117813, 19.73931689729374739 ) ) ;
#33986=CARTESIAN_POINT ( 'NONE',  ( -27.16883889988623935, 5.575000002731201221, 19.73931689729374739 ) ) ;
#33989=CARTESIAN_POINT ( 'NONE',  ( 20.08610463437158344, 67.20000000546235697, 27.64615127144129403 ) ) ;
ENDSEC;
END-ISO-10303-21;
